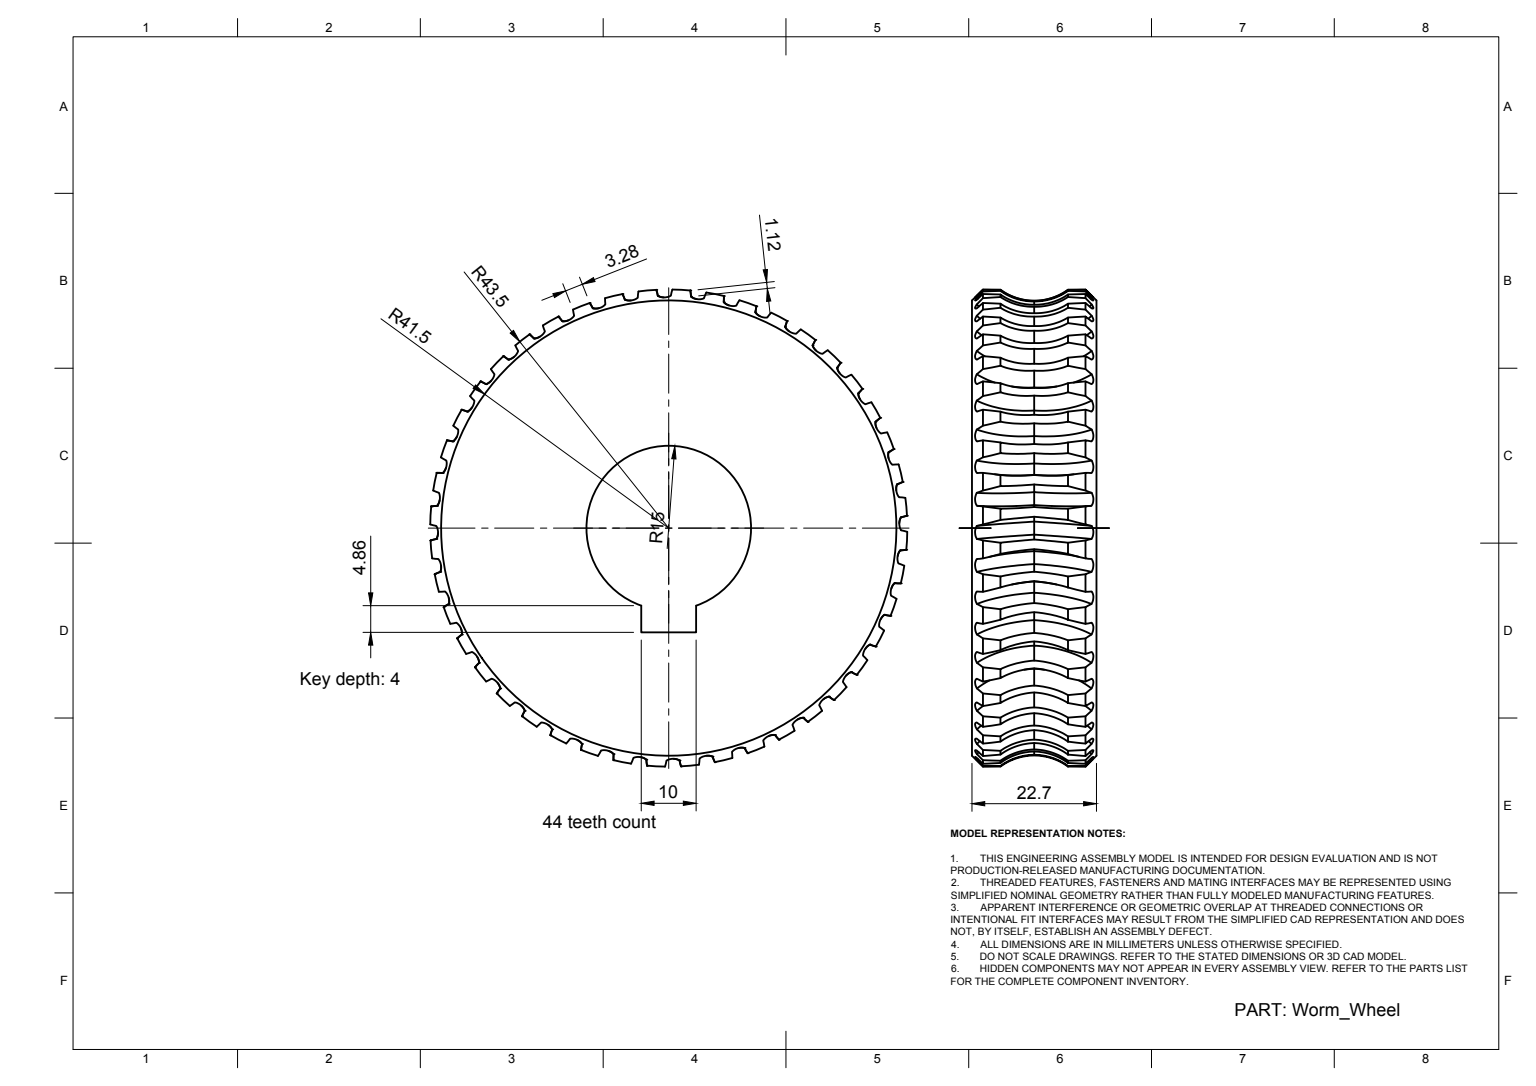
ISO-10303-21;
HEADER;
/* Generated by software containing ST-Developer
 * from STEP Tools, Inc. (www.steptools.com) 
 */

FILE_DESCRIPTION(
/* description */ ('STEP AP214'),
/* implementation_level */ '2;1');

FILE_NAME(
/* name */ 'Worm_Wheel.step',
/* time_stamp */ '2026-10-05T13:15:56-07:00',
/* author */ (''),
/* organization */ (''),
/* preprocessor_version */ 'ST-DEVELOPER v20.2',
/* originating_system */ 'Autodesk Translation Framework v15.15.0.0',
/* authorisation */ '');

FILE_SCHEMA (('AUTOMOTIVE_DESIGN { 1 0 10303 214 3 1 1 }'));
ENDSEC;

DATA;
#10=MECHANICAL_DESIGN_GEOMETRIC_PRESENTATION_REPRESENTATION('',(#1348),#37881);
#183=TOROIDAL_SURFACE('',#11111,52.,10.5);
#184=TOROIDAL_SURFACE('',#11114,52.,10.5);
#185=TOROIDAL_SURFACE('',#11117,52.,10.5);
#186=TOROIDAL_SURFACE('',#11120,52.,10.5);
#187=TOROIDAL_SURFACE('',#11123,52.,10.5);
#188=TOROIDAL_SURFACE('',#11126,52.,10.5);
#189=TOROIDAL_SURFACE('',#11129,52.,10.5);
#190=TOROIDAL_SURFACE('',#11132,52.,10.5);
#191=TOROIDAL_SURFACE('',#11135,52.,10.5);
#192=TOROIDAL_SURFACE('',#11138,52.,10.5);
#193=TOROIDAL_SURFACE('',#11141,52.,10.5);
#194=TOROIDAL_SURFACE('',#11144,52.,10.5);
#195=TOROIDAL_SURFACE('',#11147,52.,10.5);
#196=TOROIDAL_SURFACE('',#11150,52.,10.5);
#197=TOROIDAL_SURFACE('',#11153,52.,10.5);
#198=TOROIDAL_SURFACE('',#11156,52.,10.5);
#199=TOROIDAL_SURFACE('',#11159,52.,10.5);
#200=TOROIDAL_SURFACE('',#11162,52.,10.5);
#201=TOROIDAL_SURFACE('',#11165,52.,10.5);
#202=TOROIDAL_SURFACE('',#11168,52.,10.5);
#203=TOROIDAL_SURFACE('',#11171,52.,10.5);
#204=TOROIDAL_SURFACE('',#11174,52.,10.5);
#205=TOROIDAL_SURFACE('',#11177,52.,10.5);
#206=TOROIDAL_SURFACE('',#11180,52.,10.5);
#207=TOROIDAL_SURFACE('',#11183,52.,10.5);
#208=TOROIDAL_SURFACE('',#11186,52.,10.5);
#209=TOROIDAL_SURFACE('',#11189,52.,10.5);
#210=TOROIDAL_SURFACE('',#11192,52.,10.5);
#211=TOROIDAL_SURFACE('',#11195,52.,10.5);
#212=TOROIDAL_SURFACE('',#11198,52.,10.5);
#213=TOROIDAL_SURFACE('',#11201,52.,10.5);
#214=TOROIDAL_SURFACE('',#11204,52.,10.5);
#215=TOROIDAL_SURFACE('',#11207,52.,10.5);
#216=TOROIDAL_SURFACE('',#11210,52.,10.5);
#217=TOROIDAL_SURFACE('',#11213,52.,10.5);
#218=TOROIDAL_SURFACE('',#11216,52.,10.5);
#219=TOROIDAL_SURFACE('',#11219,52.,10.5);
#220=TOROIDAL_SURFACE('',#11222,52.,10.5);
#221=TOROIDAL_SURFACE('',#11225,52.,10.5);
#222=TOROIDAL_SURFACE('',#11228,52.,10.5);
#223=TOROIDAL_SURFACE('',#11231,52.,10.5);
#224=TOROIDAL_SURFACE('',#11234,52.,10.5);
#225=TOROIDAL_SURFACE('',#11237,52.,10.5);
#226=TOROIDAL_SURFACE('',#11240,52.,10.5);
#232=(
BOUNDED_CURVE()
B_SPLINE_CURVE(2,(#22947,#22948,#22949,#22950,#22951),.UNSPECIFIED.,.F.,
 .F.)
B_SPLINE_CURVE_WITH_KNOTS((3,2,3),(0.,0.25,0.459577358091282),
 .UNSPECIFIED.)
CURVE()
GEOMETRIC_REPRESENTATION_ITEM()
RATIONAL_B_SPLINE_CURVE((1.,0.974927912181824,1.,0.978981832292936,0.9932031210656))
REPRESENTATION_ITEM('')
);
#233=(
BOUNDED_CURVE()
B_SPLINE_CURVE(3,(#23082,#23083,#23084,#23085,#23086,#23087,#23088,#23089),
 .UNSPECIFIED.,.F.,.F.)
B_SPLINE_CURVE_WITH_KNOTS((4,2,2,4),(0.0783698293107414,0.308777371982556,
0.539184914655036,0.563918778704656),.UNSPECIFIED.)
CURVE()
GEOMETRIC_REPRESENTATION_ITEM()
RATIONAL_B_SPLINE_CURVE((1.,1.,1.,1.,1.,1.,1.,1.))
REPRESENTATION_ITEM('')
);
#234=(
BOUNDED_CURVE()
B_SPLINE_CURVE(2,(#23313,#23314,#23315,#23316,#23317),.UNSPECIFIED.,.F.,
 .F.)
B_SPLINE_CURVE_WITH_KNOTS((3,2,3),(0.,0.25,0.459577358091282),
 .UNSPECIFIED.)
CURVE()
GEOMETRIC_REPRESENTATION_ITEM()
RATIONAL_B_SPLINE_CURVE((1.,0.974927912181824,1.,0.978981832292936,0.9932031210656))
REPRESENTATION_ITEM('')
);
#235=(
BOUNDED_CURVE()
B_SPLINE_CURVE(2,(#23485,#23486,#23487,#23488,#23489),.UNSPECIFIED.,.F.,
 .F.)
B_SPLINE_CURVE_WITH_KNOTS((3,2,3),(0.,0.25,0.459577358091281),
 .UNSPECIFIED.)
CURVE()
GEOMETRIC_REPRESENTATION_ITEM()
RATIONAL_B_SPLINE_CURVE((1.,0.974927912181824,1.,0.978981832292936,0.9932031210656))
REPRESENTATION_ITEM('')
);
#236=(
BOUNDED_CURVE()
B_SPLINE_CURVE(2,(#23568,#23569,#23570,#23571,#23572),.UNSPECIFIED.,.F.,
 .F.)
B_SPLINE_CURVE_WITH_KNOTS((3,2,3),(0.,0.25,0.460808762537663),
 .UNSPECIFIED.)
CURVE()
GEOMETRIC_REPRESENTATION_ITEM()
RATIONAL_B_SPLINE_CURVE((1.,0.974927912181824,1.,0.978858336771259,0.993371456448429))
REPRESENTATION_ITEM('')
);
#237=(
BOUNDED_CURVE()
B_SPLINE_CURVE(2,(#23610,#23611,#23612,#23613,#23614),.UNSPECIFIED.,.F.,
 .F.)
B_SPLINE_CURVE_WITH_KNOTS((3,2,3),(0.,0.25,0.459577358091282),
 .UNSPECIFIED.)
CURVE()
GEOMETRIC_REPRESENTATION_ITEM()
RATIONAL_B_SPLINE_CURVE((1.,0.974927912181824,1.,0.978981832292936,0.9932031210656))
REPRESENTATION_ITEM('')
);
#238=(
BOUNDED_CURVE()
B_SPLINE_CURVE(2,(#23782,#23783,#23784,#23785,#23786),.UNSPECIFIED.,.F.,
 .F.)
B_SPLINE_CURVE_WITH_KNOTS((3,2,3),(0.,0.25,0.459577358091282),
 .UNSPECIFIED.)
CURVE()
GEOMETRIC_REPRESENTATION_ITEM()
RATIONAL_B_SPLINE_CURVE((1.,0.974927912181824,1.,0.978981832292936,0.9932031210656))
REPRESENTATION_ITEM('')
);
#239=(
BOUNDED_CURVE()
B_SPLINE_CURVE(2,(#23954,#23955,#23956,#23957,#23958),.UNSPECIFIED.,.F.,
 .F.)
B_SPLINE_CURVE_WITH_KNOTS((3,2,3),(0.,0.25,0.459577358091282),
 .UNSPECIFIED.)
CURVE()
GEOMETRIC_REPRESENTATION_ITEM()
RATIONAL_B_SPLINE_CURVE((1.,0.974927912181824,1.,0.978981832292936,0.9932031210656))
REPRESENTATION_ITEM('')
);
#240=(
BOUNDED_CURVE()
B_SPLINE_CURVE(2,(#24126,#24127,#24128,#24129,#24130),.UNSPECIFIED.,.F.,
 .F.)
B_SPLINE_CURVE_WITH_KNOTS((3,2,3),(0.,0.25,0.459577358091283),
 .UNSPECIFIED.)
CURVE()
GEOMETRIC_REPRESENTATION_ITEM()
RATIONAL_B_SPLINE_CURVE((1.,0.974927912181824,1.,0.978981832292936,0.9932031210656))
REPRESENTATION_ITEM('')
);
#241=(
BOUNDED_CURVE()
B_SPLINE_CURVE(2,(#24298,#24299,#24300,#24301,#24302),.UNSPECIFIED.,.F.,
 .F.)
B_SPLINE_CURVE_WITH_KNOTS((3,2,3),(0.,0.25,0.459577358091282),
 .UNSPECIFIED.)
CURVE()
GEOMETRIC_REPRESENTATION_ITEM()
RATIONAL_B_SPLINE_CURVE((1.,0.974927912181824,1.,0.978981832292936,0.9932031210656))
REPRESENTATION_ITEM('')
);
#242=(
BOUNDED_CURVE()
B_SPLINE_CURVE(2,(#24470,#24471,#24472,#24473,#24474),.UNSPECIFIED.,.F.,
 .F.)
B_SPLINE_CURVE_WITH_KNOTS((3,2,3),(0.,0.25,0.459577358091282),
 .UNSPECIFIED.)
CURVE()
GEOMETRIC_REPRESENTATION_ITEM()
RATIONAL_B_SPLINE_CURVE((1.,0.974927912181824,1.,0.978981832292936,0.9932031210656))
REPRESENTATION_ITEM('')
);
#243=(
BOUNDED_CURVE()
B_SPLINE_CURVE(2,(#24642,#24643,#24644,#24645,#24646),.UNSPECIFIED.,.F.,
 .F.)
B_SPLINE_CURVE_WITH_KNOTS((3,2,3),(0.,0.25,0.459577358091282),
 .UNSPECIFIED.)
CURVE()
GEOMETRIC_REPRESENTATION_ITEM()
RATIONAL_B_SPLINE_CURVE((1.,0.974927912181824,1.,0.978981832292936,0.9932031210656))
REPRESENTATION_ITEM('')
);
#244=(
BOUNDED_CURVE()
B_SPLINE_CURVE(2,(#24814,#24815,#24816,#24817,#24818),.UNSPECIFIED.,.F.,
 .F.)
B_SPLINE_CURVE_WITH_KNOTS((3,2,3),(0.,0.25,0.459577358091282),
 .UNSPECIFIED.)
CURVE()
GEOMETRIC_REPRESENTATION_ITEM()
RATIONAL_B_SPLINE_CURVE((1.,0.974927912181824,1.,0.978981832292936,0.9932031210656))
REPRESENTATION_ITEM('')
);
#245=(
BOUNDED_CURVE()
B_SPLINE_CURVE(2,(#24986,#24987,#24988,#24989,#24990),.UNSPECIFIED.,.F.,
 .F.)
B_SPLINE_CURVE_WITH_KNOTS((3,2,3),(0.,0.25,0.459577358091283),
 .UNSPECIFIED.)
CURVE()
GEOMETRIC_REPRESENTATION_ITEM()
RATIONAL_B_SPLINE_CURVE((1.,0.974927912181824,1.,0.978981832292936,0.9932031210656))
REPRESENTATION_ITEM('')
);
#246=(
BOUNDED_CURVE()
B_SPLINE_CURVE(2,(#25069,#25070,#25071,#25072,#25073),.UNSPECIFIED.,.F.,
 .F.)
B_SPLINE_CURVE_WITH_KNOTS((3,2,3),(0.,0.25,0.460808762537663),
 .UNSPECIFIED.)
CURVE()
GEOMETRIC_REPRESENTATION_ITEM()
RATIONAL_B_SPLINE_CURVE((1.,0.974927912181824,1.,0.978858336771258,0.993371456448429))
REPRESENTATION_ITEM('')
);
#247=(
BOUNDED_CURVE()
B_SPLINE_CURVE(2,(#25111,#25112,#25113,#25114,#25115),.UNSPECIFIED.,.F.,
 .F.)
B_SPLINE_CURVE_WITH_KNOTS((3,2,3),(0.,0.25,0.459577358091282),
 .UNSPECIFIED.)
CURVE()
GEOMETRIC_REPRESENTATION_ITEM()
RATIONAL_B_SPLINE_CURVE((1.,0.974927912181824,1.,0.978981832292936,0.9932031210656))
REPRESENTATION_ITEM('')
);
#248=(
BOUNDED_CURVE()
B_SPLINE_CURVE(2,(#25283,#25284,#25285,#25286,#25287),.UNSPECIFIED.,.F.,
 .F.)
B_SPLINE_CURVE_WITH_KNOTS((3,2,3),(0.,0.25,0.459577358091282),
 .UNSPECIFIED.)
CURVE()
GEOMETRIC_REPRESENTATION_ITEM()
RATIONAL_B_SPLINE_CURVE((1.,0.974927912181824,1.,0.978981832292936,0.9932031210656))
REPRESENTATION_ITEM('')
);
#249=(
BOUNDED_CURVE()
B_SPLINE_CURVE(2,(#25455,#25456,#25457,#25458,#25459),.UNSPECIFIED.,.F.,
 .F.)
B_SPLINE_CURVE_WITH_KNOTS((3,2,3),(0.,0.25,0.459577358091283),
 .UNSPECIFIED.)
CURVE()
GEOMETRIC_REPRESENTATION_ITEM()
RATIONAL_B_SPLINE_CURVE((1.,0.974927912181824,1.,0.978981832292936,0.9932031210656))
REPRESENTATION_ITEM('')
);
#250=(
BOUNDED_CURVE()
B_SPLINE_CURVE(2,(#25537,#25538,#25539,#25540,#25541),.UNSPECIFIED.,.F.,
 .F.)
B_SPLINE_CURVE_WITH_KNOTS((3,2,3),(0.,0.0714285714285714,0.131307816597586),
 .UNSPECIFIED.)
CURVE()
GEOMETRIC_REPRESENTATION_ITEM()
RATIONAL_B_SPLINE_CURVE((1.,0.974927912181824,1.,0.978981832292909,0.993203121065636))
REPRESENTATION_ITEM('')
);
#251=(
BOUNDED_CURVE()
B_SPLINE_CURVE(2,(#25581,#25582,#25583,#25584,#25585),.UNSPECIFIED.,.F.,
 .F.)
B_SPLINE_CURVE_WITH_KNOTS((3,2,3),(0.,0.0714285714285714,0.131659646439332),
 .UNSPECIFIED.)
CURVE()
GEOMETRIC_REPRESENTATION_ITEM()
RATIONAL_B_SPLINE_CURVE((1.,0.974927912181824,1.,0.978858336771259,0.993371456448429))
REPRESENTATION_ITEM('')
);
#252=(
BOUNDED_CURVE()
B_SPLINE_CURVE(2,(#25752,#25753,#25754,#25755,#25756),.UNSPECIFIED.,.F.,
 .F.)
B_SPLINE_CURVE_WITH_KNOTS((3,2,3),(0.,0.25,0.459577358091283),
 .UNSPECIFIED.)
CURVE()
GEOMETRIC_REPRESENTATION_ITEM()
RATIONAL_B_SPLINE_CURVE((1.,0.974927912181824,1.,0.978981832292936,0.9932031210656))
REPRESENTATION_ITEM('')
);
#253=(
BOUNDED_CURVE()
B_SPLINE_CURVE(2,(#25924,#25925,#25926,#25927,#25928),.UNSPECIFIED.,.F.,
 .F.)
B_SPLINE_CURVE_WITH_KNOTS((3,2,3),(0.,0.25,0.459577358091282),
 .UNSPECIFIED.)
CURVE()
GEOMETRIC_REPRESENTATION_ITEM()
RATIONAL_B_SPLINE_CURVE((1.,0.974927912181824,1.,0.978981832292936,0.9932031210656))
REPRESENTATION_ITEM('')
);
#254=(
BOUNDED_CURVE()
B_SPLINE_CURVE(2,(#26096,#26097,#26098,#26099,#26100),.UNSPECIFIED.,.F.,
 .F.)
B_SPLINE_CURVE_WITH_KNOTS((3,2,3),(0.,0.25,0.459577358091282),
 .UNSPECIFIED.)
CURVE()
GEOMETRIC_REPRESENTATION_ITEM()
RATIONAL_B_SPLINE_CURVE((1.,0.974927912181824,1.,0.978981832292936,0.9932031210656))
REPRESENTATION_ITEM('')
);
#255=(
BOUNDED_CURVE()
B_SPLINE_CURVE(2,(#26268,#26269,#26270,#26271,#26272),.UNSPECIFIED.,.F.,
 .F.)
B_SPLINE_CURVE_WITH_KNOTS((3,2,3),(0.,0.25,0.459577358091282),
 .UNSPECIFIED.)
CURVE()
GEOMETRIC_REPRESENTATION_ITEM()
RATIONAL_B_SPLINE_CURVE((1.,0.974927912181824,1.,0.978981832292936,0.9932031210656))
REPRESENTATION_ITEM('')
);
#256=(
BOUNDED_CURVE()
B_SPLINE_CURVE(2,(#26440,#26441,#26442,#26443,#26444),.UNSPECIFIED.,.F.,
 .F.)
B_SPLINE_CURVE_WITH_KNOTS((3,2,3),(0.,0.25,0.459577358091282),
 .UNSPECIFIED.)
CURVE()
GEOMETRIC_REPRESENTATION_ITEM()
RATIONAL_B_SPLINE_CURVE((1.,0.974927912181824,1.,0.978981832292936,0.9932031210656))
REPRESENTATION_ITEM('')
);
#257=(
BOUNDED_CURVE()
B_SPLINE_CURVE(2,(#26612,#26613,#26614,#26615,#26616),.UNSPECIFIED.,.F.,
 .F.)
B_SPLINE_CURVE_WITH_KNOTS((3,2,3),(0.,0.25,0.459577358091282),
 .UNSPECIFIED.)
CURVE()
GEOMETRIC_REPRESENTATION_ITEM()
RATIONAL_B_SPLINE_CURVE((1.,0.974927912181824,1.,0.978981832292936,0.9932031210656))
REPRESENTATION_ITEM('')
);
#258=(
BOUNDED_CURVE()
B_SPLINE_CURVE(2,(#26784,#26785,#26786,#26787,#26788),.UNSPECIFIED.,.F.,
 .F.)
B_SPLINE_CURVE_WITH_KNOTS((3,2,3),(0.,0.25,0.459577358091282),
 .UNSPECIFIED.)
CURVE()
GEOMETRIC_REPRESENTATION_ITEM()
RATIONAL_B_SPLINE_CURVE((1.,0.974927912181824,1.,0.978981832292936,0.9932031210656))
REPRESENTATION_ITEM('')
);
#259=(
BOUNDED_CURVE()
B_SPLINE_CURVE(2,(#26956,#26957,#26958,#26959,#26960),.UNSPECIFIED.,.F.,
 .F.)
B_SPLINE_CURVE_WITH_KNOTS((3,2,3),(0.,0.25,0.459577358091282),
 .UNSPECIFIED.)
CURVE()
GEOMETRIC_REPRESENTATION_ITEM()
RATIONAL_B_SPLINE_CURVE((1.,0.974927912181824,1.,0.978981832292936,0.9932031210656))
REPRESENTATION_ITEM('')
);
#260=(
BOUNDED_CURVE()
B_SPLINE_CURVE(2,(#27128,#27129,#27130,#27131,#27132),.UNSPECIFIED.,.F.,
 .F.)
B_SPLINE_CURVE_WITH_KNOTS((3,2,3),(0.,0.25,0.459577358091283),
 .UNSPECIFIED.)
CURVE()
GEOMETRIC_REPRESENTATION_ITEM()
RATIONAL_B_SPLINE_CURVE((1.,0.974927912181824,1.,0.978981832292936,0.9932031210656))
REPRESENTATION_ITEM('')
);
#261=(
BOUNDED_CURVE()
B_SPLINE_CURVE(2,(#27211,#27212,#27213,#27214,#27215),.UNSPECIFIED.,.F.,
 .F.)
B_SPLINE_CURVE_WITH_KNOTS((3,2,3),(0.,0.25,0.460808762537664),
 .UNSPECIFIED.)
CURVE()
GEOMETRIC_REPRESENTATION_ITEM()
RATIONAL_B_SPLINE_CURVE((1.,0.974927912181824,1.,0.978858336771258,0.993371456448429))
REPRESENTATION_ITEM('')
);
#262=(
BOUNDED_CURVE()
B_SPLINE_CURVE(2,(#27253,#27254,#27255,#27256,#27257),.UNSPECIFIED.,.F.,
 .F.)
B_SPLINE_CURVE_WITH_KNOTS((3,2,3),(0.,0.25,0.459577358091283),
 .UNSPECIFIED.)
CURVE()
GEOMETRIC_REPRESENTATION_ITEM()
RATIONAL_B_SPLINE_CURVE((1.,0.974927912181824,1.,0.978981832292936,0.9932031210656))
REPRESENTATION_ITEM('')
);
#263=(
BOUNDED_CURVE()
B_SPLINE_CURVE(2,(#27336,#27337,#27338,#27339,#27340),.UNSPECIFIED.,.F.,
 .F.)
B_SPLINE_CURVE_WITH_KNOTS((3,2,3),(0.,0.25,0.460808762537663),
 .UNSPECIFIED.)
CURVE()
GEOMETRIC_REPRESENTATION_ITEM()
RATIONAL_B_SPLINE_CURVE((1.,0.974927912181824,1.,0.978858336771258,0.993371456448429))
REPRESENTATION_ITEM('')
);
#264=(
BOUNDED_CURVE()
B_SPLINE_CURVE(2,(#27378,#27379,#27380,#27381,#27382),.UNSPECIFIED.,.F.,
 .F.)
B_SPLINE_CURVE_WITH_KNOTS((3,2,3),(0.,0.25,0.459577358091282),
 .UNSPECIFIED.)
CURVE()
GEOMETRIC_REPRESENTATION_ITEM()
RATIONAL_B_SPLINE_CURVE((1.,0.974927912181824,1.,0.978981832292936,0.9932031210656))
REPRESENTATION_ITEM('')
);
#265=(
BOUNDED_CURVE()
B_SPLINE_CURVE(2,(#27550,#27551,#27552,#27553,#27554),.UNSPECIFIED.,.F.,
 .F.)
B_SPLINE_CURVE_WITH_KNOTS((3,2,3),(0.,0.25,0.459577358091282),
 .UNSPECIFIED.)
CURVE()
GEOMETRIC_REPRESENTATION_ITEM()
RATIONAL_B_SPLINE_CURVE((1.,0.974927912181824,1.,0.978981832292936,0.9932031210656))
REPRESENTATION_ITEM('')
);
#266=(
BOUNDED_CURVE()
B_SPLINE_CURVE(2,(#27722,#27723,#27724,#27725,#27726),.UNSPECIFIED.,.F.,
 .F.)
B_SPLINE_CURVE_WITH_KNOTS((3,2,3),(0.,0.25,0.459577358091282),
 .UNSPECIFIED.)
CURVE()
GEOMETRIC_REPRESENTATION_ITEM()
RATIONAL_B_SPLINE_CURVE((1.,0.974927912181824,1.,0.978981832292936,0.9932031210656))
REPRESENTATION_ITEM('')
);
#267=(
BOUNDED_CURVE()
B_SPLINE_CURVE(2,(#27894,#27895,#27896,#27897,#27898),.UNSPECIFIED.,.F.,
 .F.)
B_SPLINE_CURVE_WITH_KNOTS((3,2,3),(0.,0.25,0.459577358091282),
 .UNSPECIFIED.)
CURVE()
GEOMETRIC_REPRESENTATION_ITEM()
RATIONAL_B_SPLINE_CURVE((1.,0.974927912181824,1.,0.978981832292936,0.9932031210656))
REPRESENTATION_ITEM('')
);
#268=(
BOUNDED_CURVE()
B_SPLINE_CURVE(2,(#28066,#28067,#28068,#28069,#28070),.UNSPECIFIED.,.F.,
 .F.)
B_SPLINE_CURVE_WITH_KNOTS((3,2,3),(0.,0.25,0.459577358091282),
 .UNSPECIFIED.)
CURVE()
GEOMETRIC_REPRESENTATION_ITEM()
RATIONAL_B_SPLINE_CURVE((1.,0.974927912181824,1.,0.978981832292936,0.9932031210656))
REPRESENTATION_ITEM('')
);
#269=(
BOUNDED_CURVE()
B_SPLINE_CURVE(2,(#28238,#28239,#28240,#28241,#28242),.UNSPECIFIED.,.F.,
 .F.)
B_SPLINE_CURVE_WITH_KNOTS((3,2,3),(0.,0.25,0.459577358091282),
 .UNSPECIFIED.)
CURVE()
GEOMETRIC_REPRESENTATION_ITEM()
RATIONAL_B_SPLINE_CURVE((1.,0.974927912181824,1.,0.978981832292936,0.9932031210656))
REPRESENTATION_ITEM('')
);
#270=(
BOUNDED_CURVE()
B_SPLINE_CURVE(2,(#28410,#28411,#28412,#28413,#28414),.UNSPECIFIED.,.F.,
 .F.)
B_SPLINE_CURVE_WITH_KNOTS((3,2,3),(0.,0.25,0.459577358091283),
 .UNSPECIFIED.)
CURVE()
GEOMETRIC_REPRESENTATION_ITEM()
RATIONAL_B_SPLINE_CURVE((1.,0.974927912181824,1.,0.978981832292936,0.9932031210656))
REPRESENTATION_ITEM('')
);
#271=(
BOUNDED_CURVE()
B_SPLINE_CURVE(2,(#28493,#28494,#28495,#28496,#28497),.UNSPECIFIED.,.F.,
 .F.)
B_SPLINE_CURVE_WITH_KNOTS((3,2,3),(0.,0.25,0.460808762537662),
 .UNSPECIFIED.)
CURVE()
GEOMETRIC_REPRESENTATION_ITEM()
RATIONAL_B_SPLINE_CURVE((1.,0.974927912181824,1.,0.978858336771259,0.993371456448429))
REPRESENTATION_ITEM('')
);
#272=(
BOUNDED_CURVE()
B_SPLINE_CURVE(2,(#28535,#28536,#28537,#28538,#28539),.UNSPECIFIED.,.F.,
 .F.)
B_SPLINE_CURVE_WITH_KNOTS((3,2,3),(0.,0.25,0.459577358091282),
 .UNSPECIFIED.)
CURVE()
GEOMETRIC_REPRESENTATION_ITEM()
RATIONAL_B_SPLINE_CURVE((1.,0.974927912181824,1.,0.978981832292936,0.9932031210656))
REPRESENTATION_ITEM('')
);
#273=(
BOUNDED_CURVE()
B_SPLINE_CURVE(2,(#28618,#28619,#28620,#28621,#28622),.UNSPECIFIED.,.F.,
 .F.)
B_SPLINE_CURVE_WITH_KNOTS((3,2,3),(0.,0.25,0.460808762537662),
 .UNSPECIFIED.)
CURVE()
GEOMETRIC_REPRESENTATION_ITEM()
RATIONAL_B_SPLINE_CURVE((1.,0.974927912181824,1.,0.978858336771259,0.993371456448429))
REPRESENTATION_ITEM('')
);
#274=(
BOUNDED_CURVE()
B_SPLINE_CURVE(2,(#28660,#28661,#28662,#28663,#28664),.UNSPECIFIED.,.F.,
 .F.)
B_SPLINE_CURVE_WITH_KNOTS((3,2,3),(0.,0.25,0.459577358091282),
 .UNSPECIFIED.)
CURVE()
GEOMETRIC_REPRESENTATION_ITEM()
RATIONAL_B_SPLINE_CURVE((1.,0.974927912181824,1.,0.978981832292936,0.9932031210656))
REPRESENTATION_ITEM('')
);
#275=(
BOUNDED_CURVE()
B_SPLINE_CURVE(2,(#28832,#28833,#28834,#28835,#28836),.UNSPECIFIED.,.F.,
 .F.)
B_SPLINE_CURVE_WITH_KNOTS((3,2,3),(0.,0.25,0.459577358091282),
 .UNSPECIFIED.)
CURVE()
GEOMETRIC_REPRESENTATION_ITEM()
RATIONAL_B_SPLINE_CURVE((1.,0.974927912181824,1.,0.978981832292936,0.9932031210656))
REPRESENTATION_ITEM('')
);
#276=(
BOUNDED_CURVE()
B_SPLINE_CURVE(2,(#29004,#29005,#29006,#29007,#29008),.UNSPECIFIED.,.F.,
 .F.)
B_SPLINE_CURVE_WITH_KNOTS((3,2,3),(0.,0.25,0.459577358091281),
 .UNSPECIFIED.)
CURVE()
GEOMETRIC_REPRESENTATION_ITEM()
RATIONAL_B_SPLINE_CURVE((1.,0.974927912181824,1.,0.978981832292936,0.9932031210656))
REPRESENTATION_ITEM('')
);
#277=(
BOUNDED_CURVE()
B_SPLINE_CURVE(2,(#29086,#29087,#29088,#29089,#29090),.UNSPECIFIED.,.F.,
 .F.)
B_SPLINE_CURVE_WITH_KNOTS((3,2,3),(0.,0.0714285714285714,0.131307816597586),
 .UNSPECIFIED.)
CURVE()
GEOMETRIC_REPRESENTATION_ITEM()
RATIONAL_B_SPLINE_CURVE((1.,0.974927912181824,1.,0.978981832292909,0.993203121065636))
REPRESENTATION_ITEM('')
);
#278=(
BOUNDED_CURVE()
B_SPLINE_CURVE(2,(#29130,#29131,#29132,#29133,#29134),.UNSPECIFIED.,.F.,
 .F.)
B_SPLINE_CURVE_WITH_KNOTS((3,2,3),(0.,0.0714285714285714,0.131659646439332),
 .UNSPECIFIED.)
CURVE()
GEOMETRIC_REPRESENTATION_ITEM()
RATIONAL_B_SPLINE_CURVE((1.,0.974927912181824,1.,0.978858336771259,0.993371456448429))
REPRESENTATION_ITEM('')
);
#279=(
BOUNDED_CURVE()
B_SPLINE_CURVE(2,(#29301,#29302,#29303,#29304,#29305),.UNSPECIFIED.,.F.,
 .F.)
B_SPLINE_CURVE_WITH_KNOTS((3,2,3),(0.,0.25,0.459577358091283),
 .UNSPECIFIED.)
CURVE()
GEOMETRIC_REPRESENTATION_ITEM()
RATIONAL_B_SPLINE_CURVE((1.,0.974927912181824,1.,0.978981832292936,0.9932031210656))
REPRESENTATION_ITEM('')
);
#280=(
BOUNDED_CURVE()
B_SPLINE_CURVE(2,(#29473,#29474,#29475,#29476,#29477),.UNSPECIFIED.,.F.,
 .F.)
B_SPLINE_CURVE_WITH_KNOTS((3,2,3),(0.,0.25,0.459577358091283),
 .UNSPECIFIED.)
CURVE()
GEOMETRIC_REPRESENTATION_ITEM()
RATIONAL_B_SPLINE_CURVE((1.,0.974927912181824,1.,0.978981832292936,0.9932031210656))
REPRESENTATION_ITEM('')
);
#281=(
BOUNDED_CURVE()
B_SPLINE_CURVE(2,(#29645,#29646,#29647,#29648,#29649),.UNSPECIFIED.,.F.,
 .F.)
B_SPLINE_CURVE_WITH_KNOTS((3,2,3),(0.,0.25,0.459577358091282),
 .UNSPECIFIED.)
CURVE()
GEOMETRIC_REPRESENTATION_ITEM()
RATIONAL_B_SPLINE_CURVE((1.,0.974927912181824,1.,0.978981832292936,0.9932031210656))
REPRESENTATION_ITEM('')
);
#282=(
BOUNDED_CURVE()
B_SPLINE_CURVE(2,(#29817,#29818,#29819,#29820,#29821),.UNSPECIFIED.,.F.,
 .F.)
B_SPLINE_CURVE_WITH_KNOTS((3,2,3),(0.,0.25,0.459577358091283),
 .UNSPECIFIED.)
CURVE()
GEOMETRIC_REPRESENTATION_ITEM()
RATIONAL_B_SPLINE_CURVE((1.,0.974927912181824,1.,0.978981832292936,0.9932031210656))
REPRESENTATION_ITEM('')
);
#283=(
BOUNDED_CURVE()
B_SPLINE_CURVE(2,(#29989,#29990,#29991,#29992,#29993),.UNSPECIFIED.,.F.,
 .F.)
B_SPLINE_CURVE_WITH_KNOTS((3,2,3),(0.,0.25,0.459577358091282),
 .UNSPECIFIED.)
CURVE()
GEOMETRIC_REPRESENTATION_ITEM()
RATIONAL_B_SPLINE_CURVE((1.,0.974927912181824,1.,0.978981832292936,0.9932031210656))
REPRESENTATION_ITEM('')
);
#284=(
BOUNDED_CURVE()
B_SPLINE_CURVE(2,(#30072,#30073,#30074,#30075,#30076),.UNSPECIFIED.,.F.,
 .F.)
B_SPLINE_CURVE_WITH_KNOTS((3,2,3),(0.,0.25,0.460808762537663),
 .UNSPECIFIED.)
CURVE()
GEOMETRIC_REPRESENTATION_ITEM()
RATIONAL_B_SPLINE_CURVE((1.,0.974927912181824,1.,0.978858336771258,0.993371456448429))
REPRESENTATION_ITEM('')
);
#285=(
BOUNDED_CURVE()
B_SPLINE_CURVE(2,(#30114,#30115,#30116,#30117,#30118),.UNSPECIFIED.,.F.,
 .F.)
B_SPLINE_CURVE_WITH_KNOTS((3,2,3),(0.,0.25,0.459577358091282),
 .UNSPECIFIED.)
CURVE()
GEOMETRIC_REPRESENTATION_ITEM()
RATIONAL_B_SPLINE_CURVE((1.,0.974927912181824,1.,0.978981832292936,0.9932031210656))
REPRESENTATION_ITEM('')
);
#286=(
BOUNDED_CURVE()
B_SPLINE_CURVE(3,(#30215,#30216,#30217,#30218,#30219,#30220,#30221,#30222),
 .UNSPECIFIED.,.F.,.F.)
B_SPLINE_CURVE_WITH_KNOTS((4,2,2,4),(0.0783698352504338,0.308777376437326,
0.539184917624882,0.563918781515205),.UNSPECIFIED.)
CURVE()
GEOMETRIC_REPRESENTATION_ITEM()
RATIONAL_B_SPLINE_CURVE((1.,1.,1.,1.,1.,1.,1.,1.))
REPRESENTATION_ITEM('')
);
#287=(
BOUNDED_CURVE()
B_SPLINE_CURVE(3,(#30375,#30376,#30377,#30378,#30379,#30380,#30381,#30382),
 .UNSPECIFIED.,.F.,.F.)
B_SPLINE_CURVE_WITH_KNOTS((4,2,2,4),(0.0783698388401176,0.308777379129589,
0.539184919419725,0.563918783213387),.UNSPECIFIED.)
CURVE()
GEOMETRIC_REPRESENTATION_ITEM()
RATIONAL_B_SPLINE_CURVE((1.,1.,1.,1.,1.,1.,1.,1.))
REPRESENTATION_ITEM('')
);
#288=(
BOUNDED_CURVE()
B_SPLINE_CURVE(3,(#30721,#30722,#30723,#30724,#30725,#30726,#30727,#30728),
 .UNSPECIFIED.,.F.,.F.)
B_SPLINE_CURVE_WITH_KNOTS((4,2,2,4),(0.0783698481609191,0.30877738612019,
0.539184924080125,0.563918787623825),.UNSPECIFIED.)
CURVE()
GEOMETRIC_REPRESENTATION_ITEM()
RATIONAL_B_SPLINE_CURVE((1.,1.,1.,1.,1.,1.,1.,1.))
REPRESENTATION_ITEM('')
);
#289=(
BOUNDED_CURVE()
B_SPLINE_CURVE(3,(#30881,#30882,#30883,#30884,#30885,#30886,#30887,#30888),
 .UNSPECIFIED.,.F.,.F.)
B_SPLINE_CURVE_WITH_KNOTS((4,2,2,4),(0.0783698504851113,0.308777387863334,
0.539184925242222,0.563918788723451),.UNSPECIFIED.)
CURVE()
GEOMETRIC_REPRESENTATION_ITEM()
RATIONAL_B_SPLINE_CURVE((1.,1.,1.,1.,1.,1.,1.,1.))
REPRESENTATION_ITEM('')
);
#290=(
BOUNDED_CURVE()
B_SPLINE_CURVE(3,(#31041,#31042,#31043,#31044,#31045,#31046,#31047,#31048),
 .UNSPECIFIED.,.F.,.F.)
B_SPLINE_CURVE_WITH_KNOTS((4,2,2,4),(0.0783698504851048,0.308777387863329,
0.539184925242218,0.563918788723618),.UNSPECIFIED.)
CURVE()
GEOMETRIC_REPRESENTATION_ITEM()
RATIONAL_B_SPLINE_CURVE((1.,1.,1.,1.,1.,1.,1.,1.))
REPRESENTATION_ITEM('')
);
#291=(
BOUNDED_CURVE()
B_SPLINE_CURVE(3,(#31201,#31202,#31203,#31204,#31205,#31206,#31207,#31208),
 .UNSPECIFIED.,.F.,.F.)
B_SPLINE_CURVE_WITH_KNOTS((4,2,2,4),(0.0783698481609166,0.308777386120188,
0.539184924080124,0.563918787623731),.UNSPECIFIED.)
CURVE()
GEOMETRIC_REPRESENTATION_ITEM()
RATIONAL_B_SPLINE_CURVE((1.,1.,1.,1.,1.,1.,1.,1.))
REPRESENTATION_ITEM('')
);
#292=(
BOUNDED_CURVE()
B_SPLINE_CURVE(3,(#31361,#31362,#31363,#31364,#31365,#31366,#31367,#31368),
 .UNSPECIFIED.,.F.,.F.)
B_SPLINE_CURVE_WITH_KNOTS((4,2,2,4),(0.0783698437311068,0.308777382797831,
0.539184921865219,0.56391878552778),.UNSPECIFIED.)
CURVE()
GEOMETRIC_REPRESENTATION_ITEM()
RATIONAL_B_SPLINE_CURVE((1.,1.,1.,1.,1.,1.,1.,1.))
REPRESENTATION_ITEM('')
);
#293=(
BOUNDED_CURVE()
B_SPLINE_CURVE(3,(#31521,#31522,#31523,#31524,#31525,#31526,#31527,#31528),
 .UNSPECIFIED.,.F.,.F.)
B_SPLINE_CURVE_WITH_KNOTS((4,2,2,4),(0.078369838840124,0.308777379129593,
0.539184919419728,0.563918783213485),.UNSPECIFIED.)
CURVE()
GEOMETRIC_REPRESENTATION_ITEM()
RATIONAL_B_SPLINE_CURVE((1.,1.,1.,1.,1.,1.,1.,1.))
REPRESENTATION_ITEM('')
);
#294=(
BOUNDED_CURVE()
B_SPLINE_CURVE(3,(#31681,#31682,#31683,#31684,#31685,#31686,#31687,#31688),
 .UNSPECIFIED.,.F.,.F.)
B_SPLINE_CURVE_WITH_KNOTS((4,2,2,4),(0.0783698352504276,0.308777376437321,
0.539184917624879,0.563918781514921),.UNSPECIFIED.)
CURVE()
GEOMETRIC_REPRESENTATION_ITEM()
RATIONAL_B_SPLINE_CURVE((1.,1.,1.,1.,1.,1.,1.,1.))
REPRESENTATION_ITEM('')
);
#295=(
BOUNDED_CURVE()
B_SPLINE_CURVE(3,(#31841,#31842,#31843,#31844,#31845,#31846,#31847,#31848),
 .UNSPECIFIED.,.F.,.F.)
B_SPLINE_CURVE_WITH_KNOTS((4,2,2,4),(0.0783698293107417,0.308777371982557,
0.539184914655036,0.563918778704716),.UNSPECIFIED.)
CURVE()
GEOMETRIC_REPRESENTATION_ITEM()
RATIONAL_B_SPLINE_CURVE((1.,1.,1.,1.,1.,1.,1.,1.))
REPRESENTATION_ITEM('')
);
#296=(
BOUNDED_CURVE()
B_SPLINE_CURVE(3,(#32187,#32188,#32189,#32190,#32191,#32192,#32193,#32194),
 .UNSPECIFIED.,.F.,.F.)
B_SPLINE_CURVE_WITH_KNOTS((4,2,2,4),(0.0783698388401176,0.308777379129589,
0.539184919419725,0.563918783213641),.UNSPECIFIED.)
CURVE()
GEOMETRIC_REPRESENTATION_ITEM()
RATIONAL_B_SPLINE_CURVE((1.,1.,1.,1.,1.,1.,1.,1.))
REPRESENTATION_ITEM('')
);
#297=(
BOUNDED_CURVE()
B_SPLINE_CURVE(3,(#32347,#32348,#32349,#32350,#32351,#32352,#32353,#32354),
 .UNSPECIFIED.,.F.,.F.)
B_SPLINE_CURVE_WITH_KNOTS((4,2,2,4),(0.0783698437311062,0.30877738279783,
0.539184921865219,0.563918785528064),.UNSPECIFIED.)
CURVE()
GEOMETRIC_REPRESENTATION_ITEM()
RATIONAL_B_SPLINE_CURVE((1.,1.,1.,1.,1.,1.,1.,1.))
REPRESENTATION_ITEM('')
);
#298=(
BOUNDED_CURVE()
B_SPLINE_CURVE(3,(#32499,#32500,#32501,#32502,#32503,#32504,#32505,#32506),
 .UNSPECIFIED.,.F.,.F.)
B_SPLINE_CURVE_WITH_KNOTS((4,2,2,4),(0.0783698481609152,0.308777386120187,
0.539184924080123,0.563918787623673),.UNSPECIFIED.)
CURVE()
GEOMETRIC_REPRESENTATION_ITEM()
RATIONAL_B_SPLINE_CURVE((1.,1.,1.,1.,1.,1.,1.,1.))
REPRESENTATION_ITEM('')
);
#299=(
BOUNDED_CURVE()
B_SPLINE_CURVE(3,(#32667,#32668,#32669,#32670,#32671,#32672,#32673,#32674),
 .UNSPECIFIED.,.F.,.F.)
B_SPLINE_CURVE_WITH_KNOTS((4,2,2,4),(0.0783698504851105,0.308777387863333,
0.539184925242221,0.563918788723755),.UNSPECIFIED.)
CURVE()
GEOMETRIC_REPRESENTATION_ITEM()
RATIONAL_B_SPLINE_CURVE((1.,1.,1.,1.,1.,1.,1.,1.))
REPRESENTATION_ITEM('')
);
#300=(
BOUNDED_CURVE()
B_SPLINE_CURVE(3,(#32827,#32828,#32829,#32830,#32831,#32832,#32833,#32834),
 .UNSPECIFIED.,.F.,.F.)
B_SPLINE_CURVE_WITH_KNOTS((4,2,2,4),(0.0783698504851009,0.308777387863326,
0.539184925242216,0.563918788723615),.UNSPECIFIED.)
CURVE()
GEOMETRIC_REPRESENTATION_ITEM()
RATIONAL_B_SPLINE_CURVE((1.,1.,1.,1.,1.,1.,1.,1.))
REPRESENTATION_ITEM('')
);
#301=(
BOUNDED_CURVE()
B_SPLINE_CURVE(3,(#32987,#32988,#32989,#32990,#32991,#32992,#32993,#32994),
 .UNSPECIFIED.,.F.,.F.)
B_SPLINE_CURVE_WITH_KNOTS((4,2,2,4),(0.0783698481609159,0.308777386120187,
0.539184924080124,0.563918787623773),.UNSPECIFIED.)
CURVE()
GEOMETRIC_REPRESENTATION_ITEM()
RATIONAL_B_SPLINE_CURVE((1.,1.,1.,1.,1.,1.,1.,1.))
REPRESENTATION_ITEM('')
);
#302=(
BOUNDED_CURVE()
B_SPLINE_CURVE(3,(#33147,#33148,#33149,#33150,#33151,#33152,#33153,#33154),
 .UNSPECIFIED.,.F.,.F.)
B_SPLINE_CURVE_WITH_KNOTS((4,2,2,4),(0.0783698437310911,0.308777382797819,
0.539184921865211,0.563918785527635),.UNSPECIFIED.)
CURVE()
GEOMETRIC_REPRESENTATION_ITEM()
RATIONAL_B_SPLINE_CURVE((1.,1.,1.,1.,1.,1.,1.,1.))
REPRESENTATION_ITEM('')
);
#303=(
BOUNDED_CURVE()
B_SPLINE_CURVE(3,(#33307,#33308,#33309,#33310,#33311,#33312,#33313,#33314),
 .UNSPECIFIED.,.F.,.F.)
B_SPLINE_CURVE_WITH_KNOTS((4,2,2,4),(0.0783698388401225,0.308777379129592,
0.539184919419727,0.563918783213193),.UNSPECIFIED.)
CURVE()
GEOMETRIC_REPRESENTATION_ITEM()
RATIONAL_B_SPLINE_CURVE((1.,1.,1.,1.,1.,1.,1.,1.))
REPRESENTATION_ITEM('')
);
#304=(
BOUNDED_CURVE()
B_SPLINE_CURVE(3,(#33467,#33468,#33469,#33470,#33471,#33472,#33473,#33474),
 .UNSPECIFIED.,.F.,.F.)
B_SPLINE_CURVE_WITH_KNOTS((4,2,2,4),(0.078369835250435,0.308777376437327,
0.539184917624883,0.563918781515067),.UNSPECIFIED.)
CURVE()
GEOMETRIC_REPRESENTATION_ITEM()
RATIONAL_B_SPLINE_CURVE((1.,1.,1.,1.,1.,1.,1.,1.))
REPRESENTATION_ITEM('')
);
#305=(
BOUNDED_CURVE()
B_SPLINE_CURVE(3,(#33627,#33628,#33629,#33630,#33631,#33632,#33633,#33634),
 .UNSPECIFIED.,.F.,.F.)
B_SPLINE_CURVE_WITH_KNOTS((4,2,2,4),(0.0783698293107414,0.308777371982556,
0.539184914655036,0.563918778704657),.UNSPECIFIED.)
CURVE()
GEOMETRIC_REPRESENTATION_ITEM()
RATIONAL_B_SPLINE_CURVE((1.,1.,1.,1.,1.,1.,1.,1.))
REPRESENTATION_ITEM('')
);
#306=(
BOUNDED_CURVE()
B_SPLINE_CURVE(3,(#33787,#33788,#33789,#33790,#33791,#33792,#33793,#33794),
 .UNSPECIFIED.,.F.,.F.)
B_SPLINE_CURVE_WITH_KNOTS((4,2,2,4),(0.0783698352504223,0.308777376437317,
0.539184917624877,0.563918781514814),.UNSPECIFIED.)
CURVE()
GEOMETRIC_REPRESENTATION_ITEM()
RATIONAL_B_SPLINE_CURVE((1.,1.,1.,1.,1.,1.,1.,1.))
REPRESENTATION_ITEM('')
);
#307=(
BOUNDED_CURVE()
B_SPLINE_CURVE(3,(#33947,#33948,#33949,#33950,#33951,#33952,#33953,#33954),
 .UNSPECIFIED.,.F.,.F.)
B_SPLINE_CURVE_WITH_KNOTS((4,2,2,4),(0.0783698388401235,0.308777379129593,
0.539184919419728,0.563918783213176),.UNSPECIFIED.)
CURVE()
GEOMETRIC_REPRESENTATION_ITEM()
RATIONAL_B_SPLINE_CURVE((1.,1.,1.,1.,1.,1.,1.,1.))
REPRESENTATION_ITEM('')
);
#308=(
BOUNDED_CURVE()
B_SPLINE_CURVE(3,(#34479,#34480,#34481,#34482,#34483,#34484,#34485,#34486),
 .UNSPECIFIED.,.F.,.F.)
B_SPLINE_CURVE_WITH_KNOTS((4,2,2,4),(0.0783698504850856,0.308777387863315,
0.539184925242209,0.56391878872357),.UNSPECIFIED.)
CURVE()
GEOMETRIC_REPRESENTATION_ITEM()
RATIONAL_B_SPLINE_CURVE((1.,1.,1.,1.,1.,1.,1.,1.))
REPRESENTATION_ITEM('')
);
#309=(
BOUNDED_CURVE()
B_SPLINE_CURVE(3,(#34639,#34640,#34641,#34642,#34643,#34644,#34645,#34646),
 .UNSPECIFIED.,.F.,.F.)
B_SPLINE_CURVE_WITH_KNOTS((4,2,2,4),(0.0783698504851055,0.30877738786333,
0.539184925242219,0.563918788723501),.UNSPECIFIED.)
CURVE()
GEOMETRIC_REPRESENTATION_ITEM()
RATIONAL_B_SPLINE_CURVE((1.,1.,1.,1.,1.,1.,1.,1.))
REPRESENTATION_ITEM('')
);
#310=(
BOUNDED_CURVE()
B_SPLINE_CURVE(3,(#34799,#34800,#34801,#34802,#34803,#34804,#34805,#34806),
 .UNSPECIFIED.,.F.,.F.)
B_SPLINE_CURVE_WITH_KNOTS((4,2,2,4),(0.0783698481609002,0.308777386120176,
0.539184924080116,0.563918787623726),.UNSPECIFIED.)
CURVE()
GEOMETRIC_REPRESENTATION_ITEM()
RATIONAL_B_SPLINE_CURVE((1.,1.,1.,1.,1.,1.,1.,1.))
REPRESENTATION_ITEM('')
);
#311=(
BOUNDED_CURVE()
B_SPLINE_CURVE(3,(#34959,#34960,#34961,#34962,#34963,#34964,#34965,#34966),
 .UNSPECIFIED.,.F.,.F.)
B_SPLINE_CURVE_WITH_KNOTS((4,2,2,4),(0.0783698437310988,0.308777382797825,
0.539184921865215,0.563918785527758),.UNSPECIFIED.)
CURVE()
GEOMETRIC_REPRESENTATION_ITEM()
RATIONAL_B_SPLINE_CURVE((1.,1.,1.,1.,1.,1.,1.,1.))
REPRESENTATION_ITEM('')
);
#312=(
BOUNDED_CURVE()
B_SPLINE_CURVE(3,(#35119,#35120,#35121,#35122,#35123,#35124,#35125,#35126),
 .UNSPECIFIED.,.F.,.F.)
B_SPLINE_CURVE_WITH_KNOTS((4,2,2,4),(0.078369838840116,0.308777379129587,
0.539184919419724,0.563918783213258),.UNSPECIFIED.)
CURVE()
GEOMETRIC_REPRESENTATION_ITEM()
RATIONAL_B_SPLINE_CURVE((1.,1.,1.,1.,1.,1.,1.,1.))
REPRESENTATION_ITEM('')
);
#313=(
BOUNDED_CURVE()
B_SPLINE_CURVE(3,(#35279,#35280,#35281,#35282,#35283,#35284,#35285,#35286),
 .UNSPECIFIED.,.F.,.F.)
B_SPLINE_CURVE_WITH_KNOTS((4,2,2,4),(0.0783698352504284,0.308777376437322,
0.53918491762488,0.563918781514946),.UNSPECIFIED.)
CURVE()
GEOMETRIC_REPRESENTATION_ITEM()
RATIONAL_B_SPLINE_CURVE((1.,1.,1.,1.,1.,1.,1.,1.))
REPRESENTATION_ITEM('')
);
#314=(
BOUNDED_CURVE()
B_SPLINE_CURVE(3,(#35811,#35812,#35813,#35814,#35815,#35816,#35817,#35818),
 .UNSPECIFIED.,.F.,.F.)
B_SPLINE_CURVE_WITH_KNOTS((4,2,2,4),(0.078369838840114,0.308777379129586,
0.539184919419723,0.56391878321367),.UNSPECIFIED.)
CURVE()
GEOMETRIC_REPRESENTATION_ITEM()
RATIONAL_B_SPLINE_CURVE((1.,1.,1.,1.,1.,1.,1.,1.))
REPRESENTATION_ITEM('')
);
#315=(
BOUNDED_CURVE()
B_SPLINE_CURVE(3,(#35971,#35972,#35973,#35974,#35975,#35976,#35977,#35978),
 .UNSPECIFIED.,.F.,.F.)
B_SPLINE_CURVE_WITH_KNOTS((4,2,2,4),(0.078369843731106,0.30877738279783,
0.539184921865219,0.563918785527521),.UNSPECIFIED.)
CURVE()
GEOMETRIC_REPRESENTATION_ITEM()
RATIONAL_B_SPLINE_CURVE((1.,1.,1.,1.,1.,1.,1.,1.))
REPRESENTATION_ITEM('')
);
#316=(
BOUNDED_CURVE()
B_SPLINE_CURVE(3,(#36123,#36124,#36125,#36126,#36127,#36128,#36129,#36130),
 .UNSPECIFIED.,.F.,.F.)
B_SPLINE_CURVE_WITH_KNOTS((4,2,2,4),(0.0783698481609171,0.308777386120188,
0.539184924080125,0.563918787623751),.UNSPECIFIED.)
CURVE()
GEOMETRIC_REPRESENTATION_ITEM()
RATIONAL_B_SPLINE_CURVE((1.,1.,1.,1.,1.,1.,1.,1.))
REPRESENTATION_ITEM('')
);
#317=(
BOUNDED_CURVE()
B_SPLINE_CURVE(3,(#36291,#36292,#36293,#36294,#36295,#36296,#36297,#36298),
 .UNSPECIFIED.,.F.,.F.)
B_SPLINE_CURVE_WITH_KNOTS((4,2,2,4),(0.0783698504850854,0.308777387863314,
0.539184925242208,0.563918788723659),.UNSPECIFIED.)
CURVE()
GEOMETRIC_REPRESENTATION_ITEM()
RATIONAL_B_SPLINE_CURVE((1.,1.,1.,1.,1.,1.,1.,1.))
REPRESENTATION_ITEM('')
);
#318=(
BOUNDED_CURVE()
B_SPLINE_CURVE(3,(#36451,#36452,#36453,#36454,#36455,#36456,#36457,#36458),
 .UNSPECIFIED.,.F.,.F.)
B_SPLINE_CURVE_WITH_KNOTS((4,2,2,4),(0.0783698504851048,0.308777387863329,
0.539184925242218,0.563918788723504),.UNSPECIFIED.)
CURVE()
GEOMETRIC_REPRESENTATION_ITEM()
RATIONAL_B_SPLINE_CURVE((1.,1.,1.,1.,1.,1.,1.,1.))
REPRESENTATION_ITEM('')
);
#319=(
BOUNDED_CURVE()
B_SPLINE_CURVE(3,(#36611,#36612,#36613,#36614,#36615,#36616,#36617,#36618),
 .UNSPECIFIED.,.F.,.F.)
B_SPLINE_CURVE_WITH_KNOTS((4,2,2,4),(0.0783698481609187,0.30877738612019,
0.539184924080125,0.563918787623611),.UNSPECIFIED.)
CURVE()
GEOMETRIC_REPRESENTATION_ITEM()
RATIONAL_B_SPLINE_CURVE((1.,1.,1.,1.,1.,1.,1.,1.))
REPRESENTATION_ITEM('')
);
#320=(
BOUNDED_CURVE()
B_SPLINE_CURVE(3,(#36771,#36772,#36773,#36774,#36775,#36776,#36777,#36778),
 .UNSPECIFIED.,.F.,.F.)
B_SPLINE_CURVE_WITH_KNOTS((4,2,2,4),(0.0783698437311103,0.308777382797833,
0.539184921865221,0.563918785527852),.UNSPECIFIED.)
CURVE()
GEOMETRIC_REPRESENTATION_ITEM()
RATIONAL_B_SPLINE_CURVE((1.,1.,1.,1.,1.,1.,1.,1.))
REPRESENTATION_ITEM('')
);
#321=(
BOUNDED_CURVE()
B_SPLINE_CURVE(3,(#36931,#36932,#36933,#36934,#36935,#36936,#36937,#36938),
 .UNSPECIFIED.,.F.,.F.)
B_SPLINE_CURVE_WITH_KNOTS((4,2,2,4),(0.0783698388401129,0.308777379129585,
0.539184919419723,0.563918783213525),.UNSPECIFIED.)
CURVE()
GEOMETRIC_REPRESENTATION_ITEM()
RATIONAL_B_SPLINE_CURVE((1.,1.,1.,1.,1.,1.,1.,1.))
REPRESENTATION_ITEM('')
);
#328=(
BOUNDED_SURFACE()
B_SPLINE_SURFACE(3,2,((#22854,#22855,#22856,#22857,#22858,#22859,#22860,
#22861,#22862),(#22863,#22864,#22865,#22866,#22867,#22868,#22869,#22870,
#22871),(#22872,#22873,#22874,#22875,#22876,#22877,#22878,#22879,#22880),
(#22881,#22882,#22883,#22884,#22885,#22886,#22887,#22888,#22889)),
 .UNSPECIFIED.,.F.,.F.,.F.)
B_SPLINE_SURFACE_WITH_KNOTS((4,4),(3,2,2,2,3),(0.,1.),(0.,0.25,0.5,0.75,
1.),.UNSPECIFIED.)
GEOMETRIC_REPRESENTATION_ITEM()
RATIONAL_B_SPLINE_SURFACE(((1.,0.974927912181824,1.,0.974927912181824,1.,
0.974927912181824,1.,0.974927912181824,1.),(0.833333333333332,0.812439926818185,
0.833333333333332,0.812439926818185,0.833333333333332,0.812439926818185,
0.833333333333332,0.812439926818185,0.833333333333332),(0.833333333333332,
0.812439926818185,0.833333333333332,0.812439926818185,0.833333333333332,
0.812439926818185,0.833333333333332,0.812439926818185,0.833333333333332),
(1.,0.974927912181824,1.,0.974927912181824,1.,0.974927912181824,1.,0.974927912181824,
1.)))
REPRESENTATION_ITEM('')
SURFACE()
);
#329=(
BOUNDED_SURFACE()
B_SPLINE_SURFACE(3,2,((#22952,#22953,#22954,#22955,#22956,#22957,#22958,
#22959,#22960),(#22961,#22962,#22963,#22964,#22965,#22966,#22967,#22968,
#22969),(#22970,#22971,#22972,#22973,#22974,#22975,#22976,#22977,#22978),
(#22979,#22980,#22981,#22982,#22983,#22984,#22985,#22986,#22987)),
 .UNSPECIFIED.,.F.,.F.,.F.)
B_SPLINE_SURFACE_WITH_KNOTS((4,4),(3,2,2,2,3),(0.,1.),(0.,0.25,0.5,0.75,
1.),.UNSPECIFIED.)
GEOMETRIC_REPRESENTATION_ITEM()
RATIONAL_B_SPLINE_SURFACE(((1.,0.974927912181824,1.,0.974927912181824,1.,
0.974927912181824,1.,0.974927912181824,1.),(0.987189825241073,0.962438915249418,
0.987189825241073,0.962438915249418,0.987189825241073,0.962438915249418,
0.987189825241073,0.962438915249418,0.987189825241073),(0.987189825241073,
0.962438915249418,0.987189825241073,0.962438915249418,0.987189825241073,
0.962438915249418,0.987189825241073,0.962438915249418,0.987189825241073),
(1.,0.974927912181824,1.,0.974927912181824,1.,0.974927912181824,1.,0.974927912181824,
1.)))
REPRESENTATION_ITEM('')
SURFACE()
);
#330=(
BOUNDED_SURFACE()
B_SPLINE_SURFACE(3,2,((#22989,#22990,#22991,#22992,#22993,#22994,#22995,
#22996,#22997),(#22998,#22999,#23000,#23001,#23002,#23003,#23004,#23005,
#23006),(#23007,#23008,#23009,#23010,#23011,#23012,#23013,#23014,#23015),
(#23016,#23017,#23018,#23019,#23020,#23021,#23022,#23023,#23024)),
 .UNSPECIFIED.,.F.,.F.,.F.)
B_SPLINE_SURFACE_WITH_KNOTS((4,4),(3,2,2,2,3),(0.,1.),(0.,0.25,0.5,0.75,
1.),.UNSPECIFIED.)
GEOMETRIC_REPRESENTATION_ITEM()
RATIONAL_B_SPLINE_SURFACE(((1.,0.974927912181824,1.,0.974927912181824,1.,
0.974927912181824,1.,0.974927912181824,1.),(0.987189825241073,0.962438915249418,
0.987189825241073,0.962438915249418,0.987189825241073,0.962438915249418,
0.987189825241073,0.962438915249418,0.987189825241073),(0.987189825241073,
0.962438915249418,0.987189825241073,0.962438915249418,0.987189825241073,
0.962438915249418,0.987189825241073,0.962438915249418,0.987189825241073),
(1.,0.974927912181824,1.,0.974927912181824,1.,0.974927912181824,1.,0.974927912181824,
1.)))
REPRESENTATION_ITEM('')
SURFACE()
);
#331=(
BOUNDED_SURFACE()
B_SPLINE_SURFACE(3,3,((#23026,#23027,#23028,#23029,#23030,#23031,#23032,
#23033,#23034,#23035,#23036,#23037),(#23038,#23039,#23040,#23041,#23042,
#23043,#23044,#23045,#23046,#23047,#23048,#23049),(#23050,#23051,#23052,
#23053,#23054,#23055,#23056,#23057,#23058,#23059,#23060,#23061),(#23062,
#23063,#23064,#23065,#23066,#23067,#23068,#23069,#23070,#23071,#23072,#23073)),
 .UNSPECIFIED.,.F.,.F.,.F.)
B_SPLINE_SURFACE_WITH_KNOTS((4,4),(4,2,2,2,2,4),(0.,1.),(0.,0.0783698293107414,
0.308777371982556,0.539184914655036,0.769592457327518,1.),.UNSPECIFIED.)
GEOMETRIC_REPRESENTATION_ITEM()
RATIONAL_B_SPLINE_SURFACE(((1.,1.,1.,1.,1.,1.,1.,1.,1.,1.,1.,1.),(0.833333333333332,
0.833333333333332,0.833333333333332,0.833333333333332,0.833333333333332,
0.833333333333332,0.833333333333332,0.833333333333332,0.833333333333332,
0.833333333333332,0.833333333333332,0.833333333333332),(0.833333333333332,
0.833333333333332,0.833333333333332,0.833333333333332,0.833333333333332,
0.833333333333332,0.833333333333332,0.833333333333332,0.833333333333332,
0.833333333333332,0.833333333333332,0.833333333333332),(1.,1.,1.,1.,1.,
1.,1.,1.,1.,1.,1.,1.)))
REPRESENTATION_ITEM('')
SURFACE()
);
#332=(
BOUNDED_SURFACE()
B_SPLINE_SURFACE(3,3,((#23090,#23091,#23092,#23093,#23094,#23095,#23096,
#23097,#23098,#23099,#23100,#23101),(#23102,#23103,#23104,#23105,#23106,
#23107,#23108,#23109,#23110,#23111,#23112,#23113),(#23114,#23115,#23116,
#23117,#23118,#23119,#23120,#23121,#23122,#23123,#23124,#23125),(#23126,
#23127,#23128,#23129,#23130,#23131,#23132,#23133,#23134,#23135,#23136,#23137)),
 .UNSPECIFIED.,.F.,.F.,.F.)
B_SPLINE_SURFACE_WITH_KNOTS((4,4),(4,2,2,2,2,4),(0.,1.),(0.,0.0783698293107414,
0.308777371982556,0.539184914655036,0.769592457327518,1.),.UNSPECIFIED.)
GEOMETRIC_REPRESENTATION_ITEM()
RATIONAL_B_SPLINE_SURFACE(((1.,1.,1.,1.,1.,1.,1.,1.,1.,1.,1.,1.),(0.987189825241073,
0.987189825241073,0.987189825241073,0.987189825241073,0.987189825241073,
0.987189825241073,0.987189825241073,0.987189825241073,0.987189825241073,
0.987189825241073,0.987189825241073,0.987189825241073),(0.987189825241073,
0.987189825241073,0.987189825241073,0.987189825241073,0.987189825241073,
0.987189825241073,0.987189825241073,0.987189825241073,0.987189825241073,
0.987189825241073,0.987189825241073,0.987189825241073),(1.,1.,1.,1.,1.,
1.,1.,1.,1.,1.,1.,1.)))
REPRESENTATION_ITEM('')
SURFACE()
);
#333=(
BOUNDED_SURFACE()
B_SPLINE_SURFACE(3,3,((#23138,#23139,#23140,#23141,#23142,#23143,#23144,
#23145,#23146,#23147,#23148,#23149),(#23150,#23151,#23152,#23153,#23154,
#23155,#23156,#23157,#23158,#23159,#23160,#23161),(#23162,#23163,#23164,
#23165,#23166,#23167,#23168,#23169,#23170,#23171,#23172,#23173),(#23174,
#23175,#23176,#23177,#23178,#23179,#23180,#23181,#23182,#23183,#23184,#23185)),
 .UNSPECIFIED.,.F.,.F.,.F.)
B_SPLINE_SURFACE_WITH_KNOTS((4,4),(4,2,2,2,2,4),(0.,1.),(0.,0.0783698293107414,
0.308777371982556,0.539184914655036,0.769592457327518,1.),.UNSPECIFIED.)
GEOMETRIC_REPRESENTATION_ITEM()
RATIONAL_B_SPLINE_SURFACE(((1.,1.,1.,1.,1.,1.,1.,1.,1.,1.,1.,1.),(0.987189825241073,
0.987189825241073,0.987189825241073,0.987189825241073,0.987189825241073,
0.987189825241073,0.987189825241073,0.987189825241073,0.987189825241073,
0.987189825241073,0.987189825241073,0.987189825241073),(0.987189825241073,
0.987189825241073,0.987189825241073,0.987189825241073,0.987189825241073,
0.987189825241073,0.987189825241073,0.987189825241073,0.987189825241073,
0.987189825241073,0.987189825241073,0.987189825241073),(1.,1.,1.,1.,1.,
1.,1.,1.,1.,1.,1.,1.)))
REPRESENTATION_ITEM('')
SURFACE()
);
#334=(
BOUNDED_SURFACE()
B_SPLINE_SURFACE(3,2,((#23186,#23187,#23188,#23189,#23190,#23191,#23192,
#23193,#23194),(#23195,#23196,#23197,#23198,#23199,#23200,#23201,#23202,
#23203),(#23204,#23205,#23206,#23207,#23208,#23209,#23210,#23211,#23212),
(#23213,#23214,#23215,#23216,#23217,#23218,#23219,#23220,#23221)),
 .UNSPECIFIED.,.F.,.F.,.F.)
B_SPLINE_SURFACE_WITH_KNOTS((4,4),(3,2,2,2,3),(0.,1.),(0.,0.25,0.5,0.75,
1.),.UNSPECIFIED.)
GEOMETRIC_REPRESENTATION_ITEM()
RATIONAL_B_SPLINE_SURFACE(((1.,0.974927912181824,1.,0.974927912181824,1.,
0.974927912181824,1.,0.974927912181824,1.),(0.987189825241073,0.962438915249418,
0.987189825241073,0.962438915249418,0.987189825241073,0.962438915249418,
0.987189825241073,0.962438915249418,0.987189825241073),(0.987189825241073,
0.962438915249418,0.987189825241073,0.962438915249418,0.987189825241073,
0.962438915249418,0.987189825241073,0.962438915249418,0.987189825241073),
(1.,0.974927912181824,1.,0.974927912181824,1.,0.974927912181824,1.,0.974927912181824,
1.)))
REPRESENTATION_ITEM('')
SURFACE()
);
#335=(
BOUNDED_SURFACE()
B_SPLINE_SURFACE(3,2,((#23276,#23277,#23278,#23279,#23280,#23281,#23282,
#23283,#23284),(#23285,#23286,#23287,#23288,#23289,#23290,#23291,#23292,
#23293),(#23294,#23295,#23296,#23297,#23298,#23299,#23300,#23301,#23302),
(#23303,#23304,#23305,#23306,#23307,#23308,#23309,#23310,#23311)),
 .UNSPECIFIED.,.F.,.F.,.F.)
B_SPLINE_SURFACE_WITH_KNOTS((4,4),(3,2,2,2,3),(0.,1.),(0.,0.25,0.5,0.75,
1.),.UNSPECIFIED.)
GEOMETRIC_REPRESENTATION_ITEM()
RATIONAL_B_SPLINE_SURFACE(((1.,0.974927912181824,1.,0.974927912181824,1.,
0.974927912181824,1.,0.974927912181824,1.),(0.987189825241073,0.962438915249418,
0.987189825241073,0.962438915249418,0.987189825241073,0.962438915249418,
0.987189825241073,0.962438915249418,0.987189825241073),(0.987189825241073,
0.962438915249418,0.987189825241073,0.962438915249418,0.987189825241073,
0.962438915249418,0.987189825241073,0.962438915249418,0.987189825241073),
(1.,0.974927912181824,1.,0.974927912181824,1.,0.974927912181824,1.,0.974927912181824,
1.)))
REPRESENTATION_ITEM('')
SURFACE()
);
#336=(
BOUNDED_SURFACE()
B_SPLINE_SURFACE(3,2,((#23319,#23320,#23321,#23322,#23323,#23324,#23325,
#23326,#23327),(#23328,#23329,#23330,#23331,#23332,#23333,#23334,#23335,
#23336),(#23337,#23338,#23339,#23340,#23341,#23342,#23343,#23344,#23345),
(#23346,#23347,#23348,#23349,#23350,#23351,#23352,#23353,#23354)),
 .UNSPECIFIED.,.F.,.F.,.F.)
B_SPLINE_SURFACE_WITH_KNOTS((4,4),(3,2,2,2,3),(0.,1.),(0.,0.25,0.5,0.75,
1.),.UNSPECIFIED.)
GEOMETRIC_REPRESENTATION_ITEM()
RATIONAL_B_SPLINE_SURFACE(((1.,0.974927912181824,1.,0.974927912181824,1.,
0.974927912181824,1.,0.974927912181824,1.),(0.833333333333332,0.812439926818185,
0.833333333333332,0.812439926818185,0.833333333333332,0.812439926818185,
0.833333333333332,0.812439926818185,0.833333333333332),(0.833333333333332,
0.812439926818185,0.833333333333332,0.812439926818185,0.833333333333332,
0.812439926818185,0.833333333333332,0.812439926818185,0.833333333333332),
(1.,0.974927912181824,1.,0.974927912181824,1.,0.974927912181824,1.,0.974927912181824,
1.)))
REPRESENTATION_ITEM('')
SURFACE()
);
#337=(
BOUNDED_SURFACE()
B_SPLINE_SURFACE(3,2,((#23358,#23359,#23360,#23361,#23362,#23363,#23364,
#23365,#23366),(#23367,#23368,#23369,#23370,#23371,#23372,#23373,#23374,
#23375),(#23376,#23377,#23378,#23379,#23380,#23381,#23382,#23383,#23384),
(#23385,#23386,#23387,#23388,#23389,#23390,#23391,#23392,#23393)),
 .UNSPECIFIED.,.F.,.F.,.F.)
B_SPLINE_SURFACE_WITH_KNOTS((4,4),(3,2,2,2,3),(0.,1.),(0.,0.25,0.5,0.75,
1.),.UNSPECIFIED.)
GEOMETRIC_REPRESENTATION_ITEM()
RATIONAL_B_SPLINE_SURFACE(((1.,0.974927912181824,1.,0.974927912181824,1.,
0.974927912181824,1.,0.974927912181824,1.),(0.987189825241073,0.962438915249418,
0.987189825241073,0.962438915249418,0.987189825241073,0.962438915249418,
0.987189825241073,0.962438915249418,0.987189825241073),(0.987189825241073,
0.962438915249418,0.987189825241073,0.962438915249418,0.987189825241073,
0.962438915249418,0.987189825241073,0.962438915249418,0.987189825241073),
(1.,0.974927912181824,1.,0.974927912181824,1.,0.974927912181824,1.,0.974927912181824,
1.)))
REPRESENTATION_ITEM('')
SURFACE()
);
#338=(
BOUNDED_SURFACE()
B_SPLINE_SURFACE(3,2,((#23448,#23449,#23450,#23451,#23452,#23453,#23454,
#23455,#23456),(#23457,#23458,#23459,#23460,#23461,#23462,#23463,#23464,
#23465),(#23466,#23467,#23468,#23469,#23470,#23471,#23472,#23473,#23474),
(#23475,#23476,#23477,#23478,#23479,#23480,#23481,#23482,#23483)),
 .UNSPECIFIED.,.F.,.F.,.F.)
B_SPLINE_SURFACE_WITH_KNOTS((4,4),(3,2,2,2,3),(0.,1.),(0.,0.25,0.5,0.75,
1.),.UNSPECIFIED.)
GEOMETRIC_REPRESENTATION_ITEM()
RATIONAL_B_SPLINE_SURFACE(((1.,0.974927912181824,1.,0.974927912181824,1.,
0.974927912181824,1.,0.974927912181824,1.),(0.987189825241073,0.962438915249418,
0.987189825241073,0.962438915249418,0.987189825241073,0.962438915249418,
0.987189825241073,0.962438915249418,0.987189825241073),(0.987189825241073,
0.962438915249418,0.987189825241073,0.962438915249418,0.987189825241073,
0.962438915249418,0.987189825241073,0.962438915249418,0.987189825241073),
(1.,0.974927912181824,1.,0.974927912181824,1.,0.974927912181824,1.,0.974927912181824,
1.)))
REPRESENTATION_ITEM('')
SURFACE()
);
#339=(
BOUNDED_SURFACE()
B_SPLINE_SURFACE(3,2,((#23491,#23492,#23493,#23494,#23495,#23496,#23497,
#23498,#23499),(#23500,#23501,#23502,#23503,#23504,#23505,#23506,#23507,
#23508),(#23509,#23510,#23511,#23512,#23513,#23514,#23515,#23516,#23517),
(#23518,#23519,#23520,#23521,#23522,#23523,#23524,#23525,#23526)),
 .UNSPECIFIED.,.F.,.F.,.F.)
B_SPLINE_SURFACE_WITH_KNOTS((4,4),(3,2,2,2,3),(0.,1.),(0.,0.25,0.5,0.75,
1.),.UNSPECIFIED.)
GEOMETRIC_REPRESENTATION_ITEM()
RATIONAL_B_SPLINE_SURFACE(((1.,0.974927912181824,1.,0.974927912181824,1.,
0.974927912181824,1.,0.974927912181824,1.),(0.833333333333333,0.812439926818186,
0.833333333333333,0.812439926818186,0.833333333333333,0.812439926818186,
0.833333333333333,0.812439926818186,0.833333333333333),(0.833333333333333,
0.812439926818186,0.833333333333333,0.812439926818186,0.833333333333333,
0.812439926818186,0.833333333333333,0.812439926818186,0.833333333333333),
(1.,0.974927912181824,1.,0.974927912181824,1.,0.974927912181824,1.,0.974927912181824,
1.)))
REPRESENTATION_ITEM('')
SURFACE()
);
#340=(
BOUNDED_SURFACE()
B_SPLINE_SURFACE(3,2,((#23530,#23531,#23532,#23533,#23534,#23535,#23536,
#23537,#23538),(#23539,#23540,#23541,#23542,#23543,#23544,#23545,#23546,
#23547),(#23548,#23549,#23550,#23551,#23552,#23553,#23554,#23555,#23556),
(#23557,#23558,#23559,#23560,#23561,#23562,#23563,#23564,#23565)),
 .UNSPECIFIED.,.F.,.F.,.F.)
B_SPLINE_SURFACE_WITH_KNOTS((4,4),(3,2,2,2,3),(0.,1.),(0.,0.25,0.5,0.75,
1.),.UNSPECIFIED.)
GEOMETRIC_REPRESENTATION_ITEM()
RATIONAL_B_SPLINE_SURFACE(((1.,0.974927912181824,1.,0.974927912181824,1.,
0.974927912181824,1.,0.974927912181824,1.),(0.987189825241073,0.962438915249418,
0.987189825241073,0.962438915249418,0.987189825241073,0.962438915249418,
0.987189825241073,0.962438915249418,0.987189825241073),(0.987189825241073,
0.962438915249418,0.987189825241073,0.962438915249418,0.987189825241073,
0.962438915249418,0.987189825241073,0.962438915249418,0.987189825241073),
(1.,0.974927912181824,1.,0.974927912181824,1.,0.974927912181824,1.,0.974927912181824,
1.)))
REPRESENTATION_ITEM('')
SURFACE()
);
#341=(
BOUNDED_SURFACE()
B_SPLINE_SURFACE(3,2,((#23573,#23574,#23575,#23576,#23577,#23578,#23579,
#23580,#23581),(#23582,#23583,#23584,#23585,#23586,#23587,#23588,#23589,
#23590),(#23591,#23592,#23593,#23594,#23595,#23596,#23597,#23598,#23599),
(#23600,#23601,#23602,#23603,#23604,#23605,#23606,#23607,#23608)),
 .UNSPECIFIED.,.F.,.F.,.F.)
B_SPLINE_SURFACE_WITH_KNOTS((4,4),(3,2,2,2,3),(0.,1.),(0.,0.25,0.5,0.75,
1.),.UNSPECIFIED.)
GEOMETRIC_REPRESENTATION_ITEM()
RATIONAL_B_SPLINE_SURFACE(((1.,0.974927912181824,1.,0.974927912181824,1.,
0.974927912181824,1.,0.974927912181824,1.),(0.987189825241073,0.962438915249418,
0.987189825241073,0.962438915249418,0.987189825241073,0.962438915249418,
0.987189825241073,0.962438915249418,0.987189825241073),(0.987189825241073,
0.962438915249418,0.987189825241073,0.962438915249418,0.987189825241073,
0.962438915249418,0.987189825241073,0.962438915249418,0.987189825241073),
(1.,0.974927912181824,1.,0.974927912181824,1.,0.974927912181824,1.,0.974927912181824,
1.)))
REPRESENTATION_ITEM('')
SURFACE()
);
#342=(
BOUNDED_SURFACE()
B_SPLINE_SURFACE(3,2,((#23616,#23617,#23618,#23619,#23620,#23621,#23622,
#23623,#23624),(#23625,#23626,#23627,#23628,#23629,#23630,#23631,#23632,
#23633),(#23634,#23635,#23636,#23637,#23638,#23639,#23640,#23641,#23642),
(#23643,#23644,#23645,#23646,#23647,#23648,#23649,#23650,#23651)),
 .UNSPECIFIED.,.F.,.F.,.F.)
B_SPLINE_SURFACE_WITH_KNOTS((4,4),(3,2,2,2,3),(0.,1.),(0.,0.25,0.5,0.75,
1.),.UNSPECIFIED.)
GEOMETRIC_REPRESENTATION_ITEM()
RATIONAL_B_SPLINE_SURFACE(((1.,0.974927912181824,1.,0.974927912181824,1.,
0.974927912181824,1.,0.974927912181824,1.),(0.833333333333331,0.812439926818184,
0.833333333333331,0.812439926818184,0.833333333333331,0.812439926818184,
0.833333333333331,0.812439926818184,0.833333333333331),(0.833333333333331,
0.812439926818184,0.833333333333331,0.812439926818184,0.833333333333331,
0.812439926818184,0.833333333333331,0.812439926818184,0.833333333333331),
(1.,0.974927912181824,1.,0.974927912181824,1.,0.974927912181824,1.,0.974927912181824,
1.)))
REPRESENTATION_ITEM('')
SURFACE()
);
#343=(
BOUNDED_SURFACE()
B_SPLINE_SURFACE(3,2,((#23655,#23656,#23657,#23658,#23659,#23660,#23661,
#23662,#23663),(#23664,#23665,#23666,#23667,#23668,#23669,#23670,#23671,
#23672),(#23673,#23674,#23675,#23676,#23677,#23678,#23679,#23680,#23681),
(#23682,#23683,#23684,#23685,#23686,#23687,#23688,#23689,#23690)),
 .UNSPECIFIED.,.F.,.F.,.F.)
B_SPLINE_SURFACE_WITH_KNOTS((4,4),(3,2,2,2,3),(0.,1.),(0.,0.25,0.5,0.75,
1.),.UNSPECIFIED.)
GEOMETRIC_REPRESENTATION_ITEM()
RATIONAL_B_SPLINE_SURFACE(((1.,0.974927912181824,1.,0.974927912181824,1.,
0.974927912181824,1.,0.974927912181824,1.),(0.987189825241073,0.962438915249418,
0.987189825241073,0.962438915249418,0.987189825241073,0.962438915249418,
0.987189825241073,0.962438915249418,0.987189825241073),(0.987189825241073,
0.962438915249418,0.987189825241073,0.962438915249418,0.987189825241073,
0.962438915249418,0.987189825241073,0.962438915249418,0.987189825241073),
(1.,0.974927912181824,1.,0.974927912181824,1.,0.974927912181824,1.,0.974927912181824,
1.)))
REPRESENTATION_ITEM('')
SURFACE()
);
#344=(
BOUNDED_SURFACE()
B_SPLINE_SURFACE(3,2,((#23745,#23746,#23747,#23748,#23749,#23750,#23751,
#23752,#23753),(#23754,#23755,#23756,#23757,#23758,#23759,#23760,#23761,
#23762),(#23763,#23764,#23765,#23766,#23767,#23768,#23769,#23770,#23771),
(#23772,#23773,#23774,#23775,#23776,#23777,#23778,#23779,#23780)),
 .UNSPECIFIED.,.F.,.F.,.F.)
B_SPLINE_SURFACE_WITH_KNOTS((4,4),(3,2,2,2,3),(0.,1.),(0.,0.25,0.5,0.75,
1.),.UNSPECIFIED.)
GEOMETRIC_REPRESENTATION_ITEM()
RATIONAL_B_SPLINE_SURFACE(((1.,0.974927912181824,1.,0.974927912181824,1.,
0.974927912181824,1.,0.974927912181824,1.),(0.987189825241073,0.962438915249418,
0.987189825241073,0.962438915249418,0.987189825241073,0.962438915249418,
0.987189825241073,0.962438915249418,0.987189825241073),(0.987189825241073,
0.962438915249418,0.987189825241073,0.962438915249418,0.987189825241073,
0.962438915249418,0.987189825241073,0.962438915249418,0.987189825241073),
(1.,0.974927912181824,1.,0.974927912181824,1.,0.974927912181824,1.,0.974927912181824,
1.)))
REPRESENTATION_ITEM('')
SURFACE()
);
#345=(
BOUNDED_SURFACE()
B_SPLINE_SURFACE(3,2,((#23788,#23789,#23790,#23791,#23792,#23793,#23794,
#23795,#23796),(#23797,#23798,#23799,#23800,#23801,#23802,#23803,#23804,
#23805),(#23806,#23807,#23808,#23809,#23810,#23811,#23812,#23813,#23814),
(#23815,#23816,#23817,#23818,#23819,#23820,#23821,#23822,#23823)),
 .UNSPECIFIED.,.F.,.F.,.F.)
B_SPLINE_SURFACE_WITH_KNOTS((4,4),(3,2,2,2,3),(0.,1.),(0.,0.25,0.5,0.75,
1.),.UNSPECIFIED.)
GEOMETRIC_REPRESENTATION_ITEM()
RATIONAL_B_SPLINE_SURFACE(((1.,0.974927912181824,1.,0.974927912181824,1.,
0.974927912181824,1.,0.974927912181824,1.),(0.833333333333333,0.812439926818186,
0.833333333333333,0.812439926818186,0.833333333333333,0.812439926818186,
0.833333333333333,0.812439926818186,0.833333333333333),(0.833333333333333,
0.812439926818186,0.833333333333333,0.812439926818186,0.833333333333333,
0.812439926818186,0.833333333333333,0.812439926818186,0.833333333333333),
(1.,0.974927912181824,1.,0.974927912181824,1.,0.974927912181824,1.,0.974927912181824,
1.)))
REPRESENTATION_ITEM('')
SURFACE()
);
#346=(
BOUNDED_SURFACE()
B_SPLINE_SURFACE(3,2,((#23827,#23828,#23829,#23830,#23831,#23832,#23833,
#23834,#23835),(#23836,#23837,#23838,#23839,#23840,#23841,#23842,#23843,
#23844),(#23845,#23846,#23847,#23848,#23849,#23850,#23851,#23852,#23853),
(#23854,#23855,#23856,#23857,#23858,#23859,#23860,#23861,#23862)),
 .UNSPECIFIED.,.F.,.F.,.F.)
B_SPLINE_SURFACE_WITH_KNOTS((4,4),(3,2,2,2,3),(0.,1.),(0.,0.25,0.5,0.75,
1.),.UNSPECIFIED.)
GEOMETRIC_REPRESENTATION_ITEM()
RATIONAL_B_SPLINE_SURFACE(((1.,0.974927912181824,1.,0.974927912181824,1.,
0.974927912181824,1.,0.974927912181824,1.),(0.987189825241073,0.962438915249418,
0.987189825241073,0.962438915249418,0.987189825241073,0.962438915249418,
0.987189825241073,0.962438915249418,0.987189825241073),(0.987189825241073,
0.962438915249418,0.987189825241073,0.962438915249418,0.987189825241073,
0.962438915249418,0.987189825241073,0.962438915249418,0.987189825241073),
(1.,0.974927912181824,1.,0.974927912181824,1.,0.974927912181824,1.,0.974927912181824,
1.)))
REPRESENTATION_ITEM('')
SURFACE()
);
#347=(
BOUNDED_SURFACE()
B_SPLINE_SURFACE(3,2,((#23917,#23918,#23919,#23920,#23921,#23922,#23923,
#23924,#23925),(#23926,#23927,#23928,#23929,#23930,#23931,#23932,#23933,
#23934),(#23935,#23936,#23937,#23938,#23939,#23940,#23941,#23942,#23943),
(#23944,#23945,#23946,#23947,#23948,#23949,#23950,#23951,#23952)),
 .UNSPECIFIED.,.F.,.F.,.F.)
B_SPLINE_SURFACE_WITH_KNOTS((4,4),(3,2,2,2,3),(0.,1.),(0.,0.25,0.5,0.75,
1.),.UNSPECIFIED.)
GEOMETRIC_REPRESENTATION_ITEM()
RATIONAL_B_SPLINE_SURFACE(((1.,0.974927912181824,1.,0.974927912181824,1.,
0.974927912181824,1.,0.974927912181824,1.),(0.987189825241073,0.962438915249418,
0.987189825241073,0.962438915249418,0.987189825241073,0.962438915249418,
0.987189825241073,0.962438915249418,0.987189825241073),(0.987189825241073,
0.962438915249418,0.987189825241073,0.962438915249418,0.987189825241073,
0.962438915249418,0.987189825241073,0.962438915249418,0.987189825241073),
(1.,0.974927912181824,1.,0.974927912181824,1.,0.974927912181824,1.,0.974927912181824,
1.)))
REPRESENTATION_ITEM('')
SURFACE()
);
#348=(
BOUNDED_SURFACE()
B_SPLINE_SURFACE(3,2,((#23960,#23961,#23962,#23963,#23964,#23965,#23966,
#23967,#23968),(#23969,#23970,#23971,#23972,#23973,#23974,#23975,#23976,
#23977),(#23978,#23979,#23980,#23981,#23982,#23983,#23984,#23985,#23986),
(#23987,#23988,#23989,#23990,#23991,#23992,#23993,#23994,#23995)),
 .UNSPECIFIED.,.F.,.F.,.F.)
B_SPLINE_SURFACE_WITH_KNOTS((4,4),(3,2,2,2,3),(0.,1.),(0.,0.25,0.5,0.75,
1.),.UNSPECIFIED.)
GEOMETRIC_REPRESENTATION_ITEM()
RATIONAL_B_SPLINE_SURFACE(((1.,0.974927912181824,1.,0.974927912181824,1.,
0.974927912181824,1.,0.974927912181824,1.),(0.833333333333332,0.812439926818185,
0.833333333333332,0.812439926818185,0.833333333333332,0.812439926818185,
0.833333333333332,0.812439926818185,0.833333333333332),(0.833333333333332,
0.812439926818185,0.833333333333332,0.812439926818185,0.833333333333332,
0.812439926818185,0.833333333333332,0.812439926818185,0.833333333333332),
(1.,0.974927912181824,1.,0.974927912181824,1.,0.974927912181824,1.,0.974927912181824,
1.)))
REPRESENTATION_ITEM('')
SURFACE()
);
#349=(
BOUNDED_SURFACE()
B_SPLINE_SURFACE(3,2,((#23999,#24000,#24001,#24002,#24003,#24004,#24005,
#24006,#24007),(#24008,#24009,#24010,#24011,#24012,#24013,#24014,#24015,
#24016),(#24017,#24018,#24019,#24020,#24021,#24022,#24023,#24024,#24025),
(#24026,#24027,#24028,#24029,#24030,#24031,#24032,#24033,#24034)),
 .UNSPECIFIED.,.F.,.F.,.F.)
B_SPLINE_SURFACE_WITH_KNOTS((4,4),(3,2,2,2,3),(0.,1.),(0.,0.25,0.5,0.75,
1.),.UNSPECIFIED.)
GEOMETRIC_REPRESENTATION_ITEM()
RATIONAL_B_SPLINE_SURFACE(((1.,0.974927912181824,1.,0.974927912181824,1.,
0.974927912181824,1.,0.974927912181824,1.),(0.987189825241073,0.962438915249418,
0.987189825241073,0.962438915249418,0.987189825241073,0.962438915249418,
0.987189825241073,0.962438915249418,0.987189825241073),(0.987189825241073,
0.962438915249418,0.987189825241073,0.962438915249418,0.987189825241073,
0.962438915249418,0.987189825241073,0.962438915249418,0.987189825241073),
(1.,0.974927912181824,1.,0.974927912181824,1.,0.974927912181824,1.,0.974927912181824,
1.)))
REPRESENTATION_ITEM('')
SURFACE()
);
#350=(
BOUNDED_SURFACE()
B_SPLINE_SURFACE(3,2,((#24089,#24090,#24091,#24092,#24093,#24094,#24095,
#24096,#24097),(#24098,#24099,#24100,#24101,#24102,#24103,#24104,#24105,
#24106),(#24107,#24108,#24109,#24110,#24111,#24112,#24113,#24114,#24115),
(#24116,#24117,#24118,#24119,#24120,#24121,#24122,#24123,#24124)),
 .UNSPECIFIED.,.F.,.F.,.F.)
B_SPLINE_SURFACE_WITH_KNOTS((4,4),(3,2,2,2,3),(0.,1.),(0.,0.25,0.5,0.75,
1.),.UNSPECIFIED.)
GEOMETRIC_REPRESENTATION_ITEM()
RATIONAL_B_SPLINE_SURFACE(((1.,0.974927912181824,1.,0.974927912181824,1.,
0.974927912181824,1.,0.974927912181824,1.),(0.987189825241073,0.962438915249418,
0.987189825241073,0.962438915249418,0.987189825241073,0.962438915249418,
0.987189825241073,0.962438915249418,0.987189825241073),(0.987189825241073,
0.962438915249418,0.987189825241073,0.962438915249418,0.987189825241073,
0.962438915249418,0.987189825241073,0.962438915249418,0.987189825241073),
(1.,0.974927912181824,1.,0.974927912181824,1.,0.974927912181824,1.,0.974927912181824,
1.)))
REPRESENTATION_ITEM('')
SURFACE()
);
#351=(
BOUNDED_SURFACE()
B_SPLINE_SURFACE(3,2,((#24132,#24133,#24134,#24135,#24136,#24137,#24138,
#24139,#24140),(#24141,#24142,#24143,#24144,#24145,#24146,#24147,#24148,
#24149),(#24150,#24151,#24152,#24153,#24154,#24155,#24156,#24157,#24158),
(#24159,#24160,#24161,#24162,#24163,#24164,#24165,#24166,#24167)),
 .UNSPECIFIED.,.F.,.F.,.F.)
B_SPLINE_SURFACE_WITH_KNOTS((4,4),(3,2,2,2,3),(0.,1.),(0.,0.25,0.5,0.75,
1.),.UNSPECIFIED.)
GEOMETRIC_REPRESENTATION_ITEM()
RATIONAL_B_SPLINE_SURFACE(((1.,0.974927912181824,1.,0.974927912181824,1.,
0.974927912181824,1.,0.974927912181824,1.),(0.833333333333332,0.812439926818185,
0.833333333333332,0.812439926818185,0.833333333333332,0.812439926818185,
0.833333333333332,0.812439926818185,0.833333333333332),(0.833333333333332,
0.812439926818185,0.833333333333332,0.812439926818185,0.833333333333332,
0.812439926818185,0.833333333333332,0.812439926818185,0.833333333333332),
(1.,0.974927912181824,1.,0.974927912181824,1.,0.974927912181824,1.,0.974927912181824,
1.)))
REPRESENTATION_ITEM('')
SURFACE()
);
#352=(
BOUNDED_SURFACE()
B_SPLINE_SURFACE(3,2,((#24171,#24172,#24173,#24174,#24175,#24176,#24177,
#24178,#24179),(#24180,#24181,#24182,#24183,#24184,#24185,#24186,#24187,
#24188),(#24189,#24190,#24191,#24192,#24193,#24194,#24195,#24196,#24197),
(#24198,#24199,#24200,#24201,#24202,#24203,#24204,#24205,#24206)),
 .UNSPECIFIED.,.F.,.F.,.F.)
B_SPLINE_SURFACE_WITH_KNOTS((4,4),(3,2,2,2,3),(0.,1.),(0.,0.25,0.5,0.75,
1.),.UNSPECIFIED.)
GEOMETRIC_REPRESENTATION_ITEM()
RATIONAL_B_SPLINE_SURFACE(((1.,0.974927912181824,1.,0.974927912181824,1.,
0.974927912181824,1.,0.974927912181824,1.),(0.987189825241073,0.962438915249418,
0.987189825241073,0.962438915249418,0.987189825241073,0.962438915249418,
0.987189825241073,0.962438915249418,0.987189825241073),(0.987189825241073,
0.962438915249418,0.987189825241073,0.962438915249418,0.987189825241073,
0.962438915249418,0.987189825241073,0.962438915249418,0.987189825241073),
(1.,0.974927912181824,1.,0.974927912181824,1.,0.974927912181824,1.,0.974927912181824,
1.)))
REPRESENTATION_ITEM('')
SURFACE()
);
#353=(
BOUNDED_SURFACE()
B_SPLINE_SURFACE(3,2,((#24261,#24262,#24263,#24264,#24265,#24266,#24267,
#24268,#24269),(#24270,#24271,#24272,#24273,#24274,#24275,#24276,#24277,
#24278),(#24279,#24280,#24281,#24282,#24283,#24284,#24285,#24286,#24287),
(#24288,#24289,#24290,#24291,#24292,#24293,#24294,#24295,#24296)),
 .UNSPECIFIED.,.F.,.F.,.F.)
B_SPLINE_SURFACE_WITH_KNOTS((4,4),(3,2,2,2,3),(0.,1.),(0.,0.25,0.5,0.75,
1.),.UNSPECIFIED.)
GEOMETRIC_REPRESENTATION_ITEM()
RATIONAL_B_SPLINE_SURFACE(((1.,0.974927912181824,1.,0.974927912181824,1.,
0.974927912181824,1.,0.974927912181824,1.),(0.987189825241073,0.962438915249418,
0.987189825241073,0.962438915249418,0.987189825241073,0.962438915249418,
0.987189825241073,0.962438915249418,0.987189825241073),(0.987189825241073,
0.962438915249418,0.987189825241073,0.962438915249418,0.987189825241073,
0.962438915249418,0.987189825241073,0.962438915249418,0.987189825241073),
(1.,0.974927912181824,1.,0.974927912181824,1.,0.974927912181824,1.,0.974927912181824,
1.)))
REPRESENTATION_ITEM('')
SURFACE()
);
#354=(
BOUNDED_SURFACE()
B_SPLINE_SURFACE(3,2,((#24304,#24305,#24306,#24307,#24308,#24309,#24310,
#24311,#24312),(#24313,#24314,#24315,#24316,#24317,#24318,#24319,#24320,
#24321),(#24322,#24323,#24324,#24325,#24326,#24327,#24328,#24329,#24330),
(#24331,#24332,#24333,#24334,#24335,#24336,#24337,#24338,#24339)),
 .UNSPECIFIED.,.F.,.F.,.F.)
B_SPLINE_SURFACE_WITH_KNOTS((4,4),(3,2,2,2,3),(0.,1.),(0.,0.25,0.5,0.75,
1.),.UNSPECIFIED.)
GEOMETRIC_REPRESENTATION_ITEM()
RATIONAL_B_SPLINE_SURFACE(((1.,0.974927912181824,1.,0.974927912181824,1.,
0.974927912181824,1.,0.974927912181824,1.),(0.833333333333333,0.812439926818186,
0.833333333333333,0.812439926818186,0.833333333333333,0.812439926818186,
0.833333333333333,0.812439926818186,0.833333333333333),(0.833333333333333,
0.812439926818186,0.833333333333333,0.812439926818186,0.833333333333333,
0.812439926818186,0.833333333333333,0.812439926818186,0.833333333333333),
(1.,0.974927912181824,1.,0.974927912181824,1.,0.974927912181824,1.,0.974927912181824,
1.)))
REPRESENTATION_ITEM('')
SURFACE()
);
#355=(
BOUNDED_SURFACE()
B_SPLINE_SURFACE(3,2,((#24343,#24344,#24345,#24346,#24347,#24348,#24349,
#24350,#24351),(#24352,#24353,#24354,#24355,#24356,#24357,#24358,#24359,
#24360),(#24361,#24362,#24363,#24364,#24365,#24366,#24367,#24368,#24369),
(#24370,#24371,#24372,#24373,#24374,#24375,#24376,#24377,#24378)),
 .UNSPECIFIED.,.F.,.F.,.F.)
B_SPLINE_SURFACE_WITH_KNOTS((4,4),(3,2,2,2,3),(0.,1.),(0.,0.25,0.5,0.75,
1.),.UNSPECIFIED.)
GEOMETRIC_REPRESENTATION_ITEM()
RATIONAL_B_SPLINE_SURFACE(((1.,0.974927912181824,1.,0.974927912181824,1.,
0.974927912181824,1.,0.974927912181824,1.),(0.987189825241073,0.962438915249418,
0.987189825241073,0.962438915249418,0.987189825241073,0.962438915249418,
0.987189825241073,0.962438915249418,0.987189825241073),(0.987189825241073,
0.962438915249418,0.987189825241073,0.962438915249418,0.987189825241073,
0.962438915249418,0.987189825241073,0.962438915249418,0.987189825241073),
(1.,0.974927912181824,1.,0.974927912181824,1.,0.974927912181824,1.,0.974927912181824,
1.)))
REPRESENTATION_ITEM('')
SURFACE()
);
#356=(
BOUNDED_SURFACE()
B_SPLINE_SURFACE(3,2,((#24433,#24434,#24435,#24436,#24437,#24438,#24439,
#24440,#24441),(#24442,#24443,#24444,#24445,#24446,#24447,#24448,#24449,
#24450),(#24451,#24452,#24453,#24454,#24455,#24456,#24457,#24458,#24459),
(#24460,#24461,#24462,#24463,#24464,#24465,#24466,#24467,#24468)),
 .UNSPECIFIED.,.F.,.F.,.F.)
B_SPLINE_SURFACE_WITH_KNOTS((4,4),(3,2,2,2,3),(0.,1.),(0.,0.25,0.5,0.75,
1.),.UNSPECIFIED.)
GEOMETRIC_REPRESENTATION_ITEM()
RATIONAL_B_SPLINE_SURFACE(((1.,0.974927912181824,1.,0.974927912181824,1.,
0.974927912181824,1.,0.974927912181824,1.),(0.987189825241073,0.962438915249418,
0.987189825241073,0.962438915249418,0.987189825241073,0.962438915249418,
0.987189825241073,0.962438915249418,0.987189825241073),(0.987189825241073,
0.962438915249418,0.987189825241073,0.962438915249418,0.987189825241073,
0.962438915249418,0.987189825241073,0.962438915249418,0.987189825241073),
(1.,0.974927912181824,1.,0.974927912181824,1.,0.974927912181824,1.,0.974927912181824,
1.)))
REPRESENTATION_ITEM('')
SURFACE()
);
#357=(
BOUNDED_SURFACE()
B_SPLINE_SURFACE(3,2,((#24476,#24477,#24478,#24479,#24480,#24481,#24482,
#24483,#24484),(#24485,#24486,#24487,#24488,#24489,#24490,#24491,#24492,
#24493),(#24494,#24495,#24496,#24497,#24498,#24499,#24500,#24501,#24502),
(#24503,#24504,#24505,#24506,#24507,#24508,#24509,#24510,#24511)),
 .UNSPECIFIED.,.F.,.F.,.F.)
B_SPLINE_SURFACE_WITH_KNOTS((4,4),(3,2,2,2,3),(0.,1.),(0.,0.25,0.5,0.75,
1.),.UNSPECIFIED.)
GEOMETRIC_REPRESENTATION_ITEM()
RATIONAL_B_SPLINE_SURFACE(((1.,0.974927912181824,1.,0.974927912181824,1.,
0.974927912181824,1.,0.974927912181824,1.),(0.833333333333331,0.812439926818184,
0.833333333333331,0.812439926818184,0.833333333333331,0.812439926818184,
0.833333333333331,0.812439926818184,0.833333333333331),(0.833333333333331,
0.812439926818184,0.833333333333331,0.812439926818184,0.833333333333331,
0.812439926818184,0.833333333333331,0.812439926818184,0.833333333333331),
(1.,0.974927912181824,1.,0.974927912181824,1.,0.974927912181824,1.,0.974927912181824,
1.)))
REPRESENTATION_ITEM('')
SURFACE()
);
#358=(
BOUNDED_SURFACE()
B_SPLINE_SURFACE(3,2,((#24515,#24516,#24517,#24518,#24519,#24520,#24521,
#24522,#24523),(#24524,#24525,#24526,#24527,#24528,#24529,#24530,#24531,
#24532),(#24533,#24534,#24535,#24536,#24537,#24538,#24539,#24540,#24541),
(#24542,#24543,#24544,#24545,#24546,#24547,#24548,#24549,#24550)),
 .UNSPECIFIED.,.F.,.F.,.F.)
B_SPLINE_SURFACE_WITH_KNOTS((4,4),(3,2,2,2,3),(0.,1.),(0.,0.25,0.5,0.75,
1.),.UNSPECIFIED.)
GEOMETRIC_REPRESENTATION_ITEM()
RATIONAL_B_SPLINE_SURFACE(((1.,0.974927912181824,1.,0.974927912181824,1.,
0.974927912181824,1.,0.974927912181824,1.),(0.987189825241073,0.962438915249418,
0.987189825241073,0.962438915249418,0.987189825241073,0.962438915249418,
0.987189825241073,0.962438915249418,0.987189825241073),(0.987189825241073,
0.962438915249418,0.987189825241073,0.962438915249418,0.987189825241073,
0.962438915249418,0.987189825241073,0.962438915249418,0.987189825241073),
(1.,0.974927912181824,1.,0.974927912181824,1.,0.974927912181824,1.,0.974927912181824,
1.)))
REPRESENTATION_ITEM('')
SURFACE()
);
#359=(
BOUNDED_SURFACE()
B_SPLINE_SURFACE(3,2,((#24605,#24606,#24607,#24608,#24609,#24610,#24611,
#24612,#24613),(#24614,#24615,#24616,#24617,#24618,#24619,#24620,#24621,
#24622),(#24623,#24624,#24625,#24626,#24627,#24628,#24629,#24630,#24631),
(#24632,#24633,#24634,#24635,#24636,#24637,#24638,#24639,#24640)),
 .UNSPECIFIED.,.F.,.F.,.F.)
B_SPLINE_SURFACE_WITH_KNOTS((4,4),(3,2,2,2,3),(0.,1.),(0.,0.25,0.5,0.75,
1.),.UNSPECIFIED.)
GEOMETRIC_REPRESENTATION_ITEM()
RATIONAL_B_SPLINE_SURFACE(((1.,0.974927912181824,1.,0.974927912181824,1.,
0.974927912181824,1.,0.974927912181824,1.),(0.987189825241073,0.962438915249418,
0.987189825241073,0.962438915249418,0.987189825241073,0.962438915249418,
0.987189825241073,0.962438915249418,0.987189825241073),(0.987189825241073,
0.962438915249418,0.987189825241073,0.962438915249418,0.987189825241073,
0.962438915249418,0.987189825241073,0.962438915249418,0.987189825241073),
(1.,0.974927912181824,1.,0.974927912181824,1.,0.974927912181824,1.,0.974927912181824,
1.)))
REPRESENTATION_ITEM('')
SURFACE()
);
#360=(
BOUNDED_SURFACE()
B_SPLINE_SURFACE(3,2,((#24648,#24649,#24650,#24651,#24652,#24653,#24654,
#24655,#24656),(#24657,#24658,#24659,#24660,#24661,#24662,#24663,#24664,
#24665),(#24666,#24667,#24668,#24669,#24670,#24671,#24672,#24673,#24674),
(#24675,#24676,#24677,#24678,#24679,#24680,#24681,#24682,#24683)),
 .UNSPECIFIED.,.F.,.F.,.F.)
B_SPLINE_SURFACE_WITH_KNOTS((4,4),(3,2,2,2,3),(0.,1.),(0.,0.25,0.5,0.75,
1.),.UNSPECIFIED.)
GEOMETRIC_REPRESENTATION_ITEM()
RATIONAL_B_SPLINE_SURFACE(((1.,0.974927912181824,1.,0.974927912181824,1.,
0.974927912181824,1.,0.974927912181824,1.),(0.833333333333332,0.812439926818185,
0.833333333333332,0.812439926818185,0.833333333333332,0.812439926818185,
0.833333333333332,0.812439926818185,0.833333333333332),(0.833333333333332,
0.812439926818185,0.833333333333332,0.812439926818185,0.833333333333332,
0.812439926818185,0.833333333333332,0.812439926818185,0.833333333333332),
(1.,0.974927912181824,1.,0.974927912181824,1.,0.974927912181824,1.,0.974927912181824,
1.)))
REPRESENTATION_ITEM('')
SURFACE()
);
#361=(
BOUNDED_SURFACE()
B_SPLINE_SURFACE(3,2,((#24687,#24688,#24689,#24690,#24691,#24692,#24693,
#24694,#24695),(#24696,#24697,#24698,#24699,#24700,#24701,#24702,#24703,
#24704),(#24705,#24706,#24707,#24708,#24709,#24710,#24711,#24712,#24713),
(#24714,#24715,#24716,#24717,#24718,#24719,#24720,#24721,#24722)),
 .UNSPECIFIED.,.F.,.F.,.F.)
B_SPLINE_SURFACE_WITH_KNOTS((4,4),(3,2,2,2,3),(0.,1.),(0.,0.25,0.5,0.75,
1.),.UNSPECIFIED.)
GEOMETRIC_REPRESENTATION_ITEM()
RATIONAL_B_SPLINE_SURFACE(((1.,0.974927912181824,1.,0.974927912181824,1.,
0.974927912181824,1.,0.974927912181824,1.),(0.987189825241073,0.962438915249418,
0.987189825241073,0.962438915249418,0.987189825241073,0.962438915249418,
0.987189825241073,0.962438915249418,0.987189825241073),(0.987189825241073,
0.962438915249418,0.987189825241073,0.962438915249418,0.987189825241073,
0.962438915249418,0.987189825241073,0.962438915249418,0.987189825241073),
(1.,0.974927912181824,1.,0.974927912181824,1.,0.974927912181824,1.,0.974927912181824,
1.)))
REPRESENTATION_ITEM('')
SURFACE()
);
#362=(
BOUNDED_SURFACE()
B_SPLINE_SURFACE(3,2,((#24777,#24778,#24779,#24780,#24781,#24782,#24783,
#24784,#24785),(#24786,#24787,#24788,#24789,#24790,#24791,#24792,#24793,
#24794),(#24795,#24796,#24797,#24798,#24799,#24800,#24801,#24802,#24803),
(#24804,#24805,#24806,#24807,#24808,#24809,#24810,#24811,#24812)),
 .UNSPECIFIED.,.F.,.F.,.F.)
B_SPLINE_SURFACE_WITH_KNOTS((4,4),(3,2,2,2,3),(0.,1.),(0.,0.25,0.5,0.75,
1.),.UNSPECIFIED.)
GEOMETRIC_REPRESENTATION_ITEM()
RATIONAL_B_SPLINE_SURFACE(((1.,0.974927912181824,1.,0.974927912181824,1.,
0.974927912181824,1.,0.974927912181824,1.),(0.987189825241073,0.962438915249418,
0.987189825241073,0.962438915249418,0.987189825241073,0.962438915249418,
0.987189825241073,0.962438915249418,0.987189825241073),(0.987189825241073,
0.962438915249418,0.987189825241073,0.962438915249418,0.987189825241073,
0.962438915249418,0.987189825241073,0.962438915249418,0.987189825241073),
(1.,0.974927912181824,1.,0.974927912181824,1.,0.974927912181824,1.,0.974927912181824,
1.)))
REPRESENTATION_ITEM('')
SURFACE()
);
#363=(
BOUNDED_SURFACE()
B_SPLINE_SURFACE(3,2,((#24820,#24821,#24822,#24823,#24824,#24825,#24826,
#24827,#24828),(#24829,#24830,#24831,#24832,#24833,#24834,#24835,#24836,
#24837),(#24838,#24839,#24840,#24841,#24842,#24843,#24844,#24845,#24846),
(#24847,#24848,#24849,#24850,#24851,#24852,#24853,#24854,#24855)),
 .UNSPECIFIED.,.F.,.F.,.F.)
B_SPLINE_SURFACE_WITH_KNOTS((4,4),(3,2,2,2,3),(0.,1.),(0.,0.25,0.5,0.75,
1.),.UNSPECIFIED.)
GEOMETRIC_REPRESENTATION_ITEM()
RATIONAL_B_SPLINE_SURFACE(((1.,0.974927912181824,1.,0.974927912181824,1.,
0.974927912181824,1.,0.974927912181824,1.),(0.833333333333332,0.812439926818185,
0.833333333333332,0.812439926818185,0.833333333333332,0.812439926818185,
0.833333333333332,0.812439926818185,0.833333333333332),(0.833333333333332,
0.812439926818185,0.833333333333332,0.812439926818185,0.833333333333332,
0.812439926818185,0.833333333333332,0.812439926818185,0.833333333333332),
(1.,0.974927912181824,1.,0.974927912181824,1.,0.974927912181824,1.,0.974927912181824,
1.)))
REPRESENTATION_ITEM('')
SURFACE()
);
#364=(
BOUNDED_SURFACE()
B_SPLINE_SURFACE(3,2,((#24859,#24860,#24861,#24862,#24863,#24864,#24865,
#24866,#24867),(#24868,#24869,#24870,#24871,#24872,#24873,#24874,#24875,
#24876),(#24877,#24878,#24879,#24880,#24881,#24882,#24883,#24884,#24885),
(#24886,#24887,#24888,#24889,#24890,#24891,#24892,#24893,#24894)),
 .UNSPECIFIED.,.F.,.F.,.F.)
B_SPLINE_SURFACE_WITH_KNOTS((4,4),(3,2,2,2,3),(0.,1.),(0.,0.25,0.5,0.75,
1.),.UNSPECIFIED.)
GEOMETRIC_REPRESENTATION_ITEM()
RATIONAL_B_SPLINE_SURFACE(((1.,0.974927912181824,1.,0.974927912181824,1.,
0.974927912181824,1.,0.974927912181824,1.),(0.987189825241073,0.962438915249418,
0.987189825241073,0.962438915249418,0.987189825241073,0.962438915249418,
0.987189825241073,0.962438915249418,0.987189825241073),(0.987189825241073,
0.962438915249418,0.987189825241073,0.962438915249418,0.987189825241073,
0.962438915249418,0.987189825241073,0.962438915249418,0.987189825241073),
(1.,0.974927912181824,1.,0.974927912181824,1.,0.974927912181824,1.,0.974927912181824,
1.)))
REPRESENTATION_ITEM('')
SURFACE()
);
#365=(
BOUNDED_SURFACE()
B_SPLINE_SURFACE(3,2,((#24949,#24950,#24951,#24952,#24953,#24954,#24955,
#24956,#24957),(#24958,#24959,#24960,#24961,#24962,#24963,#24964,#24965,
#24966),(#24967,#24968,#24969,#24970,#24971,#24972,#24973,#24974,#24975),
(#24976,#24977,#24978,#24979,#24980,#24981,#24982,#24983,#24984)),
 .UNSPECIFIED.,.F.,.F.,.F.)
B_SPLINE_SURFACE_WITH_KNOTS((4,4),(3,2,2,2,3),(0.,1.),(0.,0.25,0.5,0.75,
1.),.UNSPECIFIED.)
GEOMETRIC_REPRESENTATION_ITEM()
RATIONAL_B_SPLINE_SURFACE(((1.,0.974927912181824,1.,0.974927912181824,1.,
0.974927912181824,1.,0.974927912181824,1.),(0.987189825241073,0.962438915249418,
0.987189825241073,0.962438915249418,0.987189825241073,0.962438915249418,
0.987189825241073,0.962438915249418,0.987189825241073),(0.987189825241073,
0.962438915249418,0.987189825241073,0.962438915249418,0.987189825241073,
0.962438915249418,0.987189825241073,0.962438915249418,0.987189825241073),
(1.,0.974927912181824,1.,0.974927912181824,1.,0.974927912181824,1.,0.974927912181824,
1.)))
REPRESENTATION_ITEM('')
SURFACE()
);
#366=(
BOUNDED_SURFACE()
B_SPLINE_SURFACE(3,2,((#24992,#24993,#24994,#24995,#24996,#24997,#24998,
#24999,#25000),(#25001,#25002,#25003,#25004,#25005,#25006,#25007,#25008,
#25009),(#25010,#25011,#25012,#25013,#25014,#25015,#25016,#25017,#25018),
(#25019,#25020,#25021,#25022,#25023,#25024,#25025,#25026,#25027)),
 .UNSPECIFIED.,.F.,.F.,.F.)
B_SPLINE_SURFACE_WITH_KNOTS((4,4),(3,2,2,2,3),(0.,1.),(0.,0.25,0.5,0.75,
1.),.UNSPECIFIED.)
GEOMETRIC_REPRESENTATION_ITEM()
RATIONAL_B_SPLINE_SURFACE(((1.,0.974927912181824,1.,0.974927912181824,1.,
0.974927912181824,1.,0.974927912181824,1.),(0.833333333333332,0.812439926818185,
0.833333333333332,0.812439926818185,0.833333333333332,0.812439926818185,
0.833333333333332,0.812439926818185,0.833333333333332),(0.833333333333332,
0.812439926818185,0.833333333333332,0.812439926818185,0.833333333333332,
0.812439926818185,0.833333333333332,0.812439926818185,0.833333333333332),
(1.,0.974927912181824,1.,0.974927912181824,1.,0.974927912181824,1.,0.974927912181824,
1.)))
REPRESENTATION_ITEM('')
SURFACE()
);
#367=(
BOUNDED_SURFACE()
B_SPLINE_SURFACE(3,2,((#25031,#25032,#25033,#25034,#25035,#25036,#25037,
#25038,#25039),(#25040,#25041,#25042,#25043,#25044,#25045,#25046,#25047,
#25048),(#25049,#25050,#25051,#25052,#25053,#25054,#25055,#25056,#25057),
(#25058,#25059,#25060,#25061,#25062,#25063,#25064,#25065,#25066)),
 .UNSPECIFIED.,.F.,.F.,.F.)
B_SPLINE_SURFACE_WITH_KNOTS((4,4),(3,2,2,2,3),(0.,1.),(0.,0.25,0.5,0.75,
1.),.UNSPECIFIED.)
GEOMETRIC_REPRESENTATION_ITEM()
RATIONAL_B_SPLINE_SURFACE(((1.,0.974927912181824,1.,0.974927912181824,1.,
0.974927912181824,1.,0.974927912181824,1.),(0.987189825241073,0.962438915249418,
0.987189825241073,0.962438915249418,0.987189825241073,0.962438915249418,
0.987189825241073,0.962438915249418,0.987189825241073),(0.987189825241073,
0.962438915249418,0.987189825241073,0.962438915249418,0.987189825241073,
0.962438915249418,0.987189825241073,0.962438915249418,0.987189825241073),
(1.,0.974927912181824,1.,0.974927912181824,1.,0.974927912181824,1.,0.974927912181824,
1.)))
REPRESENTATION_ITEM('')
SURFACE()
);
#368=(
BOUNDED_SURFACE()
B_SPLINE_SURFACE(3,2,((#25074,#25075,#25076,#25077,#25078,#25079,#25080,
#25081,#25082),(#25083,#25084,#25085,#25086,#25087,#25088,#25089,#25090,
#25091),(#25092,#25093,#25094,#25095,#25096,#25097,#25098,#25099,#25100),
(#25101,#25102,#25103,#25104,#25105,#25106,#25107,#25108,#25109)),
 .UNSPECIFIED.,.F.,.F.,.F.)
B_SPLINE_SURFACE_WITH_KNOTS((4,4),(3,2,2,2,3),(0.,1.),(0.,0.25,0.5,0.75,
1.),.UNSPECIFIED.)
GEOMETRIC_REPRESENTATION_ITEM()
RATIONAL_B_SPLINE_SURFACE(((1.,0.974927912181824,1.,0.974927912181824,1.,
0.974927912181824,1.,0.974927912181824,1.),(0.987189825241073,0.962438915249418,
0.987189825241073,0.962438915249418,0.987189825241073,0.962438915249418,
0.987189825241073,0.962438915249418,0.987189825241073),(0.987189825241073,
0.962438915249418,0.987189825241073,0.962438915249418,0.987189825241073,
0.962438915249418,0.987189825241073,0.962438915249418,0.987189825241073),
(1.,0.974927912181824,1.,0.974927912181824,1.,0.974927912181824,1.,0.974927912181824,
1.)))
REPRESENTATION_ITEM('')
SURFACE()
);
#369=(
BOUNDED_SURFACE()
B_SPLINE_SURFACE(3,2,((#25117,#25118,#25119,#25120,#25121,#25122,#25123,
#25124,#25125),(#25126,#25127,#25128,#25129,#25130,#25131,#25132,#25133,
#25134),(#25135,#25136,#25137,#25138,#25139,#25140,#25141,#25142,#25143),
(#25144,#25145,#25146,#25147,#25148,#25149,#25150,#25151,#25152)),
 .UNSPECIFIED.,.F.,.F.,.F.)
B_SPLINE_SURFACE_WITH_KNOTS((4,4),(3,2,2,2,3),(0.,1.),(0.,0.25,0.5,0.75,
1.),.UNSPECIFIED.)
GEOMETRIC_REPRESENTATION_ITEM()
RATIONAL_B_SPLINE_SURFACE(((1.,0.974927912181824,1.,0.974927912181824,1.,
0.974927912181824,1.,0.974927912181824,1.),(0.833333333333332,0.812439926818185,
0.833333333333332,0.812439926818185,0.833333333333332,0.812439926818185,
0.833333333333332,0.812439926818185,0.833333333333332),(0.833333333333332,
0.812439926818185,0.833333333333332,0.812439926818185,0.833333333333332,
0.812439926818185,0.833333333333332,0.812439926818185,0.833333333333332),
(1.,0.974927912181824,1.,0.974927912181824,1.,0.974927912181824,1.,0.974927912181824,
1.)))
REPRESENTATION_ITEM('')
SURFACE()
);
#370=(
BOUNDED_SURFACE()
B_SPLINE_SURFACE(3,2,((#25156,#25157,#25158,#25159,#25160,#25161,#25162,
#25163,#25164),(#25165,#25166,#25167,#25168,#25169,#25170,#25171,#25172,
#25173),(#25174,#25175,#25176,#25177,#25178,#25179,#25180,#25181,#25182),
(#25183,#25184,#25185,#25186,#25187,#25188,#25189,#25190,#25191)),
 .UNSPECIFIED.,.F.,.F.,.F.)
B_SPLINE_SURFACE_WITH_KNOTS((4,4),(3,2,2,2,3),(0.,1.),(0.,0.25,0.5,0.75,
1.),.UNSPECIFIED.)
GEOMETRIC_REPRESENTATION_ITEM()
RATIONAL_B_SPLINE_SURFACE(((1.,0.974927912181824,1.,0.974927912181824,1.,
0.974927912181824,1.,0.974927912181824,1.),(0.987189825241073,0.962438915249418,
0.987189825241073,0.962438915249418,0.987189825241073,0.962438915249418,
0.987189825241073,0.962438915249418,0.987189825241073),(0.987189825241073,
0.962438915249418,0.987189825241073,0.962438915249418,0.987189825241073,
0.962438915249418,0.987189825241073,0.962438915249418,0.987189825241073),
(1.,0.974927912181824,1.,0.974927912181824,1.,0.974927912181824,1.,0.974927912181824,
1.)))
REPRESENTATION_ITEM('')
SURFACE()
);
#371=(
BOUNDED_SURFACE()
B_SPLINE_SURFACE(3,2,((#25246,#25247,#25248,#25249,#25250,#25251,#25252,
#25253,#25254),(#25255,#25256,#25257,#25258,#25259,#25260,#25261,#25262,
#25263),(#25264,#25265,#25266,#25267,#25268,#25269,#25270,#25271,#25272),
(#25273,#25274,#25275,#25276,#25277,#25278,#25279,#25280,#25281)),
 .UNSPECIFIED.,.F.,.F.,.F.)
B_SPLINE_SURFACE_WITH_KNOTS((4,4),(3,2,2,2,3),(0.,1.),(0.,0.25,0.5,0.75,
1.),.UNSPECIFIED.)
GEOMETRIC_REPRESENTATION_ITEM()
RATIONAL_B_SPLINE_SURFACE(((1.,0.974927912181824,1.,0.974927912181824,1.,
0.974927912181824,1.,0.974927912181824,1.),(0.987189825241073,0.962438915249418,
0.987189825241073,0.962438915249418,0.987189825241073,0.962438915249418,
0.987189825241073,0.962438915249418,0.987189825241073),(0.987189825241073,
0.962438915249418,0.987189825241073,0.962438915249418,0.987189825241073,
0.962438915249418,0.987189825241073,0.962438915249418,0.987189825241073),
(1.,0.974927912181824,1.,0.974927912181824,1.,0.974927912181824,1.,0.974927912181824,
1.)))
REPRESENTATION_ITEM('')
SURFACE()
);
#372=(
BOUNDED_SURFACE()
B_SPLINE_SURFACE(3,2,((#25289,#25290,#25291,#25292,#25293,#25294,#25295,
#25296,#25297),(#25298,#25299,#25300,#25301,#25302,#25303,#25304,#25305,
#25306),(#25307,#25308,#25309,#25310,#25311,#25312,#25313,#25314,#25315),
(#25316,#25317,#25318,#25319,#25320,#25321,#25322,#25323,#25324)),
 .UNSPECIFIED.,.F.,.F.,.F.)
B_SPLINE_SURFACE_WITH_KNOTS((4,4),(3,2,2,2,3),(0.,1.),(0.,0.25,0.5,0.75,
1.),.UNSPECIFIED.)
GEOMETRIC_REPRESENTATION_ITEM()
RATIONAL_B_SPLINE_SURFACE(((1.,0.974927912181824,1.,0.974927912181824,1.,
0.974927912181824,1.,0.974927912181824,1.),(0.833333333333331,0.812439926818184,
0.833333333333331,0.812439926818184,0.833333333333331,0.812439926818184,
0.833333333333331,0.812439926818184,0.833333333333331),(0.833333333333331,
0.812439926818184,0.833333333333331,0.812439926818184,0.833333333333331,
0.812439926818184,0.833333333333331,0.812439926818184,0.833333333333331),
(1.,0.974927912181824,1.,0.974927912181824,1.,0.974927912181824,1.,0.974927912181824,
1.)))
REPRESENTATION_ITEM('')
SURFACE()
);
#373=(
BOUNDED_SURFACE()
B_SPLINE_SURFACE(3,2,((#25328,#25329,#25330,#25331,#25332,#25333,#25334,
#25335,#25336),(#25337,#25338,#25339,#25340,#25341,#25342,#25343,#25344,
#25345),(#25346,#25347,#25348,#25349,#25350,#25351,#25352,#25353,#25354),
(#25355,#25356,#25357,#25358,#25359,#25360,#25361,#25362,#25363)),
 .UNSPECIFIED.,.F.,.F.,.F.)
B_SPLINE_SURFACE_WITH_KNOTS((4,4),(3,2,2,2,3),(0.,1.),(0.,0.25,0.5,0.75,
1.),.UNSPECIFIED.)
GEOMETRIC_REPRESENTATION_ITEM()
RATIONAL_B_SPLINE_SURFACE(((1.,0.974927912181824,1.,0.974927912181824,1.,
0.974927912181824,1.,0.974927912181824,1.),(0.987189825241073,0.962438915249418,
0.987189825241073,0.962438915249418,0.987189825241073,0.962438915249418,
0.987189825241073,0.962438915249418,0.987189825241073),(0.987189825241073,
0.962438915249418,0.987189825241073,0.962438915249418,0.987189825241073,
0.962438915249418,0.987189825241073,0.962438915249418,0.987189825241073),
(1.,0.974927912181824,1.,0.974927912181824,1.,0.974927912181824,1.,0.974927912181824,
1.)))
REPRESENTATION_ITEM('')
SURFACE()
);
#374=(
BOUNDED_SURFACE()
B_SPLINE_SURFACE(3,2,((#25418,#25419,#25420,#25421,#25422,#25423,#25424,
#25425,#25426),(#25427,#25428,#25429,#25430,#25431,#25432,#25433,#25434,
#25435),(#25436,#25437,#25438,#25439,#25440,#25441,#25442,#25443,#25444),
(#25445,#25446,#25447,#25448,#25449,#25450,#25451,#25452,#25453)),
 .UNSPECIFIED.,.F.,.F.,.F.)
B_SPLINE_SURFACE_WITH_KNOTS((4,4),(3,2,2,2,3),(0.,1.),(0.,0.25,0.5,0.75,
1.),.UNSPECIFIED.)
GEOMETRIC_REPRESENTATION_ITEM()
RATIONAL_B_SPLINE_SURFACE(((1.,0.974927912181824,1.,0.974927912181824,1.,
0.974927912181824,1.,0.974927912181824,1.),(0.987189825241073,0.962438915249418,
0.987189825241073,0.962438915249418,0.987189825241073,0.962438915249418,
0.987189825241073,0.962438915249418,0.987189825241073),(0.987189825241073,
0.962438915249418,0.987189825241073,0.962438915249418,0.987189825241073,
0.962438915249418,0.987189825241073,0.962438915249418,0.987189825241073),
(1.,0.974927912181824,1.,0.974927912181824,1.,0.974927912181824,1.,0.974927912181824,
1.)))
REPRESENTATION_ITEM('')
SURFACE()
);
#375=(
BOUNDED_SURFACE()
B_SPLINE_SURFACE(3,2,((#25461,#25462,#25463,#25464,#25465,#25466,#25467,
#25468,#25469),(#25470,#25471,#25472,#25473,#25474,#25475,#25476,#25477,
#25478),(#25479,#25480,#25481,#25482,#25483,#25484,#25485,#25486,#25487),
(#25488,#25489,#25490,#25491,#25492,#25493,#25494,#25495,#25496)),
 .UNSPECIFIED.,.F.,.F.,.F.)
B_SPLINE_SURFACE_WITH_KNOTS((4,4),(3,2,2,2,3),(0.,1.),(0.,0.25,0.5,0.75,
1.),.UNSPECIFIED.)
GEOMETRIC_REPRESENTATION_ITEM()
RATIONAL_B_SPLINE_SURFACE(((1.,0.974927912181824,1.,0.974927912181824,1.,
0.974927912181824,1.,0.974927912181824,1.),(0.833333333333332,0.812439926818185,
0.833333333333332,0.812439926818185,0.833333333333332,0.812439926818185,
0.833333333333332,0.812439926818185,0.833333333333332),(0.833333333333332,
0.812439926818185,0.833333333333332,0.812439926818185,0.833333333333332,
0.812439926818185,0.833333333333332,0.812439926818185,0.833333333333332),
(1.,0.974927912181824,1.,0.974927912181824,1.,0.974927912181824,1.,0.974927912181824,
1.)))
REPRESENTATION_ITEM('')
SURFACE()
);
#376=(
BOUNDED_SURFACE()
B_SPLINE_SURFACE(3,2,((#25500,#25501,#25502,#25503,#25504,#25505,#25506,
#25507,#25508),(#25509,#25510,#25511,#25512,#25513,#25514,#25515,#25516,
#25517),(#25518,#25519,#25520,#25521,#25522,#25523,#25524,#25525,#25526),
(#25527,#25528,#25529,#25530,#25531,#25532,#25533,#25534,#25535)),
 .UNSPECIFIED.,.F.,.F.,.F.)
B_SPLINE_SURFACE_WITH_KNOTS((4,4),(3,2,2,2,3),(0.,1.),(0.,0.0714285714285714,
0.142857142857143,0.214285714285714,0.25),.UNSPECIFIED.)
GEOMETRIC_REPRESENTATION_ITEM()
RATIONAL_B_SPLINE_SURFACE(((1.,0.974927912181824,1.,0.974927912181824,1.,
0.974927912181824,1.,0.987463956090912,0.987463956090912),(0.987189825241073,
0.962438915249418,0.987189825241073,0.962438915249418,0.987189825241073,
0.962438915249418,0.987189825241073,0.974814370245245,0.974814370245245),
(0.987189825241073,0.962438915249418,0.987189825241073,0.962438915249418,
0.987189825241073,0.962438915249418,0.987189825241073,0.974814370245245,
0.974814370245245),(1.,0.974927912181824,1.,0.974927912181824,1.,0.974927912181824,
1.,0.987463956090912,0.987463956090912)))
REPRESENTATION_ITEM('')
SURFACE()
);
#377=(
BOUNDED_SURFACE()
B_SPLINE_SURFACE(3,2,((#25543,#25544,#25545,#25546,#25547,#25548,#25549,
#25550,#25551),(#25552,#25553,#25554,#25555,#25556,#25557,#25558,#25559,
#25560),(#25561,#25562,#25563,#25564,#25565,#25566,#25567,#25568,#25569),
(#25570,#25571,#25572,#25573,#25574,#25575,#25576,#25577,#25578)),
 .UNSPECIFIED.,.F.,.F.,.F.)
B_SPLINE_SURFACE_WITH_KNOTS((4,4),(3,2,2,2,3),(0.,1.),(0.,0.0714285714285714,
0.142857142857143,0.214285714285714,0.25),.UNSPECIFIED.)
GEOMETRIC_REPRESENTATION_ITEM()
RATIONAL_B_SPLINE_SURFACE(((1.,0.974927912181824,1.,0.974927912181824,1.,
0.974927912181824,1.,0.987463956090912,0.987463956090912),(0.987189825241073,
0.962438915249418,0.987189825241073,0.962438915249418,0.987189825241073,
0.962438915249418,0.987189825241073,0.974814370245245,0.974814370245246),
(0.987189825241073,0.962438915249418,0.987189825241073,0.962438915249418,
0.987189825241073,0.962438915249418,0.987189825241073,0.974814370245245,
0.974814370245246),(1.,0.974927912181824,1.,0.974927912181824,1.,0.974927912181824,
1.,0.987463956090912,0.987463956090912)))
REPRESENTATION_ITEM('')
SURFACE()
);
#378=(
BOUNDED_SURFACE()
B_SPLINE_SURFACE(3,2,((#25586,#25587,#25588,#25589,#25590,#25591,#25592,
#25593,#25594),(#25595,#25596,#25597,#25598,#25599,#25600,#25601,#25602,
#25603),(#25604,#25605,#25606,#25607,#25608,#25609,#25610,#25611,#25612),
(#25613,#25614,#25615,#25616,#25617,#25618,#25619,#25620,#25621)),
 .UNSPECIFIED.,.F.,.F.,.F.)
B_SPLINE_SURFACE_WITH_KNOTS((4,4),(3,2,2,2,3),(0.,1.),(0.,0.0714285714285714,
0.142857142857143,0.214285714285714,0.25),.UNSPECIFIED.)
GEOMETRIC_REPRESENTATION_ITEM()
RATIONAL_B_SPLINE_SURFACE(((1.,0.974927912181824,1.,0.974927912181824,1.,
0.974927912181824,1.,0.987463956090912,0.987463956090912),(0.83333333333333,
0.812439926818183,0.83333333333333,0.812439926818183,0.83333333333333,0.812439926818183,
0.83333333333333,0.822886630075756,0.822886630075757),(0.83333333333333,
0.812439926818183,0.83333333333333,0.812439926818183,0.83333333333333,0.812439926818183,
0.83333333333333,0.822886630075756,0.822886630075757),(1.,0.974927912181824,
1.,0.974927912181824,1.,0.974927912181824,1.,0.987463956090912,0.987463956090912)))
REPRESENTATION_ITEM('')
SURFACE()
);
#379=(
BOUNDED_SURFACE()
B_SPLINE_SURFACE(3,2,((#25625,#25626,#25627,#25628,#25629,#25630,#25631,
#25632,#25633),(#25634,#25635,#25636,#25637,#25638,#25639,#25640,#25641,
#25642),(#25643,#25644,#25645,#25646,#25647,#25648,#25649,#25650,#25651),
(#25652,#25653,#25654,#25655,#25656,#25657,#25658,#25659,#25660)),
 .UNSPECIFIED.,.F.,.F.,.F.)
B_SPLINE_SURFACE_WITH_KNOTS((4,4),(3,2,2,2,3),(0.,1.),(0.,0.25,0.5,0.75,
1.),.UNSPECIFIED.)
GEOMETRIC_REPRESENTATION_ITEM()
RATIONAL_B_SPLINE_SURFACE(((1.,0.974927912181824,1.,0.974927912181824,1.,
0.974927912181824,1.,0.974927912181824,1.),(0.987189825241073,0.962438915249418,
0.987189825241073,0.962438915249418,0.987189825241073,0.962438915249418,
0.987189825241073,0.962438915249418,0.987189825241073),(0.987189825241073,
0.962438915249418,0.987189825241073,0.962438915249418,0.987189825241073,
0.962438915249418,0.987189825241073,0.962438915249418,0.987189825241073),
(1.,0.974927912181824,1.,0.974927912181824,1.,0.974927912181824,1.,0.974927912181824,
1.)))
REPRESENTATION_ITEM('')
SURFACE()
);
#380=(
BOUNDED_SURFACE()
B_SPLINE_SURFACE(3,2,((#25715,#25716,#25717,#25718,#25719,#25720,#25721,
#25722,#25723),(#25724,#25725,#25726,#25727,#25728,#25729,#25730,#25731,
#25732),(#25733,#25734,#25735,#25736,#25737,#25738,#25739,#25740,#25741),
(#25742,#25743,#25744,#25745,#25746,#25747,#25748,#25749,#25750)),
 .UNSPECIFIED.,.F.,.F.,.F.)
B_SPLINE_SURFACE_WITH_KNOTS((4,4),(3,2,2,2,3),(0.,1.),(0.,0.25,0.5,0.75,
1.),.UNSPECIFIED.)
GEOMETRIC_REPRESENTATION_ITEM()
RATIONAL_B_SPLINE_SURFACE(((1.,0.974927912181824,1.,0.974927912181824,1.,
0.974927912181824,1.,0.974927912181824,1.),(0.987189825241073,0.962438915249418,
0.987189825241073,0.962438915249418,0.987189825241073,0.962438915249418,
0.987189825241073,0.962438915249418,0.987189825241073),(0.987189825241073,
0.962438915249418,0.987189825241073,0.962438915249418,0.987189825241073,
0.962438915249418,0.987189825241073,0.962438915249418,0.987189825241073),
(1.,0.974927912181824,1.,0.974927912181824,1.,0.974927912181824,1.,0.974927912181824,
1.)))
REPRESENTATION_ITEM('')
SURFACE()
);
#381=(
BOUNDED_SURFACE()
B_SPLINE_SURFACE(3,2,((#25758,#25759,#25760,#25761,#25762,#25763,#25764,
#25765,#25766),(#25767,#25768,#25769,#25770,#25771,#25772,#25773,#25774,
#25775),(#25776,#25777,#25778,#25779,#25780,#25781,#25782,#25783,#25784),
(#25785,#25786,#25787,#25788,#25789,#25790,#25791,#25792,#25793)),
 .UNSPECIFIED.,.F.,.F.,.F.)
B_SPLINE_SURFACE_WITH_KNOTS((4,4),(3,2,2,2,3),(0.,1.),(0.,0.25,0.5,0.75,
1.),.UNSPECIFIED.)
GEOMETRIC_REPRESENTATION_ITEM()
RATIONAL_B_SPLINE_SURFACE(((1.,0.974927912181824,1.,0.974927912181824,1.,
0.974927912181824,1.,0.974927912181824,1.),(0.833333333333333,0.812439926818186,
0.833333333333333,0.812439926818186,0.833333333333333,0.812439926818186,
0.833333333333333,0.812439926818186,0.833333333333333),(0.833333333333333,
0.812439926818186,0.833333333333333,0.812439926818186,0.833333333333333,
0.812439926818186,0.833333333333333,0.812439926818186,0.833333333333333),
(1.,0.974927912181824,1.,0.974927912181824,1.,0.974927912181824,1.,0.974927912181824,
1.)))
REPRESENTATION_ITEM('')
SURFACE()
);
#382=(
BOUNDED_SURFACE()
B_SPLINE_SURFACE(3,2,((#25797,#25798,#25799,#25800,#25801,#25802,#25803,
#25804,#25805),(#25806,#25807,#25808,#25809,#25810,#25811,#25812,#25813,
#25814),(#25815,#25816,#25817,#25818,#25819,#25820,#25821,#25822,#25823),
(#25824,#25825,#25826,#25827,#25828,#25829,#25830,#25831,#25832)),
 .UNSPECIFIED.,.F.,.F.,.F.)
B_SPLINE_SURFACE_WITH_KNOTS((4,4),(3,2,2,2,3),(0.,1.),(0.,0.25,0.5,0.75,
1.),.UNSPECIFIED.)
GEOMETRIC_REPRESENTATION_ITEM()
RATIONAL_B_SPLINE_SURFACE(((1.,0.974927912181824,1.,0.974927912181824,1.,
0.974927912181824,1.,0.974927912181824,1.),(0.987189825241073,0.962438915249418,
0.987189825241073,0.962438915249418,0.987189825241073,0.962438915249418,
0.987189825241073,0.962438915249418,0.987189825241073),(0.987189825241073,
0.962438915249418,0.987189825241073,0.962438915249418,0.987189825241073,
0.962438915249418,0.987189825241073,0.962438915249418,0.987189825241073),
(1.,0.974927912181824,1.,0.974927912181824,1.,0.974927912181824,1.,0.974927912181824,
1.)))
REPRESENTATION_ITEM('')
SURFACE()
);
#383=(
BOUNDED_SURFACE()
B_SPLINE_SURFACE(3,2,((#25887,#25888,#25889,#25890,#25891,#25892,#25893,
#25894,#25895),(#25896,#25897,#25898,#25899,#25900,#25901,#25902,#25903,
#25904),(#25905,#25906,#25907,#25908,#25909,#25910,#25911,#25912,#25913),
(#25914,#25915,#25916,#25917,#25918,#25919,#25920,#25921,#25922)),
 .UNSPECIFIED.,.F.,.F.,.F.)
B_SPLINE_SURFACE_WITH_KNOTS((4,4),(3,2,2,2,3),(0.,1.),(0.,0.25,0.5,0.75,
1.),.UNSPECIFIED.)
GEOMETRIC_REPRESENTATION_ITEM()
RATIONAL_B_SPLINE_SURFACE(((1.,0.974927912181824,1.,0.974927912181824,1.,
0.974927912181824,1.,0.974927912181824,1.),(0.987189825241073,0.962438915249418,
0.987189825241073,0.962438915249418,0.987189825241073,0.962438915249418,
0.987189825241073,0.962438915249418,0.987189825241073),(0.987189825241073,
0.962438915249418,0.987189825241073,0.962438915249418,0.987189825241073,
0.962438915249418,0.987189825241073,0.962438915249418,0.987189825241073),
(1.,0.974927912181824,1.,0.974927912181824,1.,0.974927912181824,1.,0.974927912181824,
1.)))
REPRESENTATION_ITEM('')
SURFACE()
);
#384=(
BOUNDED_SURFACE()
B_SPLINE_SURFACE(3,2,((#25930,#25931,#25932,#25933,#25934,#25935,#25936,
#25937,#25938),(#25939,#25940,#25941,#25942,#25943,#25944,#25945,#25946,
#25947),(#25948,#25949,#25950,#25951,#25952,#25953,#25954,#25955,#25956),
(#25957,#25958,#25959,#25960,#25961,#25962,#25963,#25964,#25965)),
 .UNSPECIFIED.,.F.,.F.,.F.)
B_SPLINE_SURFACE_WITH_KNOTS((4,4),(3,2,2,2,3),(0.,1.),(0.,0.25,0.5,0.75,
1.),.UNSPECIFIED.)
GEOMETRIC_REPRESENTATION_ITEM()
RATIONAL_B_SPLINE_SURFACE(((1.,0.974927912181824,1.,0.974927912181824,1.,
0.974927912181824,1.,0.974927912181824,1.),(0.833333333333333,0.812439926818186,
0.833333333333333,0.812439926818186,0.833333333333333,0.812439926818186,
0.833333333333333,0.812439926818186,0.833333333333333),(0.833333333333333,
0.812439926818186,0.833333333333333,0.812439926818186,0.833333333333333,
0.812439926818186,0.833333333333333,0.812439926818186,0.833333333333333),
(1.,0.974927912181824,1.,0.974927912181824,1.,0.974927912181824,1.,0.974927912181824,
1.)))
REPRESENTATION_ITEM('')
SURFACE()
);
#385=(
BOUNDED_SURFACE()
B_SPLINE_SURFACE(3,2,((#25969,#25970,#25971,#25972,#25973,#25974,#25975,
#25976,#25977),(#25978,#25979,#25980,#25981,#25982,#25983,#25984,#25985,
#25986),(#25987,#25988,#25989,#25990,#25991,#25992,#25993,#25994,#25995),
(#25996,#25997,#25998,#25999,#26000,#26001,#26002,#26003,#26004)),
 .UNSPECIFIED.,.F.,.F.,.F.)
B_SPLINE_SURFACE_WITH_KNOTS((4,4),(3,2,2,2,3),(0.,1.),(0.,0.25,0.5,0.75,
1.),.UNSPECIFIED.)
GEOMETRIC_REPRESENTATION_ITEM()
RATIONAL_B_SPLINE_SURFACE(((1.,0.974927912181824,1.,0.974927912181824,1.,
0.974927912181824,1.,0.974927912181824,1.),(0.987189825241073,0.962438915249418,
0.987189825241073,0.962438915249418,0.987189825241073,0.962438915249418,
0.987189825241073,0.962438915249418,0.987189825241073),(0.987189825241073,
0.962438915249418,0.987189825241073,0.962438915249418,0.987189825241073,
0.962438915249418,0.987189825241073,0.962438915249418,0.987189825241073),
(1.,0.974927912181824,1.,0.974927912181824,1.,0.974927912181824,1.,0.974927912181824,
1.)))
REPRESENTATION_ITEM('')
SURFACE()
);
#386=(
BOUNDED_SURFACE()
B_SPLINE_SURFACE(3,2,((#26059,#26060,#26061,#26062,#26063,#26064,#26065,
#26066,#26067),(#26068,#26069,#26070,#26071,#26072,#26073,#26074,#26075,
#26076),(#26077,#26078,#26079,#26080,#26081,#26082,#26083,#26084,#26085),
(#26086,#26087,#26088,#26089,#26090,#26091,#26092,#26093,#26094)),
 .UNSPECIFIED.,.F.,.F.,.F.)
B_SPLINE_SURFACE_WITH_KNOTS((4,4),(3,2,2,2,3),(0.,1.),(0.,0.25,0.5,0.75,
1.),.UNSPECIFIED.)
GEOMETRIC_REPRESENTATION_ITEM()
RATIONAL_B_SPLINE_SURFACE(((1.,0.974927912181824,1.,0.974927912181824,1.,
0.974927912181824,1.,0.974927912181824,1.),(0.987189825241073,0.962438915249418,
0.987189825241073,0.962438915249418,0.987189825241073,0.962438915249418,
0.987189825241073,0.962438915249418,0.987189825241073),(0.987189825241073,
0.962438915249418,0.987189825241073,0.962438915249418,0.987189825241073,
0.962438915249418,0.987189825241073,0.962438915249418,0.987189825241073),
(1.,0.974927912181824,1.,0.974927912181824,1.,0.974927912181824,1.,0.974927912181824,
1.)))
REPRESENTATION_ITEM('')
SURFACE()
);
#387=(
BOUNDED_SURFACE()
B_SPLINE_SURFACE(3,2,((#26102,#26103,#26104,#26105,#26106,#26107,#26108,
#26109,#26110),(#26111,#26112,#26113,#26114,#26115,#26116,#26117,#26118,
#26119),(#26120,#26121,#26122,#26123,#26124,#26125,#26126,#26127,#26128),
(#26129,#26130,#26131,#26132,#26133,#26134,#26135,#26136,#26137)),
 .UNSPECIFIED.,.F.,.F.,.F.)
B_SPLINE_SURFACE_WITH_KNOTS((4,4),(3,2,2,2,3),(0.,1.),(0.,0.25,0.5,0.75,
1.),.UNSPECIFIED.)
GEOMETRIC_REPRESENTATION_ITEM()
RATIONAL_B_SPLINE_SURFACE(((1.,0.974927912181824,1.,0.974927912181824,1.,
0.974927912181824,1.,0.974927912181824,1.),(0.833333333333332,0.812439926818185,
0.833333333333332,0.812439926818185,0.833333333333332,0.812439926818185,
0.833333333333332,0.812439926818185,0.833333333333332),(0.833333333333332,
0.812439926818185,0.833333333333332,0.812439926818185,0.833333333333332,
0.812439926818185,0.833333333333332,0.812439926818185,0.833333333333332),
(1.,0.974927912181824,1.,0.974927912181824,1.,0.974927912181824,1.,0.974927912181824,
1.)))
REPRESENTATION_ITEM('')
SURFACE()
);
#388=(
BOUNDED_SURFACE()
B_SPLINE_SURFACE(3,2,((#26141,#26142,#26143,#26144,#26145,#26146,#26147,
#26148,#26149),(#26150,#26151,#26152,#26153,#26154,#26155,#26156,#26157,
#26158),(#26159,#26160,#26161,#26162,#26163,#26164,#26165,#26166,#26167),
(#26168,#26169,#26170,#26171,#26172,#26173,#26174,#26175,#26176)),
 .UNSPECIFIED.,.F.,.F.,.F.)
B_SPLINE_SURFACE_WITH_KNOTS((4,4),(3,2,2,2,3),(0.,1.),(0.,0.25,0.5,0.75,
1.),.UNSPECIFIED.)
GEOMETRIC_REPRESENTATION_ITEM()
RATIONAL_B_SPLINE_SURFACE(((1.,0.974927912181824,1.,0.974927912181824,1.,
0.974927912181824,1.,0.974927912181824,1.),(0.987189825241073,0.962438915249418,
0.987189825241073,0.962438915249418,0.987189825241073,0.962438915249418,
0.987189825241073,0.962438915249418,0.987189825241073),(0.987189825241073,
0.962438915249418,0.987189825241073,0.962438915249418,0.987189825241073,
0.962438915249418,0.987189825241073,0.962438915249418,0.987189825241073),
(1.,0.974927912181824,1.,0.974927912181824,1.,0.974927912181824,1.,0.974927912181824,
1.)))
REPRESENTATION_ITEM('')
SURFACE()
);
#389=(
BOUNDED_SURFACE()
B_SPLINE_SURFACE(3,2,((#26231,#26232,#26233,#26234,#26235,#26236,#26237,
#26238,#26239),(#26240,#26241,#26242,#26243,#26244,#26245,#26246,#26247,
#26248),(#26249,#26250,#26251,#26252,#26253,#26254,#26255,#26256,#26257),
(#26258,#26259,#26260,#26261,#26262,#26263,#26264,#26265,#26266)),
 .UNSPECIFIED.,.F.,.F.,.F.)
B_SPLINE_SURFACE_WITH_KNOTS((4,4),(3,2,2,2,3),(0.,1.),(0.,0.25,0.5,0.75,
1.),.UNSPECIFIED.)
GEOMETRIC_REPRESENTATION_ITEM()
RATIONAL_B_SPLINE_SURFACE(((1.,0.974927912181824,1.,0.974927912181824,1.,
0.974927912181824,1.,0.974927912181824,1.),(0.987189825241073,0.962438915249418,
0.987189825241073,0.962438915249418,0.987189825241073,0.962438915249418,
0.987189825241073,0.962438915249418,0.987189825241073),(0.987189825241073,
0.962438915249418,0.987189825241073,0.962438915249418,0.987189825241073,
0.962438915249418,0.987189825241073,0.962438915249418,0.987189825241073),
(1.,0.974927912181824,1.,0.974927912181824,1.,0.974927912181824,1.,0.974927912181824,
1.)))
REPRESENTATION_ITEM('')
SURFACE()
);
#390=(
BOUNDED_SURFACE()
B_SPLINE_SURFACE(3,2,((#26274,#26275,#26276,#26277,#26278,#26279,#26280,
#26281,#26282),(#26283,#26284,#26285,#26286,#26287,#26288,#26289,#26290,
#26291),(#26292,#26293,#26294,#26295,#26296,#26297,#26298,#26299,#26300),
(#26301,#26302,#26303,#26304,#26305,#26306,#26307,#26308,#26309)),
 .UNSPECIFIED.,.F.,.F.,.F.)
B_SPLINE_SURFACE_WITH_KNOTS((4,4),(3,2,2,2,3),(0.,1.),(0.,0.25,0.5,0.75,
1.),.UNSPECIFIED.)
GEOMETRIC_REPRESENTATION_ITEM()
RATIONAL_B_SPLINE_SURFACE(((1.,0.974927912181824,1.,0.974927912181824,1.,
0.974927912181824,1.,0.974927912181824,1.),(0.833333333333333,0.812439926818186,
0.833333333333333,0.812439926818186,0.833333333333333,0.812439926818186,
0.833333333333333,0.812439926818186,0.833333333333333),(0.833333333333333,
0.812439926818186,0.833333333333333,0.812439926818186,0.833333333333333,
0.812439926818186,0.833333333333333,0.812439926818186,0.833333333333333),
(1.,0.974927912181824,1.,0.974927912181824,1.,0.974927912181824,1.,0.974927912181824,
1.)))
REPRESENTATION_ITEM('')
SURFACE()
);
#391=(
BOUNDED_SURFACE()
B_SPLINE_SURFACE(3,2,((#26313,#26314,#26315,#26316,#26317,#26318,#26319,
#26320,#26321),(#26322,#26323,#26324,#26325,#26326,#26327,#26328,#26329,
#26330),(#26331,#26332,#26333,#26334,#26335,#26336,#26337,#26338,#26339),
(#26340,#26341,#26342,#26343,#26344,#26345,#26346,#26347,#26348)),
 .UNSPECIFIED.,.F.,.F.,.F.)
B_SPLINE_SURFACE_WITH_KNOTS((4,4),(3,2,2,2,3),(0.,1.),(0.,0.25,0.5,0.75,
1.),.UNSPECIFIED.)
GEOMETRIC_REPRESENTATION_ITEM()
RATIONAL_B_SPLINE_SURFACE(((1.,0.974927912181824,1.,0.974927912181824,1.,
0.974927912181824,1.,0.974927912181824,1.),(0.987189825241073,0.962438915249418,
0.987189825241073,0.962438915249418,0.987189825241073,0.962438915249418,
0.987189825241073,0.962438915249418,0.987189825241073),(0.987189825241073,
0.962438915249418,0.987189825241073,0.962438915249418,0.987189825241073,
0.962438915249418,0.987189825241073,0.962438915249418,0.987189825241073),
(1.,0.974927912181824,1.,0.974927912181824,1.,0.974927912181824,1.,0.974927912181824,
1.)))
REPRESENTATION_ITEM('')
SURFACE()
);
#392=(
BOUNDED_SURFACE()
B_SPLINE_SURFACE(3,2,((#26403,#26404,#26405,#26406,#26407,#26408,#26409,
#26410,#26411),(#26412,#26413,#26414,#26415,#26416,#26417,#26418,#26419,
#26420),(#26421,#26422,#26423,#26424,#26425,#26426,#26427,#26428,#26429),
(#26430,#26431,#26432,#26433,#26434,#26435,#26436,#26437,#26438)),
 .UNSPECIFIED.,.F.,.F.,.F.)
B_SPLINE_SURFACE_WITH_KNOTS((4,4),(3,2,2,2,3),(0.,1.),(0.,0.25,0.5,0.75,
1.),.UNSPECIFIED.)
GEOMETRIC_REPRESENTATION_ITEM()
RATIONAL_B_SPLINE_SURFACE(((1.,0.974927912181824,1.,0.974927912181824,1.,
0.974927912181824,1.,0.974927912181824,1.),(0.987189825241073,0.962438915249418,
0.987189825241073,0.962438915249418,0.987189825241073,0.962438915249418,
0.987189825241073,0.962438915249418,0.987189825241073),(0.987189825241073,
0.962438915249418,0.987189825241073,0.962438915249418,0.987189825241073,
0.962438915249418,0.987189825241073,0.962438915249418,0.987189825241073),
(1.,0.974927912181824,1.,0.974927912181824,1.,0.974927912181824,1.,0.974927912181824,
1.)))
REPRESENTATION_ITEM('')
SURFACE()
);
#393=(
BOUNDED_SURFACE()
B_SPLINE_SURFACE(3,2,((#26446,#26447,#26448,#26449,#26450,#26451,#26452,
#26453,#26454),(#26455,#26456,#26457,#26458,#26459,#26460,#26461,#26462,
#26463),(#26464,#26465,#26466,#26467,#26468,#26469,#26470,#26471,#26472),
(#26473,#26474,#26475,#26476,#26477,#26478,#26479,#26480,#26481)),
 .UNSPECIFIED.,.F.,.F.,.F.)
B_SPLINE_SURFACE_WITH_KNOTS((4,4),(3,2,2,2,3),(0.,1.),(0.,0.25,0.5,0.75,
1.),.UNSPECIFIED.)
GEOMETRIC_REPRESENTATION_ITEM()
RATIONAL_B_SPLINE_SURFACE(((1.,0.974927912181824,1.,0.974927912181824,1.,
0.974927912181824,1.,0.974927912181824,1.),(0.833333333333332,0.812439926818185,
0.833333333333332,0.812439926818185,0.833333333333332,0.812439926818185,
0.833333333333332,0.812439926818185,0.833333333333332),(0.833333333333332,
0.812439926818185,0.833333333333332,0.812439926818185,0.833333333333332,
0.812439926818185,0.833333333333332,0.812439926818185,0.833333333333332),
(1.,0.974927912181824,1.,0.974927912181824,1.,0.974927912181824,1.,0.974927912181824,
1.)))
REPRESENTATION_ITEM('')
SURFACE()
);
#394=(
BOUNDED_SURFACE()
B_SPLINE_SURFACE(3,2,((#26485,#26486,#26487,#26488,#26489,#26490,#26491,
#26492,#26493),(#26494,#26495,#26496,#26497,#26498,#26499,#26500,#26501,
#26502),(#26503,#26504,#26505,#26506,#26507,#26508,#26509,#26510,#26511),
(#26512,#26513,#26514,#26515,#26516,#26517,#26518,#26519,#26520)),
 .UNSPECIFIED.,.F.,.F.,.F.)
B_SPLINE_SURFACE_WITH_KNOTS((4,4),(3,2,2,2,3),(0.,1.),(0.,0.25,0.5,0.75,
1.),.UNSPECIFIED.)
GEOMETRIC_REPRESENTATION_ITEM()
RATIONAL_B_SPLINE_SURFACE(((1.,0.974927912181824,1.,0.974927912181824,1.,
0.974927912181824,1.,0.974927912181824,1.),(0.987189825241073,0.962438915249418,
0.987189825241073,0.962438915249418,0.987189825241073,0.962438915249418,
0.987189825241073,0.962438915249418,0.987189825241073),(0.987189825241073,
0.962438915249418,0.987189825241073,0.962438915249418,0.987189825241073,
0.962438915249418,0.987189825241073,0.962438915249418,0.987189825241073),
(1.,0.974927912181824,1.,0.974927912181824,1.,0.974927912181824,1.,0.974927912181824,
1.)))
REPRESENTATION_ITEM('')
SURFACE()
);
#395=(
BOUNDED_SURFACE()
B_SPLINE_SURFACE(3,2,((#26575,#26576,#26577,#26578,#26579,#26580,#26581,
#26582,#26583),(#26584,#26585,#26586,#26587,#26588,#26589,#26590,#26591,
#26592),(#26593,#26594,#26595,#26596,#26597,#26598,#26599,#26600,#26601),
(#26602,#26603,#26604,#26605,#26606,#26607,#26608,#26609,#26610)),
 .UNSPECIFIED.,.F.,.F.,.F.)
B_SPLINE_SURFACE_WITH_KNOTS((4,4),(3,2,2,2,3),(0.,1.),(0.,0.25,0.5,0.75,
1.),.UNSPECIFIED.)
GEOMETRIC_REPRESENTATION_ITEM()
RATIONAL_B_SPLINE_SURFACE(((1.,0.974927912181824,1.,0.974927912181824,1.,
0.974927912181824,1.,0.974927912181824,1.),(0.987189825241073,0.962438915249418,
0.987189825241073,0.962438915249418,0.987189825241073,0.962438915249418,
0.987189825241073,0.962438915249418,0.987189825241073),(0.987189825241073,
0.962438915249418,0.987189825241073,0.962438915249418,0.987189825241073,
0.962438915249418,0.987189825241073,0.962438915249418,0.987189825241073),
(1.,0.974927912181824,1.,0.974927912181824,1.,0.974927912181824,1.,0.974927912181824,
1.)))
REPRESENTATION_ITEM('')
SURFACE()
);
#396=(
BOUNDED_SURFACE()
B_SPLINE_SURFACE(3,2,((#26618,#26619,#26620,#26621,#26622,#26623,#26624,
#26625,#26626),(#26627,#26628,#26629,#26630,#26631,#26632,#26633,#26634,
#26635),(#26636,#26637,#26638,#26639,#26640,#26641,#26642,#26643,#26644),
(#26645,#26646,#26647,#26648,#26649,#26650,#26651,#26652,#26653)),
 .UNSPECIFIED.,.F.,.F.,.F.)
B_SPLINE_SURFACE_WITH_KNOTS((4,4),(3,2,2,2,3),(0.,1.),(0.,0.25,0.5,0.75,
1.),.UNSPECIFIED.)
GEOMETRIC_REPRESENTATION_ITEM()
RATIONAL_B_SPLINE_SURFACE(((1.,0.974927912181824,1.,0.974927912181824,1.,
0.974927912181824,1.,0.974927912181824,1.),(0.833333333333333,0.812439926818186,
0.833333333333333,0.812439926818186,0.833333333333333,0.812439926818186,
0.833333333333333,0.812439926818186,0.833333333333333),(0.833333333333333,
0.812439926818186,0.833333333333333,0.812439926818186,0.833333333333333,
0.812439926818186,0.833333333333333,0.812439926818186,0.833333333333333),
(1.,0.974927912181824,1.,0.974927912181824,1.,0.974927912181824,1.,0.974927912181824,
1.)))
REPRESENTATION_ITEM('')
SURFACE()
);
#397=(
BOUNDED_SURFACE()
B_SPLINE_SURFACE(3,2,((#26657,#26658,#26659,#26660,#26661,#26662,#26663,
#26664,#26665),(#26666,#26667,#26668,#26669,#26670,#26671,#26672,#26673,
#26674),(#26675,#26676,#26677,#26678,#26679,#26680,#26681,#26682,#26683),
(#26684,#26685,#26686,#26687,#26688,#26689,#26690,#26691,#26692)),
 .UNSPECIFIED.,.F.,.F.,.F.)
B_SPLINE_SURFACE_WITH_KNOTS((4,4),(3,2,2,2,3),(0.,1.),(0.,0.25,0.5,0.75,
1.),.UNSPECIFIED.)
GEOMETRIC_REPRESENTATION_ITEM()
RATIONAL_B_SPLINE_SURFACE(((1.,0.974927912181824,1.,0.974927912181824,1.,
0.974927912181824,1.,0.974927912181824,1.),(0.987189825241073,0.962438915249418,
0.987189825241073,0.962438915249418,0.987189825241073,0.962438915249418,
0.987189825241073,0.962438915249418,0.987189825241073),(0.987189825241073,
0.962438915249418,0.987189825241073,0.962438915249418,0.987189825241073,
0.962438915249418,0.987189825241073,0.962438915249418,0.987189825241073),
(1.,0.974927912181824,1.,0.974927912181824,1.,0.974927912181824,1.,0.974927912181824,
1.)))
REPRESENTATION_ITEM('')
SURFACE()
);
#398=(
BOUNDED_SURFACE()
B_SPLINE_SURFACE(3,2,((#26747,#26748,#26749,#26750,#26751,#26752,#26753,
#26754,#26755),(#26756,#26757,#26758,#26759,#26760,#26761,#26762,#26763,
#26764),(#26765,#26766,#26767,#26768,#26769,#26770,#26771,#26772,#26773),
(#26774,#26775,#26776,#26777,#26778,#26779,#26780,#26781,#26782)),
 .UNSPECIFIED.,.F.,.F.,.F.)
B_SPLINE_SURFACE_WITH_KNOTS((4,4),(3,2,2,2,3),(0.,1.),(0.,0.25,0.5,0.75,
1.),.UNSPECIFIED.)
GEOMETRIC_REPRESENTATION_ITEM()
RATIONAL_B_SPLINE_SURFACE(((1.,0.974927912181824,1.,0.974927912181824,1.,
0.974927912181824,1.,0.974927912181824,1.),(0.987189825241073,0.962438915249418,
0.987189825241073,0.962438915249418,0.987189825241073,0.962438915249418,
0.987189825241073,0.962438915249418,0.987189825241073),(0.987189825241073,
0.962438915249418,0.987189825241073,0.962438915249418,0.987189825241073,
0.962438915249418,0.987189825241073,0.962438915249418,0.987189825241073),
(1.,0.974927912181824,1.,0.974927912181824,1.,0.974927912181824,1.,0.974927912181824,
1.)))
REPRESENTATION_ITEM('')
SURFACE()
);
#399=(
BOUNDED_SURFACE()
B_SPLINE_SURFACE(3,2,((#26790,#26791,#26792,#26793,#26794,#26795,#26796,
#26797,#26798),(#26799,#26800,#26801,#26802,#26803,#26804,#26805,#26806,
#26807),(#26808,#26809,#26810,#26811,#26812,#26813,#26814,#26815,#26816),
(#26817,#26818,#26819,#26820,#26821,#26822,#26823,#26824,#26825)),
 .UNSPECIFIED.,.F.,.F.,.F.)
B_SPLINE_SURFACE_WITH_KNOTS((4,4),(3,2,2,2,3),(0.,1.),(0.,0.25,0.5,0.75,
1.),.UNSPECIFIED.)
GEOMETRIC_REPRESENTATION_ITEM()
RATIONAL_B_SPLINE_SURFACE(((1.,0.974927912181824,1.,0.974927912181824,1.,
0.974927912181824,1.,0.974927912181824,1.),(0.833333333333332,0.812439926818185,
0.833333333333332,0.812439926818185,0.833333333333332,0.812439926818185,
0.833333333333332,0.812439926818185,0.833333333333332),(0.833333333333332,
0.812439926818185,0.833333333333332,0.812439926818185,0.833333333333332,
0.812439926818185,0.833333333333332,0.812439926818185,0.833333333333332),
(1.,0.974927912181824,1.,0.974927912181824,1.,0.974927912181824,1.,0.974927912181824,
1.)))
REPRESENTATION_ITEM('')
SURFACE()
);
#400=(
BOUNDED_SURFACE()
B_SPLINE_SURFACE(3,2,((#26829,#26830,#26831,#26832,#26833,#26834,#26835,
#26836,#26837),(#26838,#26839,#26840,#26841,#26842,#26843,#26844,#26845,
#26846),(#26847,#26848,#26849,#26850,#26851,#26852,#26853,#26854,#26855),
(#26856,#26857,#26858,#26859,#26860,#26861,#26862,#26863,#26864)),
 .UNSPECIFIED.,.F.,.F.,.F.)
B_SPLINE_SURFACE_WITH_KNOTS((4,4),(3,2,2,2,3),(0.,1.),(0.,0.25,0.5,0.75,
1.),.UNSPECIFIED.)
GEOMETRIC_REPRESENTATION_ITEM()
RATIONAL_B_SPLINE_SURFACE(((1.,0.974927912181824,1.,0.974927912181824,1.,
0.974927912181824,1.,0.974927912181824,1.),(0.987189825241073,0.962438915249418,
0.987189825241073,0.962438915249418,0.987189825241073,0.962438915249418,
0.987189825241073,0.962438915249418,0.987189825241073),(0.987189825241073,
0.962438915249418,0.987189825241073,0.962438915249418,0.987189825241073,
0.962438915249418,0.987189825241073,0.962438915249418,0.987189825241073),
(1.,0.974927912181824,1.,0.974927912181824,1.,0.974927912181824,1.,0.974927912181824,
1.)))
REPRESENTATION_ITEM('')
SURFACE()
);
#401=(
BOUNDED_SURFACE()
B_SPLINE_SURFACE(3,2,((#26919,#26920,#26921,#26922,#26923,#26924,#26925,
#26926,#26927),(#26928,#26929,#26930,#26931,#26932,#26933,#26934,#26935,
#26936),(#26937,#26938,#26939,#26940,#26941,#26942,#26943,#26944,#26945),
(#26946,#26947,#26948,#26949,#26950,#26951,#26952,#26953,#26954)),
 .UNSPECIFIED.,.F.,.F.,.F.)
B_SPLINE_SURFACE_WITH_KNOTS((4,4),(3,2,2,2,3),(0.,1.),(0.,0.25,0.5,0.75,
1.),.UNSPECIFIED.)
GEOMETRIC_REPRESENTATION_ITEM()
RATIONAL_B_SPLINE_SURFACE(((1.,0.974927912181824,1.,0.974927912181824,1.,
0.974927912181824,1.,0.974927912181824,1.),(0.987189825241073,0.962438915249418,
0.987189825241073,0.962438915249418,0.987189825241073,0.962438915249418,
0.987189825241073,0.962438915249418,0.987189825241073),(0.987189825241073,
0.962438915249418,0.987189825241073,0.962438915249418,0.987189825241073,
0.962438915249418,0.987189825241073,0.962438915249418,0.987189825241073),
(1.,0.974927912181824,1.,0.974927912181824,1.,0.974927912181824,1.,0.974927912181824,
1.)))
REPRESENTATION_ITEM('')
SURFACE()
);
#402=(
BOUNDED_SURFACE()
B_SPLINE_SURFACE(3,2,((#26962,#26963,#26964,#26965,#26966,#26967,#26968,
#26969,#26970),(#26971,#26972,#26973,#26974,#26975,#26976,#26977,#26978,
#26979),(#26980,#26981,#26982,#26983,#26984,#26985,#26986,#26987,#26988),
(#26989,#26990,#26991,#26992,#26993,#26994,#26995,#26996,#26997)),
 .UNSPECIFIED.,.F.,.F.,.F.)
B_SPLINE_SURFACE_WITH_KNOTS((4,4),(3,2,2,2,3),(0.,1.),(0.,0.25,0.5,0.75,
1.),.UNSPECIFIED.)
GEOMETRIC_REPRESENTATION_ITEM()
RATIONAL_B_SPLINE_SURFACE(((1.,0.974927912181824,1.,0.974927912181824,1.,
0.974927912181824,1.,0.974927912181824,1.),(0.833333333333332,0.812439926818185,
0.833333333333332,0.812439926818185,0.833333333333332,0.812439926818185,
0.833333333333332,0.812439926818185,0.833333333333332),(0.833333333333332,
0.812439926818185,0.833333333333332,0.812439926818185,0.833333333333332,
0.812439926818185,0.833333333333332,0.812439926818185,0.833333333333332),
(1.,0.974927912181824,1.,0.974927912181824,1.,0.974927912181824,1.,0.974927912181824,
1.)))
REPRESENTATION_ITEM('')
SURFACE()
);
#403=(
BOUNDED_SURFACE()
B_SPLINE_SURFACE(3,2,((#27001,#27002,#27003,#27004,#27005,#27006,#27007,
#27008,#27009),(#27010,#27011,#27012,#27013,#27014,#27015,#27016,#27017,
#27018),(#27019,#27020,#27021,#27022,#27023,#27024,#27025,#27026,#27027),
(#27028,#27029,#27030,#27031,#27032,#27033,#27034,#27035,#27036)),
 .UNSPECIFIED.,.F.,.F.,.F.)
B_SPLINE_SURFACE_WITH_KNOTS((4,4),(3,2,2,2,3),(0.,1.),(0.,0.25,0.5,0.75,
1.),.UNSPECIFIED.)
GEOMETRIC_REPRESENTATION_ITEM()
RATIONAL_B_SPLINE_SURFACE(((1.,0.974927912181824,1.,0.974927912181824,1.,
0.974927912181824,1.,0.974927912181824,1.),(0.987189825241073,0.962438915249418,
0.987189825241073,0.962438915249418,0.987189825241073,0.962438915249418,
0.987189825241073,0.962438915249418,0.987189825241073),(0.987189825241073,
0.962438915249418,0.987189825241073,0.962438915249418,0.987189825241073,
0.962438915249418,0.987189825241073,0.962438915249418,0.987189825241073),
(1.,0.974927912181824,1.,0.974927912181824,1.,0.974927912181824,1.,0.974927912181824,
1.)))
REPRESENTATION_ITEM('')
SURFACE()
);
#404=(
BOUNDED_SURFACE()
B_SPLINE_SURFACE(3,2,((#27091,#27092,#27093,#27094,#27095,#27096,#27097,
#27098,#27099),(#27100,#27101,#27102,#27103,#27104,#27105,#27106,#27107,
#27108),(#27109,#27110,#27111,#27112,#27113,#27114,#27115,#27116,#27117),
(#27118,#27119,#27120,#27121,#27122,#27123,#27124,#27125,#27126)),
 .UNSPECIFIED.,.F.,.F.,.F.)
B_SPLINE_SURFACE_WITH_KNOTS((4,4),(3,2,2,2,3),(0.,1.),(0.,0.25,0.5,0.75,
1.),.UNSPECIFIED.)
GEOMETRIC_REPRESENTATION_ITEM()
RATIONAL_B_SPLINE_SURFACE(((1.,0.974927912181824,1.,0.974927912181824,1.,
0.974927912181824,1.,0.974927912181824,1.),(0.987189825241073,0.962438915249418,
0.987189825241073,0.962438915249418,0.987189825241073,0.962438915249418,
0.987189825241073,0.962438915249418,0.987189825241073),(0.987189825241073,
0.962438915249418,0.987189825241073,0.962438915249418,0.987189825241073,
0.962438915249418,0.987189825241073,0.962438915249418,0.987189825241073),
(1.,0.974927912181824,1.,0.974927912181824,1.,0.974927912181824,1.,0.974927912181824,
1.)))
REPRESENTATION_ITEM('')
SURFACE()
);
#405=(
BOUNDED_SURFACE()
B_SPLINE_SURFACE(3,2,((#27134,#27135,#27136,#27137,#27138,#27139,#27140,
#27141,#27142),(#27143,#27144,#27145,#27146,#27147,#27148,#27149,#27150,
#27151),(#27152,#27153,#27154,#27155,#27156,#27157,#27158,#27159,#27160),
(#27161,#27162,#27163,#27164,#27165,#27166,#27167,#27168,#27169)),
 .UNSPECIFIED.,.F.,.F.,.F.)
B_SPLINE_SURFACE_WITH_KNOTS((4,4),(3,2,2,2,3),(0.,1.),(0.,0.25,0.5,0.75,
1.),.UNSPECIFIED.)
GEOMETRIC_REPRESENTATION_ITEM()
RATIONAL_B_SPLINE_SURFACE(((1.,0.974927912181824,1.,0.974927912181824,1.,
0.974927912181824,1.,0.974927912181824,1.),(0.833333333333332,0.812439926818185,
0.833333333333332,0.812439926818185,0.833333333333332,0.812439926818185,
0.833333333333332,0.812439926818185,0.833333333333332),(0.833333333333332,
0.812439926818185,0.833333333333332,0.812439926818185,0.833333333333332,
0.812439926818185,0.833333333333332,0.812439926818185,0.833333333333332),
(1.,0.974927912181824,1.,0.974927912181824,1.,0.974927912181824,1.,0.974927912181824,
1.)))
REPRESENTATION_ITEM('')
SURFACE()
);
#406=(
BOUNDED_SURFACE()
B_SPLINE_SURFACE(3,2,((#27173,#27174,#27175,#27176,#27177,#27178,#27179,
#27180,#27181),(#27182,#27183,#27184,#27185,#27186,#27187,#27188,#27189,
#27190),(#27191,#27192,#27193,#27194,#27195,#27196,#27197,#27198,#27199),
(#27200,#27201,#27202,#27203,#27204,#27205,#27206,#27207,#27208)),
 .UNSPECIFIED.,.F.,.F.,.F.)
B_SPLINE_SURFACE_WITH_KNOTS((4,4),(3,2,2,2,3),(0.,1.),(0.,0.25,0.5,0.75,
1.),.UNSPECIFIED.)
GEOMETRIC_REPRESENTATION_ITEM()
RATIONAL_B_SPLINE_SURFACE(((1.,0.974927912181824,1.,0.974927912181824,1.,
0.974927912181824,1.,0.974927912181824,1.),(0.987189825241073,0.962438915249418,
0.987189825241073,0.962438915249418,0.987189825241073,0.962438915249418,
0.987189825241073,0.962438915249418,0.987189825241073),(0.987189825241073,
0.962438915249418,0.987189825241073,0.962438915249418,0.987189825241073,
0.962438915249418,0.987189825241073,0.962438915249418,0.987189825241073),
(1.,0.974927912181824,1.,0.974927912181824,1.,0.974927912181824,1.,0.974927912181824,
1.)))
REPRESENTATION_ITEM('')
SURFACE()
);
#407=(
BOUNDED_SURFACE()
B_SPLINE_SURFACE(3,2,((#27216,#27217,#27218,#27219,#27220,#27221,#27222,
#27223,#27224),(#27225,#27226,#27227,#27228,#27229,#27230,#27231,#27232,
#27233),(#27234,#27235,#27236,#27237,#27238,#27239,#27240,#27241,#27242),
(#27243,#27244,#27245,#27246,#27247,#27248,#27249,#27250,#27251)),
 .UNSPECIFIED.,.F.,.F.,.F.)
B_SPLINE_SURFACE_WITH_KNOTS((4,4),(3,2,2,2,3),(0.,1.),(0.,0.25,0.5,0.75,
1.),.UNSPECIFIED.)
GEOMETRIC_REPRESENTATION_ITEM()
RATIONAL_B_SPLINE_SURFACE(((1.,0.974927912181824,1.,0.974927912181824,1.,
0.974927912181824,1.,0.974927912181824,1.),(0.987189825241073,0.962438915249418,
0.987189825241073,0.962438915249418,0.987189825241073,0.962438915249418,
0.987189825241073,0.962438915249418,0.987189825241073),(0.987189825241073,
0.962438915249418,0.987189825241073,0.962438915249418,0.987189825241073,
0.962438915249418,0.987189825241073,0.962438915249418,0.987189825241073),
(1.,0.974927912181824,1.,0.974927912181824,1.,0.974927912181824,1.,0.974927912181824,
1.)))
REPRESENTATION_ITEM('')
SURFACE()
);
#408=(
BOUNDED_SURFACE()
B_SPLINE_SURFACE(3,2,((#27259,#27260,#27261,#27262,#27263,#27264,#27265,
#27266,#27267),(#27268,#27269,#27270,#27271,#27272,#27273,#27274,#27275,
#27276),(#27277,#27278,#27279,#27280,#27281,#27282,#27283,#27284,#27285),
(#27286,#27287,#27288,#27289,#27290,#27291,#27292,#27293,#27294)),
 .UNSPECIFIED.,.F.,.F.,.F.)
B_SPLINE_SURFACE_WITH_KNOTS((4,4),(3,2,2,2,3),(0.,1.),(0.,0.25,0.5,0.75,
1.),.UNSPECIFIED.)
GEOMETRIC_REPRESENTATION_ITEM()
RATIONAL_B_SPLINE_SURFACE(((1.,0.974927912181824,1.,0.974927912181824,1.,
0.974927912181824,1.,0.974927912181824,1.),(0.833333333333332,0.812439926818185,
0.833333333333332,0.812439926818185,0.833333333333332,0.812439926818185,
0.833333333333332,0.812439926818185,0.833333333333332),(0.833333333333332,
0.812439926818185,0.833333333333332,0.812439926818185,0.833333333333332,
0.812439926818185,0.833333333333332,0.812439926818185,0.833333333333332),
(1.,0.974927912181824,1.,0.974927912181824,1.,0.974927912181824,1.,0.974927912181824,
1.)))
REPRESENTATION_ITEM('')
SURFACE()
);
#409=(
BOUNDED_SURFACE()
B_SPLINE_SURFACE(3,2,((#27298,#27299,#27300,#27301,#27302,#27303,#27304,
#27305,#27306),(#27307,#27308,#27309,#27310,#27311,#27312,#27313,#27314,
#27315),(#27316,#27317,#27318,#27319,#27320,#27321,#27322,#27323,#27324),
(#27325,#27326,#27327,#27328,#27329,#27330,#27331,#27332,#27333)),
 .UNSPECIFIED.,.F.,.F.,.F.)
B_SPLINE_SURFACE_WITH_KNOTS((4,4),(3,2,2,2,3),(0.,1.),(0.,0.25,0.5,0.75,
1.),.UNSPECIFIED.)
GEOMETRIC_REPRESENTATION_ITEM()
RATIONAL_B_SPLINE_SURFACE(((1.,0.974927912181824,1.,0.974927912181824,1.,
0.974927912181824,1.,0.974927912181824,1.),(0.987189825241073,0.962438915249418,
0.987189825241073,0.962438915249418,0.987189825241073,0.962438915249418,
0.987189825241073,0.962438915249418,0.987189825241073),(0.987189825241073,
0.962438915249418,0.987189825241073,0.962438915249418,0.987189825241073,
0.962438915249418,0.987189825241073,0.962438915249418,0.987189825241073),
(1.,0.974927912181824,1.,0.974927912181824,1.,0.974927912181824,1.,0.974927912181824,
1.)))
REPRESENTATION_ITEM('')
SURFACE()
);
#410=(
BOUNDED_SURFACE()
B_SPLINE_SURFACE(3,2,((#27341,#27342,#27343,#27344,#27345,#27346,#27347,
#27348,#27349),(#27350,#27351,#27352,#27353,#27354,#27355,#27356,#27357,
#27358),(#27359,#27360,#27361,#27362,#27363,#27364,#27365,#27366,#27367),
(#27368,#27369,#27370,#27371,#27372,#27373,#27374,#27375,#27376)),
 .UNSPECIFIED.,.F.,.F.,.F.)
B_SPLINE_SURFACE_WITH_KNOTS((4,4),(3,2,2,2,3),(0.,1.),(0.,0.25,0.5,0.75,
1.),.UNSPECIFIED.)
GEOMETRIC_REPRESENTATION_ITEM()
RATIONAL_B_SPLINE_SURFACE(((1.,0.974927912181824,1.,0.974927912181824,1.,
0.974927912181824,1.,0.974927912181824,1.),(0.987189825241073,0.962438915249418,
0.987189825241073,0.962438915249418,0.987189825241073,0.962438915249418,
0.987189825241073,0.962438915249418,0.987189825241073),(0.987189825241073,
0.962438915249418,0.987189825241073,0.962438915249418,0.987189825241073,
0.962438915249418,0.987189825241073,0.962438915249418,0.987189825241073),
(1.,0.974927912181824,1.,0.974927912181824,1.,0.974927912181824,1.,0.974927912181824,
1.)))
REPRESENTATION_ITEM('')
SURFACE()
);
#411=(
BOUNDED_SURFACE()
B_SPLINE_SURFACE(3,2,((#27384,#27385,#27386,#27387,#27388,#27389,#27390,
#27391,#27392),(#27393,#27394,#27395,#27396,#27397,#27398,#27399,#27400,
#27401),(#27402,#27403,#27404,#27405,#27406,#27407,#27408,#27409,#27410),
(#27411,#27412,#27413,#27414,#27415,#27416,#27417,#27418,#27419)),
 .UNSPECIFIED.,.F.,.F.,.F.)
B_SPLINE_SURFACE_WITH_KNOTS((4,4),(3,2,2,2,3),(0.,1.),(0.,0.25,0.5,0.75,
1.),.UNSPECIFIED.)
GEOMETRIC_REPRESENTATION_ITEM()
RATIONAL_B_SPLINE_SURFACE(((1.,0.974927912181824,1.,0.974927912181824,1.,
0.974927912181824,1.,0.974927912181824,1.),(0.833333333333333,0.812439926818186,
0.833333333333333,0.812439926818186,0.833333333333333,0.812439926818186,
0.833333333333333,0.812439926818186,0.833333333333333),(0.833333333333333,
0.812439926818186,0.833333333333333,0.812439926818186,0.833333333333333,
0.812439926818186,0.833333333333333,0.812439926818186,0.833333333333333),
(1.,0.974927912181824,1.,0.974927912181824,1.,0.974927912181824,1.,0.974927912181824,
1.)))
REPRESENTATION_ITEM('')
SURFACE()
);
#412=(
BOUNDED_SURFACE()
B_SPLINE_SURFACE(3,2,((#27423,#27424,#27425,#27426,#27427,#27428,#27429,
#27430,#27431),(#27432,#27433,#27434,#27435,#27436,#27437,#27438,#27439,
#27440),(#27441,#27442,#27443,#27444,#27445,#27446,#27447,#27448,#27449),
(#27450,#27451,#27452,#27453,#27454,#27455,#27456,#27457,#27458)),
 .UNSPECIFIED.,.F.,.F.,.F.)
B_SPLINE_SURFACE_WITH_KNOTS((4,4),(3,2,2,2,3),(0.,1.),(0.,0.25,0.5,0.75,
1.),.UNSPECIFIED.)
GEOMETRIC_REPRESENTATION_ITEM()
RATIONAL_B_SPLINE_SURFACE(((1.,0.974927912181824,1.,0.974927912181824,1.,
0.974927912181824,1.,0.974927912181824,1.),(0.987189825241073,0.962438915249418,
0.987189825241073,0.962438915249418,0.987189825241073,0.962438915249418,
0.987189825241073,0.962438915249418,0.987189825241073),(0.987189825241073,
0.962438915249418,0.987189825241073,0.962438915249418,0.987189825241073,
0.962438915249418,0.987189825241073,0.962438915249418,0.987189825241073),
(1.,0.974927912181824,1.,0.974927912181824,1.,0.974927912181824,1.,0.974927912181824,
1.)))
REPRESENTATION_ITEM('')
SURFACE()
);
#413=(
BOUNDED_SURFACE()
B_SPLINE_SURFACE(3,2,((#27513,#27514,#27515,#27516,#27517,#27518,#27519,
#27520,#27521),(#27522,#27523,#27524,#27525,#27526,#27527,#27528,#27529,
#27530),(#27531,#27532,#27533,#27534,#27535,#27536,#27537,#27538,#27539),
(#27540,#27541,#27542,#27543,#27544,#27545,#27546,#27547,#27548)),
 .UNSPECIFIED.,.F.,.F.,.F.)
B_SPLINE_SURFACE_WITH_KNOTS((4,4),(3,2,2,2,3),(0.,1.),(0.,0.25,0.5,0.75,
1.),.UNSPECIFIED.)
GEOMETRIC_REPRESENTATION_ITEM()
RATIONAL_B_SPLINE_SURFACE(((1.,0.974927912181824,1.,0.974927912181824,1.,
0.974927912181824,1.,0.974927912181824,1.),(0.987189825241073,0.962438915249418,
0.987189825241073,0.962438915249418,0.987189825241073,0.962438915249418,
0.987189825241073,0.962438915249418,0.987189825241073),(0.987189825241073,
0.962438915249418,0.987189825241073,0.962438915249418,0.987189825241073,
0.962438915249418,0.987189825241073,0.962438915249418,0.987189825241073),
(1.,0.974927912181824,1.,0.974927912181824,1.,0.974927912181824,1.,0.974927912181824,
1.)))
REPRESENTATION_ITEM('')
SURFACE()
);
#414=(
BOUNDED_SURFACE()
B_SPLINE_SURFACE(3,2,((#27556,#27557,#27558,#27559,#27560,#27561,#27562,
#27563,#27564),(#27565,#27566,#27567,#27568,#27569,#27570,#27571,#27572,
#27573),(#27574,#27575,#27576,#27577,#27578,#27579,#27580,#27581,#27582),
(#27583,#27584,#27585,#27586,#27587,#27588,#27589,#27590,#27591)),
 .UNSPECIFIED.,.F.,.F.,.F.)
B_SPLINE_SURFACE_WITH_KNOTS((4,4),(3,2,2,2,3),(0.,1.),(0.,0.25,0.5,0.75,
1.),.UNSPECIFIED.)
GEOMETRIC_REPRESENTATION_ITEM()
RATIONAL_B_SPLINE_SURFACE(((1.,0.974927912181824,1.,0.974927912181824,1.,
0.974927912181824,1.,0.974927912181824,1.),(0.833333333333333,0.812439926818186,
0.833333333333333,0.812439926818186,0.833333333333333,0.812439926818186,
0.833333333333333,0.812439926818186,0.833333333333333),(0.833333333333333,
0.812439926818186,0.833333333333333,0.812439926818186,0.833333333333333,
0.812439926818186,0.833333333333333,0.812439926818186,0.833333333333333),
(1.,0.974927912181824,1.,0.974927912181824,1.,0.974927912181824,1.,0.974927912181824,
1.)))
REPRESENTATION_ITEM('')
SURFACE()
);
#415=(
BOUNDED_SURFACE()
B_SPLINE_SURFACE(3,2,((#27595,#27596,#27597,#27598,#27599,#27600,#27601,
#27602,#27603),(#27604,#27605,#27606,#27607,#27608,#27609,#27610,#27611,
#27612),(#27613,#27614,#27615,#27616,#27617,#27618,#27619,#27620,#27621),
(#27622,#27623,#27624,#27625,#27626,#27627,#27628,#27629,#27630)),
 .UNSPECIFIED.,.F.,.F.,.F.)
B_SPLINE_SURFACE_WITH_KNOTS((4,4),(3,2,2,2,3),(0.,1.),(0.,0.25,0.5,0.75,
1.),.UNSPECIFIED.)
GEOMETRIC_REPRESENTATION_ITEM()
RATIONAL_B_SPLINE_SURFACE(((1.,0.974927912181824,1.,0.974927912181824,1.,
0.974927912181824,1.,0.974927912181824,1.),(0.987189825241073,0.962438915249418,
0.987189825241073,0.962438915249418,0.987189825241073,0.962438915249418,
0.987189825241073,0.962438915249418,0.987189825241073),(0.987189825241073,
0.962438915249418,0.987189825241073,0.962438915249418,0.987189825241073,
0.962438915249418,0.987189825241073,0.962438915249418,0.987189825241073),
(1.,0.974927912181824,1.,0.974927912181824,1.,0.974927912181824,1.,0.974927912181824,
1.)))
REPRESENTATION_ITEM('')
SURFACE()
);
#416=(
BOUNDED_SURFACE()
B_SPLINE_SURFACE(3,2,((#27685,#27686,#27687,#27688,#27689,#27690,#27691,
#27692,#27693),(#27694,#27695,#27696,#27697,#27698,#27699,#27700,#27701,
#27702),(#27703,#27704,#27705,#27706,#27707,#27708,#27709,#27710,#27711),
(#27712,#27713,#27714,#27715,#27716,#27717,#27718,#27719,#27720)),
 .UNSPECIFIED.,.F.,.F.,.F.)
B_SPLINE_SURFACE_WITH_KNOTS((4,4),(3,2,2,2,3),(0.,1.),(0.,0.25,0.5,0.75,
1.),.UNSPECIFIED.)
GEOMETRIC_REPRESENTATION_ITEM()
RATIONAL_B_SPLINE_SURFACE(((1.,0.974927912181824,1.,0.974927912181824,1.,
0.974927912181824,1.,0.974927912181824,1.),(0.987189825241073,0.962438915249418,
0.987189825241073,0.962438915249418,0.987189825241073,0.962438915249418,
0.987189825241073,0.962438915249418,0.987189825241073),(0.987189825241073,
0.962438915249418,0.987189825241073,0.962438915249418,0.987189825241073,
0.962438915249418,0.987189825241073,0.962438915249418,0.987189825241073),
(1.,0.974927912181824,1.,0.974927912181824,1.,0.974927912181824,1.,0.974927912181824,
1.)))
REPRESENTATION_ITEM('')
SURFACE()
);
#417=(
BOUNDED_SURFACE()
B_SPLINE_SURFACE(3,2,((#27728,#27729,#27730,#27731,#27732,#27733,#27734,
#27735,#27736),(#27737,#27738,#27739,#27740,#27741,#27742,#27743,#27744,
#27745),(#27746,#27747,#27748,#27749,#27750,#27751,#27752,#27753,#27754),
(#27755,#27756,#27757,#27758,#27759,#27760,#27761,#27762,#27763)),
 .UNSPECIFIED.,.F.,.F.,.F.)
B_SPLINE_SURFACE_WITH_KNOTS((4,4),(3,2,2,2,3),(0.,1.),(0.,0.25,0.5,0.75,
1.),.UNSPECIFIED.)
GEOMETRIC_REPRESENTATION_ITEM()
RATIONAL_B_SPLINE_SURFACE(((1.,0.974927912181824,1.,0.974927912181824,1.,
0.974927912181824,1.,0.974927912181824,1.),(0.833333333333332,0.812439926818185,
0.833333333333332,0.812439926818185,0.833333333333332,0.812439926818185,
0.833333333333332,0.812439926818185,0.833333333333332),(0.833333333333332,
0.812439926818185,0.833333333333332,0.812439926818185,0.833333333333332,
0.812439926818185,0.833333333333332,0.812439926818185,0.833333333333332),
(1.,0.974927912181824,1.,0.974927912181824,1.,0.974927912181824,1.,0.974927912181824,
1.)))
REPRESENTATION_ITEM('')
SURFACE()
);
#418=(
BOUNDED_SURFACE()
B_SPLINE_SURFACE(3,2,((#27767,#27768,#27769,#27770,#27771,#27772,#27773,
#27774,#27775),(#27776,#27777,#27778,#27779,#27780,#27781,#27782,#27783,
#27784),(#27785,#27786,#27787,#27788,#27789,#27790,#27791,#27792,#27793),
(#27794,#27795,#27796,#27797,#27798,#27799,#27800,#27801,#27802)),
 .UNSPECIFIED.,.F.,.F.,.F.)
B_SPLINE_SURFACE_WITH_KNOTS((4,4),(3,2,2,2,3),(0.,1.),(0.,0.25,0.5,0.75,
1.),.UNSPECIFIED.)
GEOMETRIC_REPRESENTATION_ITEM()
RATIONAL_B_SPLINE_SURFACE(((1.,0.974927912181824,1.,0.974927912181824,1.,
0.974927912181824,1.,0.974927912181824,1.),(0.987189825241073,0.962438915249418,
0.987189825241073,0.962438915249418,0.987189825241073,0.962438915249418,
0.987189825241073,0.962438915249418,0.987189825241073),(0.987189825241073,
0.962438915249418,0.987189825241073,0.962438915249418,0.987189825241073,
0.962438915249418,0.987189825241073,0.962438915249418,0.987189825241073),
(1.,0.974927912181824,1.,0.974927912181824,1.,0.974927912181824,1.,0.974927912181824,
1.)))
REPRESENTATION_ITEM('')
SURFACE()
);
#419=(
BOUNDED_SURFACE()
B_SPLINE_SURFACE(3,2,((#27857,#27858,#27859,#27860,#27861,#27862,#27863,
#27864,#27865),(#27866,#27867,#27868,#27869,#27870,#27871,#27872,#27873,
#27874),(#27875,#27876,#27877,#27878,#27879,#27880,#27881,#27882,#27883),
(#27884,#27885,#27886,#27887,#27888,#27889,#27890,#27891,#27892)),
 .UNSPECIFIED.,.F.,.F.,.F.)
B_SPLINE_SURFACE_WITH_KNOTS((4,4),(3,2,2,2,3),(0.,1.),(0.,0.25,0.5,0.75,
1.),.UNSPECIFIED.)
GEOMETRIC_REPRESENTATION_ITEM()
RATIONAL_B_SPLINE_SURFACE(((1.,0.974927912181824,1.,0.974927912181824,1.,
0.974927912181824,1.,0.974927912181824,1.),(0.987189825241073,0.962438915249418,
0.987189825241073,0.962438915249418,0.987189825241073,0.962438915249418,
0.987189825241073,0.962438915249418,0.987189825241073),(0.987189825241073,
0.962438915249418,0.987189825241073,0.962438915249418,0.987189825241073,
0.962438915249418,0.987189825241073,0.962438915249418,0.987189825241073),
(1.,0.974927912181824,1.,0.974927912181824,1.,0.974927912181824,1.,0.974927912181824,
1.)))
REPRESENTATION_ITEM('')
SURFACE()
);
#420=(
BOUNDED_SURFACE()
B_SPLINE_SURFACE(3,2,((#27900,#27901,#27902,#27903,#27904,#27905,#27906,
#27907,#27908),(#27909,#27910,#27911,#27912,#27913,#27914,#27915,#27916,
#27917),(#27918,#27919,#27920,#27921,#27922,#27923,#27924,#27925,#27926),
(#27927,#27928,#27929,#27930,#27931,#27932,#27933,#27934,#27935)),
 .UNSPECIFIED.,.F.,.F.,.F.)
B_SPLINE_SURFACE_WITH_KNOTS((4,4),(3,2,2,2,3),(0.,1.),(0.,0.25,0.5,0.75,
1.),.UNSPECIFIED.)
GEOMETRIC_REPRESENTATION_ITEM()
RATIONAL_B_SPLINE_SURFACE(((1.,0.974927912181824,1.,0.974927912181824,1.,
0.974927912181824,1.,0.974927912181824,1.),(0.833333333333333,0.812439926818186,
0.833333333333333,0.812439926818186,0.833333333333333,0.812439926818186,
0.833333333333333,0.812439926818186,0.833333333333333),(0.833333333333333,
0.812439926818186,0.833333333333333,0.812439926818186,0.833333333333333,
0.812439926818186,0.833333333333333,0.812439926818186,0.833333333333333),
(1.,0.974927912181824,1.,0.974927912181824,1.,0.974927912181824,1.,0.974927912181824,
1.)))
REPRESENTATION_ITEM('')
SURFACE()
);
#421=(
BOUNDED_SURFACE()
B_SPLINE_SURFACE(3,2,((#27939,#27940,#27941,#27942,#27943,#27944,#27945,
#27946,#27947),(#27948,#27949,#27950,#27951,#27952,#27953,#27954,#27955,
#27956),(#27957,#27958,#27959,#27960,#27961,#27962,#27963,#27964,#27965),
(#27966,#27967,#27968,#27969,#27970,#27971,#27972,#27973,#27974)),
 .UNSPECIFIED.,.F.,.F.,.F.)
B_SPLINE_SURFACE_WITH_KNOTS((4,4),(3,2,2,2,3),(0.,1.),(0.,0.25,0.5,0.75,
1.),.UNSPECIFIED.)
GEOMETRIC_REPRESENTATION_ITEM()
RATIONAL_B_SPLINE_SURFACE(((1.,0.974927912181824,1.,0.974927912181824,1.,
0.974927912181824,1.,0.974927912181824,1.),(0.987189825241073,0.962438915249418,
0.987189825241073,0.962438915249418,0.987189825241073,0.962438915249418,
0.987189825241073,0.962438915249418,0.987189825241073),(0.987189825241073,
0.962438915249418,0.987189825241073,0.962438915249418,0.987189825241073,
0.962438915249418,0.987189825241073,0.962438915249418,0.987189825241073),
(1.,0.974927912181824,1.,0.974927912181824,1.,0.974927912181824,1.,0.974927912181824,
1.)))
REPRESENTATION_ITEM('')
SURFACE()
);
#422=(
BOUNDED_SURFACE()
B_SPLINE_SURFACE(3,2,((#28029,#28030,#28031,#28032,#28033,#28034,#28035,
#28036,#28037),(#28038,#28039,#28040,#28041,#28042,#28043,#28044,#28045,
#28046),(#28047,#28048,#28049,#28050,#28051,#28052,#28053,#28054,#28055),
(#28056,#28057,#28058,#28059,#28060,#28061,#28062,#28063,#28064)),
 .UNSPECIFIED.,.F.,.F.,.F.)
B_SPLINE_SURFACE_WITH_KNOTS((4,4),(3,2,2,2,3),(0.,1.),(0.,0.25,0.5,0.75,
1.),.UNSPECIFIED.)
GEOMETRIC_REPRESENTATION_ITEM()
RATIONAL_B_SPLINE_SURFACE(((1.,0.974927912181824,1.,0.974927912181824,1.,
0.974927912181824,1.,0.974927912181824,1.),(0.987189825241073,0.962438915249418,
0.987189825241073,0.962438915249418,0.987189825241073,0.962438915249418,
0.987189825241073,0.962438915249418,0.987189825241073),(0.987189825241073,
0.962438915249418,0.987189825241073,0.962438915249418,0.987189825241073,
0.962438915249418,0.987189825241073,0.962438915249418,0.987189825241073),
(1.,0.974927912181824,1.,0.974927912181824,1.,0.974927912181824,1.,0.974927912181824,
1.)))
REPRESENTATION_ITEM('')
SURFACE()
);
#423=(
BOUNDED_SURFACE()
B_SPLINE_SURFACE(3,2,((#28072,#28073,#28074,#28075,#28076,#28077,#28078,
#28079,#28080),(#28081,#28082,#28083,#28084,#28085,#28086,#28087,#28088,
#28089),(#28090,#28091,#28092,#28093,#28094,#28095,#28096,#28097,#28098),
(#28099,#28100,#28101,#28102,#28103,#28104,#28105,#28106,#28107)),
 .UNSPECIFIED.,.F.,.F.,.F.)
B_SPLINE_SURFACE_WITH_KNOTS((4,4),(3,2,2,2,3),(0.,1.),(0.,0.25,0.5,0.75,
1.),.UNSPECIFIED.)
GEOMETRIC_REPRESENTATION_ITEM()
RATIONAL_B_SPLINE_SURFACE(((1.,0.974927912181824,1.,0.974927912181824,1.,
0.974927912181824,1.,0.974927912181824,1.),(0.833333333333332,0.812439926818185,
0.833333333333332,0.812439926818185,0.833333333333332,0.812439926818185,
0.833333333333332,0.812439926818185,0.833333333333332),(0.833333333333332,
0.812439926818185,0.833333333333332,0.812439926818185,0.833333333333332,
0.812439926818185,0.833333333333332,0.812439926818185,0.833333333333332),
(1.,0.974927912181824,1.,0.974927912181824,1.,0.974927912181824,1.,0.974927912181824,
1.)))
REPRESENTATION_ITEM('')
SURFACE()
);
#424=(
BOUNDED_SURFACE()
B_SPLINE_SURFACE(3,2,((#28111,#28112,#28113,#28114,#28115,#28116,#28117,
#28118,#28119),(#28120,#28121,#28122,#28123,#28124,#28125,#28126,#28127,
#28128),(#28129,#28130,#28131,#28132,#28133,#28134,#28135,#28136,#28137),
(#28138,#28139,#28140,#28141,#28142,#28143,#28144,#28145,#28146)),
 .UNSPECIFIED.,.F.,.F.,.F.)
B_SPLINE_SURFACE_WITH_KNOTS((4,4),(3,2,2,2,3),(0.,1.),(0.,0.25,0.5,0.75,
1.),.UNSPECIFIED.)
GEOMETRIC_REPRESENTATION_ITEM()
RATIONAL_B_SPLINE_SURFACE(((1.,0.974927912181824,1.,0.974927912181824,1.,
0.974927912181824,1.,0.974927912181824,1.),(0.987189825241073,0.962438915249418,
0.987189825241073,0.962438915249418,0.987189825241073,0.962438915249418,
0.987189825241073,0.962438915249418,0.987189825241073),(0.987189825241073,
0.962438915249418,0.987189825241073,0.962438915249418,0.987189825241073,
0.962438915249418,0.987189825241073,0.962438915249418,0.987189825241073),
(1.,0.974927912181824,1.,0.974927912181824,1.,0.974927912181824,1.,0.974927912181824,
1.)))
REPRESENTATION_ITEM('')
SURFACE()
);
#425=(
BOUNDED_SURFACE()
B_SPLINE_SURFACE(3,2,((#28201,#28202,#28203,#28204,#28205,#28206,#28207,
#28208,#28209),(#28210,#28211,#28212,#28213,#28214,#28215,#28216,#28217,
#28218),(#28219,#28220,#28221,#28222,#28223,#28224,#28225,#28226,#28227),
(#28228,#28229,#28230,#28231,#28232,#28233,#28234,#28235,#28236)),
 .UNSPECIFIED.,.F.,.F.,.F.)
B_SPLINE_SURFACE_WITH_KNOTS((4,4),(3,2,2,2,3),(0.,1.),(0.,0.25,0.5,0.75,
1.),.UNSPECIFIED.)
GEOMETRIC_REPRESENTATION_ITEM()
RATIONAL_B_SPLINE_SURFACE(((1.,0.974927912181824,1.,0.974927912181824,1.,
0.974927912181824,1.,0.974927912181824,1.),(0.987189825241073,0.962438915249418,
0.987189825241073,0.962438915249418,0.987189825241073,0.962438915249418,
0.987189825241073,0.962438915249418,0.987189825241073),(0.987189825241073,
0.962438915249418,0.987189825241073,0.962438915249418,0.987189825241073,
0.962438915249418,0.987189825241073,0.962438915249418,0.987189825241073),
(1.,0.974927912181824,1.,0.974927912181824,1.,0.974927912181824,1.,0.974927912181824,
1.)))
REPRESENTATION_ITEM('')
SURFACE()
);
#426=(
BOUNDED_SURFACE()
B_SPLINE_SURFACE(3,2,((#28244,#28245,#28246,#28247,#28248,#28249,#28250,
#28251,#28252),(#28253,#28254,#28255,#28256,#28257,#28258,#28259,#28260,
#28261),(#28262,#28263,#28264,#28265,#28266,#28267,#28268,#28269,#28270),
(#28271,#28272,#28273,#28274,#28275,#28276,#28277,#28278,#28279)),
 .UNSPECIFIED.,.F.,.F.,.F.)
B_SPLINE_SURFACE_WITH_KNOTS((4,4),(3,2,2,2,3),(0.,1.),(0.,0.25,0.5,0.75,
1.),.UNSPECIFIED.)
GEOMETRIC_REPRESENTATION_ITEM()
RATIONAL_B_SPLINE_SURFACE(((1.,0.974927912181824,1.,0.974927912181824,1.,
0.974927912181824,1.,0.974927912181824,1.),(0.833333333333333,0.812439926818186,
0.833333333333333,0.812439926818186,0.833333333333333,0.812439926818186,
0.833333333333333,0.812439926818186,0.833333333333333),(0.833333333333333,
0.812439926818186,0.833333333333333,0.812439926818186,0.833333333333333,
0.812439926818186,0.833333333333333,0.812439926818186,0.833333333333333),
(1.,0.974927912181824,1.,0.974927912181824,1.,0.974927912181824,1.,0.974927912181824,
1.)))
REPRESENTATION_ITEM('')
SURFACE()
);
#427=(
BOUNDED_SURFACE()
B_SPLINE_SURFACE(3,2,((#28283,#28284,#28285,#28286,#28287,#28288,#28289,
#28290,#28291),(#28292,#28293,#28294,#28295,#28296,#28297,#28298,#28299,
#28300),(#28301,#28302,#28303,#28304,#28305,#28306,#28307,#28308,#28309),
(#28310,#28311,#28312,#28313,#28314,#28315,#28316,#28317,#28318)),
 .UNSPECIFIED.,.F.,.F.,.F.)
B_SPLINE_SURFACE_WITH_KNOTS((4,4),(3,2,2,2,3),(0.,1.),(0.,0.25,0.5,0.75,
1.),.UNSPECIFIED.)
GEOMETRIC_REPRESENTATION_ITEM()
RATIONAL_B_SPLINE_SURFACE(((1.,0.974927912181824,1.,0.974927912181824,1.,
0.974927912181824,1.,0.974927912181824,1.),(0.987189825241073,0.962438915249418,
0.987189825241073,0.962438915249418,0.987189825241073,0.962438915249418,
0.987189825241073,0.962438915249418,0.987189825241073),(0.987189825241073,
0.962438915249418,0.987189825241073,0.962438915249418,0.987189825241073,
0.962438915249418,0.987189825241073,0.962438915249418,0.987189825241073),
(1.,0.974927912181824,1.,0.974927912181824,1.,0.974927912181824,1.,0.974927912181824,
1.)))
REPRESENTATION_ITEM('')
SURFACE()
);
#428=(
BOUNDED_SURFACE()
B_SPLINE_SURFACE(3,2,((#28373,#28374,#28375,#28376,#28377,#28378,#28379,
#28380,#28381),(#28382,#28383,#28384,#28385,#28386,#28387,#28388,#28389,
#28390),(#28391,#28392,#28393,#28394,#28395,#28396,#28397,#28398,#28399),
(#28400,#28401,#28402,#28403,#28404,#28405,#28406,#28407,#28408)),
 .UNSPECIFIED.,.F.,.F.,.F.)
B_SPLINE_SURFACE_WITH_KNOTS((4,4),(3,2,2,2,3),(0.,1.),(0.,0.25,0.5,0.75,
1.),.UNSPECIFIED.)
GEOMETRIC_REPRESENTATION_ITEM()
RATIONAL_B_SPLINE_SURFACE(((1.,0.974927912181824,1.,0.974927912181824,1.,
0.974927912181824,1.,0.974927912181824,1.),(0.987189825241073,0.962438915249418,
0.987189825241073,0.962438915249418,0.987189825241073,0.962438915249418,
0.987189825241073,0.962438915249418,0.987189825241073),(0.987189825241073,
0.962438915249418,0.987189825241073,0.962438915249418,0.987189825241073,
0.962438915249418,0.987189825241073,0.962438915249418,0.987189825241073),
(1.,0.974927912181824,1.,0.974927912181824,1.,0.974927912181824,1.,0.974927912181824,
1.)))
REPRESENTATION_ITEM('')
SURFACE()
);
#429=(
BOUNDED_SURFACE()
B_SPLINE_SURFACE(3,2,((#28416,#28417,#28418,#28419,#28420,#28421,#28422,
#28423,#28424),(#28425,#28426,#28427,#28428,#28429,#28430,#28431,#28432,
#28433),(#28434,#28435,#28436,#28437,#28438,#28439,#28440,#28441,#28442),
(#28443,#28444,#28445,#28446,#28447,#28448,#28449,#28450,#28451)),
 .UNSPECIFIED.,.F.,.F.,.F.)
B_SPLINE_SURFACE_WITH_KNOTS((4,4),(3,2,2,2,3),(0.,1.),(0.,0.25,0.5,0.75,
1.),.UNSPECIFIED.)
GEOMETRIC_REPRESENTATION_ITEM()
RATIONAL_B_SPLINE_SURFACE(((1.,0.974927912181824,1.,0.974927912181824,1.,
0.974927912181824,1.,0.974927912181824,1.),(0.833333333333332,0.812439926818185,
0.833333333333332,0.812439926818185,0.833333333333332,0.812439926818185,
0.833333333333332,0.812439926818185,0.833333333333332),(0.833333333333332,
0.812439926818185,0.833333333333332,0.812439926818185,0.833333333333332,
0.812439926818185,0.833333333333332,0.812439926818185,0.833333333333332),
(1.,0.974927912181824,1.,0.974927912181824,1.,0.974927912181824,1.,0.974927912181824,
1.)))
REPRESENTATION_ITEM('')
SURFACE()
);
#430=(
BOUNDED_SURFACE()
B_SPLINE_SURFACE(3,2,((#28455,#28456,#28457,#28458,#28459,#28460,#28461,
#28462,#28463),(#28464,#28465,#28466,#28467,#28468,#28469,#28470,#28471,
#28472),(#28473,#28474,#28475,#28476,#28477,#28478,#28479,#28480,#28481),
(#28482,#28483,#28484,#28485,#28486,#28487,#28488,#28489,#28490)),
 .UNSPECIFIED.,.F.,.F.,.F.)
B_SPLINE_SURFACE_WITH_KNOTS((4,4),(3,2,2,2,3),(0.,1.),(0.,0.25,0.5,0.75,
1.),.UNSPECIFIED.)
GEOMETRIC_REPRESENTATION_ITEM()
RATIONAL_B_SPLINE_SURFACE(((1.,0.974927912181824,1.,0.974927912181824,1.,
0.974927912181824,1.,0.974927912181824,1.),(0.987189825241073,0.962438915249418,
0.987189825241073,0.962438915249418,0.987189825241073,0.962438915249418,
0.987189825241073,0.962438915249418,0.987189825241073),(0.987189825241073,
0.962438915249418,0.987189825241073,0.962438915249418,0.987189825241073,
0.962438915249418,0.987189825241073,0.962438915249418,0.987189825241073),
(1.,0.974927912181824,1.,0.974927912181824,1.,0.974927912181824,1.,0.974927912181824,
1.)))
REPRESENTATION_ITEM('')
SURFACE()
);
#431=(
BOUNDED_SURFACE()
B_SPLINE_SURFACE(3,2,((#28498,#28499,#28500,#28501,#28502,#28503,#28504,
#28505,#28506),(#28507,#28508,#28509,#28510,#28511,#28512,#28513,#28514,
#28515),(#28516,#28517,#28518,#28519,#28520,#28521,#28522,#28523,#28524),
(#28525,#28526,#28527,#28528,#28529,#28530,#28531,#28532,#28533)),
 .UNSPECIFIED.,.F.,.F.,.F.)
B_SPLINE_SURFACE_WITH_KNOTS((4,4),(3,2,2,2,3),(0.,1.),(0.,0.25,0.5,0.75,
1.),.UNSPECIFIED.)
GEOMETRIC_REPRESENTATION_ITEM()
RATIONAL_B_SPLINE_SURFACE(((1.,0.974927912181824,1.,0.974927912181824,1.,
0.974927912181824,1.,0.974927912181824,1.),(0.987189825241073,0.962438915249418,
0.987189825241073,0.962438915249418,0.987189825241073,0.962438915249418,
0.987189825241073,0.962438915249418,0.987189825241073),(0.987189825241073,
0.962438915249418,0.987189825241073,0.962438915249418,0.987189825241073,
0.962438915249418,0.987189825241073,0.962438915249418,0.987189825241073),
(1.,0.974927912181824,1.,0.974927912181824,1.,0.974927912181824,1.,0.974927912181824,
1.)))
REPRESENTATION_ITEM('')
SURFACE()
);
#432=(
BOUNDED_SURFACE()
B_SPLINE_SURFACE(3,2,((#28541,#28542,#28543,#28544,#28545,#28546,#28547,
#28548,#28549),(#28550,#28551,#28552,#28553,#28554,#28555,#28556,#28557,
#28558),(#28559,#28560,#28561,#28562,#28563,#28564,#28565,#28566,#28567),
(#28568,#28569,#28570,#28571,#28572,#28573,#28574,#28575,#28576)),
 .UNSPECIFIED.,.F.,.F.,.F.)
B_SPLINE_SURFACE_WITH_KNOTS((4,4),(3,2,2,2,3),(0.,1.),(0.,0.25,0.5,0.75,
1.),.UNSPECIFIED.)
GEOMETRIC_REPRESENTATION_ITEM()
RATIONAL_B_SPLINE_SURFACE(((1.,0.974927912181824,1.,0.974927912181824,1.,
0.974927912181824,1.,0.974927912181824,1.),(0.833333333333332,0.812439926818185,
0.833333333333332,0.812439926818185,0.833333333333332,0.812439926818185,
0.833333333333332,0.812439926818185,0.833333333333332),(0.833333333333332,
0.812439926818185,0.833333333333332,0.812439926818185,0.833333333333332,
0.812439926818185,0.833333333333332,0.812439926818185,0.833333333333332),
(1.,0.974927912181824,1.,0.974927912181824,1.,0.974927912181824,1.,0.974927912181824,
1.)))
REPRESENTATION_ITEM('')
SURFACE()
);
#433=(
BOUNDED_SURFACE()
B_SPLINE_SURFACE(3,2,((#28580,#28581,#28582,#28583,#28584,#28585,#28586,
#28587,#28588),(#28589,#28590,#28591,#28592,#28593,#28594,#28595,#28596,
#28597),(#28598,#28599,#28600,#28601,#28602,#28603,#28604,#28605,#28606),
(#28607,#28608,#28609,#28610,#28611,#28612,#28613,#28614,#28615)),
 .UNSPECIFIED.,.F.,.F.,.F.)
B_SPLINE_SURFACE_WITH_KNOTS((4,4),(3,2,2,2,3),(0.,1.),(0.,0.25,0.5,0.75,
1.),.UNSPECIFIED.)
GEOMETRIC_REPRESENTATION_ITEM()
RATIONAL_B_SPLINE_SURFACE(((1.,0.974927912181824,1.,0.974927912181824,1.,
0.974927912181824,1.,0.974927912181824,1.),(0.987189825241073,0.962438915249418,
0.987189825241073,0.962438915249418,0.987189825241073,0.962438915249418,
0.987189825241073,0.962438915249418,0.987189825241073),(0.987189825241073,
0.962438915249418,0.987189825241073,0.962438915249418,0.987189825241073,
0.962438915249418,0.987189825241073,0.962438915249418,0.987189825241073),
(1.,0.974927912181824,1.,0.974927912181824,1.,0.974927912181824,1.,0.974927912181824,
1.)))
REPRESENTATION_ITEM('')
SURFACE()
);
#434=(
BOUNDED_SURFACE()
B_SPLINE_SURFACE(3,2,((#28623,#28624,#28625,#28626,#28627,#28628,#28629,
#28630,#28631),(#28632,#28633,#28634,#28635,#28636,#28637,#28638,#28639,
#28640),(#28641,#28642,#28643,#28644,#28645,#28646,#28647,#28648,#28649),
(#28650,#28651,#28652,#28653,#28654,#28655,#28656,#28657,#28658)),
 .UNSPECIFIED.,.F.,.F.,.F.)
B_SPLINE_SURFACE_WITH_KNOTS((4,4),(3,2,2,2,3),(0.,1.),(0.,0.25,0.5,0.75,
1.),.UNSPECIFIED.)
GEOMETRIC_REPRESENTATION_ITEM()
RATIONAL_B_SPLINE_SURFACE(((1.,0.974927912181824,1.,0.974927912181824,1.,
0.974927912181824,1.,0.974927912181824,1.),(0.987189825241073,0.962438915249418,
0.987189825241073,0.962438915249418,0.987189825241073,0.962438915249418,
0.987189825241073,0.962438915249418,0.987189825241073),(0.987189825241073,
0.962438915249418,0.987189825241073,0.962438915249418,0.987189825241073,
0.962438915249418,0.987189825241073,0.962438915249418,0.987189825241073),
(1.,0.974927912181824,1.,0.974927912181824,1.,0.974927912181824,1.,0.974927912181824,
1.)))
REPRESENTATION_ITEM('')
SURFACE()
);
#435=(
BOUNDED_SURFACE()
B_SPLINE_SURFACE(3,2,((#28666,#28667,#28668,#28669,#28670,#28671,#28672,
#28673,#28674),(#28675,#28676,#28677,#28678,#28679,#28680,#28681,#28682,
#28683),(#28684,#28685,#28686,#28687,#28688,#28689,#28690,#28691,#28692),
(#28693,#28694,#28695,#28696,#28697,#28698,#28699,#28700,#28701)),
 .UNSPECIFIED.,.F.,.F.,.F.)
B_SPLINE_SURFACE_WITH_KNOTS((4,4),(3,2,2,2,3),(0.,1.),(0.,0.25,0.5,0.75,
1.),.UNSPECIFIED.)
GEOMETRIC_REPRESENTATION_ITEM()
RATIONAL_B_SPLINE_SURFACE(((1.,0.974927912181824,1.,0.974927912181824,1.,
0.974927912181824,1.,0.974927912181824,1.),(0.833333333333333,0.812439926818186,
0.833333333333333,0.812439926818186,0.833333333333333,0.812439926818186,
0.833333333333333,0.812439926818186,0.833333333333333),(0.833333333333333,
0.812439926818186,0.833333333333333,0.812439926818186,0.833333333333333,
0.812439926818186,0.833333333333333,0.812439926818186,0.833333333333333),
(1.,0.974927912181824,1.,0.974927912181824,1.,0.974927912181824,1.,0.974927912181824,
1.)))
REPRESENTATION_ITEM('')
SURFACE()
);
#436=(
BOUNDED_SURFACE()
B_SPLINE_SURFACE(3,2,((#28705,#28706,#28707,#28708,#28709,#28710,#28711,
#28712,#28713),(#28714,#28715,#28716,#28717,#28718,#28719,#28720,#28721,
#28722),(#28723,#28724,#28725,#28726,#28727,#28728,#28729,#28730,#28731),
(#28732,#28733,#28734,#28735,#28736,#28737,#28738,#28739,#28740)),
 .UNSPECIFIED.,.F.,.F.,.F.)
B_SPLINE_SURFACE_WITH_KNOTS((4,4),(3,2,2,2,3),(0.,1.),(0.,0.25,0.5,0.75,
1.),.UNSPECIFIED.)
GEOMETRIC_REPRESENTATION_ITEM()
RATIONAL_B_SPLINE_SURFACE(((1.,0.974927912181824,1.,0.974927912181824,1.,
0.974927912181824,1.,0.974927912181824,1.),(0.987189825241073,0.962438915249418,
0.987189825241073,0.962438915249418,0.987189825241073,0.962438915249418,
0.987189825241073,0.962438915249418,0.987189825241073),(0.987189825241073,
0.962438915249418,0.987189825241073,0.962438915249418,0.987189825241073,
0.962438915249418,0.987189825241073,0.962438915249418,0.987189825241073),
(1.,0.974927912181824,1.,0.974927912181824,1.,0.974927912181824,1.,0.974927912181824,
1.)))
REPRESENTATION_ITEM('')
SURFACE()
);
#437=(
BOUNDED_SURFACE()
B_SPLINE_SURFACE(3,2,((#28795,#28796,#28797,#28798,#28799,#28800,#28801,
#28802,#28803),(#28804,#28805,#28806,#28807,#28808,#28809,#28810,#28811,
#28812),(#28813,#28814,#28815,#28816,#28817,#28818,#28819,#28820,#28821),
(#28822,#28823,#28824,#28825,#28826,#28827,#28828,#28829,#28830)),
 .UNSPECIFIED.,.F.,.F.,.F.)
B_SPLINE_SURFACE_WITH_KNOTS((4,4),(3,2,2,2,3),(0.,1.),(0.,0.25,0.5,0.75,
1.),.UNSPECIFIED.)
GEOMETRIC_REPRESENTATION_ITEM()
RATIONAL_B_SPLINE_SURFACE(((1.,0.974927912181824,1.,0.974927912181824,1.,
0.974927912181824,1.,0.974927912181824,1.),(0.987189825241073,0.962438915249418,
0.987189825241073,0.962438915249418,0.987189825241073,0.962438915249418,
0.987189825241073,0.962438915249418,0.987189825241073),(0.987189825241073,
0.962438915249418,0.987189825241073,0.962438915249418,0.987189825241073,
0.962438915249418,0.987189825241073,0.962438915249418,0.987189825241073),
(1.,0.974927912181824,1.,0.974927912181824,1.,0.974927912181824,1.,0.974927912181824,
1.)))
REPRESENTATION_ITEM('')
SURFACE()
);
#438=(
BOUNDED_SURFACE()
B_SPLINE_SURFACE(3,2,((#28838,#28839,#28840,#28841,#28842,#28843,#28844,
#28845,#28846),(#28847,#28848,#28849,#28850,#28851,#28852,#28853,#28854,
#28855),(#28856,#28857,#28858,#28859,#28860,#28861,#28862,#28863,#28864),
(#28865,#28866,#28867,#28868,#28869,#28870,#28871,#28872,#28873)),
 .UNSPECIFIED.,.F.,.F.,.F.)
B_SPLINE_SURFACE_WITH_KNOTS((4,4),(3,2,2,2,3),(0.,1.),(0.,0.25,0.5,0.75,
1.),.UNSPECIFIED.)
GEOMETRIC_REPRESENTATION_ITEM()
RATIONAL_B_SPLINE_SURFACE(((1.,0.974927912181824,1.,0.974927912181824,1.,
0.974927912181824,1.,0.974927912181824,1.),(0.833333333333332,0.812439926818185,
0.833333333333332,0.812439926818185,0.833333333333332,0.812439926818185,
0.833333333333332,0.812439926818185,0.833333333333332),(0.833333333333332,
0.812439926818185,0.833333333333332,0.812439926818185,0.833333333333332,
0.812439926818185,0.833333333333332,0.812439926818185,0.833333333333332),
(1.,0.974927912181824,1.,0.974927912181824,1.,0.974927912181824,1.,0.974927912181824,
1.)))
REPRESENTATION_ITEM('')
SURFACE()
);
#439=(
BOUNDED_SURFACE()
B_SPLINE_SURFACE(3,2,((#28877,#28878,#28879,#28880,#28881,#28882,#28883,
#28884,#28885),(#28886,#28887,#28888,#28889,#28890,#28891,#28892,#28893,
#28894),(#28895,#28896,#28897,#28898,#28899,#28900,#28901,#28902,#28903),
(#28904,#28905,#28906,#28907,#28908,#28909,#28910,#28911,#28912)),
 .UNSPECIFIED.,.F.,.F.,.F.)
B_SPLINE_SURFACE_WITH_KNOTS((4,4),(3,2,2,2,3),(0.,1.),(0.,0.25,0.5,0.75,
1.),.UNSPECIFIED.)
GEOMETRIC_REPRESENTATION_ITEM()
RATIONAL_B_SPLINE_SURFACE(((1.,0.974927912181824,1.,0.974927912181824,1.,
0.974927912181824,1.,0.974927912181824,1.),(0.987189825241073,0.962438915249418,
0.987189825241073,0.962438915249418,0.987189825241073,0.962438915249418,
0.987189825241073,0.962438915249418,0.987189825241073),(0.987189825241073,
0.962438915249418,0.987189825241073,0.962438915249418,0.987189825241073,
0.962438915249418,0.987189825241073,0.962438915249418,0.987189825241073),
(1.,0.974927912181824,1.,0.974927912181824,1.,0.974927912181824,1.,0.974927912181824,
1.)))
REPRESENTATION_ITEM('')
SURFACE()
);
#440=(
BOUNDED_SURFACE()
B_SPLINE_SURFACE(3,2,((#28967,#28968,#28969,#28970,#28971,#28972,#28973,
#28974,#28975),(#28976,#28977,#28978,#28979,#28980,#28981,#28982,#28983,
#28984),(#28985,#28986,#28987,#28988,#28989,#28990,#28991,#28992,#28993),
(#28994,#28995,#28996,#28997,#28998,#28999,#29000,#29001,#29002)),
 .UNSPECIFIED.,.F.,.F.,.F.)
B_SPLINE_SURFACE_WITH_KNOTS((4,4),(3,2,2,2,3),(0.,1.),(0.,0.25,0.5,0.75,
1.),.UNSPECIFIED.)
GEOMETRIC_REPRESENTATION_ITEM()
RATIONAL_B_SPLINE_SURFACE(((1.,0.974927912181824,1.,0.974927912181824,1.,
0.974927912181824,1.,0.974927912181824,1.),(0.987189825241073,0.962438915249418,
0.987189825241073,0.962438915249418,0.987189825241073,0.962438915249418,
0.987189825241073,0.962438915249418,0.987189825241073),(0.987189825241073,
0.962438915249418,0.987189825241073,0.962438915249418,0.987189825241073,
0.962438915249418,0.987189825241073,0.962438915249418,0.987189825241073),
(1.,0.974927912181824,1.,0.974927912181824,1.,0.974927912181824,1.,0.974927912181824,
1.)))
REPRESENTATION_ITEM('')
SURFACE()
);
#441=(
BOUNDED_SURFACE()
B_SPLINE_SURFACE(3,2,((#29010,#29011,#29012,#29013,#29014,#29015,#29016,
#29017,#29018),(#29019,#29020,#29021,#29022,#29023,#29024,#29025,#29026,
#29027),(#29028,#29029,#29030,#29031,#29032,#29033,#29034,#29035,#29036),
(#29037,#29038,#29039,#29040,#29041,#29042,#29043,#29044,#29045)),
 .UNSPECIFIED.,.F.,.F.,.F.)
B_SPLINE_SURFACE_WITH_KNOTS((4,4),(3,2,2,2,3),(0.,1.),(0.,0.25,0.5,0.75,
1.),.UNSPECIFIED.)
GEOMETRIC_REPRESENTATION_ITEM()
RATIONAL_B_SPLINE_SURFACE(((1.,0.974927912181824,1.,0.974927912181824,1.,
0.974927912181824,1.,0.974927912181824,1.),(0.833333333333331,0.812439926818184,
0.833333333333331,0.812439926818184,0.833333333333331,0.812439926818184,
0.833333333333331,0.812439926818184,0.833333333333331),(0.833333333333331,
0.812439926818184,0.833333333333331,0.812439926818184,0.833333333333331,
0.812439926818184,0.833333333333331,0.812439926818184,0.833333333333331),
(1.,0.974927912181824,1.,0.974927912181824,1.,0.974927912181824,1.,0.974927912181824,
1.)))
REPRESENTATION_ITEM('')
SURFACE()
);
#442=(
BOUNDED_SURFACE()
B_SPLINE_SURFACE(3,2,((#29049,#29050,#29051,#29052,#29053,#29054,#29055,
#29056,#29057),(#29058,#29059,#29060,#29061,#29062,#29063,#29064,#29065,
#29066),(#29067,#29068,#29069,#29070,#29071,#29072,#29073,#29074,#29075),
(#29076,#29077,#29078,#29079,#29080,#29081,#29082,#29083,#29084)),
 .UNSPECIFIED.,.F.,.F.,.F.)
B_SPLINE_SURFACE_WITH_KNOTS((4,4),(3,2,2,2,3),(0.,1.),(0.,0.0714285714285714,
0.142857142857143,0.214285714285714,0.25),.UNSPECIFIED.)
GEOMETRIC_REPRESENTATION_ITEM()
RATIONAL_B_SPLINE_SURFACE(((1.,0.974927912181824,1.,0.974927912181824,1.,
0.974927912181824,1.,0.987463956090912,0.987463956090912),(0.987189825241073,
0.962438915249418,0.987189825241073,0.962438915249418,0.987189825241073,
0.962438915249418,0.987189825241073,0.974814370245245,0.974814370245245),
(0.987189825241073,0.962438915249418,0.987189825241073,0.962438915249418,
0.987189825241073,0.962438915249418,0.987189825241073,0.974814370245245,
0.974814370245245),(1.,0.974927912181824,1.,0.974927912181824,1.,0.974927912181824,
1.,0.987463956090912,0.987463956090912)))
REPRESENTATION_ITEM('')
SURFACE()
);
#443=(
BOUNDED_SURFACE()
B_SPLINE_SURFACE(3,2,((#29092,#29093,#29094,#29095,#29096,#29097,#29098,
#29099,#29100),(#29101,#29102,#29103,#29104,#29105,#29106,#29107,#29108,
#29109),(#29110,#29111,#29112,#29113,#29114,#29115,#29116,#29117,#29118),
(#29119,#29120,#29121,#29122,#29123,#29124,#29125,#29126,#29127)),
 .UNSPECIFIED.,.F.,.F.,.F.)
B_SPLINE_SURFACE_WITH_KNOTS((4,4),(3,2,2,2,3),(0.,1.),(0.,0.0714285714285714,
0.142857142857143,0.214285714285714,0.25),.UNSPECIFIED.)
GEOMETRIC_REPRESENTATION_ITEM()
RATIONAL_B_SPLINE_SURFACE(((1.,0.974927912181824,1.,0.974927912181824,1.,
0.974927912181824,1.,0.987463956090912,0.987463956090912),(0.987189825241073,
0.962438915249418,0.987189825241073,0.962438915249418,0.987189825241073,
0.962438915249418,0.987189825241073,0.974814370245245,0.974814370245245),
(0.987189825241073,0.962438915249418,0.987189825241073,0.962438915249418,
0.987189825241073,0.962438915249418,0.987189825241073,0.974814370245245,
0.974814370245245),(1.,0.974927912181824,1.,0.974927912181824,1.,0.974927912181824,
1.,0.987463956090912,0.987463956090912)))
REPRESENTATION_ITEM('')
SURFACE()
);
#444=(
BOUNDED_SURFACE()
B_SPLINE_SURFACE(3,2,((#29135,#29136,#29137,#29138,#29139,#29140,#29141,
#29142,#29143),(#29144,#29145,#29146,#29147,#29148,#29149,#29150,#29151,
#29152),(#29153,#29154,#29155,#29156,#29157,#29158,#29159,#29160,#29161),
(#29162,#29163,#29164,#29165,#29166,#29167,#29168,#29169,#29170)),
 .UNSPECIFIED.,.F.,.F.,.F.)
B_SPLINE_SURFACE_WITH_KNOTS((4,4),(3,2,2,2,3),(0.,1.),(0.,0.0714285714285714,
0.142857142857143,0.214285714285714,0.25),.UNSPECIFIED.)
GEOMETRIC_REPRESENTATION_ITEM()
RATIONAL_B_SPLINE_SURFACE(((1.,0.974927912181824,1.,0.974927912181824,1.,
0.974927912181824,1.,0.987463956090912,0.987463956090912),(0.833333333333332,
0.812439926818185,0.833333333333332,0.812439926818185,0.833333333333332,
0.812439926818185,0.833333333333332,0.822886630075758,0.822886630075758),
(0.833333333333332,0.812439926818185,0.833333333333332,0.812439926818185,
0.833333333333332,0.812439926818185,0.833333333333332,0.822886630075758,
0.822886630075758),(1.,0.974927912181824,1.,0.974927912181824,1.,0.974927912181824,
1.,0.987463956090912,0.987463956090912)))
REPRESENTATION_ITEM('')
SURFACE()
);
#445=(
BOUNDED_SURFACE()
B_SPLINE_SURFACE(3,2,((#29174,#29175,#29176,#29177,#29178,#29179,#29180,
#29181,#29182),(#29183,#29184,#29185,#29186,#29187,#29188,#29189,#29190,
#29191),(#29192,#29193,#29194,#29195,#29196,#29197,#29198,#29199,#29200),
(#29201,#29202,#29203,#29204,#29205,#29206,#29207,#29208,#29209)),
 .UNSPECIFIED.,.F.,.F.,.F.)
B_SPLINE_SURFACE_WITH_KNOTS((4,4),(3,2,2,2,3),(0.,1.),(0.,0.25,0.5,0.75,
1.),.UNSPECIFIED.)
GEOMETRIC_REPRESENTATION_ITEM()
RATIONAL_B_SPLINE_SURFACE(((1.,0.974927912181824,1.,0.974927912181824,1.,
0.974927912181824,1.,0.974927912181824,1.),(0.987189825241073,0.962438915249418,
0.987189825241073,0.962438915249418,0.987189825241073,0.962438915249418,
0.987189825241073,0.962438915249418,0.987189825241073),(0.987189825241073,
0.962438915249418,0.987189825241073,0.962438915249418,0.987189825241073,
0.962438915249418,0.987189825241073,0.962438915249418,0.987189825241073),
(1.,0.974927912181824,1.,0.974927912181824,1.,0.974927912181824,1.,0.974927912181824,
1.)))
REPRESENTATION_ITEM('')
SURFACE()
);
#446=(
BOUNDED_SURFACE()
B_SPLINE_SURFACE(3,2,((#29264,#29265,#29266,#29267,#29268,#29269,#29270,
#29271,#29272),(#29273,#29274,#29275,#29276,#29277,#29278,#29279,#29280,
#29281),(#29282,#29283,#29284,#29285,#29286,#29287,#29288,#29289,#29290),
(#29291,#29292,#29293,#29294,#29295,#29296,#29297,#29298,#29299)),
 .UNSPECIFIED.,.F.,.F.,.F.)
B_SPLINE_SURFACE_WITH_KNOTS((4,4),(3,2,2,2,3),(0.,1.),(0.,0.25,0.5,0.75,
1.),.UNSPECIFIED.)
GEOMETRIC_REPRESENTATION_ITEM()
RATIONAL_B_SPLINE_SURFACE(((1.,0.974927912181824,1.,0.974927912181824,1.,
0.974927912181824,1.,0.974927912181824,1.),(0.987189825241073,0.962438915249418,
0.987189825241073,0.962438915249418,0.987189825241073,0.962438915249418,
0.987189825241073,0.962438915249418,0.987189825241073),(0.987189825241073,
0.962438915249418,0.987189825241073,0.962438915249418,0.987189825241073,
0.962438915249418,0.987189825241073,0.962438915249418,0.987189825241073),
(1.,0.974927912181824,1.,0.974927912181824,1.,0.974927912181824,1.,0.974927912181824,
1.)))
REPRESENTATION_ITEM('')
SURFACE()
);
#447=(
BOUNDED_SURFACE()
B_SPLINE_SURFACE(3,2,((#29307,#29308,#29309,#29310,#29311,#29312,#29313,
#29314,#29315),(#29316,#29317,#29318,#29319,#29320,#29321,#29322,#29323,
#29324),(#29325,#29326,#29327,#29328,#29329,#29330,#29331,#29332,#29333),
(#29334,#29335,#29336,#29337,#29338,#29339,#29340,#29341,#29342)),
 .UNSPECIFIED.,.F.,.F.,.F.)
B_SPLINE_SURFACE_WITH_KNOTS((4,4),(3,2,2,2,3),(0.,1.),(0.,0.25,0.5,0.75,
1.),.UNSPECIFIED.)
GEOMETRIC_REPRESENTATION_ITEM()
RATIONAL_B_SPLINE_SURFACE(((1.,0.974927912181824,1.,0.974927912181824,1.,
0.974927912181824,1.,0.974927912181824,1.),(0.833333333333333,0.812439926818186,
0.833333333333333,0.812439926818186,0.833333333333333,0.812439926818186,
0.833333333333333,0.812439926818186,0.833333333333333),(0.833333333333333,
0.812439926818186,0.833333333333333,0.812439926818186,0.833333333333333,
0.812439926818186,0.833333333333333,0.812439926818186,0.833333333333333),
(1.,0.974927912181824,1.,0.974927912181824,1.,0.974927912181824,1.,0.974927912181824,
1.)))
REPRESENTATION_ITEM('')
SURFACE()
);
#448=(
BOUNDED_SURFACE()
B_SPLINE_SURFACE(3,2,((#29346,#29347,#29348,#29349,#29350,#29351,#29352,
#29353,#29354),(#29355,#29356,#29357,#29358,#29359,#29360,#29361,#29362,
#29363),(#29364,#29365,#29366,#29367,#29368,#29369,#29370,#29371,#29372),
(#29373,#29374,#29375,#29376,#29377,#29378,#29379,#29380,#29381)),
 .UNSPECIFIED.,.F.,.F.,.F.)
B_SPLINE_SURFACE_WITH_KNOTS((4,4),(3,2,2,2,3),(0.,1.),(0.,0.25,0.5,0.75,
1.),.UNSPECIFIED.)
GEOMETRIC_REPRESENTATION_ITEM()
RATIONAL_B_SPLINE_SURFACE(((1.,0.974927912181824,1.,0.974927912181824,1.,
0.974927912181824,1.,0.974927912181824,1.),(0.987189825241073,0.962438915249418,
0.987189825241073,0.962438915249418,0.987189825241073,0.962438915249418,
0.987189825241073,0.962438915249418,0.987189825241073),(0.987189825241073,
0.962438915249418,0.987189825241073,0.962438915249418,0.987189825241073,
0.962438915249418,0.987189825241073,0.962438915249418,0.987189825241073),
(1.,0.974927912181824,1.,0.974927912181824,1.,0.974927912181824,1.,0.974927912181824,
1.)))
REPRESENTATION_ITEM('')
SURFACE()
);
#449=(
BOUNDED_SURFACE()
B_SPLINE_SURFACE(3,2,((#29436,#29437,#29438,#29439,#29440,#29441,#29442,
#29443,#29444),(#29445,#29446,#29447,#29448,#29449,#29450,#29451,#29452,
#29453),(#29454,#29455,#29456,#29457,#29458,#29459,#29460,#29461,#29462),
(#29463,#29464,#29465,#29466,#29467,#29468,#29469,#29470,#29471)),
 .UNSPECIFIED.,.F.,.F.,.F.)
B_SPLINE_SURFACE_WITH_KNOTS((4,4),(3,2,2,2,3),(0.,1.),(0.,0.25,0.5,0.75,
1.),.UNSPECIFIED.)
GEOMETRIC_REPRESENTATION_ITEM()
RATIONAL_B_SPLINE_SURFACE(((1.,0.974927912181824,1.,0.974927912181824,1.,
0.974927912181824,1.,0.974927912181824,1.),(0.987189825241073,0.962438915249418,
0.987189825241073,0.962438915249418,0.987189825241073,0.962438915249418,
0.987189825241073,0.962438915249418,0.987189825241073),(0.987189825241073,
0.962438915249418,0.987189825241073,0.962438915249418,0.987189825241073,
0.962438915249418,0.987189825241073,0.962438915249418,0.987189825241073),
(1.,0.974927912181824,1.,0.974927912181824,1.,0.974927912181824,1.,0.974927912181824,
1.)))
REPRESENTATION_ITEM('')
SURFACE()
);
#450=(
BOUNDED_SURFACE()
B_SPLINE_SURFACE(3,2,((#29479,#29480,#29481,#29482,#29483,#29484,#29485,
#29486,#29487),(#29488,#29489,#29490,#29491,#29492,#29493,#29494,#29495,
#29496),(#29497,#29498,#29499,#29500,#29501,#29502,#29503,#29504,#29505),
(#29506,#29507,#29508,#29509,#29510,#29511,#29512,#29513,#29514)),
 .UNSPECIFIED.,.F.,.F.,.F.)
B_SPLINE_SURFACE_WITH_KNOTS((4,4),(3,2,2,2,3),(0.,1.),(0.,0.25,0.5,0.75,
1.),.UNSPECIFIED.)
GEOMETRIC_REPRESENTATION_ITEM()
RATIONAL_B_SPLINE_SURFACE(((1.,0.974927912181824,1.,0.974927912181824,1.,
0.974927912181824,1.,0.974927912181824,1.),(0.833333333333332,0.812439926818185,
0.833333333333332,0.812439926818185,0.833333333333332,0.812439926818185,
0.833333333333332,0.812439926818185,0.833333333333332),(0.833333333333332,
0.812439926818185,0.833333333333332,0.812439926818185,0.833333333333332,
0.812439926818185,0.833333333333332,0.812439926818185,0.833333333333332),
(1.,0.974927912181824,1.,0.974927912181824,1.,0.974927912181824,1.,0.974927912181824,
1.)))
REPRESENTATION_ITEM('')
SURFACE()
);
#451=(
BOUNDED_SURFACE()
B_SPLINE_SURFACE(3,2,((#29518,#29519,#29520,#29521,#29522,#29523,#29524,
#29525,#29526),(#29527,#29528,#29529,#29530,#29531,#29532,#29533,#29534,
#29535),(#29536,#29537,#29538,#29539,#29540,#29541,#29542,#29543,#29544),
(#29545,#29546,#29547,#29548,#29549,#29550,#29551,#29552,#29553)),
 .UNSPECIFIED.,.F.,.F.,.F.)
B_SPLINE_SURFACE_WITH_KNOTS((4,4),(3,2,2,2,3),(0.,1.),(0.,0.25,0.5,0.75,
1.),.UNSPECIFIED.)
GEOMETRIC_REPRESENTATION_ITEM()
RATIONAL_B_SPLINE_SURFACE(((1.,0.974927912181824,1.,0.974927912181824,1.,
0.974927912181824,1.,0.974927912181824,1.),(0.987189825241073,0.962438915249418,
0.987189825241073,0.962438915249418,0.987189825241073,0.962438915249418,
0.987189825241073,0.962438915249418,0.987189825241073),(0.987189825241073,
0.962438915249418,0.987189825241073,0.962438915249418,0.987189825241073,
0.962438915249418,0.987189825241073,0.962438915249418,0.987189825241073),
(1.,0.974927912181824,1.,0.974927912181824,1.,0.974927912181824,1.,0.974927912181824,
1.)))
REPRESENTATION_ITEM('')
SURFACE()
);
#452=(
BOUNDED_SURFACE()
B_SPLINE_SURFACE(3,2,((#29608,#29609,#29610,#29611,#29612,#29613,#29614,
#29615,#29616),(#29617,#29618,#29619,#29620,#29621,#29622,#29623,#29624,
#29625),(#29626,#29627,#29628,#29629,#29630,#29631,#29632,#29633,#29634),
(#29635,#29636,#29637,#29638,#29639,#29640,#29641,#29642,#29643)),
 .UNSPECIFIED.,.F.,.F.,.F.)
B_SPLINE_SURFACE_WITH_KNOTS((4,4),(3,2,2,2,3),(0.,1.),(0.,0.25,0.5,0.75,
1.),.UNSPECIFIED.)
GEOMETRIC_REPRESENTATION_ITEM()
RATIONAL_B_SPLINE_SURFACE(((1.,0.974927912181824,1.,0.974927912181824,1.,
0.974927912181824,1.,0.974927912181824,1.),(0.987189825241073,0.962438915249418,
0.987189825241073,0.962438915249418,0.987189825241073,0.962438915249418,
0.987189825241073,0.962438915249418,0.987189825241073),(0.987189825241073,
0.962438915249418,0.987189825241073,0.962438915249418,0.987189825241073,
0.962438915249418,0.987189825241073,0.962438915249418,0.987189825241073),
(1.,0.974927912181824,1.,0.974927912181824,1.,0.974927912181824,1.,0.974927912181824,
1.)))
REPRESENTATION_ITEM('')
SURFACE()
);
#453=(
BOUNDED_SURFACE()
B_SPLINE_SURFACE(3,2,((#29651,#29652,#29653,#29654,#29655,#29656,#29657,
#29658,#29659),(#29660,#29661,#29662,#29663,#29664,#29665,#29666,#29667,
#29668),(#29669,#29670,#29671,#29672,#29673,#29674,#29675,#29676,#29677),
(#29678,#29679,#29680,#29681,#29682,#29683,#29684,#29685,#29686)),
 .UNSPECIFIED.,.F.,.F.,.F.)
B_SPLINE_SURFACE_WITH_KNOTS((4,4),(3,2,2,2,3),(0.,1.),(0.,0.25,0.5,0.75,
1.),.UNSPECIFIED.)
GEOMETRIC_REPRESENTATION_ITEM()
RATIONAL_B_SPLINE_SURFACE(((1.,0.974927912181824,1.,0.974927912181824,1.,
0.974927912181824,1.,0.974927912181824,1.),(0.833333333333332,0.812439926818185,
0.833333333333332,0.812439926818185,0.833333333333332,0.812439926818185,
0.833333333333332,0.812439926818185,0.833333333333332),(0.833333333333332,
0.812439926818185,0.833333333333332,0.812439926818185,0.833333333333332,
0.812439926818185,0.833333333333332,0.812439926818185,0.833333333333332),
(1.,0.974927912181824,1.,0.974927912181824,1.,0.974927912181824,1.,0.974927912181824,
1.)))
REPRESENTATION_ITEM('')
SURFACE()
);
#454=(
BOUNDED_SURFACE()
B_SPLINE_SURFACE(3,2,((#29690,#29691,#29692,#29693,#29694,#29695,#29696,
#29697,#29698),(#29699,#29700,#29701,#29702,#29703,#29704,#29705,#29706,
#29707),(#29708,#29709,#29710,#29711,#29712,#29713,#29714,#29715,#29716),
(#29717,#29718,#29719,#29720,#29721,#29722,#29723,#29724,#29725)),
 .UNSPECIFIED.,.F.,.F.,.F.)
B_SPLINE_SURFACE_WITH_KNOTS((4,4),(3,2,2,2,3),(0.,1.),(0.,0.25,0.5,0.75,
1.),.UNSPECIFIED.)
GEOMETRIC_REPRESENTATION_ITEM()
RATIONAL_B_SPLINE_SURFACE(((1.,0.974927912181824,1.,0.974927912181824,1.,
0.974927912181824,1.,0.974927912181824,1.),(0.987189825241073,0.962438915249418,
0.987189825241073,0.962438915249418,0.987189825241073,0.962438915249418,
0.987189825241073,0.962438915249418,0.987189825241073),(0.987189825241073,
0.962438915249418,0.987189825241073,0.962438915249418,0.987189825241073,
0.962438915249418,0.987189825241073,0.962438915249418,0.987189825241073),
(1.,0.974927912181824,1.,0.974927912181824,1.,0.974927912181824,1.,0.974927912181824,
1.)))
REPRESENTATION_ITEM('')
SURFACE()
);
#455=(
BOUNDED_SURFACE()
B_SPLINE_SURFACE(3,2,((#29780,#29781,#29782,#29783,#29784,#29785,#29786,
#29787,#29788),(#29789,#29790,#29791,#29792,#29793,#29794,#29795,#29796,
#29797),(#29798,#29799,#29800,#29801,#29802,#29803,#29804,#29805,#29806),
(#29807,#29808,#29809,#29810,#29811,#29812,#29813,#29814,#29815)),
 .UNSPECIFIED.,.F.,.F.,.F.)
B_SPLINE_SURFACE_WITH_KNOTS((4,4),(3,2,2,2,3),(0.,1.),(0.,0.25,0.5,0.75,
1.),.UNSPECIFIED.)
GEOMETRIC_REPRESENTATION_ITEM()
RATIONAL_B_SPLINE_SURFACE(((1.,0.974927912181824,1.,0.974927912181824,1.,
0.974927912181824,1.,0.974927912181824,1.),(0.987189825241073,0.962438915249418,
0.987189825241073,0.962438915249418,0.987189825241073,0.962438915249418,
0.987189825241073,0.962438915249418,0.987189825241073),(0.987189825241073,
0.962438915249418,0.987189825241073,0.962438915249418,0.987189825241073,
0.962438915249418,0.987189825241073,0.962438915249418,0.987189825241073),
(1.,0.974927912181824,1.,0.974927912181824,1.,0.974927912181824,1.,0.974927912181824,
1.)))
REPRESENTATION_ITEM('')
SURFACE()
);
#456=(
BOUNDED_SURFACE()
B_SPLINE_SURFACE(3,2,((#29823,#29824,#29825,#29826,#29827,#29828,#29829,
#29830,#29831),(#29832,#29833,#29834,#29835,#29836,#29837,#29838,#29839,
#29840),(#29841,#29842,#29843,#29844,#29845,#29846,#29847,#29848,#29849),
(#29850,#29851,#29852,#29853,#29854,#29855,#29856,#29857,#29858)),
 .UNSPECIFIED.,.F.,.F.,.F.)
B_SPLINE_SURFACE_WITH_KNOTS((4,4),(3,2,2,2,3),(0.,1.),(0.,0.25,0.5,0.75,
1.),.UNSPECIFIED.)
GEOMETRIC_REPRESENTATION_ITEM()
RATIONAL_B_SPLINE_SURFACE(((1.,0.974927912181824,1.,0.974927912181824,1.,
0.974927912181824,1.,0.974927912181824,1.),(0.833333333333332,0.812439926818185,
0.833333333333332,0.812439926818185,0.833333333333332,0.812439926818185,
0.833333333333332,0.812439926818185,0.833333333333332),(0.833333333333332,
0.812439926818185,0.833333333333332,0.812439926818185,0.833333333333332,
0.812439926818185,0.833333333333332,0.812439926818185,0.833333333333332),
(1.,0.974927912181824,1.,0.974927912181824,1.,0.974927912181824,1.,0.974927912181824,
1.)))
REPRESENTATION_ITEM('')
SURFACE()
);
#457=(
BOUNDED_SURFACE()
B_SPLINE_SURFACE(3,2,((#29862,#29863,#29864,#29865,#29866,#29867,#29868,
#29869,#29870),(#29871,#29872,#29873,#29874,#29875,#29876,#29877,#29878,
#29879),(#29880,#29881,#29882,#29883,#29884,#29885,#29886,#29887,#29888),
(#29889,#29890,#29891,#29892,#29893,#29894,#29895,#29896,#29897)),
 .UNSPECIFIED.,.F.,.F.,.F.)
B_SPLINE_SURFACE_WITH_KNOTS((4,4),(3,2,2,2,3),(0.,1.),(0.,0.25,0.5,0.75,
1.),.UNSPECIFIED.)
GEOMETRIC_REPRESENTATION_ITEM()
RATIONAL_B_SPLINE_SURFACE(((1.,0.974927912181824,1.,0.974927912181824,1.,
0.974927912181824,1.,0.974927912181824,1.),(0.987189825241073,0.962438915249418,
0.987189825241073,0.962438915249418,0.987189825241073,0.962438915249418,
0.987189825241073,0.962438915249418,0.987189825241073),(0.987189825241073,
0.962438915249418,0.987189825241073,0.962438915249418,0.987189825241073,
0.962438915249418,0.987189825241073,0.962438915249418,0.987189825241073),
(1.,0.974927912181824,1.,0.974927912181824,1.,0.974927912181824,1.,0.974927912181824,
1.)))
REPRESENTATION_ITEM('')
SURFACE()
);
#458=(
BOUNDED_SURFACE()
B_SPLINE_SURFACE(3,2,((#29952,#29953,#29954,#29955,#29956,#29957,#29958,
#29959,#29960),(#29961,#29962,#29963,#29964,#29965,#29966,#29967,#29968,
#29969),(#29970,#29971,#29972,#29973,#29974,#29975,#29976,#29977,#29978),
(#29979,#29980,#29981,#29982,#29983,#29984,#29985,#29986,#29987)),
 .UNSPECIFIED.,.F.,.F.,.F.)
B_SPLINE_SURFACE_WITH_KNOTS((4,4),(3,2,2,2,3),(0.,1.),(0.,0.25,0.5,0.75,
1.),.UNSPECIFIED.)
GEOMETRIC_REPRESENTATION_ITEM()
RATIONAL_B_SPLINE_SURFACE(((1.,0.974927912181824,1.,0.974927912181824,1.,
0.974927912181824,1.,0.974927912181824,1.),(0.987189825241073,0.962438915249418,
0.987189825241073,0.962438915249418,0.987189825241073,0.962438915249418,
0.987189825241073,0.962438915249418,0.987189825241073),(0.987189825241073,
0.962438915249418,0.987189825241073,0.962438915249418,0.987189825241073,
0.962438915249418,0.987189825241073,0.962438915249418,0.987189825241073),
(1.,0.974927912181824,1.,0.974927912181824,1.,0.974927912181824,1.,0.974927912181824,
1.)))
REPRESENTATION_ITEM('')
SURFACE()
);
#459=(
BOUNDED_SURFACE()
B_SPLINE_SURFACE(3,2,((#29995,#29996,#29997,#29998,#29999,#30000,#30001,
#30002,#30003),(#30004,#30005,#30006,#30007,#30008,#30009,#30010,#30011,
#30012),(#30013,#30014,#30015,#30016,#30017,#30018,#30019,#30020,#30021),
(#30022,#30023,#30024,#30025,#30026,#30027,#30028,#30029,#30030)),
 .UNSPECIFIED.,.F.,.F.,.F.)
B_SPLINE_SURFACE_WITH_KNOTS((4,4),(3,2,2,2,3),(0.,1.),(0.,0.25,0.5,0.75,
1.),.UNSPECIFIED.)
GEOMETRIC_REPRESENTATION_ITEM()
RATIONAL_B_SPLINE_SURFACE(((1.,0.974927912181824,1.,0.974927912181824,1.,
0.974927912181824,1.,0.974927912181824,1.),(0.833333333333333,0.812439926818186,
0.833333333333333,0.812439926818186,0.833333333333333,0.812439926818186,
0.833333333333333,0.812439926818186,0.833333333333333),(0.833333333333333,
0.812439926818186,0.833333333333333,0.812439926818186,0.833333333333333,
0.812439926818186,0.833333333333333,0.812439926818186,0.833333333333333),
(1.,0.974927912181824,1.,0.974927912181824,1.,0.974927912181824,1.,0.974927912181824,
1.)))
REPRESENTATION_ITEM('')
SURFACE()
);
#460=(
BOUNDED_SURFACE()
B_SPLINE_SURFACE(3,2,((#30034,#30035,#30036,#30037,#30038,#30039,#30040,
#30041,#30042),(#30043,#30044,#30045,#30046,#30047,#30048,#30049,#30050,
#30051),(#30052,#30053,#30054,#30055,#30056,#30057,#30058,#30059,#30060),
(#30061,#30062,#30063,#30064,#30065,#30066,#30067,#30068,#30069)),
 .UNSPECIFIED.,.F.,.F.,.F.)
B_SPLINE_SURFACE_WITH_KNOTS((4,4),(3,2,2,2,3),(0.,1.),(0.,0.25,0.5,0.75,
1.),.UNSPECIFIED.)
GEOMETRIC_REPRESENTATION_ITEM()
RATIONAL_B_SPLINE_SURFACE(((1.,0.974927912181824,1.,0.974927912181824,1.,
0.974927912181824,1.,0.974927912181824,1.),(0.987189825241073,0.962438915249418,
0.987189825241073,0.962438915249418,0.987189825241073,0.962438915249418,
0.987189825241073,0.962438915249418,0.987189825241073),(0.987189825241073,
0.962438915249418,0.987189825241073,0.962438915249418,0.987189825241073,
0.962438915249418,0.987189825241073,0.962438915249418,0.987189825241073),
(1.,0.974927912181824,1.,0.974927912181824,1.,0.974927912181824,1.,0.974927912181824,
1.)))
REPRESENTATION_ITEM('')
SURFACE()
);
#461=(
BOUNDED_SURFACE()
B_SPLINE_SURFACE(3,2,((#30077,#30078,#30079,#30080,#30081,#30082,#30083,
#30084,#30085),(#30086,#30087,#30088,#30089,#30090,#30091,#30092,#30093,
#30094),(#30095,#30096,#30097,#30098,#30099,#30100,#30101,#30102,#30103),
(#30104,#30105,#30106,#30107,#30108,#30109,#30110,#30111,#30112)),
 .UNSPECIFIED.,.F.,.F.,.F.)
B_SPLINE_SURFACE_WITH_KNOTS((4,4),(3,2,2,2,3),(0.,1.),(0.,0.25,0.5,0.75,
1.),.UNSPECIFIED.)
GEOMETRIC_REPRESENTATION_ITEM()
RATIONAL_B_SPLINE_SURFACE(((1.,0.974927912181824,1.,0.974927912181824,1.,
0.974927912181824,1.,0.974927912181824,1.),(0.987189825241073,0.962438915249418,
0.987189825241073,0.962438915249418,0.987189825241073,0.962438915249418,
0.987189825241073,0.962438915249418,0.987189825241073),(0.987189825241073,
0.962438915249418,0.987189825241073,0.962438915249418,0.987189825241073,
0.962438915249418,0.987189825241073,0.962438915249418,0.987189825241073),
(1.,0.974927912181824,1.,0.974927912181824,1.,0.974927912181824,1.,0.974927912181824,
1.)))
REPRESENTATION_ITEM('')
SURFACE()
);
#462=(
BOUNDED_SURFACE()
B_SPLINE_SURFACE(3,2,((#30120,#30121,#30122,#30123,#30124,#30125,#30126,
#30127,#30128),(#30129,#30130,#30131,#30132,#30133,#30134,#30135,#30136,
#30137),(#30138,#30139,#30140,#30141,#30142,#30143,#30144,#30145,#30146),
(#30147,#30148,#30149,#30150,#30151,#30152,#30153,#30154,#30155)),
 .UNSPECIFIED.,.F.,.F.,.F.)
B_SPLINE_SURFACE_WITH_KNOTS((4,4),(3,2,2,2,3),(0.,1.),(0.,0.25,0.5,0.75,
1.),.UNSPECIFIED.)
GEOMETRIC_REPRESENTATION_ITEM()
RATIONAL_B_SPLINE_SURFACE(((1.,0.974927912181824,1.,0.974927912181824,1.,
0.974927912181824,1.,0.974927912181824,1.),(0.833333333333332,0.812439926818185,
0.833333333333332,0.812439926818185,0.833333333333332,0.812439926818185,
0.833333333333332,0.812439926818185,0.833333333333332),(0.833333333333332,
0.812439926818185,0.833333333333332,0.812439926818185,0.833333333333332,
0.812439926818185,0.833333333333332,0.812439926818185,0.833333333333332),
(1.,0.974927912181824,1.,0.974927912181824,1.,0.974927912181824,1.,0.974927912181824,
1.)))
REPRESENTATION_ITEM('')
SURFACE()
);
#463=(
BOUNDED_SURFACE()
B_SPLINE_SURFACE(3,3,((#30159,#30160,#30161,#30162,#30163,#30164,#30165,
#30166,#30167,#30168,#30169,#30170),(#30171,#30172,#30173,#30174,#30175,
#30176,#30177,#30178,#30179,#30180,#30181,#30182),(#30183,#30184,#30185,
#30186,#30187,#30188,#30189,#30190,#30191,#30192,#30193,#30194),(#30195,
#30196,#30197,#30198,#30199,#30200,#30201,#30202,#30203,#30204,#30205,#30206)),
 .UNSPECIFIED.,.F.,.F.,.F.)
B_SPLINE_SURFACE_WITH_KNOTS((4,4),(4,2,2,2,2,4),(0.,1.),(0.,0.0783698352504338,
0.308777376437326,0.539184917624882,0.769592458812441,1.),.UNSPECIFIED.)
GEOMETRIC_REPRESENTATION_ITEM()
RATIONAL_B_SPLINE_SURFACE(((1.,1.,1.,1.,1.,1.,1.,1.,1.,1.,1.,1.),(0.833333333333332,
0.833333333333332,0.833333333333332,0.833333333333332,0.833333333333332,
0.833333333333332,0.833333333333332,0.833333333333332,0.833333333333332,
0.833333333333332,0.833333333333332,0.833333333333332),(0.833333333333332,
0.833333333333332,0.833333333333332,0.833333333333332,0.833333333333332,
0.833333333333332,0.833333333333332,0.833333333333332,0.833333333333332,
0.833333333333332,0.833333333333332,0.833333333333332),(1.,1.,1.,1.,1.,
1.,1.,1.,1.,1.,1.,1.)))
REPRESENTATION_ITEM('')
SURFACE()
);
#464=(
BOUNDED_SURFACE()
B_SPLINE_SURFACE(3,3,((#30223,#30224,#30225,#30226,#30227,#30228,#30229,
#30230,#30231,#30232,#30233,#30234),(#30235,#30236,#30237,#30238,#30239,
#30240,#30241,#30242,#30243,#30244,#30245,#30246),(#30247,#30248,#30249,
#30250,#30251,#30252,#30253,#30254,#30255,#30256,#30257,#30258),(#30259,
#30260,#30261,#30262,#30263,#30264,#30265,#30266,#30267,#30268,#30269,#30270)),
 .UNSPECIFIED.,.F.,.F.,.F.)
B_SPLINE_SURFACE_WITH_KNOTS((4,4),(4,2,2,2,2,4),(0.,1.),(0.,0.0783698352504338,
0.308777376437326,0.539184917624882,0.769592458812441,1.),.UNSPECIFIED.)
GEOMETRIC_REPRESENTATION_ITEM()
RATIONAL_B_SPLINE_SURFACE(((1.,1.,1.,1.,1.,1.,1.,1.,1.,1.,1.,1.),(0.987189825241073,
0.987189825241073,0.987189825241073,0.987189825241073,0.987189825241073,
0.987189825241073,0.987189825241073,0.987189825241073,0.987189825241073,
0.987189825241073,0.987189825241073,0.987189825241073),(0.987189825241073,
0.987189825241073,0.987189825241073,0.987189825241073,0.987189825241073,
0.987189825241073,0.987189825241073,0.987189825241073,0.987189825241073,
0.987189825241073,0.987189825241073,0.987189825241073),(1.,1.,1.,1.,1.,
1.,1.,1.,1.,1.,1.,1.)))
REPRESENTATION_ITEM('')
SURFACE()
);
#465=(
BOUNDED_SURFACE()
B_SPLINE_SURFACE(3,3,((#30271,#30272,#30273,#30274,#30275,#30276,#30277,
#30278,#30279,#30280,#30281,#30282),(#30283,#30284,#30285,#30286,#30287,
#30288,#30289,#30290,#30291,#30292,#30293,#30294),(#30295,#30296,#30297,
#30298,#30299,#30300,#30301,#30302,#30303,#30304,#30305,#30306),(#30307,
#30308,#30309,#30310,#30311,#30312,#30313,#30314,#30315,#30316,#30317,#30318)),
 .UNSPECIFIED.,.F.,.F.,.F.)
B_SPLINE_SURFACE_WITH_KNOTS((4,4),(4,2,2,2,2,4),(0.,1.),(0.,0.0783698352504338,
0.308777376437326,0.539184917624882,0.769592458812441,1.),.UNSPECIFIED.)
GEOMETRIC_REPRESENTATION_ITEM()
RATIONAL_B_SPLINE_SURFACE(((1.,1.,1.,1.,1.,1.,1.,1.,1.,1.,1.,1.),(0.987189825241073,
0.987189825241073,0.987189825241073,0.987189825241073,0.987189825241073,
0.987189825241073,0.987189825241073,0.987189825241073,0.987189825241073,
0.987189825241073,0.987189825241073,0.987189825241073),(0.987189825241073,
0.987189825241073,0.987189825241073,0.987189825241073,0.987189825241073,
0.987189825241073,0.987189825241073,0.987189825241073,0.987189825241073,
0.987189825241073,0.987189825241073,0.987189825241073),(1.,1.,1.,1.,1.,
1.,1.,1.,1.,1.,1.,1.)))
REPRESENTATION_ITEM('')
SURFACE()
);
#466=(
BOUNDED_SURFACE()
B_SPLINE_SURFACE(3,3,((#30319,#30320,#30321,#30322,#30323,#30324,#30325,
#30326,#30327,#30328,#30329,#30330),(#30331,#30332,#30333,#30334,#30335,
#30336,#30337,#30338,#30339,#30340,#30341,#30342),(#30343,#30344,#30345,
#30346,#30347,#30348,#30349,#30350,#30351,#30352,#30353,#30354),(#30355,
#30356,#30357,#30358,#30359,#30360,#30361,#30362,#30363,#30364,#30365,#30366)),
 .UNSPECIFIED.,.F.,.F.,.F.)
B_SPLINE_SURFACE_WITH_KNOTS((4,4),(4,2,2,2,2,4),(0.,1.),(0.,0.0783698388401176,
0.308777379129589,0.539184919419725,0.769592459709862,1.),.UNSPECIFIED.)
GEOMETRIC_REPRESENTATION_ITEM()
RATIONAL_B_SPLINE_SURFACE(((1.,1.,1.,1.,1.,1.,1.,1.,1.,1.,1.,1.),(0.833333333333333,
0.833333333333333,0.833333333333333,0.833333333333333,0.833333333333333,
0.833333333333333,0.833333333333333,0.833333333333333,0.833333333333333,
0.833333333333333,0.833333333333333,0.833333333333333),(0.833333333333333,
0.833333333333333,0.833333333333333,0.833333333333333,0.833333333333333,
0.833333333333333,0.833333333333333,0.833333333333333,0.833333333333333,
0.833333333333333,0.833333333333333,0.833333333333333),(1.,1.,1.,1.,1.,
1.,1.,1.,1.,1.,1.,1.)))
REPRESENTATION_ITEM('')
SURFACE()
);
#467=(
BOUNDED_SURFACE()
B_SPLINE_SURFACE(3,3,((#30383,#30384,#30385,#30386,#30387,#30388,#30389,
#30390,#30391,#30392,#30393,#30394),(#30395,#30396,#30397,#30398,#30399,
#30400,#30401,#30402,#30403,#30404,#30405,#30406),(#30407,#30408,#30409,
#30410,#30411,#30412,#30413,#30414,#30415,#30416,#30417,#30418),(#30419,
#30420,#30421,#30422,#30423,#30424,#30425,#30426,#30427,#30428,#30429,#30430)),
 .UNSPECIFIED.,.F.,.F.,.F.)
B_SPLINE_SURFACE_WITH_KNOTS((4,4),(4,2,2,2,2,4),(0.,1.),(0.,0.0783698388401176,
0.308777379129589,0.539184919419725,0.769592459709862,1.),.UNSPECIFIED.)
GEOMETRIC_REPRESENTATION_ITEM()
RATIONAL_B_SPLINE_SURFACE(((1.,1.,1.,1.,1.,1.,1.,1.,1.,1.,1.,1.),(0.987189825241073,
0.987189825241073,0.987189825241073,0.987189825241073,0.987189825241073,
0.987189825241073,0.987189825241073,0.987189825241073,0.987189825241073,
0.987189825241073,0.987189825241073,0.987189825241073),(0.987189825241073,
0.987189825241073,0.987189825241073,0.987189825241073,0.987189825241073,
0.987189825241073,0.987189825241073,0.987189825241073,0.987189825241073,
0.987189825241073,0.987189825241073,0.987189825241073),(1.,1.,1.,1.,1.,
1.,1.,1.,1.,1.,1.,1.)))
REPRESENTATION_ITEM('')
SURFACE()
);
#468=(
BOUNDED_SURFACE()
B_SPLINE_SURFACE(3,3,((#30431,#30432,#30433,#30434,#30435,#30436,#30437,
#30438,#30439,#30440,#30441,#30442),(#30443,#30444,#30445,#30446,#30447,
#30448,#30449,#30450,#30451,#30452,#30453,#30454),(#30455,#30456,#30457,
#30458,#30459,#30460,#30461,#30462,#30463,#30464,#30465,#30466),(#30467,
#30468,#30469,#30470,#30471,#30472,#30473,#30474,#30475,#30476,#30477,#30478)),
 .UNSPECIFIED.,.F.,.F.,.F.)
B_SPLINE_SURFACE_WITH_KNOTS((4,4),(4,2,2,2,2,4),(0.,1.),(0.,0.0783698388401176,
0.308777379129589,0.539184919419725,0.769592459709862,1.),.UNSPECIFIED.)
GEOMETRIC_REPRESENTATION_ITEM()
RATIONAL_B_SPLINE_SURFACE(((1.,1.,1.,1.,1.,1.,1.,1.,1.,1.,1.,1.),(0.987189825241073,
0.987189825241073,0.987189825241073,0.987189825241073,0.987189825241073,
0.987189825241073,0.987189825241073,0.987189825241073,0.987189825241073,
0.987189825241073,0.987189825241073,0.987189825241073),(0.987189825241073,
0.987189825241073,0.987189825241073,0.987189825241073,0.987189825241073,
0.987189825241073,0.987189825241073,0.987189825241073,0.987189825241073,
0.987189825241073,0.987189825241073,0.987189825241073),(1.,1.,1.,1.,1.,
1.,1.,1.,1.,1.,1.,1.)))
REPRESENTATION_ITEM('')
SURFACE()
);
#469=(
BOUNDED_SURFACE()
B_SPLINE_SURFACE(3,3,((#30479,#30480,#30481,#30482,#30483,#30484,#30485,
#30486,#30487,#30488,#30489,#30490,#30491,#30492),(#30493,#30494,#30495,
#30496,#30497,#30498,#30499,#30500,#30501,#30502,#30503,#30504,#30505,#30506),
(#30507,#30508,#30509,#30510,#30511,#30512,#30513,#30514,#30515,#30516,
#30517,#30518,#30519,#30520),(#30521,#30522,#30523,#30524,#30525,#30526,
#30527,#30528,#30529,#30530,#30531,#30532,#30533,#30534)),.UNSPECIFIED.,
 .F.,.F.,.F.)
B_SPLINE_SURFACE_WITH_KNOTS((4,4),(4,2,2,2,2,2,4),(0.,1.),(0.,0.0183879322611553,
0.0783698437311047,0.308777382797829,0.539184921865218,0.769592460932609,
1.),.UNSPECIFIED.)
GEOMETRIC_REPRESENTATION_ITEM()
RATIONAL_B_SPLINE_SURFACE(((1.,1.,1.,1.,1.,1.,1.,1.,1.,1.,1.,1.,1.,1.),
(0.833333333333331,0.833333333333331,0.833333333333331,0.833333333333331,
0.833333333333331,0.833333333333331,0.833333333333331,0.833333333333331,
0.833333333333331,0.833333333333331,0.833333333333331,0.833333333333331,
0.833333333333331,0.833333333333331),(0.833333333333331,0.833333333333331,
0.833333333333331,0.833333333333331,0.833333333333331,0.833333333333331,
0.833333333333331,0.833333333333331,0.833333333333331,0.833333333333331,
0.833333333333331,0.833333333333331,0.833333333333331,0.833333333333331),
(1.,1.,1.,1.,1.,1.,1.,1.,1.,1.,1.,1.,1.,1.)))
REPRESENTATION_ITEM('')
SURFACE()
);
#470=(
BOUNDED_SURFACE()
B_SPLINE_SURFACE(3,3,((#30553,#30554,#30555,#30556,#30557,#30558,#30559,
#30560,#30561,#30562,#30563,#30564,#30565,#30566),(#30567,#30568,#30569,
#30570,#30571,#30572,#30573,#30574,#30575,#30576,#30577,#30578,#30579,#30580),
(#30581,#30582,#30583,#30584,#30585,#30586,#30587,#30588,#30589,#30590,
#30591,#30592,#30593,#30594),(#30595,#30596,#30597,#30598,#30599,#30600,
#30601,#30602,#30603,#30604,#30605,#30606,#30607,#30608)),.UNSPECIFIED.,
 .F.,.F.,.F.)
B_SPLINE_SURFACE_WITH_KNOTS((4,4),(4,2,2,2,2,2,4),(0.,1.),(0.,0.0183879322611553,
0.0783698437311047,0.308777382797829,0.539184921865218,0.769592460932609,
1.),.UNSPECIFIED.)
GEOMETRIC_REPRESENTATION_ITEM()
RATIONAL_B_SPLINE_SURFACE(((1.,1.,1.,1.,1.,1.,1.,1.,1.,1.,1.,1.,1.,1.),
(0.987189825241073,0.987189825241073,0.987189825241073,0.987189825241073,
0.987189825241073,0.987189825241073,0.987189825241073,0.987189825241073,
0.987189825241073,0.987189825241073,0.987189825241073,0.987189825241073,
0.987189825241073,0.987189825241073),(0.987189825241073,0.987189825241073,
0.987189825241073,0.987189825241073,0.987189825241073,0.987189825241073,
0.987189825241073,0.987189825241073,0.987189825241073,0.987189825241073,
0.987189825241073,0.987189825241073,0.987189825241073,0.987189825241073),
(1.,1.,1.,1.,1.,1.,1.,1.,1.,1.,1.,1.,1.,1.)))
REPRESENTATION_ITEM('')
SURFACE()
);
#471=(
BOUNDED_SURFACE()
B_SPLINE_SURFACE(3,3,((#30609,#30610,#30611,#30612,#30613,#30614,#30615,
#30616,#30617,#30618,#30619,#30620,#30621,#30622),(#30623,#30624,#30625,
#30626,#30627,#30628,#30629,#30630,#30631,#30632,#30633,#30634,#30635,#30636),
(#30637,#30638,#30639,#30640,#30641,#30642,#30643,#30644,#30645,#30646,
#30647,#30648,#30649,#30650),(#30651,#30652,#30653,#30654,#30655,#30656,
#30657,#30658,#30659,#30660,#30661,#30662,#30663,#30664)),.UNSPECIFIED.,
 .F.,.F.,.F.)
B_SPLINE_SURFACE_WITH_KNOTS((4,4),(4,2,2,2,2,2,4),(0.,1.),(0.,0.0183879322611553,
0.0783698437311047,0.308777382797829,0.539184921865218,0.769592460932609,
1.),.UNSPECIFIED.)
GEOMETRIC_REPRESENTATION_ITEM()
RATIONAL_B_SPLINE_SURFACE(((1.,1.,1.,1.,1.,1.,1.,1.,1.,1.,1.,1.,1.,1.),
(0.987189825241073,0.987189825241073,0.987189825241073,0.987189825241073,
0.987189825241073,0.987189825241073,0.987189825241073,0.987189825241073,
0.987189825241073,0.987189825241073,0.987189825241073,0.987189825241073,
0.987189825241073,0.987189825241073),(0.987189825241073,0.987189825241073,
0.987189825241073,0.987189825241073,0.987189825241073,0.987189825241073,
0.987189825241073,0.987189825241073,0.987189825241073,0.987189825241073,
0.987189825241073,0.987189825241073,0.987189825241073,0.987189825241073),
(1.,1.,1.,1.,1.,1.,1.,1.,1.,1.,1.,1.,1.,1.)))
REPRESENTATION_ITEM('')
SURFACE()
);
#472=(
BOUNDED_SURFACE()
B_SPLINE_SURFACE(3,3,((#30665,#30666,#30667,#30668,#30669,#30670,#30671,
#30672,#30673,#30674,#30675,#30676),(#30677,#30678,#30679,#30680,#30681,
#30682,#30683,#30684,#30685,#30686,#30687,#30688),(#30689,#30690,#30691,
#30692,#30693,#30694,#30695,#30696,#30697,#30698,#30699,#30700),(#30701,
#30702,#30703,#30704,#30705,#30706,#30707,#30708,#30709,#30710,#30711,#30712)),
 .UNSPECIFIED.,.F.,.F.,.F.)
B_SPLINE_SURFACE_WITH_KNOTS((4,4),(4,2,2,2,2,4),(0.,1.),(0.,0.0783698481609191,
0.30877738612019,0.539184924080125,0.769592462040062,1.),.UNSPECIFIED.)
GEOMETRIC_REPRESENTATION_ITEM()
RATIONAL_B_SPLINE_SURFACE(((1.,1.,1.,1.,1.,1.,1.,1.,1.,1.,1.,1.),(0.833333333333333,
0.833333333333333,0.833333333333333,0.833333333333333,0.833333333333333,
0.833333333333333,0.833333333333333,0.833333333333333,0.833333333333333,
0.833333333333333,0.833333333333333,0.833333333333333),(0.833333333333333,
0.833333333333333,0.833333333333333,0.833333333333333,0.833333333333333,
0.833333333333333,0.833333333333333,0.833333333333333,0.833333333333333,
0.833333333333333,0.833333333333333,0.833333333333333),(1.,1.,1.,1.,1.,
1.,1.,1.,1.,1.,1.,1.)))
REPRESENTATION_ITEM('')
SURFACE()
);
#473=(
BOUNDED_SURFACE()
B_SPLINE_SURFACE(3,3,((#30729,#30730,#30731,#30732,#30733,#30734,#30735,
#30736,#30737,#30738,#30739,#30740),(#30741,#30742,#30743,#30744,#30745,
#30746,#30747,#30748,#30749,#30750,#30751,#30752),(#30753,#30754,#30755,
#30756,#30757,#30758,#30759,#30760,#30761,#30762,#30763,#30764),(#30765,
#30766,#30767,#30768,#30769,#30770,#30771,#30772,#30773,#30774,#30775,#30776)),
 .UNSPECIFIED.,.F.,.F.,.F.)
B_SPLINE_SURFACE_WITH_KNOTS((4,4),(4,2,2,2,2,4),(0.,1.),(0.,0.0783698481609191,
0.30877738612019,0.539184924080125,0.769592462040062,1.),.UNSPECIFIED.)
GEOMETRIC_REPRESENTATION_ITEM()
RATIONAL_B_SPLINE_SURFACE(((1.,1.,1.,1.,1.,1.,1.,1.,1.,1.,1.,1.),(0.987189825241073,
0.987189825241073,0.987189825241073,0.987189825241073,0.987189825241073,
0.987189825241073,0.987189825241073,0.987189825241073,0.987189825241073,
0.987189825241073,0.987189825241073,0.987189825241073),(0.987189825241073,
0.987189825241073,0.987189825241073,0.987189825241073,0.987189825241073,
0.987189825241073,0.987189825241073,0.987189825241073,0.987189825241073,
0.987189825241073,0.987189825241073,0.987189825241073),(1.,1.,1.,1.,1.,
1.,1.,1.,1.,1.,1.,1.)))
REPRESENTATION_ITEM('')
SURFACE()
);
#474=(
BOUNDED_SURFACE()
B_SPLINE_SURFACE(3,3,((#30777,#30778,#30779,#30780,#30781,#30782,#30783,
#30784,#30785,#30786,#30787,#30788),(#30789,#30790,#30791,#30792,#30793,
#30794,#30795,#30796,#30797,#30798,#30799,#30800),(#30801,#30802,#30803,
#30804,#30805,#30806,#30807,#30808,#30809,#30810,#30811,#30812),(#30813,
#30814,#30815,#30816,#30817,#30818,#30819,#30820,#30821,#30822,#30823,#30824)),
 .UNSPECIFIED.,.F.,.F.,.F.)
B_SPLINE_SURFACE_WITH_KNOTS((4,4),(4,2,2,2,2,4),(0.,1.),(0.,0.0783698481609191,
0.30877738612019,0.539184924080125,0.769592462040062,1.),.UNSPECIFIED.)
GEOMETRIC_REPRESENTATION_ITEM()
RATIONAL_B_SPLINE_SURFACE(((1.,1.,1.,1.,1.,1.,1.,1.,1.,1.,1.,1.),(0.987189825241073,
0.987189825241073,0.987189825241073,0.987189825241073,0.987189825241073,
0.987189825241073,0.987189825241073,0.987189825241073,0.987189825241073,
0.987189825241073,0.987189825241073,0.987189825241073),(0.987189825241073,
0.987189825241073,0.987189825241073,0.987189825241073,0.987189825241073,
0.987189825241073,0.987189825241073,0.987189825241073,0.987189825241073,
0.987189825241073,0.987189825241073,0.987189825241073),(1.,1.,1.,1.,1.,
1.,1.,1.,1.,1.,1.,1.)))
REPRESENTATION_ITEM('')
SURFACE()
);
#475=(
BOUNDED_SURFACE()
B_SPLINE_SURFACE(3,3,((#30825,#30826,#30827,#30828,#30829,#30830,#30831,
#30832,#30833,#30834,#30835,#30836),(#30837,#30838,#30839,#30840,#30841,
#30842,#30843,#30844,#30845,#30846,#30847,#30848),(#30849,#30850,#30851,
#30852,#30853,#30854,#30855,#30856,#30857,#30858,#30859,#30860),(#30861,
#30862,#30863,#30864,#30865,#30866,#30867,#30868,#30869,#30870,#30871,#30872)),
 .UNSPECIFIED.,.F.,.F.,.F.)
B_SPLINE_SURFACE_WITH_KNOTS((4,4),(4,2,2,2,2,4),(0.,1.),(0.,0.0783698504851113,
0.308777387863334,0.539184925242222,0.769592462621111,1.),.UNSPECIFIED.)
GEOMETRIC_REPRESENTATION_ITEM()
RATIONAL_B_SPLINE_SURFACE(((1.,1.,1.,1.,1.,1.,1.,1.,1.,1.,1.,1.),(0.833333333333332,
0.833333333333332,0.833333333333332,0.833333333333332,0.833333333333332,
0.833333333333332,0.833333333333332,0.833333333333332,0.833333333333332,
0.833333333333332,0.833333333333332,0.833333333333332),(0.833333333333332,
0.833333333333332,0.833333333333332,0.833333333333332,0.833333333333332,
0.833333333333332,0.833333333333332,0.833333333333332,0.833333333333332,
0.833333333333332,0.833333333333332,0.833333333333332),(1.,1.,1.,1.,1.,
1.,1.,1.,1.,1.,1.,1.)))
REPRESENTATION_ITEM('')
SURFACE()
);
#476=(
BOUNDED_SURFACE()
B_SPLINE_SURFACE(3,3,((#30889,#30890,#30891,#30892,#30893,#30894,#30895,
#30896,#30897,#30898,#30899,#30900),(#30901,#30902,#30903,#30904,#30905,
#30906,#30907,#30908,#30909,#30910,#30911,#30912),(#30913,#30914,#30915,
#30916,#30917,#30918,#30919,#30920,#30921,#30922,#30923,#30924),(#30925,
#30926,#30927,#30928,#30929,#30930,#30931,#30932,#30933,#30934,#30935,#30936)),
 .UNSPECIFIED.,.F.,.F.,.F.)
B_SPLINE_SURFACE_WITH_KNOTS((4,4),(4,2,2,2,2,4),(0.,1.),(0.,0.0783698504851113,
0.308777387863334,0.539184925242222,0.769592462621111,1.),.UNSPECIFIED.)
GEOMETRIC_REPRESENTATION_ITEM()
RATIONAL_B_SPLINE_SURFACE(((1.,1.,1.,1.,1.,1.,1.,1.,1.,1.,1.,1.),(0.987189825241073,
0.987189825241073,0.987189825241073,0.987189825241073,0.987189825241073,
0.987189825241073,0.987189825241073,0.987189825241073,0.987189825241073,
0.987189825241073,0.987189825241073,0.987189825241073),(0.987189825241073,
0.987189825241073,0.987189825241073,0.987189825241073,0.987189825241073,
0.987189825241073,0.987189825241073,0.987189825241073,0.987189825241073,
0.987189825241073,0.987189825241073,0.987189825241073),(1.,1.,1.,1.,1.,
1.,1.,1.,1.,1.,1.,1.)))
REPRESENTATION_ITEM('')
SURFACE()
);
#477=(
BOUNDED_SURFACE()
B_SPLINE_SURFACE(3,3,((#30937,#30938,#30939,#30940,#30941,#30942,#30943,
#30944,#30945,#30946,#30947,#30948),(#30949,#30950,#30951,#30952,#30953,
#30954,#30955,#30956,#30957,#30958,#30959,#30960),(#30961,#30962,#30963,
#30964,#30965,#30966,#30967,#30968,#30969,#30970,#30971,#30972),(#30973,
#30974,#30975,#30976,#30977,#30978,#30979,#30980,#30981,#30982,#30983,#30984)),
 .UNSPECIFIED.,.F.,.F.,.F.)
B_SPLINE_SURFACE_WITH_KNOTS((4,4),(4,2,2,2,2,4),(0.,1.),(0.,0.0783698504851113,
0.308777387863334,0.539184925242222,0.769592462621111,1.),.UNSPECIFIED.)
GEOMETRIC_REPRESENTATION_ITEM()
RATIONAL_B_SPLINE_SURFACE(((1.,1.,1.,1.,1.,1.,1.,1.,1.,1.,1.,1.),(0.987189825241073,
0.987189825241073,0.987189825241073,0.987189825241073,0.987189825241073,
0.987189825241073,0.987189825241073,0.987189825241073,0.987189825241073,
0.987189825241073,0.987189825241073,0.987189825241073),(0.987189825241073,
0.987189825241073,0.987189825241073,0.987189825241073,0.987189825241073,
0.987189825241073,0.987189825241073,0.987189825241073,0.987189825241073,
0.987189825241073,0.987189825241073,0.987189825241073),(1.,1.,1.,1.,1.,
1.,1.,1.,1.,1.,1.,1.)))
REPRESENTATION_ITEM('')
SURFACE()
);
#478=(
BOUNDED_SURFACE()
B_SPLINE_SURFACE(3,3,((#30985,#30986,#30987,#30988,#30989,#30990,#30991,
#30992,#30993,#30994,#30995,#30996),(#30997,#30998,#30999,#31000,#31001,
#31002,#31003,#31004,#31005,#31006,#31007,#31008),(#31009,#31010,#31011,
#31012,#31013,#31014,#31015,#31016,#31017,#31018,#31019,#31020),(#31021,
#31022,#31023,#31024,#31025,#31026,#31027,#31028,#31029,#31030,#31031,#31032)),
 .UNSPECIFIED.,.F.,.F.,.F.)
B_SPLINE_SURFACE_WITH_KNOTS((4,4),(4,2,2,2,2,4),(0.,1.),(0.,0.0783698504851048,
0.308777387863329,0.539184925242218,0.769592462621109,1.),.UNSPECIFIED.)
GEOMETRIC_REPRESENTATION_ITEM()
RATIONAL_B_SPLINE_SURFACE(((1.,1.,1.,1.,1.,1.,1.,1.,1.,1.,1.,1.),(0.833333333333332,
0.833333333333332,0.833333333333332,0.833333333333332,0.833333333333332,
0.833333333333332,0.833333333333332,0.833333333333332,0.833333333333332,
0.833333333333332,0.833333333333332,0.833333333333332),(0.833333333333332,
0.833333333333332,0.833333333333332,0.833333333333332,0.833333333333332,
0.833333333333332,0.833333333333332,0.833333333333332,0.833333333333332,
0.833333333333332,0.833333333333332,0.833333333333332),(1.,1.,1.,1.,1.,
1.,1.,1.,1.,1.,1.,1.)))
REPRESENTATION_ITEM('')
SURFACE()
);
#479=(
BOUNDED_SURFACE()
B_SPLINE_SURFACE(3,3,((#31049,#31050,#31051,#31052,#31053,#31054,#31055,
#31056,#31057,#31058,#31059,#31060),(#31061,#31062,#31063,#31064,#31065,
#31066,#31067,#31068,#31069,#31070,#31071,#31072),(#31073,#31074,#31075,
#31076,#31077,#31078,#31079,#31080,#31081,#31082,#31083,#31084),(#31085,
#31086,#31087,#31088,#31089,#31090,#31091,#31092,#31093,#31094,#31095,#31096)),
 .UNSPECIFIED.,.F.,.F.,.F.)
B_SPLINE_SURFACE_WITH_KNOTS((4,4),(4,2,2,2,2,4),(0.,1.),(0.,0.0783698504851048,
0.308777387863329,0.539184925242218,0.769592462621109,1.),.UNSPECIFIED.)
GEOMETRIC_REPRESENTATION_ITEM()
RATIONAL_B_SPLINE_SURFACE(((1.,1.,1.,1.,1.,1.,1.,1.,1.,1.,1.,1.),(0.987189825241073,
0.987189825241073,0.987189825241073,0.987189825241073,0.987189825241073,
0.987189825241073,0.987189825241073,0.987189825241073,0.987189825241073,
0.987189825241073,0.987189825241073,0.987189825241073),(0.987189825241073,
0.987189825241073,0.987189825241073,0.987189825241073,0.987189825241073,
0.987189825241073,0.987189825241073,0.987189825241073,0.987189825241073,
0.987189825241073,0.987189825241073,0.987189825241073),(1.,1.,1.,1.,1.,
1.,1.,1.,1.,1.,1.,1.)))
REPRESENTATION_ITEM('')
SURFACE()
);
#480=(
BOUNDED_SURFACE()
B_SPLINE_SURFACE(3,3,((#31097,#31098,#31099,#31100,#31101,#31102,#31103,
#31104,#31105,#31106,#31107,#31108),(#31109,#31110,#31111,#31112,#31113,
#31114,#31115,#31116,#31117,#31118,#31119,#31120),(#31121,#31122,#31123,
#31124,#31125,#31126,#31127,#31128,#31129,#31130,#31131,#31132),(#31133,
#31134,#31135,#31136,#31137,#31138,#31139,#31140,#31141,#31142,#31143,#31144)),
 .UNSPECIFIED.,.F.,.F.,.F.)
B_SPLINE_SURFACE_WITH_KNOTS((4,4),(4,2,2,2,2,4),(0.,1.),(0.,0.0783698504851048,
0.308777387863329,0.539184925242218,0.769592462621109,1.),.UNSPECIFIED.)
GEOMETRIC_REPRESENTATION_ITEM()
RATIONAL_B_SPLINE_SURFACE(((1.,1.,1.,1.,1.,1.,1.,1.,1.,1.,1.,1.),(0.987189825241073,
0.987189825241073,0.987189825241073,0.987189825241073,0.987189825241073,
0.987189825241073,0.987189825241073,0.987189825241073,0.987189825241073,
0.987189825241073,0.987189825241073,0.987189825241073),(0.987189825241073,
0.987189825241073,0.987189825241073,0.987189825241073,0.987189825241073,
0.987189825241073,0.987189825241073,0.987189825241073,0.987189825241073,
0.987189825241073,0.987189825241073,0.987189825241073),(1.,1.,1.,1.,1.,
1.,1.,1.,1.,1.,1.,1.)))
REPRESENTATION_ITEM('')
SURFACE()
);
#481=(
BOUNDED_SURFACE()
B_SPLINE_SURFACE(3,3,((#31145,#31146,#31147,#31148,#31149,#31150,#31151,
#31152,#31153,#31154,#31155,#31156),(#31157,#31158,#31159,#31160,#31161,
#31162,#31163,#31164,#31165,#31166,#31167,#31168),(#31169,#31170,#31171,
#31172,#31173,#31174,#31175,#31176,#31177,#31178,#31179,#31180),(#31181,
#31182,#31183,#31184,#31185,#31186,#31187,#31188,#31189,#31190,#31191,#31192)),
 .UNSPECIFIED.,.F.,.F.,.F.)
B_SPLINE_SURFACE_WITH_KNOTS((4,4),(4,2,2,2,2,4),(0.,1.),(0.,0.0783698481609166,
0.308777386120188,0.539184924080124,0.769592462040062,1.),.UNSPECIFIED.)
GEOMETRIC_REPRESENTATION_ITEM()
RATIONAL_B_SPLINE_SURFACE(((1.,1.,1.,1.,1.,1.,1.,1.,1.,1.,1.,1.),(0.833333333333333,
0.833333333333333,0.833333333333333,0.833333333333333,0.833333333333333,
0.833333333333333,0.833333333333333,0.833333333333333,0.833333333333333,
0.833333333333333,0.833333333333333,0.833333333333333),(0.833333333333333,
0.833333333333333,0.833333333333333,0.833333333333333,0.833333333333333,
0.833333333333333,0.833333333333333,0.833333333333333,0.833333333333333,
0.833333333333333,0.833333333333333,0.833333333333333),(1.,1.,1.,1.,1.,
1.,1.,1.,1.,1.,1.,1.)))
REPRESENTATION_ITEM('')
SURFACE()
);
#482=(
BOUNDED_SURFACE()
B_SPLINE_SURFACE(3,3,((#31209,#31210,#31211,#31212,#31213,#31214,#31215,
#31216,#31217,#31218,#31219,#31220),(#31221,#31222,#31223,#31224,#31225,
#31226,#31227,#31228,#31229,#31230,#31231,#31232),(#31233,#31234,#31235,
#31236,#31237,#31238,#31239,#31240,#31241,#31242,#31243,#31244),(#31245,
#31246,#31247,#31248,#31249,#31250,#31251,#31252,#31253,#31254,#31255,#31256)),
 .UNSPECIFIED.,.F.,.F.,.F.)
B_SPLINE_SURFACE_WITH_KNOTS((4,4),(4,2,2,2,2,4),(0.,1.),(0.,0.0783698481609166,
0.308777386120188,0.539184924080124,0.769592462040062,1.),.UNSPECIFIED.)
GEOMETRIC_REPRESENTATION_ITEM()
RATIONAL_B_SPLINE_SURFACE(((1.,1.,1.,1.,1.,1.,1.,1.,1.,1.,1.,1.),(0.987189825241073,
0.987189825241073,0.987189825241073,0.987189825241073,0.987189825241073,
0.987189825241073,0.987189825241073,0.987189825241073,0.987189825241073,
0.987189825241073,0.987189825241073,0.987189825241073),(0.987189825241073,
0.987189825241073,0.987189825241073,0.987189825241073,0.987189825241073,
0.987189825241073,0.987189825241073,0.987189825241073,0.987189825241073,
0.987189825241073,0.987189825241073,0.987189825241073),(1.,1.,1.,1.,1.,
1.,1.,1.,1.,1.,1.,1.)))
REPRESENTATION_ITEM('')
SURFACE()
);
#483=(
BOUNDED_SURFACE()
B_SPLINE_SURFACE(3,3,((#31257,#31258,#31259,#31260,#31261,#31262,#31263,
#31264,#31265,#31266,#31267,#31268),(#31269,#31270,#31271,#31272,#31273,
#31274,#31275,#31276,#31277,#31278,#31279,#31280),(#31281,#31282,#31283,
#31284,#31285,#31286,#31287,#31288,#31289,#31290,#31291,#31292),(#31293,
#31294,#31295,#31296,#31297,#31298,#31299,#31300,#31301,#31302,#31303,#31304)),
 .UNSPECIFIED.,.F.,.F.,.F.)
B_SPLINE_SURFACE_WITH_KNOTS((4,4),(4,2,2,2,2,4),(0.,1.),(0.,0.0783698481609166,
0.308777386120188,0.539184924080124,0.769592462040062,1.),.UNSPECIFIED.)
GEOMETRIC_REPRESENTATION_ITEM()
RATIONAL_B_SPLINE_SURFACE(((1.,1.,1.,1.,1.,1.,1.,1.,1.,1.,1.,1.),(0.987189825241073,
0.987189825241073,0.987189825241073,0.987189825241073,0.987189825241073,
0.987189825241073,0.987189825241073,0.987189825241073,0.987189825241073,
0.987189825241073,0.987189825241073,0.987189825241073),(0.987189825241073,
0.987189825241073,0.987189825241073,0.987189825241073,0.987189825241073,
0.987189825241073,0.987189825241073,0.987189825241073,0.987189825241073,
0.987189825241073,0.987189825241073,0.987189825241073),(1.,1.,1.,1.,1.,
1.,1.,1.,1.,1.,1.,1.)))
REPRESENTATION_ITEM('')
SURFACE()
);
#484=(
BOUNDED_SURFACE()
B_SPLINE_SURFACE(3,3,((#31305,#31306,#31307,#31308,#31309,#31310,#31311,
#31312,#31313,#31314,#31315,#31316),(#31317,#31318,#31319,#31320,#31321,
#31322,#31323,#31324,#31325,#31326,#31327,#31328),(#31329,#31330,#31331,
#31332,#31333,#31334,#31335,#31336,#31337,#31338,#31339,#31340),(#31341,
#31342,#31343,#31344,#31345,#31346,#31347,#31348,#31349,#31350,#31351,#31352)),
 .UNSPECIFIED.,.F.,.F.,.F.)
B_SPLINE_SURFACE_WITH_KNOTS((4,4),(4,2,2,2,2,4),(0.,1.),(0.,0.0783698437311068,
0.308777382797831,0.539184921865219,0.769592460932609,1.),.UNSPECIFIED.)
GEOMETRIC_REPRESENTATION_ITEM()
RATIONAL_B_SPLINE_SURFACE(((1.,1.,1.,1.,1.,1.,1.,1.,1.,1.,1.,1.),(0.833333333333331,
0.833333333333331,0.833333333333331,0.833333333333331,0.833333333333331,
0.833333333333331,0.833333333333331,0.833333333333331,0.833333333333331,
0.833333333333331,0.833333333333331,0.833333333333331),(0.833333333333331,
0.833333333333331,0.833333333333331,0.833333333333331,0.833333333333331,
0.833333333333331,0.833333333333331,0.833333333333331,0.833333333333331,
0.833333333333331,0.833333333333331,0.833333333333331),(1.,1.,1.,1.,1.,
1.,1.,1.,1.,1.,1.,1.)))
REPRESENTATION_ITEM('')
SURFACE()
);
#485=(
BOUNDED_SURFACE()
B_SPLINE_SURFACE(3,3,((#31369,#31370,#31371,#31372,#31373,#31374,#31375,
#31376,#31377,#31378,#31379,#31380),(#31381,#31382,#31383,#31384,#31385,
#31386,#31387,#31388,#31389,#31390,#31391,#31392),(#31393,#31394,#31395,
#31396,#31397,#31398,#31399,#31400,#31401,#31402,#31403,#31404),(#31405,
#31406,#31407,#31408,#31409,#31410,#31411,#31412,#31413,#31414,#31415,#31416)),
 .UNSPECIFIED.,.F.,.F.,.F.)
B_SPLINE_SURFACE_WITH_KNOTS((4,4),(4,2,2,2,2,4),(0.,1.),(0.,0.0783698437311068,
0.308777382797831,0.539184921865219,0.769592460932609,1.),.UNSPECIFIED.)
GEOMETRIC_REPRESENTATION_ITEM()
RATIONAL_B_SPLINE_SURFACE(((1.,1.,1.,1.,1.,1.,1.,1.,1.,1.,1.,1.),(0.987189825241073,
0.987189825241073,0.987189825241073,0.987189825241073,0.987189825241073,
0.987189825241073,0.987189825241073,0.987189825241073,0.987189825241073,
0.987189825241073,0.987189825241073,0.987189825241073),(0.987189825241073,
0.987189825241073,0.987189825241073,0.987189825241073,0.987189825241073,
0.987189825241073,0.987189825241073,0.987189825241073,0.987189825241073,
0.987189825241073,0.987189825241073,0.987189825241073),(1.,1.,1.,1.,1.,
1.,1.,1.,1.,1.,1.,1.)))
REPRESENTATION_ITEM('')
SURFACE()
);
#486=(
BOUNDED_SURFACE()
B_SPLINE_SURFACE(3,3,((#31417,#31418,#31419,#31420,#31421,#31422,#31423,
#31424,#31425,#31426,#31427,#31428),(#31429,#31430,#31431,#31432,#31433,
#31434,#31435,#31436,#31437,#31438,#31439,#31440),(#31441,#31442,#31443,
#31444,#31445,#31446,#31447,#31448,#31449,#31450,#31451,#31452),(#31453,
#31454,#31455,#31456,#31457,#31458,#31459,#31460,#31461,#31462,#31463,#31464)),
 .UNSPECIFIED.,.F.,.F.,.F.)
B_SPLINE_SURFACE_WITH_KNOTS((4,4),(4,2,2,2,2,4),(0.,1.),(0.,0.0783698437311068,
0.308777382797831,0.539184921865219,0.769592460932609,1.),.UNSPECIFIED.)
GEOMETRIC_REPRESENTATION_ITEM()
RATIONAL_B_SPLINE_SURFACE(((1.,1.,1.,1.,1.,1.,1.,1.,1.,1.,1.,1.),(0.987189825241073,
0.987189825241073,0.987189825241073,0.987189825241073,0.987189825241073,
0.987189825241073,0.987189825241073,0.987189825241073,0.987189825241073,
0.987189825241073,0.987189825241073,0.987189825241073),(0.987189825241073,
0.987189825241073,0.987189825241073,0.987189825241073,0.987189825241073,
0.987189825241073,0.987189825241073,0.987189825241073,0.987189825241073,
0.987189825241073,0.987189825241073,0.987189825241073),(1.,1.,1.,1.,1.,
1.,1.,1.,1.,1.,1.,1.)))
REPRESENTATION_ITEM('')
SURFACE()
);
#487=(
BOUNDED_SURFACE()
B_SPLINE_SURFACE(3,3,((#31465,#31466,#31467,#31468,#31469,#31470,#31471,
#31472,#31473,#31474,#31475,#31476),(#31477,#31478,#31479,#31480,#31481,
#31482,#31483,#31484,#31485,#31486,#31487,#31488),(#31489,#31490,#31491,
#31492,#31493,#31494,#31495,#31496,#31497,#31498,#31499,#31500),(#31501,
#31502,#31503,#31504,#31505,#31506,#31507,#31508,#31509,#31510,#31511,#31512)),
 .UNSPECIFIED.,.F.,.F.,.F.)
B_SPLINE_SURFACE_WITH_KNOTS((4,4),(4,2,2,2,2,4),(0.,1.),(0.,0.078369838840124,
0.308777379129593,0.539184919419728,0.769592459709864,1.),.UNSPECIFIED.)
GEOMETRIC_REPRESENTATION_ITEM()
RATIONAL_B_SPLINE_SURFACE(((1.,1.,1.,1.,1.,1.,1.,1.,1.,1.,1.,1.),(0.833333333333332,
0.833333333333332,0.833333333333332,0.833333333333332,0.833333333333332,
0.833333333333332,0.833333333333332,0.833333333333332,0.833333333333332,
0.833333333333332,0.833333333333332,0.833333333333332),(0.833333333333332,
0.833333333333332,0.833333333333332,0.833333333333332,0.833333333333332,
0.833333333333332,0.833333333333332,0.833333333333332,0.833333333333332,
0.833333333333332,0.833333333333332,0.833333333333332),(1.,1.,1.,1.,1.,
1.,1.,1.,1.,1.,1.,1.)))
REPRESENTATION_ITEM('')
SURFACE()
);
#488=(
BOUNDED_SURFACE()
B_SPLINE_SURFACE(3,3,((#31529,#31530,#31531,#31532,#31533,#31534,#31535,
#31536,#31537,#31538,#31539,#31540),(#31541,#31542,#31543,#31544,#31545,
#31546,#31547,#31548,#31549,#31550,#31551,#31552),(#31553,#31554,#31555,
#31556,#31557,#31558,#31559,#31560,#31561,#31562,#31563,#31564),(#31565,
#31566,#31567,#31568,#31569,#31570,#31571,#31572,#31573,#31574,#31575,#31576)),
 .UNSPECIFIED.,.F.,.F.,.F.)
B_SPLINE_SURFACE_WITH_KNOTS((4,4),(4,2,2,2,2,4),(0.,1.),(0.,0.078369838840124,
0.308777379129593,0.539184919419728,0.769592459709864,1.),.UNSPECIFIED.)
GEOMETRIC_REPRESENTATION_ITEM()
RATIONAL_B_SPLINE_SURFACE(((1.,1.,1.,1.,1.,1.,1.,1.,1.,1.,1.,1.),(0.987189825241073,
0.987189825241073,0.987189825241073,0.987189825241073,0.987189825241073,
0.987189825241073,0.987189825241073,0.987189825241073,0.987189825241073,
0.987189825241073,0.987189825241073,0.987189825241073),(0.987189825241073,
0.987189825241073,0.987189825241073,0.987189825241073,0.987189825241073,
0.987189825241073,0.987189825241073,0.987189825241073,0.987189825241073,
0.987189825241073,0.987189825241073,0.987189825241073),(1.,1.,1.,1.,1.,
1.,1.,1.,1.,1.,1.,1.)))
REPRESENTATION_ITEM('')
SURFACE()
);
#489=(
BOUNDED_SURFACE()
B_SPLINE_SURFACE(3,3,((#31577,#31578,#31579,#31580,#31581,#31582,#31583,
#31584,#31585,#31586,#31587,#31588),(#31589,#31590,#31591,#31592,#31593,
#31594,#31595,#31596,#31597,#31598,#31599,#31600),(#31601,#31602,#31603,
#31604,#31605,#31606,#31607,#31608,#31609,#31610,#31611,#31612),(#31613,
#31614,#31615,#31616,#31617,#31618,#31619,#31620,#31621,#31622,#31623,#31624)),
 .UNSPECIFIED.,.F.,.F.,.F.)
B_SPLINE_SURFACE_WITH_KNOTS((4,4),(4,2,2,2,2,4),(0.,1.),(0.,0.078369838840124,
0.308777379129593,0.539184919419728,0.769592459709864,1.),.UNSPECIFIED.)
GEOMETRIC_REPRESENTATION_ITEM()
RATIONAL_B_SPLINE_SURFACE(((1.,1.,1.,1.,1.,1.,1.,1.,1.,1.,1.,1.),(0.987189825241073,
0.987189825241073,0.987189825241073,0.987189825241073,0.987189825241073,
0.987189825241073,0.987189825241073,0.987189825241073,0.987189825241073,
0.987189825241073,0.987189825241073,0.987189825241073),(0.987189825241073,
0.987189825241073,0.987189825241073,0.987189825241073,0.987189825241073,
0.987189825241073,0.987189825241073,0.987189825241073,0.987189825241073,
0.987189825241073,0.987189825241073,0.987189825241073),(1.,1.,1.,1.,1.,
1.,1.,1.,1.,1.,1.,1.)))
REPRESENTATION_ITEM('')
SURFACE()
);
#490=(
BOUNDED_SURFACE()
B_SPLINE_SURFACE(3,3,((#31625,#31626,#31627,#31628,#31629,#31630,#31631,
#31632,#31633,#31634,#31635,#31636),(#31637,#31638,#31639,#31640,#31641,
#31642,#31643,#31644,#31645,#31646,#31647,#31648),(#31649,#31650,#31651,
#31652,#31653,#31654,#31655,#31656,#31657,#31658,#31659,#31660),(#31661,
#31662,#31663,#31664,#31665,#31666,#31667,#31668,#31669,#31670,#31671,#31672)),
 .UNSPECIFIED.,.F.,.F.,.F.)
B_SPLINE_SURFACE_WITH_KNOTS((4,4),(4,2,2,2,2,4),(0.,1.),(0.,0.0783698352504276,
0.308777376437321,0.539184917624879,0.76959245881244,1.),.UNSPECIFIED.)
GEOMETRIC_REPRESENTATION_ITEM()
RATIONAL_B_SPLINE_SURFACE(((1.,1.,1.,1.,1.,1.,1.,1.,1.,1.,1.,1.),(0.833333333333332,
0.833333333333332,0.833333333333332,0.833333333333332,0.833333333333332,
0.833333333333332,0.833333333333332,0.833333333333332,0.833333333333332,
0.833333333333332,0.833333333333332,0.833333333333332),(0.833333333333332,
0.833333333333332,0.833333333333332,0.833333333333332,0.833333333333332,
0.833333333333332,0.833333333333332,0.833333333333332,0.833333333333332,
0.833333333333332,0.833333333333332,0.833333333333332),(1.,1.,1.,1.,1.,
1.,1.,1.,1.,1.,1.,1.)))
REPRESENTATION_ITEM('')
SURFACE()
);
#491=(
BOUNDED_SURFACE()
B_SPLINE_SURFACE(3,3,((#31689,#31690,#31691,#31692,#31693,#31694,#31695,
#31696,#31697,#31698,#31699,#31700),(#31701,#31702,#31703,#31704,#31705,
#31706,#31707,#31708,#31709,#31710,#31711,#31712),(#31713,#31714,#31715,
#31716,#31717,#31718,#31719,#31720,#31721,#31722,#31723,#31724),(#31725,
#31726,#31727,#31728,#31729,#31730,#31731,#31732,#31733,#31734,#31735,#31736)),
 .UNSPECIFIED.,.F.,.F.,.F.)
B_SPLINE_SURFACE_WITH_KNOTS((4,4),(4,2,2,2,2,4),(0.,1.),(0.,0.0783698352504276,
0.308777376437321,0.539184917624879,0.76959245881244,1.),.UNSPECIFIED.)
GEOMETRIC_REPRESENTATION_ITEM()
RATIONAL_B_SPLINE_SURFACE(((1.,1.,1.,1.,1.,1.,1.,1.,1.,1.,1.,1.),(0.987189825241073,
0.987189825241073,0.987189825241073,0.987189825241073,0.987189825241073,
0.987189825241073,0.987189825241073,0.987189825241073,0.987189825241073,
0.987189825241073,0.987189825241073,0.987189825241073),(0.987189825241073,
0.987189825241073,0.987189825241073,0.987189825241073,0.987189825241073,
0.987189825241073,0.987189825241073,0.987189825241073,0.987189825241073,
0.987189825241073,0.987189825241073,0.987189825241073),(1.,1.,1.,1.,1.,
1.,1.,1.,1.,1.,1.,1.)))
REPRESENTATION_ITEM('')
SURFACE()
);
#492=(
BOUNDED_SURFACE()
B_SPLINE_SURFACE(3,3,((#31737,#31738,#31739,#31740,#31741,#31742,#31743,
#31744,#31745,#31746,#31747,#31748),(#31749,#31750,#31751,#31752,#31753,
#31754,#31755,#31756,#31757,#31758,#31759,#31760),(#31761,#31762,#31763,
#31764,#31765,#31766,#31767,#31768,#31769,#31770,#31771,#31772),(#31773,
#31774,#31775,#31776,#31777,#31778,#31779,#31780,#31781,#31782,#31783,#31784)),
 .UNSPECIFIED.,.F.,.F.,.F.)
B_SPLINE_SURFACE_WITH_KNOTS((4,4),(4,2,2,2,2,4),(0.,1.),(0.,0.0783698352504276,
0.308777376437321,0.539184917624879,0.76959245881244,1.),.UNSPECIFIED.)
GEOMETRIC_REPRESENTATION_ITEM()
RATIONAL_B_SPLINE_SURFACE(((1.,1.,1.,1.,1.,1.,1.,1.,1.,1.,1.,1.),(0.987189825241073,
0.987189825241073,0.987189825241073,0.987189825241073,0.987189825241073,
0.987189825241073,0.987189825241073,0.987189825241073,0.987189825241073,
0.987189825241073,0.987189825241073,0.987189825241073),(0.987189825241073,
0.987189825241073,0.987189825241073,0.987189825241073,0.987189825241073,
0.987189825241073,0.987189825241073,0.987189825241073,0.987189825241073,
0.987189825241073,0.987189825241073,0.987189825241073),(1.,1.,1.,1.,1.,
1.,1.,1.,1.,1.,1.,1.)))
REPRESENTATION_ITEM('')
SURFACE()
);
#493=(
BOUNDED_SURFACE()
B_SPLINE_SURFACE(3,3,((#31785,#31786,#31787,#31788,#31789,#31790,#31791,
#31792,#31793,#31794,#31795,#31796),(#31797,#31798,#31799,#31800,#31801,
#31802,#31803,#31804,#31805,#31806,#31807,#31808),(#31809,#31810,#31811,
#31812,#31813,#31814,#31815,#31816,#31817,#31818,#31819,#31820),(#31821,
#31822,#31823,#31824,#31825,#31826,#31827,#31828,#31829,#31830,#31831,#31832)),
 .UNSPECIFIED.,.F.,.F.,.F.)
B_SPLINE_SURFACE_WITH_KNOTS((4,4),(4,2,2,2,2,4),(0.,1.),(0.,0.0783698293107417,
0.308777371982557,0.539184914655036,0.769592457327518,1.),.UNSPECIFIED.)
GEOMETRIC_REPRESENTATION_ITEM()
RATIONAL_B_SPLINE_SURFACE(((1.,1.,1.,1.,1.,1.,1.,1.,1.,1.,1.,1.),(0.833333333333332,
0.833333333333332,0.833333333333332,0.833333333333332,0.833333333333332,
0.833333333333332,0.833333333333332,0.833333333333332,0.833333333333332,
0.833333333333332,0.833333333333332,0.833333333333332),(0.833333333333332,
0.833333333333332,0.833333333333332,0.833333333333332,0.833333333333332,
0.833333333333332,0.833333333333332,0.833333333333332,0.833333333333332,
0.833333333333332,0.833333333333332,0.833333333333332),(1.,1.,1.,1.,1.,
1.,1.,1.,1.,1.,1.,1.)))
REPRESENTATION_ITEM('')
SURFACE()
);
#494=(
BOUNDED_SURFACE()
B_SPLINE_SURFACE(3,3,((#31849,#31850,#31851,#31852,#31853,#31854,#31855,
#31856,#31857,#31858,#31859,#31860),(#31861,#31862,#31863,#31864,#31865,
#31866,#31867,#31868,#31869,#31870,#31871,#31872),(#31873,#31874,#31875,
#31876,#31877,#31878,#31879,#31880,#31881,#31882,#31883,#31884),(#31885,
#31886,#31887,#31888,#31889,#31890,#31891,#31892,#31893,#31894,#31895,#31896)),
 .UNSPECIFIED.,.F.,.F.,.F.)
B_SPLINE_SURFACE_WITH_KNOTS((4,4),(4,2,2,2,2,4),(0.,1.),(0.,0.0783698293107417,
0.308777371982557,0.539184914655036,0.769592457327518,1.),.UNSPECIFIED.)
GEOMETRIC_REPRESENTATION_ITEM()
RATIONAL_B_SPLINE_SURFACE(((1.,1.,1.,1.,1.,1.,1.,1.,1.,1.,1.,1.),(0.987189825241073,
0.987189825241073,0.987189825241073,0.987189825241073,0.987189825241073,
0.987189825241073,0.987189825241073,0.987189825241073,0.987189825241073,
0.987189825241073,0.987189825241073,0.987189825241073),(0.987189825241073,
0.987189825241073,0.987189825241073,0.987189825241073,0.987189825241073,
0.987189825241073,0.987189825241073,0.987189825241073,0.987189825241073,
0.987189825241073,0.987189825241073,0.987189825241073),(1.,1.,1.,1.,1.,
1.,1.,1.,1.,1.,1.,1.)))
REPRESENTATION_ITEM('')
SURFACE()
);
#495=(
BOUNDED_SURFACE()
B_SPLINE_SURFACE(3,3,((#31897,#31898,#31899,#31900,#31901,#31902,#31903,
#31904,#31905,#31906,#31907,#31908),(#31909,#31910,#31911,#31912,#31913,
#31914,#31915,#31916,#31917,#31918,#31919,#31920),(#31921,#31922,#31923,
#31924,#31925,#31926,#31927,#31928,#31929,#31930,#31931,#31932),(#31933,
#31934,#31935,#31936,#31937,#31938,#31939,#31940,#31941,#31942,#31943,#31944)),
 .UNSPECIFIED.,.F.,.F.,.F.)
B_SPLINE_SURFACE_WITH_KNOTS((4,4),(4,2,2,2,2,4),(0.,1.),(0.,0.0783698293107417,
0.308777371982557,0.539184914655036,0.769592457327518,1.),.UNSPECIFIED.)
GEOMETRIC_REPRESENTATION_ITEM()
RATIONAL_B_SPLINE_SURFACE(((1.,1.,1.,1.,1.,1.,1.,1.,1.,1.,1.,1.),(0.987189825241073,
0.987189825241073,0.987189825241073,0.987189825241073,0.987189825241073,
0.987189825241073,0.987189825241073,0.987189825241073,0.987189825241073,
0.987189825241073,0.987189825241073,0.987189825241073),(0.987189825241073,
0.987189825241073,0.987189825241073,0.987189825241073,0.987189825241073,
0.987189825241073,0.987189825241073,0.987189825241073,0.987189825241073,
0.987189825241073,0.987189825241073,0.987189825241073),(1.,1.,1.,1.,1.,
1.,1.,1.,1.,1.,1.,1.)))
REPRESENTATION_ITEM('')
SURFACE()
);
#496=(
BOUNDED_SURFACE()
B_SPLINE_SURFACE(3,3,((#31945,#31946,#31947,#31948,#31949,#31950,#31951,
#31952,#31953,#31954,#31955,#31956,#31957,#31958),(#31959,#31960,#31961,
#31962,#31963,#31964,#31965,#31966,#31967,#31968,#31969,#31970,#31971,#31972),
(#31973,#31974,#31975,#31976,#31977,#31978,#31979,#31980,#31981,#31982,
#31983,#31984,#31985,#31986),(#31987,#31988,#31989,#31990,#31991,#31992,
#31993,#31994,#31995,#31996,#31997,#31998,#31999,#32000)),.UNSPECIFIED.,
 .F.,.F.,.F.)
B_SPLINE_SURFACE_WITH_KNOTS((4,4),(4,2,2,2,2,2,4),(0.,1.),(0.,0.0183879232268621,
0.0783698352504225,0.308777376437317,0.539184917624877,0.769592458812438,
1.),.UNSPECIFIED.)
GEOMETRIC_REPRESENTATION_ITEM()
RATIONAL_B_SPLINE_SURFACE(((1.,1.,1.,1.,1.,1.,1.,1.,1.,1.,1.,1.,1.,1.),
(0.833333333333332,0.833333333333332,0.833333333333332,0.833333333333332,
0.833333333333332,0.833333333333332,0.833333333333332,0.833333333333332,
0.833333333333332,0.833333333333332,0.833333333333332,0.833333333333332,
0.833333333333332,0.833333333333332),(0.833333333333332,0.833333333333332,
0.833333333333332,0.833333333333332,0.833333333333332,0.833333333333332,
0.833333333333332,0.833333333333332,0.833333333333332,0.833333333333332,
0.833333333333332,0.833333333333332,0.833333333333332,0.833333333333332),
(1.,1.,1.,1.,1.,1.,1.,1.,1.,1.,1.,1.,1.,1.)))
REPRESENTATION_ITEM('')
SURFACE()
);
#497=(
BOUNDED_SURFACE()
B_SPLINE_SURFACE(3,3,((#32019,#32020,#32021,#32022,#32023,#32024,#32025,
#32026,#32027,#32028,#32029,#32030,#32031,#32032),(#32033,#32034,#32035,
#32036,#32037,#32038,#32039,#32040,#32041,#32042,#32043,#32044,#32045,#32046),
(#32047,#32048,#32049,#32050,#32051,#32052,#32053,#32054,#32055,#32056,
#32057,#32058,#32059,#32060),(#32061,#32062,#32063,#32064,#32065,#32066,
#32067,#32068,#32069,#32070,#32071,#32072,#32073,#32074)),.UNSPECIFIED.,
 .F.,.F.,.F.)
B_SPLINE_SURFACE_WITH_KNOTS((4,4),(4,2,2,2,2,2,4),(0.,1.),(0.,0.0183879232268621,
0.0783698352504225,0.308777376437317,0.539184917624877,0.769592458812438,
1.),.UNSPECIFIED.)
GEOMETRIC_REPRESENTATION_ITEM()
RATIONAL_B_SPLINE_SURFACE(((1.,1.,1.,1.,1.,1.,1.,1.,1.,1.,1.,1.,1.,1.),
(0.987189825241073,0.987189825241073,0.987189825241073,0.987189825241073,
0.987189825241073,0.987189825241073,0.987189825241073,0.987189825241073,
0.987189825241073,0.987189825241073,0.987189825241073,0.987189825241073,
0.987189825241073,0.987189825241073),(0.987189825241073,0.987189825241073,
0.987189825241073,0.987189825241073,0.987189825241073,0.987189825241073,
0.987189825241073,0.987189825241073,0.987189825241073,0.987189825241073,
0.987189825241073,0.987189825241073,0.987189825241073,0.987189825241073),
(1.,1.,1.,1.,1.,1.,1.,1.,1.,1.,1.,1.,1.,1.)))
REPRESENTATION_ITEM('')
SURFACE()
);
#498=(
BOUNDED_SURFACE()
B_SPLINE_SURFACE(3,3,((#32075,#32076,#32077,#32078,#32079,#32080,#32081,
#32082,#32083,#32084,#32085,#32086,#32087,#32088),(#32089,#32090,#32091,
#32092,#32093,#32094,#32095,#32096,#32097,#32098,#32099,#32100,#32101,#32102),
(#32103,#32104,#32105,#32106,#32107,#32108,#32109,#32110,#32111,#32112,
#32113,#32114,#32115,#32116),(#32117,#32118,#32119,#32120,#32121,#32122,
#32123,#32124,#32125,#32126,#32127,#32128,#32129,#32130)),.UNSPECIFIED.,
 .F.,.F.,.F.)
B_SPLINE_SURFACE_WITH_KNOTS((4,4),(4,2,2,2,2,2,4),(0.,1.),(0.,0.0183879232268621,
0.0783698352504225,0.308777376437317,0.539184917624877,0.769592458812438,
1.),.UNSPECIFIED.)
GEOMETRIC_REPRESENTATION_ITEM()
RATIONAL_B_SPLINE_SURFACE(((1.,1.,1.,1.,1.,1.,1.,1.,1.,1.,1.,1.,1.,1.),
(0.987189825241073,0.987189825241073,0.987189825241073,0.987189825241073,
0.987189825241073,0.987189825241073,0.987189825241073,0.987189825241073,
0.987189825241073,0.987189825241073,0.987189825241073,0.987189825241073,
0.987189825241073,0.987189825241073),(0.987189825241073,0.987189825241073,
0.987189825241073,0.987189825241073,0.987189825241073,0.987189825241073,
0.987189825241073,0.987189825241073,0.987189825241073,0.987189825241073,
0.987189825241073,0.987189825241073,0.987189825241073,0.987189825241073),
(1.,1.,1.,1.,1.,1.,1.,1.,1.,1.,1.,1.,1.,1.)))
REPRESENTATION_ITEM('')
SURFACE()
);
#499=(
BOUNDED_SURFACE()
B_SPLINE_SURFACE(3,3,((#32131,#32132,#32133,#32134,#32135,#32136,#32137,
#32138,#32139,#32140,#32141,#32142),(#32143,#32144,#32145,#32146,#32147,
#32148,#32149,#32150,#32151,#32152,#32153,#32154),(#32155,#32156,#32157,
#32158,#32159,#32160,#32161,#32162,#32163,#32164,#32165,#32166),(#32167,
#32168,#32169,#32170,#32171,#32172,#32173,#32174,#32175,#32176,#32177,#32178)),
 .UNSPECIFIED.,.F.,.F.,.F.)
B_SPLINE_SURFACE_WITH_KNOTS((4,4),(4,2,2,2,2,4),(0.,1.),(0.,0.0783698388401176,
0.308777379129589,0.539184919419725,0.769592459709862,1.),.UNSPECIFIED.)
GEOMETRIC_REPRESENTATION_ITEM()
RATIONAL_B_SPLINE_SURFACE(((1.,1.,1.,1.,1.,1.,1.,1.,1.,1.,1.,1.),(0.833333333333331,
0.833333333333331,0.833333333333331,0.833333333333331,0.833333333333331,
0.833333333333331,0.833333333333331,0.833333333333331,0.833333333333331,
0.833333333333331,0.833333333333331,0.833333333333331),(0.833333333333331,
0.833333333333331,0.833333333333331,0.833333333333331,0.833333333333331,
0.833333333333331,0.833333333333331,0.833333333333331,0.833333333333331,
0.833333333333331,0.833333333333331,0.833333333333331),(1.,1.,1.,1.,1.,
1.,1.,1.,1.,1.,1.,1.)))
REPRESENTATION_ITEM('')
SURFACE()
);
#500=(
BOUNDED_SURFACE()
B_SPLINE_SURFACE(3,3,((#32195,#32196,#32197,#32198,#32199,#32200,#32201,
#32202,#32203,#32204,#32205,#32206),(#32207,#32208,#32209,#32210,#32211,
#32212,#32213,#32214,#32215,#32216,#32217,#32218),(#32219,#32220,#32221,
#32222,#32223,#32224,#32225,#32226,#32227,#32228,#32229,#32230),(#32231,
#32232,#32233,#32234,#32235,#32236,#32237,#32238,#32239,#32240,#32241,#32242)),
 .UNSPECIFIED.,.F.,.F.,.F.)
B_SPLINE_SURFACE_WITH_KNOTS((4,4),(4,2,2,2,2,4),(0.,1.),(0.,0.0783698388401176,
0.308777379129589,0.539184919419725,0.769592459709862,1.),.UNSPECIFIED.)
GEOMETRIC_REPRESENTATION_ITEM()
RATIONAL_B_SPLINE_SURFACE(((1.,1.,1.,1.,1.,1.,1.,1.,1.,1.,1.,1.),(0.987189825241073,
0.987189825241073,0.987189825241073,0.987189825241073,0.987189825241073,
0.987189825241073,0.987189825241073,0.987189825241073,0.987189825241073,
0.987189825241073,0.987189825241073,0.987189825241073),(0.987189825241073,
0.987189825241073,0.987189825241073,0.987189825241073,0.987189825241073,
0.987189825241073,0.987189825241073,0.987189825241073,0.987189825241073,
0.987189825241073,0.987189825241073,0.987189825241073),(1.,1.,1.,1.,1.,
1.,1.,1.,1.,1.,1.,1.)))
REPRESENTATION_ITEM('')
SURFACE()
);
#501=(
BOUNDED_SURFACE()
B_SPLINE_SURFACE(3,3,((#32243,#32244,#32245,#32246,#32247,#32248,#32249,
#32250,#32251,#32252,#32253,#32254),(#32255,#32256,#32257,#32258,#32259,
#32260,#32261,#32262,#32263,#32264,#32265,#32266),(#32267,#32268,#32269,
#32270,#32271,#32272,#32273,#32274,#32275,#32276,#32277,#32278),(#32279,
#32280,#32281,#32282,#32283,#32284,#32285,#32286,#32287,#32288,#32289,#32290)),
 .UNSPECIFIED.,.F.,.F.,.F.)
B_SPLINE_SURFACE_WITH_KNOTS((4,4),(4,2,2,2,2,4),(0.,1.),(0.,0.0783698388401176,
0.308777379129589,0.539184919419725,0.769592459709862,1.),.UNSPECIFIED.)
GEOMETRIC_REPRESENTATION_ITEM()
RATIONAL_B_SPLINE_SURFACE(((1.,1.,1.,1.,1.,1.,1.,1.,1.,1.,1.,1.),(0.987189825241073,
0.987189825241073,0.987189825241073,0.987189825241073,0.987189825241073,
0.987189825241073,0.987189825241073,0.987189825241073,0.987189825241073,
0.987189825241073,0.987189825241073,0.987189825241073),(0.987189825241073,
0.987189825241073,0.987189825241073,0.987189825241073,0.987189825241073,
0.987189825241073,0.987189825241073,0.987189825241073,0.987189825241073,
0.987189825241073,0.987189825241073,0.987189825241073),(1.,1.,1.,1.,1.,
1.,1.,1.,1.,1.,1.,1.)))
REPRESENTATION_ITEM('')
SURFACE()
);
#502=(
BOUNDED_SURFACE()
B_SPLINE_SURFACE(3,3,((#32291,#32292,#32293,#32294,#32295,#32296,#32297,
#32298,#32299,#32300,#32301,#32302),(#32303,#32304,#32305,#32306,#32307,
#32308,#32309,#32310,#32311,#32312,#32313,#32314),(#32315,#32316,#32317,
#32318,#32319,#32320,#32321,#32322,#32323,#32324,#32325,#32326),(#32327,
#32328,#32329,#32330,#32331,#32332,#32333,#32334,#32335,#32336,#32337,#32338)),
 .UNSPECIFIED.,.F.,.F.,.F.)
B_SPLINE_SURFACE_WITH_KNOTS((4,4),(4,2,2,2,2,4),(0.,1.),(0.,0.0783698437311062,
0.30877738279783,0.539184921865219,0.76959246093261,1.),.UNSPECIFIED.)
GEOMETRIC_REPRESENTATION_ITEM()
RATIONAL_B_SPLINE_SURFACE(((1.,1.,1.,1.,1.,1.,1.,1.,1.,1.,1.,1.),(0.833333333333332,
0.833333333333332,0.833333333333332,0.833333333333332,0.833333333333332,
0.833333333333332,0.833333333333332,0.833333333333332,0.833333333333332,
0.833333333333332,0.833333333333332,0.833333333333332),(0.833333333333332,
0.833333333333332,0.833333333333332,0.833333333333332,0.833333333333332,
0.833333333333332,0.833333333333332,0.833333333333332,0.833333333333332,
0.833333333333332,0.833333333333332,0.833333333333332),(1.,1.,1.,1.,1.,
1.,1.,1.,1.,1.,1.,1.)))
REPRESENTATION_ITEM('')
SURFACE()
);
#503=(
BOUNDED_SURFACE()
B_SPLINE_SURFACE(3,3,((#32355,#32356,#32357,#32358,#32359,#32360,#32361,
#32362,#32363,#32364,#32365,#32366),(#32367,#32368,#32369,#32370,#32371,
#32372,#32373,#32374,#32375,#32376,#32377,#32378),(#32379,#32380,#32381,
#32382,#32383,#32384,#32385,#32386,#32387,#32388,#32389,#32390),(#32391,
#32392,#32393,#32394,#32395,#32396,#32397,#32398,#32399,#32400,#32401,#32402)),
 .UNSPECIFIED.,.F.,.F.,.F.)
B_SPLINE_SURFACE_WITH_KNOTS((4,4),(4,2,2,2,2,4),(0.,1.),(0.,0.0783698437311062,
0.30877738279783,0.539184921865219,0.76959246093261,1.),.UNSPECIFIED.)
GEOMETRIC_REPRESENTATION_ITEM()
RATIONAL_B_SPLINE_SURFACE(((1.,1.,1.,1.,1.,1.,1.,1.,1.,1.,1.,1.),(0.987189825241073,
0.987189825241073,0.987189825241073,0.987189825241073,0.987189825241073,
0.987189825241073,0.987189825241073,0.987189825241073,0.987189825241073,
0.987189825241073,0.987189825241073,0.987189825241073),(0.987189825241073,
0.987189825241073,0.987189825241073,0.987189825241073,0.987189825241073,
0.987189825241073,0.987189825241073,0.987189825241073,0.987189825241073,
0.987189825241073,0.987189825241073,0.987189825241073),(1.,1.,1.,1.,1.,
1.,1.,1.,1.,1.,1.,1.)))
REPRESENTATION_ITEM('')
SURFACE()
);
#504=(
BOUNDED_SURFACE()
B_SPLINE_SURFACE(3,3,((#32403,#32404,#32405,#32406,#32407,#32408,#32409,
#32410,#32411,#32412,#32413,#32414),(#32415,#32416,#32417,#32418,#32419,
#32420,#32421,#32422,#32423,#32424,#32425,#32426),(#32427,#32428,#32429,
#32430,#32431,#32432,#32433,#32434,#32435,#32436,#32437,#32438),(#32439,
#32440,#32441,#32442,#32443,#32444,#32445,#32446,#32447,#32448,#32449,#32450)),
 .UNSPECIFIED.,.F.,.F.,.F.)
B_SPLINE_SURFACE_WITH_KNOTS((4,4),(4,2,2,2,2,4),(0.,1.),(0.,0.0783698437311062,
0.30877738279783,0.539184921865219,0.76959246093261,1.),.UNSPECIFIED.)
GEOMETRIC_REPRESENTATION_ITEM()
RATIONAL_B_SPLINE_SURFACE(((1.,1.,1.,1.,1.,1.,1.,1.,1.,1.,1.,1.),(0.987189825241073,
0.987189825241073,0.987189825241073,0.987189825241073,0.987189825241073,
0.987189825241073,0.987189825241073,0.987189825241073,0.987189825241073,
0.987189825241073,0.987189825241073,0.987189825241073),(0.987189825241073,
0.987189825241073,0.987189825241073,0.987189825241073,0.987189825241073,
0.987189825241073,0.987189825241073,0.987189825241073,0.987189825241073,
0.987189825241073,0.987189825241073,0.987189825241073),(1.,1.,1.,1.,1.,
1.,1.,1.,1.,1.,1.,1.)))
REPRESENTATION_ITEM('')
SURFACE()
);
#505=(
BOUNDED_SURFACE()
B_SPLINE_SURFACE(3,3,((#32451,#32452,#32453,#32454,#32455,#32456,#32457,
#32458,#32459,#32460,#32461,#32462),(#32463,#32464,#32465,#32466,#32467,
#32468,#32469,#32470,#32471,#32472,#32473,#32474),(#32475,#32476,#32477,
#32478,#32479,#32480,#32481,#32482,#32483,#32484,#32485,#32486),(#32487,
#32488,#32489,#32490,#32491,#32492,#32493,#32494,#32495,#32496,#32497,#32498)),
 .UNSPECIFIED.,.F.,.F.,.F.)
B_SPLINE_SURFACE_WITH_KNOTS((4,4),(4,2,2,2,2,4),(0.,1.),(0.,0.0783698481609152,
0.308777386120187,0.539184924080123,0.769592462040061,1.),.UNSPECIFIED.)
GEOMETRIC_REPRESENTATION_ITEM()
RATIONAL_B_SPLINE_SURFACE(((1.,1.,1.,1.,1.,1.,1.,1.,1.,1.,1.,1.),(0.987189825241073,
0.987189825241073,0.987189825241073,0.987189825241073,0.987189825241073,
0.987189825241073,0.987189825241073,0.987189825241073,0.987189825241073,
0.987189825241073,0.987189825241073,0.987189825241073),(0.987189825241073,
0.987189825241073,0.987189825241073,0.987189825241073,0.987189825241073,
0.987189825241073,0.987189825241073,0.987189825241073,0.987189825241073,
0.987189825241073,0.987189825241073,0.987189825241073),(1.,1.,1.,1.,1.,
1.,1.,1.,1.,1.,1.,1.)))
REPRESENTATION_ITEM('')
SURFACE()
);
#506=(
BOUNDED_SURFACE()
B_SPLINE_SURFACE(3,3,((#32507,#32508,#32509,#32510,#32511,#32512,#32513,
#32514,#32515,#32516,#32517,#32518),(#32519,#32520,#32521,#32522,#32523,
#32524,#32525,#32526,#32527,#32528,#32529,#32530),(#32531,#32532,#32533,
#32534,#32535,#32536,#32537,#32538,#32539,#32540,#32541,#32542),(#32543,
#32544,#32545,#32546,#32547,#32548,#32549,#32550,#32551,#32552,#32553,#32554)),
 .UNSPECIFIED.,.F.,.F.,.F.)
B_SPLINE_SURFACE_WITH_KNOTS((4,4),(4,2,2,2,2,4),(0.,1.),(0.,0.0783698481609152,
0.308777386120187,0.539184924080123,0.769592462040061,1.),.UNSPECIFIED.)
GEOMETRIC_REPRESENTATION_ITEM()
RATIONAL_B_SPLINE_SURFACE(((1.,1.,1.,1.,1.,1.,1.,1.,1.,1.,1.,1.),(0.987189825241073,
0.987189825241073,0.987189825241073,0.987189825241073,0.987189825241073,
0.987189825241073,0.987189825241073,0.987189825241073,0.987189825241073,
0.987189825241073,0.987189825241073,0.987189825241073),(0.987189825241073,
0.987189825241073,0.987189825241073,0.987189825241073,0.987189825241073,
0.987189825241073,0.987189825241073,0.987189825241073,0.987189825241073,
0.987189825241073,0.987189825241073,0.987189825241073),(1.,1.,1.,1.,1.,
1.,1.,1.,1.,1.,1.,1.)))
REPRESENTATION_ITEM('')
SURFACE()
);
#507=(
BOUNDED_SURFACE()
B_SPLINE_SURFACE(3,3,((#32563,#32564,#32565,#32566,#32567,#32568,#32569,
#32570,#32571,#32572,#32573,#32574),(#32575,#32576,#32577,#32578,#32579,
#32580,#32581,#32582,#32583,#32584,#32585,#32586),(#32587,#32588,#32589,
#32590,#32591,#32592,#32593,#32594,#32595,#32596,#32597,#32598),(#32599,
#32600,#32601,#32602,#32603,#32604,#32605,#32606,#32607,#32608,#32609,#32610)),
 .UNSPECIFIED.,.F.,.F.,.F.)
B_SPLINE_SURFACE_WITH_KNOTS((4,4),(4,2,2,2,2,4),(0.,1.),(0.,0.0783698481609152,
0.308777386120187,0.539184924080123,0.769592462040061,1.),.UNSPECIFIED.)
GEOMETRIC_REPRESENTATION_ITEM()
RATIONAL_B_SPLINE_SURFACE(((1.,1.,1.,1.,1.,1.,1.,1.,1.,1.,1.,1.),(0.833333333333331,
0.833333333333331,0.833333333333331,0.833333333333331,0.833333333333331,
0.833333333333331,0.833333333333331,0.833333333333331,0.833333333333331,
0.833333333333331,0.833333333333331,0.833333333333331),(0.833333333333331,
0.833333333333331,0.833333333333331,0.833333333333331,0.833333333333331,
0.833333333333331,0.833333333333331,0.833333333333331,0.833333333333331,
0.833333333333331,0.833333333333331,0.833333333333331),(1.,1.,1.,1.,1.,
1.,1.,1.,1.,1.,1.,1.)))
REPRESENTATION_ITEM('')
SURFACE()
);
#508=(
BOUNDED_SURFACE()
B_SPLINE_SURFACE(3,3,((#32611,#32612,#32613,#32614,#32615,#32616,#32617,
#32618,#32619,#32620,#32621,#32622),(#32623,#32624,#32625,#32626,#32627,
#32628,#32629,#32630,#32631,#32632,#32633,#32634),(#32635,#32636,#32637,
#32638,#32639,#32640,#32641,#32642,#32643,#32644,#32645,#32646),(#32647,
#32648,#32649,#32650,#32651,#32652,#32653,#32654,#32655,#32656,#32657,#32658)),
 .UNSPECIFIED.,.F.,.F.,.F.)
B_SPLINE_SURFACE_WITH_KNOTS((4,4),(4,2,2,2,2,4),(0.,1.),(0.,0.0783698504851105,
0.308777387863333,0.539184925242221,0.76959246262111,1.),.UNSPECIFIED.)
GEOMETRIC_REPRESENTATION_ITEM()
RATIONAL_B_SPLINE_SURFACE(((1.,1.,1.,1.,1.,1.,1.,1.,1.,1.,1.,1.),(0.833333333333333,
0.833333333333333,0.833333333333333,0.833333333333333,0.833333333333333,
0.833333333333333,0.833333333333333,0.833333333333333,0.833333333333333,
0.833333333333333,0.833333333333333,0.833333333333333),(0.833333333333333,
0.833333333333333,0.833333333333333,0.833333333333333,0.833333333333333,
0.833333333333333,0.833333333333333,0.833333333333333,0.833333333333333,
0.833333333333333,0.833333333333333,0.833333333333333),(1.,1.,1.,1.,1.,
1.,1.,1.,1.,1.,1.,1.)))
REPRESENTATION_ITEM('')
SURFACE()
);
#509=(
BOUNDED_SURFACE()
B_SPLINE_SURFACE(3,3,((#32675,#32676,#32677,#32678,#32679,#32680,#32681,
#32682,#32683,#32684,#32685,#32686),(#32687,#32688,#32689,#32690,#32691,
#32692,#32693,#32694,#32695,#32696,#32697,#32698),(#32699,#32700,#32701,
#32702,#32703,#32704,#32705,#32706,#32707,#32708,#32709,#32710),(#32711,
#32712,#32713,#32714,#32715,#32716,#32717,#32718,#32719,#32720,#32721,#32722)),
 .UNSPECIFIED.,.F.,.F.,.F.)
B_SPLINE_SURFACE_WITH_KNOTS((4,4),(4,2,2,2,2,4),(0.,1.),(0.,0.0783698504851105,
0.308777387863333,0.539184925242221,0.76959246262111,1.),.UNSPECIFIED.)
GEOMETRIC_REPRESENTATION_ITEM()
RATIONAL_B_SPLINE_SURFACE(((1.,1.,1.,1.,1.,1.,1.,1.,1.,1.,1.,1.),(0.987189825241073,
0.987189825241073,0.987189825241073,0.987189825241073,0.987189825241073,
0.987189825241073,0.987189825241073,0.987189825241073,0.987189825241073,
0.987189825241073,0.987189825241073,0.987189825241073),(0.987189825241073,
0.987189825241073,0.987189825241073,0.987189825241073,0.987189825241073,
0.987189825241073,0.987189825241073,0.987189825241073,0.987189825241073,
0.987189825241073,0.987189825241073,0.987189825241073),(1.,1.,1.,1.,1.,
1.,1.,1.,1.,1.,1.,1.)))
REPRESENTATION_ITEM('')
SURFACE()
);
#510=(
BOUNDED_SURFACE()
B_SPLINE_SURFACE(3,3,((#32723,#32724,#32725,#32726,#32727,#32728,#32729,
#32730,#32731,#32732,#32733,#32734),(#32735,#32736,#32737,#32738,#32739,
#32740,#32741,#32742,#32743,#32744,#32745,#32746),(#32747,#32748,#32749,
#32750,#32751,#32752,#32753,#32754,#32755,#32756,#32757,#32758),(#32759,
#32760,#32761,#32762,#32763,#32764,#32765,#32766,#32767,#32768,#32769,#32770)),
 .UNSPECIFIED.,.F.,.F.,.F.)
B_SPLINE_SURFACE_WITH_KNOTS((4,4),(4,2,2,2,2,4),(0.,1.),(0.,0.0783698504851105,
0.308777387863333,0.539184925242221,0.76959246262111,1.),.UNSPECIFIED.)
GEOMETRIC_REPRESENTATION_ITEM()
RATIONAL_B_SPLINE_SURFACE(((1.,1.,1.,1.,1.,1.,1.,1.,1.,1.,1.,1.),(0.987189825241073,
0.987189825241073,0.987189825241073,0.987189825241073,0.987189825241073,
0.987189825241073,0.987189825241073,0.987189825241073,0.987189825241073,
0.987189825241073,0.987189825241073,0.987189825241073),(0.987189825241073,
0.987189825241073,0.987189825241073,0.987189825241073,0.987189825241073,
0.987189825241073,0.987189825241073,0.987189825241073,0.987189825241073,
0.987189825241073,0.987189825241073,0.987189825241073),(1.,1.,1.,1.,1.,
1.,1.,1.,1.,1.,1.,1.)))
REPRESENTATION_ITEM('')
SURFACE()
);
#511=(
BOUNDED_SURFACE()
B_SPLINE_SURFACE(3,3,((#32771,#32772,#32773,#32774,#32775,#32776,#32777,
#32778,#32779,#32780,#32781,#32782),(#32783,#32784,#32785,#32786,#32787,
#32788,#32789,#32790,#32791,#32792,#32793,#32794),(#32795,#32796,#32797,
#32798,#32799,#32800,#32801,#32802,#32803,#32804,#32805,#32806),(#32807,
#32808,#32809,#32810,#32811,#32812,#32813,#32814,#32815,#32816,#32817,#32818)),
 .UNSPECIFIED.,.F.,.F.,.F.)
B_SPLINE_SURFACE_WITH_KNOTS((4,4),(4,2,2,2,2,4),(0.,1.),(0.,0.0783698504851009,
0.308777387863326,0.539184925242216,0.769592462621108,1.),.UNSPECIFIED.)
GEOMETRIC_REPRESENTATION_ITEM()
RATIONAL_B_SPLINE_SURFACE(((1.,1.,1.,1.,1.,1.,1.,1.,1.,1.,1.,1.),(0.833333333333333,
0.833333333333333,0.833333333333333,0.833333333333333,0.833333333333333,
0.833333333333333,0.833333333333333,0.833333333333333,0.833333333333333,
0.833333333333333,0.833333333333333,0.833333333333333),(0.833333333333333,
0.833333333333333,0.833333333333333,0.833333333333333,0.833333333333333,
0.833333333333333,0.833333333333333,0.833333333333333,0.833333333333333,
0.833333333333333,0.833333333333333,0.833333333333333),(1.,1.,1.,1.,1.,
1.,1.,1.,1.,1.,1.,1.)))
REPRESENTATION_ITEM('')
SURFACE()
);
#512=(
BOUNDED_SURFACE()
B_SPLINE_SURFACE(3,3,((#32835,#32836,#32837,#32838,#32839,#32840,#32841,
#32842,#32843,#32844,#32845,#32846),(#32847,#32848,#32849,#32850,#32851,
#32852,#32853,#32854,#32855,#32856,#32857,#32858),(#32859,#32860,#32861,
#32862,#32863,#32864,#32865,#32866,#32867,#32868,#32869,#32870),(#32871,
#32872,#32873,#32874,#32875,#32876,#32877,#32878,#32879,#32880,#32881,#32882)),
 .UNSPECIFIED.,.F.,.F.,.F.)
B_SPLINE_SURFACE_WITH_KNOTS((4,4),(4,2,2,2,2,4),(0.,1.),(0.,0.0783698504851009,
0.308777387863326,0.539184925242216,0.769592462621108,1.),.UNSPECIFIED.)
GEOMETRIC_REPRESENTATION_ITEM()
RATIONAL_B_SPLINE_SURFACE(((1.,1.,1.,1.,1.,1.,1.,1.,1.,1.,1.,1.),(0.987189825241073,
0.987189825241073,0.987189825241073,0.987189825241073,0.987189825241073,
0.987189825241073,0.987189825241073,0.987189825241073,0.987189825241073,
0.987189825241073,0.987189825241073,0.987189825241073),(0.987189825241073,
0.987189825241073,0.987189825241073,0.987189825241073,0.987189825241073,
0.987189825241073,0.987189825241073,0.987189825241073,0.987189825241073,
0.987189825241073,0.987189825241073,0.987189825241073),(1.,1.,1.,1.,1.,
1.,1.,1.,1.,1.,1.,1.)))
REPRESENTATION_ITEM('')
SURFACE()
);
#513=(
BOUNDED_SURFACE()
B_SPLINE_SURFACE(3,3,((#32883,#32884,#32885,#32886,#32887,#32888,#32889,
#32890,#32891,#32892,#32893,#32894),(#32895,#32896,#32897,#32898,#32899,
#32900,#32901,#32902,#32903,#32904,#32905,#32906),(#32907,#32908,#32909,
#32910,#32911,#32912,#32913,#32914,#32915,#32916,#32917,#32918),(#32919,
#32920,#32921,#32922,#32923,#32924,#32925,#32926,#32927,#32928,#32929,#32930)),
 .UNSPECIFIED.,.F.,.F.,.F.)
B_SPLINE_SURFACE_WITH_KNOTS((4,4),(4,2,2,2,2,4),(0.,1.),(0.,0.0783698504851009,
0.308777387863326,0.539184925242216,0.769592462621108,1.),.UNSPECIFIED.)
GEOMETRIC_REPRESENTATION_ITEM()
RATIONAL_B_SPLINE_SURFACE(((1.,1.,1.,1.,1.,1.,1.,1.,1.,1.,1.,1.),(0.987189825241073,
0.987189825241073,0.987189825241073,0.987189825241073,0.987189825241073,
0.987189825241073,0.987189825241073,0.987189825241073,0.987189825241073,
0.987189825241073,0.987189825241073,0.987189825241073),(0.987189825241073,
0.987189825241073,0.987189825241073,0.987189825241073,0.987189825241073,
0.987189825241073,0.987189825241073,0.987189825241073,0.987189825241073,
0.987189825241073,0.987189825241073,0.987189825241073),(1.,1.,1.,1.,1.,
1.,1.,1.,1.,1.,1.,1.)))
REPRESENTATION_ITEM('')
SURFACE()
);
#514=(
BOUNDED_SURFACE()
B_SPLINE_SURFACE(3,3,((#32931,#32932,#32933,#32934,#32935,#32936,#32937,
#32938,#32939,#32940,#32941,#32942),(#32943,#32944,#32945,#32946,#32947,
#32948,#32949,#32950,#32951,#32952,#32953,#32954),(#32955,#32956,#32957,
#32958,#32959,#32960,#32961,#32962,#32963,#32964,#32965,#32966),(#32967,
#32968,#32969,#32970,#32971,#32972,#32973,#32974,#32975,#32976,#32977,#32978)),
 .UNSPECIFIED.,.F.,.F.,.F.)
B_SPLINE_SURFACE_WITH_KNOTS((4,4),(4,2,2,2,2,4),(0.,1.),(0.,0.0783698481609159,
0.308777386120187,0.539184924080124,0.769592462040061,1.),.UNSPECIFIED.)
GEOMETRIC_REPRESENTATION_ITEM()
RATIONAL_B_SPLINE_SURFACE(((1.,1.,1.,1.,1.,1.,1.,1.,1.,1.,1.,1.),(0.833333333333332,
0.833333333333332,0.833333333333332,0.833333333333332,0.833333333333332,
0.833333333333332,0.833333333333332,0.833333333333332,0.833333333333332,
0.833333333333332,0.833333333333332,0.833333333333332),(0.833333333333332,
0.833333333333332,0.833333333333332,0.833333333333332,0.833333333333332,
0.833333333333332,0.833333333333332,0.833333333333332,0.833333333333332,
0.833333333333332,0.833333333333332,0.833333333333332),(1.,1.,1.,1.,1.,
1.,1.,1.,1.,1.,1.,1.)))
REPRESENTATION_ITEM('')
SURFACE()
);
#515=(
BOUNDED_SURFACE()
B_SPLINE_SURFACE(3,3,((#32995,#32996,#32997,#32998,#32999,#33000,#33001,
#33002,#33003,#33004,#33005,#33006),(#33007,#33008,#33009,#33010,#33011,
#33012,#33013,#33014,#33015,#33016,#33017,#33018),(#33019,#33020,#33021,
#33022,#33023,#33024,#33025,#33026,#33027,#33028,#33029,#33030),(#33031,
#33032,#33033,#33034,#33035,#33036,#33037,#33038,#33039,#33040,#33041,#33042)),
 .UNSPECIFIED.,.F.,.F.,.F.)
B_SPLINE_SURFACE_WITH_KNOTS((4,4),(4,2,2,2,2,4),(0.,1.),(0.,0.0783698481609159,
0.308777386120187,0.539184924080124,0.769592462040061,1.),.UNSPECIFIED.)
GEOMETRIC_REPRESENTATION_ITEM()
RATIONAL_B_SPLINE_SURFACE(((1.,1.,1.,1.,1.,1.,1.,1.,1.,1.,1.,1.),(0.987189825241073,
0.987189825241073,0.987189825241073,0.987189825241073,0.987189825241073,
0.987189825241073,0.987189825241073,0.987189825241073,0.987189825241073,
0.987189825241073,0.987189825241073,0.987189825241073),(0.987189825241073,
0.987189825241073,0.987189825241073,0.987189825241073,0.987189825241073,
0.987189825241073,0.987189825241073,0.987189825241073,0.987189825241073,
0.987189825241073,0.987189825241073,0.987189825241073),(1.,1.,1.,1.,1.,
1.,1.,1.,1.,1.,1.,1.)))
REPRESENTATION_ITEM('')
SURFACE()
);
#516=(
BOUNDED_SURFACE()
B_SPLINE_SURFACE(3,3,((#33043,#33044,#33045,#33046,#33047,#33048,#33049,
#33050,#33051,#33052,#33053,#33054),(#33055,#33056,#33057,#33058,#33059,
#33060,#33061,#33062,#33063,#33064,#33065,#33066),(#33067,#33068,#33069,
#33070,#33071,#33072,#33073,#33074,#33075,#33076,#33077,#33078),(#33079,
#33080,#33081,#33082,#33083,#33084,#33085,#33086,#33087,#33088,#33089,#33090)),
 .UNSPECIFIED.,.F.,.F.,.F.)
B_SPLINE_SURFACE_WITH_KNOTS((4,4),(4,2,2,2,2,4),(0.,1.),(0.,0.0783698481609159,
0.308777386120187,0.539184924080124,0.769592462040061,1.),.UNSPECIFIED.)
GEOMETRIC_REPRESENTATION_ITEM()
RATIONAL_B_SPLINE_SURFACE(((1.,1.,1.,1.,1.,1.,1.,1.,1.,1.,1.,1.),(0.987189825241073,
0.987189825241073,0.987189825241073,0.987189825241073,0.987189825241073,
0.987189825241073,0.987189825241073,0.987189825241073,0.987189825241073,
0.987189825241073,0.987189825241073,0.987189825241073),(0.987189825241073,
0.987189825241073,0.987189825241073,0.987189825241073,0.987189825241073,
0.987189825241073,0.987189825241073,0.987189825241073,0.987189825241073,
0.987189825241073,0.987189825241073,0.987189825241073),(1.,1.,1.,1.,1.,
1.,1.,1.,1.,1.,1.,1.)))
REPRESENTATION_ITEM('')
SURFACE()
);
#517=(
BOUNDED_SURFACE()
B_SPLINE_SURFACE(3,3,((#33091,#33092,#33093,#33094,#33095,#33096,#33097,
#33098,#33099,#33100,#33101,#33102),(#33103,#33104,#33105,#33106,#33107,
#33108,#33109,#33110,#33111,#33112,#33113,#33114),(#33115,#33116,#33117,
#33118,#33119,#33120,#33121,#33122,#33123,#33124,#33125,#33126),(#33127,
#33128,#33129,#33130,#33131,#33132,#33133,#33134,#33135,#33136,#33137,#33138)),
 .UNSPECIFIED.,.F.,.F.,.F.)
B_SPLINE_SURFACE_WITH_KNOTS((4,4),(4,2,2,2,2,4),(0.,1.),(0.,0.0783698437310911,
0.308777382797819,0.539184921865211,0.769592460932606,1.),.UNSPECIFIED.)
GEOMETRIC_REPRESENTATION_ITEM()
RATIONAL_B_SPLINE_SURFACE(((1.,1.,1.,1.,1.,1.,1.,1.,1.,1.,1.,1.),(0.833333333333333,
0.833333333333333,0.833333333333333,0.833333333333333,0.833333333333333,
0.833333333333333,0.833333333333333,0.833333333333333,0.833333333333333,
0.833333333333333,0.833333333333333,0.833333333333333),(0.833333333333333,
0.833333333333333,0.833333333333333,0.833333333333333,0.833333333333333,
0.833333333333333,0.833333333333333,0.833333333333333,0.833333333333333,
0.833333333333333,0.833333333333333,0.833333333333333),(1.,1.,1.,1.,1.,
1.,1.,1.,1.,1.,1.,1.)))
REPRESENTATION_ITEM('')
SURFACE()
);
#518=(
BOUNDED_SURFACE()
B_SPLINE_SURFACE(3,3,((#33155,#33156,#33157,#33158,#33159,#33160,#33161,
#33162,#33163,#33164,#33165,#33166),(#33167,#33168,#33169,#33170,#33171,
#33172,#33173,#33174,#33175,#33176,#33177,#33178),(#33179,#33180,#33181,
#33182,#33183,#33184,#33185,#33186,#33187,#33188,#33189,#33190),(#33191,
#33192,#33193,#33194,#33195,#33196,#33197,#33198,#33199,#33200,#33201,#33202)),
 .UNSPECIFIED.,.F.,.F.,.F.)
B_SPLINE_SURFACE_WITH_KNOTS((4,4),(4,2,2,2,2,4),(0.,1.),(0.,0.0783698437310911,
0.308777382797819,0.539184921865211,0.769592460932606,1.),.UNSPECIFIED.)
GEOMETRIC_REPRESENTATION_ITEM()
RATIONAL_B_SPLINE_SURFACE(((1.,1.,1.,1.,1.,1.,1.,1.,1.,1.,1.,1.),(0.987189825241073,
0.987189825241073,0.987189825241073,0.987189825241073,0.987189825241073,
0.987189825241073,0.987189825241073,0.987189825241073,0.987189825241073,
0.987189825241073,0.987189825241073,0.987189825241073),(0.987189825241073,
0.987189825241073,0.987189825241073,0.987189825241073,0.987189825241073,
0.987189825241073,0.987189825241073,0.987189825241073,0.987189825241073,
0.987189825241073,0.987189825241073,0.987189825241073),(1.,1.,1.,1.,1.,
1.,1.,1.,1.,1.,1.,1.)))
REPRESENTATION_ITEM('')
SURFACE()
);
#519=(
BOUNDED_SURFACE()
B_SPLINE_SURFACE(3,3,((#33203,#33204,#33205,#33206,#33207,#33208,#33209,
#33210,#33211,#33212,#33213,#33214),(#33215,#33216,#33217,#33218,#33219,
#33220,#33221,#33222,#33223,#33224,#33225,#33226),(#33227,#33228,#33229,
#33230,#33231,#33232,#33233,#33234,#33235,#33236,#33237,#33238),(#33239,
#33240,#33241,#33242,#33243,#33244,#33245,#33246,#33247,#33248,#33249,#33250)),
 .UNSPECIFIED.,.F.,.F.,.F.)
B_SPLINE_SURFACE_WITH_KNOTS((4,4),(4,2,2,2,2,4),(0.,1.),(0.,0.0783698437310911,
0.308777382797819,0.539184921865211,0.769592460932606,1.),.UNSPECIFIED.)
GEOMETRIC_REPRESENTATION_ITEM()
RATIONAL_B_SPLINE_SURFACE(((1.,1.,1.,1.,1.,1.,1.,1.,1.,1.,1.,1.),(0.987189825241073,
0.987189825241073,0.987189825241073,0.987189825241073,0.987189825241073,
0.987189825241073,0.987189825241073,0.987189825241073,0.987189825241073,
0.987189825241073,0.987189825241073,0.987189825241073),(0.987189825241073,
0.987189825241073,0.987189825241073,0.987189825241073,0.987189825241073,
0.987189825241073,0.987189825241073,0.987189825241073,0.987189825241073,
0.987189825241073,0.987189825241073,0.987189825241073),(1.,1.,1.,1.,1.,
1.,1.,1.,1.,1.,1.,1.)))
REPRESENTATION_ITEM('')
SURFACE()
);
#520=(
BOUNDED_SURFACE()
B_SPLINE_SURFACE(3,3,((#33251,#33252,#33253,#33254,#33255,#33256,#33257,
#33258,#33259,#33260,#33261,#33262),(#33263,#33264,#33265,#33266,#33267,
#33268,#33269,#33270,#33271,#33272,#33273,#33274),(#33275,#33276,#33277,
#33278,#33279,#33280,#33281,#33282,#33283,#33284,#33285,#33286),(#33287,
#33288,#33289,#33290,#33291,#33292,#33293,#33294,#33295,#33296,#33297,#33298)),
 .UNSPECIFIED.,.F.,.F.,.F.)
B_SPLINE_SURFACE_WITH_KNOTS((4,4),(4,2,2,2,2,4),(0.,1.),(0.,0.0783698388401225,
0.308777379129592,0.539184919419727,0.769592459709863,1.),.UNSPECIFIED.)
GEOMETRIC_REPRESENTATION_ITEM()
RATIONAL_B_SPLINE_SURFACE(((1.,1.,1.,1.,1.,1.,1.,1.,1.,1.,1.,1.),(0.833333333333332,
0.833333333333332,0.833333333333332,0.833333333333332,0.833333333333332,
0.833333333333332,0.833333333333332,0.833333333333332,0.833333333333332,
0.833333333333332,0.833333333333332,0.833333333333332),(0.833333333333332,
0.833333333333332,0.833333333333332,0.833333333333332,0.833333333333332,
0.833333333333332,0.833333333333332,0.833333333333332,0.833333333333332,
0.833333333333332,0.833333333333332,0.833333333333332),(1.,1.,1.,1.,1.,
1.,1.,1.,1.,1.,1.,1.)))
REPRESENTATION_ITEM('')
SURFACE()
);
#521=(
BOUNDED_SURFACE()
B_SPLINE_SURFACE(3,3,((#33315,#33316,#33317,#33318,#33319,#33320,#33321,
#33322,#33323,#33324,#33325,#33326),(#33327,#33328,#33329,#33330,#33331,
#33332,#33333,#33334,#33335,#33336,#33337,#33338),(#33339,#33340,#33341,
#33342,#33343,#33344,#33345,#33346,#33347,#33348,#33349,#33350),(#33351,
#33352,#33353,#33354,#33355,#33356,#33357,#33358,#33359,#33360,#33361,#33362)),
 .UNSPECIFIED.,.F.,.F.,.F.)
B_SPLINE_SURFACE_WITH_KNOTS((4,4),(4,2,2,2,2,4),(0.,1.),(0.,0.0783698388401225,
0.308777379129592,0.539184919419727,0.769592459709863,1.),.UNSPECIFIED.)
GEOMETRIC_REPRESENTATION_ITEM()
RATIONAL_B_SPLINE_SURFACE(((1.,1.,1.,1.,1.,1.,1.,1.,1.,1.,1.,1.),(0.987189825241073,
0.987189825241073,0.987189825241073,0.987189825241073,0.987189825241073,
0.987189825241073,0.987189825241073,0.987189825241073,0.987189825241073,
0.987189825241073,0.987189825241073,0.987189825241073),(0.987189825241073,
0.987189825241073,0.987189825241073,0.987189825241073,0.987189825241073,
0.987189825241073,0.987189825241073,0.987189825241073,0.987189825241073,
0.987189825241073,0.987189825241073,0.987189825241073),(1.,1.,1.,1.,1.,
1.,1.,1.,1.,1.,1.,1.)))
REPRESENTATION_ITEM('')
SURFACE()
);
#522=(
BOUNDED_SURFACE()
B_SPLINE_SURFACE(3,3,((#33363,#33364,#33365,#33366,#33367,#33368,#33369,
#33370,#33371,#33372,#33373,#33374),(#33375,#33376,#33377,#33378,#33379,
#33380,#33381,#33382,#33383,#33384,#33385,#33386),(#33387,#33388,#33389,
#33390,#33391,#33392,#33393,#33394,#33395,#33396,#33397,#33398),(#33399,
#33400,#33401,#33402,#33403,#33404,#33405,#33406,#33407,#33408,#33409,#33410)),
 .UNSPECIFIED.,.F.,.F.,.F.)
B_SPLINE_SURFACE_WITH_KNOTS((4,4),(4,2,2,2,2,4),(0.,1.),(0.,0.0783698388401225,
0.308777379129592,0.539184919419727,0.769592459709863,1.),.UNSPECIFIED.)
GEOMETRIC_REPRESENTATION_ITEM()
RATIONAL_B_SPLINE_SURFACE(((1.,1.,1.,1.,1.,1.,1.,1.,1.,1.,1.,1.),(0.987189825241073,
0.987189825241073,0.987189825241073,0.987189825241073,0.987189825241073,
0.987189825241073,0.987189825241073,0.987189825241073,0.987189825241073,
0.987189825241073,0.987189825241073,0.987189825241073),(0.987189825241073,
0.987189825241073,0.987189825241073,0.987189825241073,0.987189825241073,
0.987189825241073,0.987189825241073,0.987189825241073,0.987189825241073,
0.987189825241073,0.987189825241073,0.987189825241073),(1.,1.,1.,1.,1.,
1.,1.,1.,1.,1.,1.,1.)))
REPRESENTATION_ITEM('')
SURFACE()
);
#523=(
BOUNDED_SURFACE()
B_SPLINE_SURFACE(3,3,((#33411,#33412,#33413,#33414,#33415,#33416,#33417,
#33418,#33419,#33420,#33421,#33422),(#33423,#33424,#33425,#33426,#33427,
#33428,#33429,#33430,#33431,#33432,#33433,#33434),(#33435,#33436,#33437,
#33438,#33439,#33440,#33441,#33442,#33443,#33444,#33445,#33446),(#33447,
#33448,#33449,#33450,#33451,#33452,#33453,#33454,#33455,#33456,#33457,#33458)),
 .UNSPECIFIED.,.F.,.F.,.F.)
B_SPLINE_SURFACE_WITH_KNOTS((4,4),(4,2,2,2,2,4),(0.,1.),(0.,0.078369835250435,
0.308777376437327,0.539184917624883,0.769592458812442,1.),.UNSPECIFIED.)
GEOMETRIC_REPRESENTATION_ITEM()
RATIONAL_B_SPLINE_SURFACE(((1.,1.,1.,1.,1.,1.,1.,1.,1.,1.,1.,1.),(0.833333333333333,
0.833333333333333,0.833333333333333,0.833333333333333,0.833333333333333,
0.833333333333333,0.833333333333333,0.833333333333333,0.833333333333333,
0.833333333333333,0.833333333333333,0.833333333333333),(0.833333333333333,
0.833333333333333,0.833333333333333,0.833333333333333,0.833333333333333,
0.833333333333333,0.833333333333333,0.833333333333333,0.833333333333333,
0.833333333333333,0.833333333333333,0.833333333333333),(1.,1.,1.,1.,1.,
1.,1.,1.,1.,1.,1.,1.)))
REPRESENTATION_ITEM('')
SURFACE()
);
#524=(
BOUNDED_SURFACE()
B_SPLINE_SURFACE(3,3,((#33475,#33476,#33477,#33478,#33479,#33480,#33481,
#33482,#33483,#33484,#33485,#33486),(#33487,#33488,#33489,#33490,#33491,
#33492,#33493,#33494,#33495,#33496,#33497,#33498),(#33499,#33500,#33501,
#33502,#33503,#33504,#33505,#33506,#33507,#33508,#33509,#33510),(#33511,
#33512,#33513,#33514,#33515,#33516,#33517,#33518,#33519,#33520,#33521,#33522)),
 .UNSPECIFIED.,.F.,.F.,.F.)
B_SPLINE_SURFACE_WITH_KNOTS((4,4),(4,2,2,2,2,4),(0.,1.),(0.,0.078369835250435,
0.308777376437327,0.539184917624883,0.769592458812442,1.),.UNSPECIFIED.)
GEOMETRIC_REPRESENTATION_ITEM()
RATIONAL_B_SPLINE_SURFACE(((1.,1.,1.,1.,1.,1.,1.,1.,1.,1.,1.,1.),(0.987189825241073,
0.987189825241073,0.987189825241073,0.987189825241073,0.987189825241073,
0.987189825241073,0.987189825241073,0.987189825241073,0.987189825241073,
0.987189825241073,0.987189825241073,0.987189825241073),(0.987189825241073,
0.987189825241073,0.987189825241073,0.987189825241073,0.987189825241073,
0.987189825241073,0.987189825241073,0.987189825241073,0.987189825241073,
0.987189825241073,0.987189825241073,0.987189825241073),(1.,1.,1.,1.,1.,
1.,1.,1.,1.,1.,1.,1.)))
REPRESENTATION_ITEM('')
SURFACE()
);
#525=(
BOUNDED_SURFACE()
B_SPLINE_SURFACE(3,3,((#33523,#33524,#33525,#33526,#33527,#33528,#33529,
#33530,#33531,#33532,#33533,#33534),(#33535,#33536,#33537,#33538,#33539,
#33540,#33541,#33542,#33543,#33544,#33545,#33546),(#33547,#33548,#33549,
#33550,#33551,#33552,#33553,#33554,#33555,#33556,#33557,#33558),(#33559,
#33560,#33561,#33562,#33563,#33564,#33565,#33566,#33567,#33568,#33569,#33570)),
 .UNSPECIFIED.,.F.,.F.,.F.)
B_SPLINE_SURFACE_WITH_KNOTS((4,4),(4,2,2,2,2,4),(0.,1.),(0.,0.078369835250435,
0.308777376437327,0.539184917624883,0.769592458812442,1.),.UNSPECIFIED.)
GEOMETRIC_REPRESENTATION_ITEM()
RATIONAL_B_SPLINE_SURFACE(((1.,1.,1.,1.,1.,1.,1.,1.,1.,1.,1.,1.),(0.987189825241073,
0.987189825241073,0.987189825241073,0.987189825241073,0.987189825241073,
0.987189825241073,0.987189825241073,0.987189825241073,0.987189825241073,
0.987189825241073,0.987189825241073,0.987189825241073),(0.987189825241073,
0.987189825241073,0.987189825241073,0.987189825241073,0.987189825241073,
0.987189825241073,0.987189825241073,0.987189825241073,0.987189825241073,
0.987189825241073,0.987189825241073,0.987189825241073),(1.,1.,1.,1.,1.,
1.,1.,1.,1.,1.,1.,1.)))
REPRESENTATION_ITEM('')
SURFACE()
);
#526=(
BOUNDED_SURFACE()
B_SPLINE_SURFACE(3,3,((#33571,#33572,#33573,#33574,#33575,#33576,#33577,
#33578,#33579,#33580,#33581,#33582),(#33583,#33584,#33585,#33586,#33587,
#33588,#33589,#33590,#33591,#33592,#33593,#33594),(#33595,#33596,#33597,
#33598,#33599,#33600,#33601,#33602,#33603,#33604,#33605,#33606),(#33607,
#33608,#33609,#33610,#33611,#33612,#33613,#33614,#33615,#33616,#33617,#33618)),
 .UNSPECIFIED.,.F.,.F.,.F.)
B_SPLINE_SURFACE_WITH_KNOTS((4,4),(4,2,2,2,2,4),(0.,1.),(0.,0.0783698293107414,
0.308777371982556,0.539184914655036,0.769592457327518,1.),.UNSPECIFIED.)
GEOMETRIC_REPRESENTATION_ITEM()
RATIONAL_B_SPLINE_SURFACE(((1.,1.,1.,1.,1.,1.,1.,1.,1.,1.,1.,1.),(0.833333333333332,
0.833333333333332,0.833333333333332,0.833333333333332,0.833333333333332,
0.833333333333332,0.833333333333332,0.833333333333332,0.833333333333332,
0.833333333333332,0.833333333333332,0.833333333333332),(0.833333333333332,
0.833333333333332,0.833333333333332,0.833333333333332,0.833333333333332,
0.833333333333332,0.833333333333332,0.833333333333332,0.833333333333332,
0.833333333333332,0.833333333333332,0.833333333333332),(1.,1.,1.,1.,1.,
1.,1.,1.,1.,1.,1.,1.)))
REPRESENTATION_ITEM('')
SURFACE()
);
#527=(
BOUNDED_SURFACE()
B_SPLINE_SURFACE(3,3,((#33635,#33636,#33637,#33638,#33639,#33640,#33641,
#33642,#33643,#33644,#33645,#33646),(#33647,#33648,#33649,#33650,#33651,
#33652,#33653,#33654,#33655,#33656,#33657,#33658),(#33659,#33660,#33661,
#33662,#33663,#33664,#33665,#33666,#33667,#33668,#33669,#33670),(#33671,
#33672,#33673,#33674,#33675,#33676,#33677,#33678,#33679,#33680,#33681,#33682)),
 .UNSPECIFIED.,.F.,.F.,.F.)
B_SPLINE_SURFACE_WITH_KNOTS((4,4),(4,2,2,2,2,4),(0.,1.),(0.,0.0783698293107414,
0.308777371982556,0.539184914655036,0.769592457327518,1.),.UNSPECIFIED.)
GEOMETRIC_REPRESENTATION_ITEM()
RATIONAL_B_SPLINE_SURFACE(((1.,1.,1.,1.,1.,1.,1.,1.,1.,1.,1.,1.),(0.987189825241073,
0.987189825241073,0.987189825241073,0.987189825241073,0.987189825241073,
0.987189825241073,0.987189825241073,0.987189825241073,0.987189825241073,
0.987189825241073,0.987189825241073,0.987189825241073),(0.987189825241073,
0.987189825241073,0.987189825241073,0.987189825241073,0.987189825241073,
0.987189825241073,0.987189825241073,0.987189825241073,0.987189825241073,
0.987189825241073,0.987189825241073,0.987189825241073),(1.,1.,1.,1.,1.,
1.,1.,1.,1.,1.,1.,1.)))
REPRESENTATION_ITEM('')
SURFACE()
);
#528=(
BOUNDED_SURFACE()
B_SPLINE_SURFACE(3,3,((#33683,#33684,#33685,#33686,#33687,#33688,#33689,
#33690,#33691,#33692,#33693,#33694),(#33695,#33696,#33697,#33698,#33699,
#33700,#33701,#33702,#33703,#33704,#33705,#33706),(#33707,#33708,#33709,
#33710,#33711,#33712,#33713,#33714,#33715,#33716,#33717,#33718),(#33719,
#33720,#33721,#33722,#33723,#33724,#33725,#33726,#33727,#33728,#33729,#33730)),
 .UNSPECIFIED.,.F.,.F.,.F.)
B_SPLINE_SURFACE_WITH_KNOTS((4,4),(4,2,2,2,2,4),(0.,1.),(0.,0.0783698293107414,
0.308777371982556,0.539184914655036,0.769592457327518,1.),.UNSPECIFIED.)
GEOMETRIC_REPRESENTATION_ITEM()
RATIONAL_B_SPLINE_SURFACE(((1.,1.,1.,1.,1.,1.,1.,1.,1.,1.,1.,1.),(0.987189825241073,
0.987189825241073,0.987189825241073,0.987189825241073,0.987189825241073,
0.987189825241073,0.987189825241073,0.987189825241073,0.987189825241073,
0.987189825241073,0.987189825241073,0.987189825241073),(0.987189825241073,
0.987189825241073,0.987189825241073,0.987189825241073,0.987189825241073,
0.987189825241073,0.987189825241073,0.987189825241073,0.987189825241073,
0.987189825241073,0.987189825241073,0.987189825241073),(1.,1.,1.,1.,1.,
1.,1.,1.,1.,1.,1.,1.)))
REPRESENTATION_ITEM('')
SURFACE()
);
#529=(
BOUNDED_SURFACE()
B_SPLINE_SURFACE(3,3,((#33731,#33732,#33733,#33734,#33735,#33736,#33737,
#33738,#33739,#33740,#33741,#33742),(#33743,#33744,#33745,#33746,#33747,
#33748,#33749,#33750,#33751,#33752,#33753,#33754),(#33755,#33756,#33757,
#33758,#33759,#33760,#33761,#33762,#33763,#33764,#33765,#33766),(#33767,
#33768,#33769,#33770,#33771,#33772,#33773,#33774,#33775,#33776,#33777,#33778)),
 .UNSPECIFIED.,.F.,.F.,.F.)
B_SPLINE_SURFACE_WITH_KNOTS((4,4),(4,2,2,2,2,4),(0.,1.),(0.,0.0783698352504223,
0.308777376437317,0.539184917624877,0.769592458812438,1.),.UNSPECIFIED.)
GEOMETRIC_REPRESENTATION_ITEM()
RATIONAL_B_SPLINE_SURFACE(((1.,1.,1.,1.,1.,1.,1.,1.,1.,1.,1.,1.),(0.833333333333332,
0.833333333333332,0.833333333333332,0.833333333333332,0.833333333333332,
0.833333333333332,0.833333333333332,0.833333333333332,0.833333333333332,
0.833333333333332,0.833333333333332,0.833333333333332),(0.833333333333332,
0.833333333333332,0.833333333333332,0.833333333333332,0.833333333333332,
0.833333333333332,0.833333333333332,0.833333333333332,0.833333333333332,
0.833333333333332,0.833333333333332,0.833333333333332),(1.,1.,1.,1.,1.,
1.,1.,1.,1.,1.,1.,1.)))
REPRESENTATION_ITEM('')
SURFACE()
);
#530=(
BOUNDED_SURFACE()
B_SPLINE_SURFACE(3,3,((#33795,#33796,#33797,#33798,#33799,#33800,#33801,
#33802,#33803,#33804,#33805,#33806),(#33807,#33808,#33809,#33810,#33811,
#33812,#33813,#33814,#33815,#33816,#33817,#33818),(#33819,#33820,#33821,
#33822,#33823,#33824,#33825,#33826,#33827,#33828,#33829,#33830),(#33831,
#33832,#33833,#33834,#33835,#33836,#33837,#33838,#33839,#33840,#33841,#33842)),
 .UNSPECIFIED.,.F.,.F.,.F.)
B_SPLINE_SURFACE_WITH_KNOTS((4,4),(4,2,2,2,2,4),(0.,1.),(0.,0.0783698352504223,
0.308777376437317,0.539184917624877,0.769592458812438,1.),.UNSPECIFIED.)
GEOMETRIC_REPRESENTATION_ITEM()
RATIONAL_B_SPLINE_SURFACE(((1.,1.,1.,1.,1.,1.,1.,1.,1.,1.,1.,1.),(0.987189825241073,
0.987189825241073,0.987189825241073,0.987189825241073,0.987189825241073,
0.987189825241073,0.987189825241073,0.987189825241073,0.987189825241073,
0.987189825241073,0.987189825241073,0.987189825241073),(0.987189825241073,
0.987189825241073,0.987189825241073,0.987189825241073,0.987189825241073,
0.987189825241073,0.987189825241073,0.987189825241073,0.987189825241073,
0.987189825241073,0.987189825241073,0.987189825241073),(1.,1.,1.,1.,1.,
1.,1.,1.,1.,1.,1.,1.)))
REPRESENTATION_ITEM('')
SURFACE()
);
#531=(
BOUNDED_SURFACE()
B_SPLINE_SURFACE(3,3,((#33843,#33844,#33845,#33846,#33847,#33848,#33849,
#33850,#33851,#33852,#33853,#33854),(#33855,#33856,#33857,#33858,#33859,
#33860,#33861,#33862,#33863,#33864,#33865,#33866),(#33867,#33868,#33869,
#33870,#33871,#33872,#33873,#33874,#33875,#33876,#33877,#33878),(#33879,
#33880,#33881,#33882,#33883,#33884,#33885,#33886,#33887,#33888,#33889,#33890)),
 .UNSPECIFIED.,.F.,.F.,.F.)
B_SPLINE_SURFACE_WITH_KNOTS((4,4),(4,2,2,2,2,4),(0.,1.),(0.,0.0783698352504223,
0.308777376437317,0.539184917624877,0.769592458812438,1.),.UNSPECIFIED.)
GEOMETRIC_REPRESENTATION_ITEM()
RATIONAL_B_SPLINE_SURFACE(((1.,1.,1.,1.,1.,1.,1.,1.,1.,1.,1.,1.),(0.987189825241073,
0.987189825241073,0.987189825241073,0.987189825241073,0.987189825241073,
0.987189825241073,0.987189825241073,0.987189825241073,0.987189825241073,
0.987189825241073,0.987189825241073,0.987189825241073),(0.987189825241073,
0.987189825241073,0.987189825241073,0.987189825241073,0.987189825241073,
0.987189825241073,0.987189825241073,0.987189825241073,0.987189825241073,
0.987189825241073,0.987189825241073,0.987189825241073),(1.,1.,1.,1.,1.,
1.,1.,1.,1.,1.,1.,1.)))
REPRESENTATION_ITEM('')
SURFACE()
);
#532=(
BOUNDED_SURFACE()
B_SPLINE_SURFACE(3,3,((#33891,#33892,#33893,#33894,#33895,#33896,#33897,
#33898,#33899,#33900,#33901,#33902),(#33903,#33904,#33905,#33906,#33907,
#33908,#33909,#33910,#33911,#33912,#33913,#33914),(#33915,#33916,#33917,
#33918,#33919,#33920,#33921,#33922,#33923,#33924,#33925,#33926),(#33927,
#33928,#33929,#33930,#33931,#33932,#33933,#33934,#33935,#33936,#33937,#33938)),
 .UNSPECIFIED.,.F.,.F.,.F.)
B_SPLINE_SURFACE_WITH_KNOTS((4,4),(4,2,2,2,2,4),(0.,1.),(0.,0.0783698388401235,
0.308777379129593,0.539184919419728,0.769592459709863,1.),.UNSPECIFIED.)
GEOMETRIC_REPRESENTATION_ITEM()
RATIONAL_B_SPLINE_SURFACE(((1.,1.,1.,1.,1.,1.,1.,1.,1.,1.,1.,1.),(0.833333333333332,
0.833333333333332,0.833333333333332,0.833333333333332,0.833333333333332,
0.833333333333332,0.833333333333332,0.833333333333332,0.833333333333332,
0.833333333333332,0.833333333333332,0.833333333333332),(0.833333333333332,
0.833333333333332,0.833333333333332,0.833333333333332,0.833333333333332,
0.833333333333332,0.833333333333332,0.833333333333332,0.833333333333332,
0.833333333333332,0.833333333333332,0.833333333333332),(1.,1.,1.,1.,1.,
1.,1.,1.,1.,1.,1.,1.)))
REPRESENTATION_ITEM('')
SURFACE()
);
#533=(
BOUNDED_SURFACE()
B_SPLINE_SURFACE(3,3,((#33955,#33956,#33957,#33958,#33959,#33960,#33961,
#33962,#33963,#33964,#33965,#33966),(#33967,#33968,#33969,#33970,#33971,
#33972,#33973,#33974,#33975,#33976,#33977,#33978),(#33979,#33980,#33981,
#33982,#33983,#33984,#33985,#33986,#33987,#33988,#33989,#33990),(#33991,
#33992,#33993,#33994,#33995,#33996,#33997,#33998,#33999,#34000,#34001,#34002)),
 .UNSPECIFIED.,.F.,.F.,.F.)
B_SPLINE_SURFACE_WITH_KNOTS((4,4),(4,2,2,2,2,4),(0.,1.),(0.,0.0783698388401235,
0.308777379129593,0.539184919419728,0.769592459709863,1.),.UNSPECIFIED.)
GEOMETRIC_REPRESENTATION_ITEM()
RATIONAL_B_SPLINE_SURFACE(((1.,1.,1.,1.,1.,1.,1.,1.,1.,1.,1.,1.),(0.987189825241073,
0.987189825241073,0.987189825241073,0.987189825241073,0.987189825241073,
0.987189825241073,0.987189825241073,0.987189825241073,0.987189825241073,
0.987189825241073,0.987189825241073,0.987189825241073),(0.987189825241073,
0.987189825241073,0.987189825241073,0.987189825241073,0.987189825241073,
0.987189825241073,0.987189825241073,0.987189825241073,0.987189825241073,
0.987189825241073,0.987189825241073,0.987189825241073),(1.,1.,1.,1.,1.,
1.,1.,1.,1.,1.,1.,1.)))
REPRESENTATION_ITEM('')
SURFACE()
);
#534=(
BOUNDED_SURFACE()
B_SPLINE_SURFACE(3,3,((#34003,#34004,#34005,#34006,#34007,#34008,#34009,
#34010,#34011,#34012,#34013,#34014),(#34015,#34016,#34017,#34018,#34019,
#34020,#34021,#34022,#34023,#34024,#34025,#34026),(#34027,#34028,#34029,
#34030,#34031,#34032,#34033,#34034,#34035,#34036,#34037,#34038),(#34039,
#34040,#34041,#34042,#34043,#34044,#34045,#34046,#34047,#34048,#34049,#34050)),
 .UNSPECIFIED.,.F.,.F.,.F.)
B_SPLINE_SURFACE_WITH_KNOTS((4,4),(4,2,2,2,2,4),(0.,1.),(0.,0.0783698388401235,
0.308777379129593,0.539184919419728,0.769592459709863,1.),.UNSPECIFIED.)
GEOMETRIC_REPRESENTATION_ITEM()
RATIONAL_B_SPLINE_SURFACE(((1.,1.,1.,1.,1.,1.,1.,1.,1.,1.,1.,1.),(0.987189825241073,
0.987189825241073,0.987189825241073,0.987189825241073,0.987189825241073,
0.987189825241073,0.987189825241073,0.987189825241073,0.987189825241073,
0.987189825241073,0.987189825241073,0.987189825241073),(0.987189825241073,
0.987189825241073,0.987189825241073,0.987189825241073,0.987189825241073,
0.987189825241073,0.987189825241073,0.987189825241073,0.987189825241073,
0.987189825241073,0.987189825241073,0.987189825241073),(1.,1.,1.,1.,1.,
1.,1.,1.,1.,1.,1.,1.)))
REPRESENTATION_ITEM('')
SURFACE()
);
#535=(
BOUNDED_SURFACE()
B_SPLINE_SURFACE(3,3,((#34051,#34052,#34053,#34054,#34055,#34056,#34057,
#34058,#34059,#34060,#34061,#34062,#34063,#34064),(#34065,#34066,#34067,
#34068,#34069,#34070,#34071,#34072,#34073,#34074,#34075,#34076,#34077,#34078),
(#34079,#34080,#34081,#34082,#34083,#34084,#34085,#34086,#34087,#34088,
#34089,#34090,#34091,#34092),(#34093,#34094,#34095,#34096,#34097,#34098,
#34099,#34100,#34101,#34102,#34103,#34104,#34105,#34106)),.UNSPECIFIED.,
 .F.,.F.,.F.)
B_SPLINE_SURFACE_WITH_KNOTS((4,4),(4,2,2,2,2,2,4),(0.,1.),(0.,0.0183879322611598,
0.0783698437311081,0.308777382797832,0.53918492186522,0.76959246093261,
1.),.UNSPECIFIED.)
GEOMETRIC_REPRESENTATION_ITEM()
RATIONAL_B_SPLINE_SURFACE(((1.,1.,1.,1.,1.,1.,1.,1.,1.,1.,1.,1.,1.,1.),
(0.833333333333332,0.833333333333332,0.833333333333332,0.833333333333332,
0.833333333333332,0.833333333333332,0.833333333333332,0.833333333333332,
0.833333333333332,0.833333333333332,0.833333333333332,0.833333333333332,
0.833333333333332,0.833333333333332),(0.833333333333332,0.833333333333332,
0.833333333333332,0.833333333333332,0.833333333333332,0.833333333333332,
0.833333333333332,0.833333333333332,0.833333333333332,0.833333333333332,
0.833333333333332,0.833333333333332,0.833333333333332,0.833333333333332),
(1.,1.,1.,1.,1.,1.,1.,1.,1.,1.,1.,1.,1.,1.)))
REPRESENTATION_ITEM('')
SURFACE()
);
#536=(
BOUNDED_SURFACE()
B_SPLINE_SURFACE(3,3,((#34125,#34126,#34127,#34128,#34129,#34130,#34131,
#34132,#34133,#34134,#34135,#34136,#34137,#34138),(#34139,#34140,#34141,
#34142,#34143,#34144,#34145,#34146,#34147,#34148,#34149,#34150,#34151,#34152),
(#34153,#34154,#34155,#34156,#34157,#34158,#34159,#34160,#34161,#34162,
#34163,#34164,#34165,#34166),(#34167,#34168,#34169,#34170,#34171,#34172,
#34173,#34174,#34175,#34176,#34177,#34178,#34179,#34180)),.UNSPECIFIED.,
 .F.,.F.,.F.)
B_SPLINE_SURFACE_WITH_KNOTS((4,4),(4,2,2,2,2,2,4),(0.,1.),(0.,0.0183879322611598,
0.0783698437311081,0.308777382797832,0.53918492186522,0.76959246093261,
1.),.UNSPECIFIED.)
GEOMETRIC_REPRESENTATION_ITEM()
RATIONAL_B_SPLINE_SURFACE(((1.,1.,1.,1.,1.,1.,1.,1.,1.,1.,1.,1.,1.,1.),
(0.987189825241073,0.987189825241073,0.987189825241073,0.987189825241073,
0.987189825241073,0.987189825241073,0.987189825241073,0.987189825241073,
0.987189825241073,0.987189825241073,0.987189825241073,0.987189825241073,
0.987189825241073,0.987189825241073),(0.987189825241073,0.987189825241073,
0.987189825241073,0.987189825241073,0.987189825241073,0.987189825241073,
0.987189825241073,0.987189825241073,0.987189825241073,0.987189825241073,
0.987189825241073,0.987189825241073,0.987189825241073,0.987189825241073),
(1.,1.,1.,1.,1.,1.,1.,1.,1.,1.,1.,1.,1.,1.)))
REPRESENTATION_ITEM('')
SURFACE()
);
#537=(
BOUNDED_SURFACE()
B_SPLINE_SURFACE(3,3,((#34181,#34182,#34183,#34184,#34185,#34186,#34187,
#34188,#34189,#34190,#34191,#34192,#34193,#34194),(#34195,#34196,#34197,
#34198,#34199,#34200,#34201,#34202,#34203,#34204,#34205,#34206,#34207,#34208),
(#34209,#34210,#34211,#34212,#34213,#34214,#34215,#34216,#34217,#34218,
#34219,#34220,#34221,#34222),(#34223,#34224,#34225,#34226,#34227,#34228,
#34229,#34230,#34231,#34232,#34233,#34234,#34235,#34236)),.UNSPECIFIED.,
 .F.,.F.,.F.)
B_SPLINE_SURFACE_WITH_KNOTS((4,4),(4,2,2,2,2,2,4),(0.,1.),(0.,0.0183879322611598,
0.0783698437311081,0.308777382797832,0.53918492186522,0.76959246093261,
1.),.UNSPECIFIED.)
GEOMETRIC_REPRESENTATION_ITEM()
RATIONAL_B_SPLINE_SURFACE(((1.,1.,1.,1.,1.,1.,1.,1.,1.,1.,1.,1.,1.,1.),
(0.987189825241073,0.987189825241073,0.987189825241073,0.987189825241073,
0.987189825241073,0.987189825241073,0.987189825241073,0.987189825241073,
0.987189825241073,0.987189825241073,0.987189825241073,0.987189825241073,
0.987189825241073,0.987189825241073),(0.987189825241073,0.987189825241073,
0.987189825241073,0.987189825241073,0.987189825241073,0.987189825241073,
0.987189825241073,0.987189825241073,0.987189825241073,0.987189825241073,
0.987189825241073,0.987189825241073,0.987189825241073,0.987189825241073),
(1.,1.,1.,1.,1.,1.,1.,1.,1.,1.,1.,1.,1.,1.)))
REPRESENTATION_ITEM('')
SURFACE()
);
#538=(
BOUNDED_SURFACE()
B_SPLINE_SURFACE(3,3,((#34237,#34238,#34239,#34240,#34241,#34242,#34243,
#34244,#34245,#34246,#34247,#34248,#34249,#34250),(#34251,#34252,#34253,
#34254,#34255,#34256,#34257,#34258,#34259,#34260,#34261,#34262,#34263,#34264),
(#34265,#34266,#34267,#34268,#34269,#34270,#34271,#34272,#34273,#34274,
#34275,#34276,#34277,#34278),(#34279,#34280,#34281,#34282,#34283,#34284,
#34285,#34286,#34287,#34288,#34289,#34290,#34291,#34292)),.UNSPECIFIED.,
 .F.,.F.,.F.)
B_SPLINE_SURFACE_WITH_KNOTS((4,4),(4,2,2,2,2,2,4),(0.,1.),(0.,0.0183879369801425,
0.078369848160917,0.308777386120188,0.539184924080124,0.769592462040062,
1.),.UNSPECIFIED.)
GEOMETRIC_REPRESENTATION_ITEM()
RATIONAL_B_SPLINE_SURFACE(((1.,1.,1.,1.,1.,1.,1.,1.,1.,1.,1.,1.,1.,1.),
(0.833333333333333,0.833333333333333,0.833333333333333,0.833333333333333,
0.833333333333333,0.833333333333333,0.833333333333333,0.833333333333333,
0.833333333333333,0.833333333333333,0.833333333333333,0.833333333333333,
0.833333333333333,0.833333333333333),(0.833333333333333,0.833333333333333,
0.833333333333333,0.833333333333333,0.833333333333333,0.833333333333333,
0.833333333333333,0.833333333333333,0.833333333333333,0.833333333333333,
0.833333333333333,0.833333333333333,0.833333333333333,0.833333333333333),
(1.,1.,1.,1.,1.,1.,1.,1.,1.,1.,1.,1.,1.,1.)))
REPRESENTATION_ITEM('')
SURFACE()
);
#539=(
BOUNDED_SURFACE()
B_SPLINE_SURFACE(3,3,((#34311,#34312,#34313,#34314,#34315,#34316,#34317,
#34318,#34319,#34320,#34321,#34322,#34323,#34324),(#34325,#34326,#34327,
#34328,#34329,#34330,#34331,#34332,#34333,#34334,#34335,#34336,#34337,#34338),
(#34339,#34340,#34341,#34342,#34343,#34344,#34345,#34346,#34347,#34348,
#34349,#34350,#34351,#34352),(#34353,#34354,#34355,#34356,#34357,#34358,
#34359,#34360,#34361,#34362,#34363,#34364,#34365,#34366)),.UNSPECIFIED.,
 .F.,.F.,.F.)
B_SPLINE_SURFACE_WITH_KNOTS((4,4),(4,2,2,2,2,2,4),(0.,1.),(0.,0.0183879369801425,
0.078369848160917,0.308777386120188,0.539184924080124,0.769592462040062,
1.),.UNSPECIFIED.)
GEOMETRIC_REPRESENTATION_ITEM()
RATIONAL_B_SPLINE_SURFACE(((1.,1.,1.,1.,1.,1.,1.,1.,1.,1.,1.,1.,1.,1.),
(0.987189825241073,0.987189825241073,0.987189825241073,0.987189825241073,
0.987189825241073,0.987189825241073,0.987189825241073,0.987189825241073,
0.987189825241073,0.987189825241073,0.987189825241073,0.987189825241073,
0.987189825241073,0.987189825241073),(0.987189825241073,0.987189825241073,
0.987189825241073,0.987189825241073,0.987189825241073,0.987189825241073,
0.987189825241073,0.987189825241073,0.987189825241073,0.987189825241073,
0.987189825241073,0.987189825241073,0.987189825241073,0.987189825241073),
(1.,1.,1.,1.,1.,1.,1.,1.,1.,1.,1.,1.,1.,1.)))
REPRESENTATION_ITEM('')
SURFACE()
);
#540=(
BOUNDED_SURFACE()
B_SPLINE_SURFACE(3,3,((#34367,#34368,#34369,#34370,#34371,#34372,#34373,
#34374,#34375,#34376,#34377,#34378,#34379,#34380),(#34381,#34382,#34383,
#34384,#34385,#34386,#34387,#34388,#34389,#34390,#34391,#34392,#34393,#34394),
(#34395,#34396,#34397,#34398,#34399,#34400,#34401,#34402,#34403,#34404,
#34405,#34406,#34407,#34408),(#34409,#34410,#34411,#34412,#34413,#34414,
#34415,#34416,#34417,#34418,#34419,#34420,#34421,#34422)),.UNSPECIFIED.,
 .F.,.F.,.F.)
B_SPLINE_SURFACE_WITH_KNOTS((4,4),(4,2,2,2,2,2,4),(0.,1.),(0.,0.0183879369801425,
0.078369848160917,0.308777386120188,0.539184924080124,0.769592462040062,
1.),.UNSPECIFIED.)
GEOMETRIC_REPRESENTATION_ITEM()
RATIONAL_B_SPLINE_SURFACE(((1.,1.,1.,1.,1.,1.,1.,1.,1.,1.,1.,1.,1.,1.),
(0.987189825241073,0.987189825241073,0.987189825241073,0.987189825241073,
0.987189825241073,0.987189825241073,0.987189825241073,0.987189825241073,
0.987189825241073,0.987189825241073,0.987189825241073,0.987189825241073,
0.987189825241073,0.987189825241073),(0.987189825241073,0.987189825241073,
0.987189825241073,0.987189825241073,0.987189825241073,0.987189825241073,
0.987189825241073,0.987189825241073,0.987189825241073,0.987189825241073,
0.987189825241073,0.987189825241073,0.987189825241073,0.987189825241073),
(1.,1.,1.,1.,1.,1.,1.,1.,1.,1.,1.,1.,1.,1.)))
REPRESENTATION_ITEM('')
SURFACE()
);
#541=(
BOUNDED_SURFACE()
B_SPLINE_SURFACE(3,3,((#34423,#34424,#34425,#34426,#34427,#34428,#34429,
#34430,#34431,#34432,#34433,#34434),(#34435,#34436,#34437,#34438,#34439,
#34440,#34441,#34442,#34443,#34444,#34445,#34446),(#34447,#34448,#34449,
#34450,#34451,#34452,#34453,#34454,#34455,#34456,#34457,#34458),(#34459,
#34460,#34461,#34462,#34463,#34464,#34465,#34466,#34467,#34468,#34469,#34470)),
 .UNSPECIFIED.,.F.,.F.,.F.)
B_SPLINE_SURFACE_WITH_KNOTS((4,4),(4,2,2,2,2,4),(0.,1.),(0.,0.0783698504850856,
0.308777387863315,0.539184925242209,0.769592462621105,1.),.UNSPECIFIED.)
GEOMETRIC_REPRESENTATION_ITEM()
RATIONAL_B_SPLINE_SURFACE(((1.,1.,1.,1.,1.,1.,1.,1.,1.,1.,1.,1.),(0.833333333333333,
0.833333333333333,0.833333333333333,0.833333333333333,0.833333333333333,
0.833333333333333,0.833333333333333,0.833333333333333,0.833333333333333,
0.833333333333333,0.833333333333333,0.833333333333333),(0.833333333333333,
0.833333333333333,0.833333333333333,0.833333333333333,0.833333333333333,
0.833333333333333,0.833333333333333,0.833333333333333,0.833333333333333,
0.833333333333333,0.833333333333333,0.833333333333333),(1.,1.,1.,1.,1.,
1.,1.,1.,1.,1.,1.,1.)))
REPRESENTATION_ITEM('')
SURFACE()
);
#542=(
BOUNDED_SURFACE()
B_SPLINE_SURFACE(3,3,((#34487,#34488,#34489,#34490,#34491,#34492,#34493,
#34494,#34495,#34496,#34497,#34498),(#34499,#34500,#34501,#34502,#34503,
#34504,#34505,#34506,#34507,#34508,#34509,#34510),(#34511,#34512,#34513,
#34514,#34515,#34516,#34517,#34518,#34519,#34520,#34521,#34522),(#34523,
#34524,#34525,#34526,#34527,#34528,#34529,#34530,#34531,#34532,#34533,#34534)),
 .UNSPECIFIED.,.F.,.F.,.F.)
B_SPLINE_SURFACE_WITH_KNOTS((4,4),(4,2,2,2,2,4),(0.,1.),(0.,0.0783698504850856,
0.308777387863315,0.539184925242209,0.769592462621105,1.),.UNSPECIFIED.)
GEOMETRIC_REPRESENTATION_ITEM()
RATIONAL_B_SPLINE_SURFACE(((1.,1.,1.,1.,1.,1.,1.,1.,1.,1.,1.,1.),(0.987189825241073,
0.987189825241073,0.987189825241073,0.987189825241073,0.987189825241073,
0.987189825241073,0.987189825241073,0.987189825241073,0.987189825241073,
0.987189825241073,0.987189825241073,0.987189825241073),(0.987189825241073,
0.987189825241073,0.987189825241073,0.987189825241073,0.987189825241073,
0.987189825241073,0.987189825241073,0.987189825241073,0.987189825241073,
0.987189825241073,0.987189825241073,0.987189825241073),(1.,1.,1.,1.,1.,
1.,1.,1.,1.,1.,1.,1.)))
REPRESENTATION_ITEM('')
SURFACE()
);
#543=(
BOUNDED_SURFACE()
B_SPLINE_SURFACE(3,3,((#34535,#34536,#34537,#34538,#34539,#34540,#34541,
#34542,#34543,#34544,#34545,#34546),(#34547,#34548,#34549,#34550,#34551,
#34552,#34553,#34554,#34555,#34556,#34557,#34558),(#34559,#34560,#34561,
#34562,#34563,#34564,#34565,#34566,#34567,#34568,#34569,#34570),(#34571,
#34572,#34573,#34574,#34575,#34576,#34577,#34578,#34579,#34580,#34581,#34582)),
 .UNSPECIFIED.,.F.,.F.,.F.)
B_SPLINE_SURFACE_WITH_KNOTS((4,4),(4,2,2,2,2,4),(0.,1.),(0.,0.0783698504850856,
0.308777387863315,0.539184925242209,0.769592462621105,1.),.UNSPECIFIED.)
GEOMETRIC_REPRESENTATION_ITEM()
RATIONAL_B_SPLINE_SURFACE(((1.,1.,1.,1.,1.,1.,1.,1.,1.,1.,1.,1.),(0.987189825241073,
0.987189825241073,0.987189825241073,0.987189825241073,0.987189825241073,
0.987189825241073,0.987189825241073,0.987189825241073,0.987189825241073,
0.987189825241073,0.987189825241073,0.987189825241073),(0.987189825241073,
0.987189825241073,0.987189825241073,0.987189825241073,0.987189825241073,
0.987189825241073,0.987189825241073,0.987189825241073,0.987189825241073,
0.987189825241073,0.987189825241073,0.987189825241073),(1.,1.,1.,1.,1.,
1.,1.,1.,1.,1.,1.,1.)))
REPRESENTATION_ITEM('')
SURFACE()
);
#544=(
BOUNDED_SURFACE()
B_SPLINE_SURFACE(3,3,((#34583,#34584,#34585,#34586,#34587,#34588,#34589,
#34590,#34591,#34592,#34593,#34594),(#34595,#34596,#34597,#34598,#34599,
#34600,#34601,#34602,#34603,#34604,#34605,#34606),(#34607,#34608,#34609,
#34610,#34611,#34612,#34613,#34614,#34615,#34616,#34617,#34618),(#34619,
#34620,#34621,#34622,#34623,#34624,#34625,#34626,#34627,#34628,#34629,#34630)),
 .UNSPECIFIED.,.F.,.F.,.F.)
B_SPLINE_SURFACE_WITH_KNOTS((4,4),(4,2,2,2,2,4),(0.,1.),(0.,0.0783698504851055,
0.30877738786333,0.539184925242219,0.769592462621109,1.),.UNSPECIFIED.)
GEOMETRIC_REPRESENTATION_ITEM()
RATIONAL_B_SPLINE_SURFACE(((1.,1.,1.,1.,1.,1.,1.,1.,1.,1.,1.,1.),(0.833333333333332,
0.833333333333332,0.833333333333332,0.833333333333332,0.833333333333332,
0.833333333333332,0.833333333333332,0.833333333333332,0.833333333333332,
0.833333333333332,0.833333333333332,0.833333333333332),(0.833333333333332,
0.833333333333332,0.833333333333332,0.833333333333332,0.833333333333332,
0.833333333333332,0.833333333333332,0.833333333333332,0.833333333333332,
0.833333333333332,0.833333333333332,0.833333333333332),(1.,1.,1.,1.,1.,
1.,1.,1.,1.,1.,1.,1.)))
REPRESENTATION_ITEM('')
SURFACE()
);
#545=(
BOUNDED_SURFACE()
B_SPLINE_SURFACE(3,3,((#34647,#34648,#34649,#34650,#34651,#34652,#34653,
#34654,#34655,#34656,#34657,#34658),(#34659,#34660,#34661,#34662,#34663,
#34664,#34665,#34666,#34667,#34668,#34669,#34670),(#34671,#34672,#34673,
#34674,#34675,#34676,#34677,#34678,#34679,#34680,#34681,#34682),(#34683,
#34684,#34685,#34686,#34687,#34688,#34689,#34690,#34691,#34692,#34693,#34694)),
 .UNSPECIFIED.,.F.,.F.,.F.)
B_SPLINE_SURFACE_WITH_KNOTS((4,4),(4,2,2,2,2,4),(0.,1.),(0.,0.0783698504851055,
0.30877738786333,0.539184925242219,0.769592462621109,1.),.UNSPECIFIED.)
GEOMETRIC_REPRESENTATION_ITEM()
RATIONAL_B_SPLINE_SURFACE(((1.,1.,1.,1.,1.,1.,1.,1.,1.,1.,1.,1.),(0.987189825241073,
0.987189825241073,0.987189825241073,0.987189825241073,0.987189825241073,
0.987189825241073,0.987189825241073,0.987189825241073,0.987189825241073,
0.987189825241073,0.987189825241073,0.987189825241073),(0.987189825241073,
0.987189825241073,0.987189825241073,0.987189825241073,0.987189825241073,
0.987189825241073,0.987189825241073,0.987189825241073,0.987189825241073,
0.987189825241073,0.987189825241073,0.987189825241073),(1.,1.,1.,1.,1.,
1.,1.,1.,1.,1.,1.,1.)))
REPRESENTATION_ITEM('')
SURFACE()
);
#546=(
BOUNDED_SURFACE()
B_SPLINE_SURFACE(3,3,((#34695,#34696,#34697,#34698,#34699,#34700,#34701,
#34702,#34703,#34704,#34705,#34706),(#34707,#34708,#34709,#34710,#34711,
#34712,#34713,#34714,#34715,#34716,#34717,#34718),(#34719,#34720,#34721,
#34722,#34723,#34724,#34725,#34726,#34727,#34728,#34729,#34730),(#34731,
#34732,#34733,#34734,#34735,#34736,#34737,#34738,#34739,#34740,#34741,#34742)),
 .UNSPECIFIED.,.F.,.F.,.F.)
B_SPLINE_SURFACE_WITH_KNOTS((4,4),(4,2,2,2,2,4),(0.,1.),(0.,0.0783698504851055,
0.30877738786333,0.539184925242219,0.769592462621109,1.),.UNSPECIFIED.)
GEOMETRIC_REPRESENTATION_ITEM()
RATIONAL_B_SPLINE_SURFACE(((1.,1.,1.,1.,1.,1.,1.,1.,1.,1.,1.,1.),(0.987189825241073,
0.987189825241073,0.987189825241073,0.987189825241073,0.987189825241073,
0.987189825241073,0.987189825241073,0.987189825241073,0.987189825241073,
0.987189825241073,0.987189825241073,0.987189825241073),(0.987189825241073,
0.987189825241073,0.987189825241073,0.987189825241073,0.987189825241073,
0.987189825241073,0.987189825241073,0.987189825241073,0.987189825241073,
0.987189825241073,0.987189825241073,0.987189825241073),(1.,1.,1.,1.,1.,
1.,1.,1.,1.,1.,1.,1.)))
REPRESENTATION_ITEM('')
SURFACE()
);
#547=(
BOUNDED_SURFACE()
B_SPLINE_SURFACE(3,3,((#34743,#34744,#34745,#34746,#34747,#34748,#34749,
#34750,#34751,#34752,#34753,#34754),(#34755,#34756,#34757,#34758,#34759,
#34760,#34761,#34762,#34763,#34764,#34765,#34766),(#34767,#34768,#34769,
#34770,#34771,#34772,#34773,#34774,#34775,#34776,#34777,#34778),(#34779,
#34780,#34781,#34782,#34783,#34784,#34785,#34786,#34787,#34788,#34789,#34790)),
 .UNSPECIFIED.,.F.,.F.,.F.)
B_SPLINE_SURFACE_WITH_KNOTS((4,4),(4,2,2,2,2,4),(0.,1.),(0.,0.0783698481609002,
0.308777386120176,0.539184924080116,0.769592462040058,1.),.UNSPECIFIED.)
GEOMETRIC_REPRESENTATION_ITEM()
RATIONAL_B_SPLINE_SURFACE(((1.,1.,1.,1.,1.,1.,1.,1.,1.,1.,1.,1.),(0.833333333333333,
0.833333333333333,0.833333333333333,0.833333333333333,0.833333333333333,
0.833333333333333,0.833333333333333,0.833333333333333,0.833333333333333,
0.833333333333333,0.833333333333333,0.833333333333333),(0.833333333333333,
0.833333333333333,0.833333333333333,0.833333333333333,0.833333333333333,
0.833333333333333,0.833333333333333,0.833333333333333,0.833333333333333,
0.833333333333333,0.833333333333333,0.833333333333333),(1.,1.,1.,1.,1.,
1.,1.,1.,1.,1.,1.,1.)))
REPRESENTATION_ITEM('')
SURFACE()
);
#548=(
BOUNDED_SURFACE()
B_SPLINE_SURFACE(3,3,((#34807,#34808,#34809,#34810,#34811,#34812,#34813,
#34814,#34815,#34816,#34817,#34818),(#34819,#34820,#34821,#34822,#34823,
#34824,#34825,#34826,#34827,#34828,#34829,#34830),(#34831,#34832,#34833,
#34834,#34835,#34836,#34837,#34838,#34839,#34840,#34841,#34842),(#34843,
#34844,#34845,#34846,#34847,#34848,#34849,#34850,#34851,#34852,#34853,#34854)),
 .UNSPECIFIED.,.F.,.F.,.F.)
B_SPLINE_SURFACE_WITH_KNOTS((4,4),(4,2,2,2,2,4),(0.,1.),(0.,0.0783698481609002,
0.308777386120176,0.539184924080116,0.769592462040058,1.),.UNSPECIFIED.)
GEOMETRIC_REPRESENTATION_ITEM()
RATIONAL_B_SPLINE_SURFACE(((1.,1.,1.,1.,1.,1.,1.,1.,1.,1.,1.,1.),(0.987189825241073,
0.987189825241073,0.987189825241073,0.987189825241073,0.987189825241073,
0.987189825241073,0.987189825241073,0.987189825241073,0.987189825241073,
0.987189825241073,0.987189825241073,0.987189825241073),(0.987189825241073,
0.987189825241073,0.987189825241073,0.987189825241073,0.987189825241073,
0.987189825241073,0.987189825241073,0.987189825241073,0.987189825241073,
0.987189825241073,0.987189825241073,0.987189825241073),(1.,1.,1.,1.,1.,
1.,1.,1.,1.,1.,1.,1.)))
REPRESENTATION_ITEM('')
SURFACE()
);
#549=(
BOUNDED_SURFACE()
B_SPLINE_SURFACE(3,3,((#34855,#34856,#34857,#34858,#34859,#34860,#34861,
#34862,#34863,#34864,#34865,#34866),(#34867,#34868,#34869,#34870,#34871,
#34872,#34873,#34874,#34875,#34876,#34877,#34878),(#34879,#34880,#34881,
#34882,#34883,#34884,#34885,#34886,#34887,#34888,#34889,#34890),(#34891,
#34892,#34893,#34894,#34895,#34896,#34897,#34898,#34899,#34900,#34901,#34902)),
 .UNSPECIFIED.,.F.,.F.,.F.)
B_SPLINE_SURFACE_WITH_KNOTS((4,4),(4,2,2,2,2,4),(0.,1.),(0.,0.0783698481609002,
0.308777386120176,0.539184924080116,0.769592462040058,1.),.UNSPECIFIED.)
GEOMETRIC_REPRESENTATION_ITEM()
RATIONAL_B_SPLINE_SURFACE(((1.,1.,1.,1.,1.,1.,1.,1.,1.,1.,1.,1.),(0.987189825241073,
0.987189825241073,0.987189825241073,0.987189825241073,0.987189825241073,
0.987189825241073,0.987189825241073,0.987189825241073,0.987189825241073,
0.987189825241073,0.987189825241073,0.987189825241073),(0.987189825241073,
0.987189825241073,0.987189825241073,0.987189825241073,0.987189825241073,
0.987189825241073,0.987189825241073,0.987189825241073,0.987189825241073,
0.987189825241073,0.987189825241073,0.987189825241073),(1.,1.,1.,1.,1.,
1.,1.,1.,1.,1.,1.,1.)))
REPRESENTATION_ITEM('')
SURFACE()
);
#550=(
BOUNDED_SURFACE()
B_SPLINE_SURFACE(3,3,((#34903,#34904,#34905,#34906,#34907,#34908,#34909,
#34910,#34911,#34912,#34913,#34914),(#34915,#34916,#34917,#34918,#34919,
#34920,#34921,#34922,#34923,#34924,#34925,#34926),(#34927,#34928,#34929,
#34930,#34931,#34932,#34933,#34934,#34935,#34936,#34937,#34938),(#34939,
#34940,#34941,#34942,#34943,#34944,#34945,#34946,#34947,#34948,#34949,#34950)),
 .UNSPECIFIED.,.F.,.F.,.F.)
B_SPLINE_SURFACE_WITH_KNOTS((4,4),(4,2,2,2,2,4),(0.,1.),(0.,0.0783698437310988,
0.308777382797825,0.539184921865215,0.769592460932608,1.),.UNSPECIFIED.)
GEOMETRIC_REPRESENTATION_ITEM()
RATIONAL_B_SPLINE_SURFACE(((1.,1.,1.,1.,1.,1.,1.,1.,1.,1.,1.,1.),(0.833333333333332,
0.833333333333332,0.833333333333332,0.833333333333332,0.833333333333332,
0.833333333333332,0.833333333333332,0.833333333333332,0.833333333333332,
0.833333333333332,0.833333333333332,0.833333333333332),(0.833333333333332,
0.833333333333332,0.833333333333332,0.833333333333332,0.833333333333332,
0.833333333333332,0.833333333333332,0.833333333333332,0.833333333333332,
0.833333333333332,0.833333333333332,0.833333333333332),(1.,1.,1.,1.,1.,
1.,1.,1.,1.,1.,1.,1.)))
REPRESENTATION_ITEM('')
SURFACE()
);
#551=(
BOUNDED_SURFACE()
B_SPLINE_SURFACE(3,3,((#34967,#34968,#34969,#34970,#34971,#34972,#34973,
#34974,#34975,#34976,#34977,#34978),(#34979,#34980,#34981,#34982,#34983,
#34984,#34985,#34986,#34987,#34988,#34989,#34990),(#34991,#34992,#34993,
#34994,#34995,#34996,#34997,#34998,#34999,#35000,#35001,#35002),(#35003,
#35004,#35005,#35006,#35007,#35008,#35009,#35010,#35011,#35012,#35013,#35014)),
 .UNSPECIFIED.,.F.,.F.,.F.)
B_SPLINE_SURFACE_WITH_KNOTS((4,4),(4,2,2,2,2,4),(0.,1.),(0.,0.0783698437310988,
0.308777382797825,0.539184921865215,0.769592460932608,1.),.UNSPECIFIED.)
GEOMETRIC_REPRESENTATION_ITEM()
RATIONAL_B_SPLINE_SURFACE(((1.,1.,1.,1.,1.,1.,1.,1.,1.,1.,1.,1.),(0.987189825241073,
0.987189825241073,0.987189825241073,0.987189825241073,0.987189825241073,
0.987189825241073,0.987189825241073,0.987189825241073,0.987189825241073,
0.987189825241073,0.987189825241073,0.987189825241073),(0.987189825241073,
0.987189825241073,0.987189825241073,0.987189825241073,0.987189825241073,
0.987189825241073,0.987189825241073,0.987189825241073,0.987189825241073,
0.987189825241073,0.987189825241073,0.987189825241073),(1.,1.,1.,1.,1.,
1.,1.,1.,1.,1.,1.,1.)))
REPRESENTATION_ITEM('')
SURFACE()
);
#552=(
BOUNDED_SURFACE()
B_SPLINE_SURFACE(3,3,((#35015,#35016,#35017,#35018,#35019,#35020,#35021,
#35022,#35023,#35024,#35025,#35026),(#35027,#35028,#35029,#35030,#35031,
#35032,#35033,#35034,#35035,#35036,#35037,#35038),(#35039,#35040,#35041,
#35042,#35043,#35044,#35045,#35046,#35047,#35048,#35049,#35050),(#35051,
#35052,#35053,#35054,#35055,#35056,#35057,#35058,#35059,#35060,#35061,#35062)),
 .UNSPECIFIED.,.F.,.F.,.F.)
B_SPLINE_SURFACE_WITH_KNOTS((4,4),(4,2,2,2,2,4),(0.,1.),(0.,0.0783698437310988,
0.308777382797825,0.539184921865215,0.769592460932608,1.),.UNSPECIFIED.)
GEOMETRIC_REPRESENTATION_ITEM()
RATIONAL_B_SPLINE_SURFACE(((1.,1.,1.,1.,1.,1.,1.,1.,1.,1.,1.,1.),(0.987189825241073,
0.987189825241073,0.987189825241073,0.987189825241073,0.987189825241073,
0.987189825241073,0.987189825241073,0.987189825241073,0.987189825241073,
0.987189825241073,0.987189825241073,0.987189825241073),(0.987189825241073,
0.987189825241073,0.987189825241073,0.987189825241073,0.987189825241073,
0.987189825241073,0.987189825241073,0.987189825241073,0.987189825241073,
0.987189825241073,0.987189825241073,0.987189825241073),(1.,1.,1.,1.,1.,
1.,1.,1.,1.,1.,1.,1.)))
REPRESENTATION_ITEM('')
SURFACE()
);
#553=(
BOUNDED_SURFACE()
B_SPLINE_SURFACE(3,3,((#35063,#35064,#35065,#35066,#35067,#35068,#35069,
#35070,#35071,#35072,#35073,#35074),(#35075,#35076,#35077,#35078,#35079,
#35080,#35081,#35082,#35083,#35084,#35085,#35086),(#35087,#35088,#35089,
#35090,#35091,#35092,#35093,#35094,#35095,#35096,#35097,#35098),(#35099,
#35100,#35101,#35102,#35103,#35104,#35105,#35106,#35107,#35108,#35109,#35110)),
 .UNSPECIFIED.,.F.,.F.,.F.)
B_SPLINE_SURFACE_WITH_KNOTS((4,4),(4,2,2,2,2,4),(0.,1.),(0.,0.078369838840116,
0.308777379129587,0.539184919419724,0.769592459709862,1.),.UNSPECIFIED.)
GEOMETRIC_REPRESENTATION_ITEM()
RATIONAL_B_SPLINE_SURFACE(((1.,1.,1.,1.,1.,1.,1.,1.,1.,1.,1.,1.),(0.833333333333333,
0.833333333333333,0.833333333333333,0.833333333333333,0.833333333333333,
0.833333333333333,0.833333333333333,0.833333333333333,0.833333333333333,
0.833333333333333,0.833333333333333,0.833333333333333),(0.833333333333333,
0.833333333333333,0.833333333333333,0.833333333333333,0.833333333333333,
0.833333333333333,0.833333333333333,0.833333333333333,0.833333333333333,
0.833333333333333,0.833333333333333,0.833333333333333),(1.,1.,1.,1.,1.,
1.,1.,1.,1.,1.,1.,1.)))
REPRESENTATION_ITEM('')
SURFACE()
);
#554=(
BOUNDED_SURFACE()
B_SPLINE_SURFACE(3,3,((#35127,#35128,#35129,#35130,#35131,#35132,#35133,
#35134,#35135,#35136,#35137,#35138),(#35139,#35140,#35141,#35142,#35143,
#35144,#35145,#35146,#35147,#35148,#35149,#35150),(#35151,#35152,#35153,
#35154,#35155,#35156,#35157,#35158,#35159,#35160,#35161,#35162),(#35163,
#35164,#35165,#35166,#35167,#35168,#35169,#35170,#35171,#35172,#35173,#35174)),
 .UNSPECIFIED.,.F.,.F.,.F.)
B_SPLINE_SURFACE_WITH_KNOTS((4,4),(4,2,2,2,2,4),(0.,1.),(0.,0.078369838840116,
0.308777379129587,0.539184919419724,0.769592459709862,1.),.UNSPECIFIED.)
GEOMETRIC_REPRESENTATION_ITEM()
RATIONAL_B_SPLINE_SURFACE(((1.,1.,1.,1.,1.,1.,1.,1.,1.,1.,1.,1.),(0.987189825241073,
0.987189825241073,0.987189825241073,0.987189825241073,0.987189825241073,
0.987189825241073,0.987189825241073,0.987189825241073,0.987189825241073,
0.987189825241073,0.987189825241073,0.987189825241073),(0.987189825241073,
0.987189825241073,0.987189825241073,0.987189825241073,0.987189825241073,
0.987189825241073,0.987189825241073,0.987189825241073,0.987189825241073,
0.987189825241073,0.987189825241073,0.987189825241073),(1.,1.,1.,1.,1.,
1.,1.,1.,1.,1.,1.,1.)))
REPRESENTATION_ITEM('')
SURFACE()
);
#555=(
BOUNDED_SURFACE()
B_SPLINE_SURFACE(3,3,((#35175,#35176,#35177,#35178,#35179,#35180,#35181,
#35182,#35183,#35184,#35185,#35186),(#35187,#35188,#35189,#35190,#35191,
#35192,#35193,#35194,#35195,#35196,#35197,#35198),(#35199,#35200,#35201,
#35202,#35203,#35204,#35205,#35206,#35207,#35208,#35209,#35210),(#35211,
#35212,#35213,#35214,#35215,#35216,#35217,#35218,#35219,#35220,#35221,#35222)),
 .UNSPECIFIED.,.F.,.F.,.F.)
B_SPLINE_SURFACE_WITH_KNOTS((4,4),(4,2,2,2,2,4),(0.,1.),(0.,0.078369838840116,
0.308777379129587,0.539184919419724,0.769592459709862,1.),.UNSPECIFIED.)
GEOMETRIC_REPRESENTATION_ITEM()
RATIONAL_B_SPLINE_SURFACE(((1.,1.,1.,1.,1.,1.,1.,1.,1.,1.,1.,1.),(0.987189825241073,
0.987189825241073,0.987189825241073,0.987189825241073,0.987189825241073,
0.987189825241073,0.987189825241073,0.987189825241073,0.987189825241073,
0.987189825241073,0.987189825241073,0.987189825241073),(0.987189825241073,
0.987189825241073,0.987189825241073,0.987189825241073,0.987189825241073,
0.987189825241073,0.987189825241073,0.987189825241073,0.987189825241073,
0.987189825241073,0.987189825241073,0.987189825241073),(1.,1.,1.,1.,1.,
1.,1.,1.,1.,1.,1.,1.)))
REPRESENTATION_ITEM('')
SURFACE()
);
#556=(
BOUNDED_SURFACE()
B_SPLINE_SURFACE(3,3,((#35223,#35224,#35225,#35226,#35227,#35228,#35229,
#35230,#35231,#35232,#35233,#35234),(#35235,#35236,#35237,#35238,#35239,
#35240,#35241,#35242,#35243,#35244,#35245,#35246),(#35247,#35248,#35249,
#35250,#35251,#35252,#35253,#35254,#35255,#35256,#35257,#35258),(#35259,
#35260,#35261,#35262,#35263,#35264,#35265,#35266,#35267,#35268,#35269,#35270)),
 .UNSPECIFIED.,.F.,.F.,.F.)
B_SPLINE_SURFACE_WITH_KNOTS((4,4),(4,2,2,2,2,4),(0.,1.),(0.,0.0783698352504284,
0.308777376437322,0.53918491762488,0.76959245881244,1.),.UNSPECIFIED.)
GEOMETRIC_REPRESENTATION_ITEM()
RATIONAL_B_SPLINE_SURFACE(((1.,1.,1.,1.,1.,1.,1.,1.,1.,1.,1.,1.),(0.833333333333332,
0.833333333333332,0.833333333333332,0.833333333333332,0.833333333333332,
0.833333333333332,0.833333333333332,0.833333333333332,0.833333333333332,
0.833333333333332,0.833333333333332,0.833333333333332),(0.833333333333332,
0.833333333333332,0.833333333333332,0.833333333333332,0.833333333333332,
0.833333333333332,0.833333333333332,0.833333333333332,0.833333333333332,
0.833333333333332,0.833333333333332,0.833333333333332),(1.,1.,1.,1.,1.,
1.,1.,1.,1.,1.,1.,1.)))
REPRESENTATION_ITEM('')
SURFACE()
);
#557=(
BOUNDED_SURFACE()
B_SPLINE_SURFACE(3,3,((#35287,#35288,#35289,#35290,#35291,#35292,#35293,
#35294,#35295,#35296,#35297,#35298),(#35299,#35300,#35301,#35302,#35303,
#35304,#35305,#35306,#35307,#35308,#35309,#35310),(#35311,#35312,#35313,
#35314,#35315,#35316,#35317,#35318,#35319,#35320,#35321,#35322),(#35323,
#35324,#35325,#35326,#35327,#35328,#35329,#35330,#35331,#35332,#35333,#35334)),
 .UNSPECIFIED.,.F.,.F.,.F.)
B_SPLINE_SURFACE_WITH_KNOTS((4,4),(4,2,2,2,2,4),(0.,1.),(0.,0.0783698352504284,
0.308777376437322,0.53918491762488,0.76959245881244,1.),.UNSPECIFIED.)
GEOMETRIC_REPRESENTATION_ITEM()
RATIONAL_B_SPLINE_SURFACE(((1.,1.,1.,1.,1.,1.,1.,1.,1.,1.,1.,1.),(0.987189825241073,
0.987189825241073,0.987189825241073,0.987189825241073,0.987189825241073,
0.987189825241073,0.987189825241073,0.987189825241073,0.987189825241073,
0.987189825241073,0.987189825241073,0.987189825241073),(0.987189825241073,
0.987189825241073,0.987189825241073,0.987189825241073,0.987189825241073,
0.987189825241073,0.987189825241073,0.987189825241073,0.987189825241073,
0.987189825241073,0.987189825241073,0.987189825241073),(1.,1.,1.,1.,1.,
1.,1.,1.,1.,1.,1.,1.)))
REPRESENTATION_ITEM('')
SURFACE()
);
#558=(
BOUNDED_SURFACE()
B_SPLINE_SURFACE(3,3,((#35335,#35336,#35337,#35338,#35339,#35340,#35341,
#35342,#35343,#35344,#35345,#35346),(#35347,#35348,#35349,#35350,#35351,
#35352,#35353,#35354,#35355,#35356,#35357,#35358),(#35359,#35360,#35361,
#35362,#35363,#35364,#35365,#35366,#35367,#35368,#35369,#35370),(#35371,
#35372,#35373,#35374,#35375,#35376,#35377,#35378,#35379,#35380,#35381,#35382)),
 .UNSPECIFIED.,.F.,.F.,.F.)
B_SPLINE_SURFACE_WITH_KNOTS((4,4),(4,2,2,2,2,4),(0.,1.),(0.,0.0783698352504284,
0.308777376437322,0.53918491762488,0.76959245881244,1.),.UNSPECIFIED.)
GEOMETRIC_REPRESENTATION_ITEM()
RATIONAL_B_SPLINE_SURFACE(((1.,1.,1.,1.,1.,1.,1.,1.,1.,1.,1.,1.),(0.987189825241073,
0.987189825241073,0.987189825241073,0.987189825241073,0.987189825241073,
0.987189825241073,0.987189825241073,0.987189825241073,0.987189825241073,
0.987189825241073,0.987189825241073,0.987189825241073),(0.987189825241073,
0.987189825241073,0.987189825241073,0.987189825241073,0.987189825241073,
0.987189825241073,0.987189825241073,0.987189825241073,0.987189825241073,
0.987189825241073,0.987189825241073,0.987189825241073),(1.,1.,1.,1.,1.,
1.,1.,1.,1.,1.,1.,1.)))
REPRESENTATION_ITEM('')
SURFACE()
);
#559=(
BOUNDED_SURFACE()
B_SPLINE_SURFACE(3,3,((#35383,#35384,#35385,#35386,#35387,#35388,#35389,
#35390,#35391,#35392,#35393,#35394,#35395,#35396),(#35397,#35398,#35399,
#35400,#35401,#35402,#35403,#35404,#35405,#35406,#35407,#35408,#35409,#35410),
(#35411,#35412,#35413,#35414,#35415,#35416,#35417,#35418,#35419,#35420,
#35421,#35422,#35423,#35424),(#35425,#35426,#35427,#35428,#35429,#35430,
#35431,#35432,#35433,#35434,#35435,#35436,#35437,#35438)),.UNSPECIFIED.,
 .F.,.F.,.F.)
B_SPLINE_SURFACE_WITH_KNOTS((4,4),(4,2,2,2,2,2,4),(0.,1.),(0.,0.0183879168994272,
0.0783698293107271,0.308777371982546,0.53918491465503,0.769592457327514,
1.),.UNSPECIFIED.)
GEOMETRIC_REPRESENTATION_ITEM()
RATIONAL_B_SPLINE_SURFACE(((1.,1.,1.,1.,1.,1.,1.,1.,1.,1.,1.,1.,1.,1.),
(0.833333333333332,0.833333333333332,0.833333333333332,0.833333333333332,
0.833333333333332,0.833333333333332,0.833333333333332,0.833333333333332,
0.833333333333332,0.833333333333332,0.833333333333332,0.833333333333332,
0.833333333333332,0.833333333333332),(0.833333333333332,0.833333333333332,
0.833333333333332,0.833333333333332,0.833333333333332,0.833333333333332,
0.833333333333332,0.833333333333332,0.833333333333332,0.833333333333332,
0.833333333333332,0.833333333333332,0.833333333333332,0.833333333333332),
(1.,1.,1.,1.,1.,1.,1.,1.,1.,1.,1.,1.,1.,1.)))
REPRESENTATION_ITEM('')
SURFACE()
);
#560=(
BOUNDED_SURFACE()
B_SPLINE_SURFACE(3,3,((#35457,#35458,#35459,#35460,#35461,#35462,#35463,
#35464,#35465,#35466,#35467,#35468,#35469,#35470),(#35471,#35472,#35473,
#35474,#35475,#35476,#35477,#35478,#35479,#35480,#35481,#35482,#35483,#35484),
(#35485,#35486,#35487,#35488,#35489,#35490,#35491,#35492,#35493,#35494,
#35495,#35496,#35497,#35498),(#35499,#35500,#35501,#35502,#35503,#35504,
#35505,#35506,#35507,#35508,#35509,#35510,#35511,#35512)),.UNSPECIFIED.,
 .F.,.F.,.F.)
B_SPLINE_SURFACE_WITH_KNOTS((4,4),(4,2,2,2,2,2,4),(0.,1.),(0.,0.0183879168994272,
0.0783698293107271,0.308777371982546,0.53918491465503,0.769592457327514,
1.),.UNSPECIFIED.)
GEOMETRIC_REPRESENTATION_ITEM()
RATIONAL_B_SPLINE_SURFACE(((1.,1.,1.,1.,1.,1.,1.,1.,1.,1.,1.,1.,1.,1.),
(0.987189825241073,0.987189825241073,0.987189825241073,0.987189825241073,
0.987189825241073,0.987189825241073,0.987189825241073,0.987189825241073,
0.987189825241073,0.987189825241073,0.987189825241073,0.987189825241073,
0.987189825241073,0.987189825241073),(0.987189825241073,0.987189825241073,
0.987189825241073,0.987189825241073,0.987189825241073,0.987189825241073,
0.987189825241073,0.987189825241073,0.987189825241073,0.987189825241073,
0.987189825241073,0.987189825241073,0.987189825241073,0.987189825241073),
(1.,1.,1.,1.,1.,1.,1.,1.,1.,1.,1.,1.,1.,1.)))
REPRESENTATION_ITEM('')
SURFACE()
);
#561=(
BOUNDED_SURFACE()
B_SPLINE_SURFACE(3,3,((#35513,#35514,#35515,#35516,#35517,#35518,#35519,
#35520,#35521,#35522,#35523,#35524,#35525,#35526),(#35527,#35528,#35529,
#35530,#35531,#35532,#35533,#35534,#35535,#35536,#35537,#35538,#35539,#35540),
(#35541,#35542,#35543,#35544,#35545,#35546,#35547,#35548,#35549,#35550,
#35551,#35552,#35553,#35554),(#35555,#35556,#35557,#35558,#35559,#35560,
#35561,#35562,#35563,#35564,#35565,#35566,#35567,#35568)),.UNSPECIFIED.,
 .F.,.F.,.F.)
B_SPLINE_SURFACE_WITH_KNOTS((4,4),(4,2,2,2,2,2,4),(0.,1.),(0.,0.0183879168994272,
0.0783698293107271,0.308777371982546,0.53918491465503,0.769592457327514,
1.),.UNSPECIFIED.)
GEOMETRIC_REPRESENTATION_ITEM()
RATIONAL_B_SPLINE_SURFACE(((1.,1.,1.,1.,1.,1.,1.,1.,1.,1.,1.,1.,1.,1.),
(0.987189825241073,0.987189825241073,0.987189825241073,0.987189825241073,
0.987189825241073,0.987189825241073,0.987189825241073,0.987189825241073,
0.987189825241073,0.987189825241073,0.987189825241073,0.987189825241073,
0.987189825241073,0.987189825241073),(0.987189825241073,0.987189825241073,
0.987189825241073,0.987189825241073,0.987189825241073,0.987189825241073,
0.987189825241073,0.987189825241073,0.987189825241073,0.987189825241073,
0.987189825241073,0.987189825241073,0.987189825241073,0.987189825241073),
(1.,1.,1.,1.,1.,1.,1.,1.,1.,1.,1.,1.,1.,1.)))
REPRESENTATION_ITEM('')
SURFACE()
);
#562=(
BOUNDED_SURFACE()
B_SPLINE_SURFACE(3,3,((#35569,#35570,#35571,#35572,#35573,#35574,#35575,
#35576,#35577,#35578,#35579,#35580,#35581,#35582),(#35583,#35584,#35585,
#35586,#35587,#35588,#35589,#35590,#35591,#35592,#35593,#35594,#35595,#35596),
(#35597,#35598,#35599,#35600,#35601,#35602,#35603,#35604,#35605,#35606,
#35607,#35608,#35609,#35610),(#35611,#35612,#35613,#35614,#35615,#35616,
#35617,#35618,#35619,#35620,#35621,#35622,#35623,#35624)),.UNSPECIFIED.,
 .F.,.F.,.F.)
B_SPLINE_SURFACE_WITH_KNOTS((4,4),(4,2,2,2,2,2,4),(0.,1.),(0.,0.0183879232268624,
0.0783698352504226,0.308777376437317,0.539184917624878,0.769592458812438,
1.),.UNSPECIFIED.)
GEOMETRIC_REPRESENTATION_ITEM()
RATIONAL_B_SPLINE_SURFACE(((1.,1.,1.,1.,1.,1.,1.,1.,1.,1.,1.,1.,1.,1.),
(0.833333333333333,0.833333333333333,0.833333333333333,0.833333333333333,
0.833333333333333,0.833333333333333,0.833333333333333,0.833333333333333,
0.833333333333333,0.833333333333333,0.833333333333333,0.833333333333333,
0.833333333333333,0.833333333333333),(0.833333333333333,0.833333333333333,
0.833333333333333,0.833333333333333,0.833333333333333,0.833333333333333,
0.833333333333333,0.833333333333333,0.833333333333333,0.833333333333333,
0.833333333333333,0.833333333333333,0.833333333333333,0.833333333333333),
(1.,1.,1.,1.,1.,1.,1.,1.,1.,1.,1.,1.,1.,1.)))
REPRESENTATION_ITEM('')
SURFACE()
);
#563=(
BOUNDED_SURFACE()
B_SPLINE_SURFACE(3,3,((#35643,#35644,#35645,#35646,#35647,#35648,#35649,
#35650,#35651,#35652,#35653,#35654,#35655,#35656),(#35657,#35658,#35659,
#35660,#35661,#35662,#35663,#35664,#35665,#35666,#35667,#35668,#35669,#35670),
(#35671,#35672,#35673,#35674,#35675,#35676,#35677,#35678,#35679,#35680,
#35681,#35682,#35683,#35684),(#35685,#35686,#35687,#35688,#35689,#35690,
#35691,#35692,#35693,#35694,#35695,#35696,#35697,#35698)),.UNSPECIFIED.,
 .F.,.F.,.F.)
B_SPLINE_SURFACE_WITH_KNOTS((4,4),(4,2,2,2,2,2,4),(0.,1.),(0.,0.0183879232268624,
0.0783698352504226,0.308777376437317,0.539184917624878,0.769592458812438,
1.),.UNSPECIFIED.)
GEOMETRIC_REPRESENTATION_ITEM()
RATIONAL_B_SPLINE_SURFACE(((1.,1.,1.,1.,1.,1.,1.,1.,1.,1.,1.,1.,1.,1.),
(0.987189825241073,0.987189825241073,0.987189825241073,0.987189825241073,
0.987189825241073,0.987189825241073,0.987189825241073,0.987189825241073,
0.987189825241073,0.987189825241073,0.987189825241073,0.987189825241073,
0.987189825241073,0.987189825241073),(0.987189825241073,0.987189825241073,
0.987189825241073,0.987189825241073,0.987189825241073,0.987189825241073,
0.987189825241073,0.987189825241073,0.987189825241073,0.987189825241073,
0.987189825241073,0.987189825241073,0.987189825241073,0.987189825241073),
(1.,1.,1.,1.,1.,1.,1.,1.,1.,1.,1.,1.,1.,1.)))
REPRESENTATION_ITEM('')
SURFACE()
);
#564=(
BOUNDED_SURFACE()
B_SPLINE_SURFACE(3,3,((#35699,#35700,#35701,#35702,#35703,#35704,#35705,
#35706,#35707,#35708,#35709,#35710,#35711,#35712),(#35713,#35714,#35715,
#35716,#35717,#35718,#35719,#35720,#35721,#35722,#35723,#35724,#35725,#35726),
(#35727,#35728,#35729,#35730,#35731,#35732,#35733,#35734,#35735,#35736,
#35737,#35738,#35739,#35740),(#35741,#35742,#35743,#35744,#35745,#35746,
#35747,#35748,#35749,#35750,#35751,#35752,#35753,#35754)),.UNSPECIFIED.,
 .F.,.F.,.F.)
B_SPLINE_SURFACE_WITH_KNOTS((4,4),(4,2,2,2,2,2,4),(0.,1.),(0.,0.0183879232268624,
0.0783698352504226,0.308777376437317,0.539184917624878,0.769592458812438,
1.),.UNSPECIFIED.)
GEOMETRIC_REPRESENTATION_ITEM()
RATIONAL_B_SPLINE_SURFACE(((1.,1.,1.,1.,1.,1.,1.,1.,1.,1.,1.,1.,1.,1.),
(0.987189825241073,0.987189825241073,0.987189825241073,0.987189825241073,
0.987189825241073,0.987189825241073,0.987189825241073,0.987189825241073,
0.987189825241073,0.987189825241073,0.987189825241073,0.987189825241073,
0.987189825241073,0.987189825241073),(0.987189825241073,0.987189825241073,
0.987189825241073,0.987189825241073,0.987189825241073,0.987189825241073,
0.987189825241073,0.987189825241073,0.987189825241073,0.987189825241073,
0.987189825241073,0.987189825241073,0.987189825241073,0.987189825241073),
(1.,1.,1.,1.,1.,1.,1.,1.,1.,1.,1.,1.,1.,1.)))
REPRESENTATION_ITEM('')
SURFACE()
);
#565=(
BOUNDED_SURFACE()
B_SPLINE_SURFACE(3,3,((#35755,#35756,#35757,#35758,#35759,#35760,#35761,
#35762,#35763,#35764,#35765,#35766),(#35767,#35768,#35769,#35770,#35771,
#35772,#35773,#35774,#35775,#35776,#35777,#35778),(#35779,#35780,#35781,
#35782,#35783,#35784,#35785,#35786,#35787,#35788,#35789,#35790),(#35791,
#35792,#35793,#35794,#35795,#35796,#35797,#35798,#35799,#35800,#35801,#35802)),
 .UNSPECIFIED.,.F.,.F.,.F.)
B_SPLINE_SURFACE_WITH_KNOTS((4,4),(4,2,2,2,2,4),(0.,1.),(0.,0.078369838840114,
0.308777379129586,0.539184919419723,0.769592459709861,1.),.UNSPECIFIED.)
GEOMETRIC_REPRESENTATION_ITEM()
RATIONAL_B_SPLINE_SURFACE(((1.,1.,1.,1.,1.,1.,1.,1.,1.,1.,1.,1.),(0.833333333333332,
0.833333333333332,0.833333333333332,0.833333333333332,0.833333333333332,
0.833333333333332,0.833333333333332,0.833333333333332,0.833333333333332,
0.833333333333332,0.833333333333332,0.833333333333332),(0.833333333333332,
0.833333333333332,0.833333333333332,0.833333333333332,0.833333333333332,
0.833333333333332,0.833333333333332,0.833333333333332,0.833333333333332,
0.833333333333332,0.833333333333332,0.833333333333332),(1.,1.,1.,1.,1.,
1.,1.,1.,1.,1.,1.,1.)))
REPRESENTATION_ITEM('')
SURFACE()
);
#566=(
BOUNDED_SURFACE()
B_SPLINE_SURFACE(3,3,((#35819,#35820,#35821,#35822,#35823,#35824,#35825,
#35826,#35827,#35828,#35829,#35830),(#35831,#35832,#35833,#35834,#35835,
#35836,#35837,#35838,#35839,#35840,#35841,#35842),(#35843,#35844,#35845,
#35846,#35847,#35848,#35849,#35850,#35851,#35852,#35853,#35854),(#35855,
#35856,#35857,#35858,#35859,#35860,#35861,#35862,#35863,#35864,#35865,#35866)),
 .UNSPECIFIED.,.F.,.F.,.F.)
B_SPLINE_SURFACE_WITH_KNOTS((4,4),(4,2,2,2,2,4),(0.,1.),(0.,0.078369838840114,
0.308777379129586,0.539184919419723,0.769592459709861,1.),.UNSPECIFIED.)
GEOMETRIC_REPRESENTATION_ITEM()
RATIONAL_B_SPLINE_SURFACE(((1.,1.,1.,1.,1.,1.,1.,1.,1.,1.,1.,1.),(0.987189825241073,
0.987189825241073,0.987189825241073,0.987189825241073,0.987189825241073,
0.987189825241073,0.987189825241073,0.987189825241073,0.987189825241073,
0.987189825241073,0.987189825241073,0.987189825241073),(0.987189825241073,
0.987189825241073,0.987189825241073,0.987189825241073,0.987189825241073,
0.987189825241073,0.987189825241073,0.987189825241073,0.987189825241073,
0.987189825241073,0.987189825241073,0.987189825241073),(1.,1.,1.,1.,1.,
1.,1.,1.,1.,1.,1.,1.)))
REPRESENTATION_ITEM('')
SURFACE()
);
#567=(
BOUNDED_SURFACE()
B_SPLINE_SURFACE(3,3,((#35867,#35868,#35869,#35870,#35871,#35872,#35873,
#35874,#35875,#35876,#35877,#35878),(#35879,#35880,#35881,#35882,#35883,
#35884,#35885,#35886,#35887,#35888,#35889,#35890),(#35891,#35892,#35893,
#35894,#35895,#35896,#35897,#35898,#35899,#35900,#35901,#35902),(#35903,
#35904,#35905,#35906,#35907,#35908,#35909,#35910,#35911,#35912,#35913,#35914)),
 .UNSPECIFIED.,.F.,.F.,.F.)
B_SPLINE_SURFACE_WITH_KNOTS((4,4),(4,2,2,2,2,4),(0.,1.),(0.,0.078369838840114,
0.308777379129586,0.539184919419723,0.769592459709861,1.),.UNSPECIFIED.)
GEOMETRIC_REPRESENTATION_ITEM()
RATIONAL_B_SPLINE_SURFACE(((1.,1.,1.,1.,1.,1.,1.,1.,1.,1.,1.,1.),(0.987189825241073,
0.987189825241073,0.987189825241073,0.987189825241073,0.987189825241073,
0.987189825241073,0.987189825241073,0.987189825241073,0.987189825241073,
0.987189825241073,0.987189825241073,0.987189825241073),(0.987189825241073,
0.987189825241073,0.987189825241073,0.987189825241073,0.987189825241073,
0.987189825241073,0.987189825241073,0.987189825241073,0.987189825241073,
0.987189825241073,0.987189825241073,0.987189825241073),(1.,1.,1.,1.,1.,
1.,1.,1.,1.,1.,1.,1.)))
REPRESENTATION_ITEM('')
SURFACE()
);
#568=(
BOUNDED_SURFACE()
B_SPLINE_SURFACE(3,3,((#35915,#35916,#35917,#35918,#35919,#35920,#35921,
#35922,#35923,#35924,#35925,#35926),(#35927,#35928,#35929,#35930,#35931,
#35932,#35933,#35934,#35935,#35936,#35937,#35938),(#35939,#35940,#35941,
#35942,#35943,#35944,#35945,#35946,#35947,#35948,#35949,#35950),(#35951,
#35952,#35953,#35954,#35955,#35956,#35957,#35958,#35959,#35960,#35961,#35962)),
 .UNSPECIFIED.,.F.,.F.,.F.)
B_SPLINE_SURFACE_WITH_KNOTS((4,4),(4,2,2,2,2,4),(0.,1.),(0.,0.078369843731106,
0.30877738279783,0.539184921865219,0.769592460932609,1.),.UNSPECIFIED.)
GEOMETRIC_REPRESENTATION_ITEM()
RATIONAL_B_SPLINE_SURFACE(((1.,1.,1.,1.,1.,1.,1.,1.,1.,1.,1.,1.),(0.833333333333331,
0.833333333333331,0.833333333333331,0.833333333333331,0.833333333333331,
0.833333333333331,0.833333333333331,0.833333333333331,0.833333333333331,
0.833333333333331,0.833333333333331,0.833333333333331),(0.833333333333331,
0.833333333333331,0.833333333333331,0.833333333333331,0.833333333333331,
0.833333333333331,0.833333333333331,0.833333333333331,0.833333333333331,
0.833333333333331,0.833333333333331,0.833333333333331),(1.,1.,1.,1.,1.,
1.,1.,1.,1.,1.,1.,1.)))
REPRESENTATION_ITEM('')
SURFACE()
);
#569=(
BOUNDED_SURFACE()
B_SPLINE_SURFACE(3,3,((#35979,#35980,#35981,#35982,#35983,#35984,#35985,
#35986,#35987,#35988,#35989,#35990),(#35991,#35992,#35993,#35994,#35995,
#35996,#35997,#35998,#35999,#36000,#36001,#36002),(#36003,#36004,#36005,
#36006,#36007,#36008,#36009,#36010,#36011,#36012,#36013,#36014),(#36015,
#36016,#36017,#36018,#36019,#36020,#36021,#36022,#36023,#36024,#36025,#36026)),
 .UNSPECIFIED.,.F.,.F.,.F.)
B_SPLINE_SURFACE_WITH_KNOTS((4,4),(4,2,2,2,2,4),(0.,1.),(0.,0.078369843731106,
0.30877738279783,0.539184921865219,0.769592460932609,1.),.UNSPECIFIED.)
GEOMETRIC_REPRESENTATION_ITEM()
RATIONAL_B_SPLINE_SURFACE(((1.,1.,1.,1.,1.,1.,1.,1.,1.,1.,1.,1.),(0.987189825241073,
0.987189825241073,0.987189825241073,0.987189825241073,0.987189825241073,
0.987189825241073,0.987189825241073,0.987189825241073,0.987189825241073,
0.987189825241073,0.987189825241073,0.987189825241073),(0.987189825241073,
0.987189825241073,0.987189825241073,0.987189825241073,0.987189825241073,
0.987189825241073,0.987189825241073,0.987189825241073,0.987189825241073,
0.987189825241073,0.987189825241073,0.987189825241073),(1.,1.,1.,1.,1.,
1.,1.,1.,1.,1.,1.,1.)))
REPRESENTATION_ITEM('')
SURFACE()
);
#570=(
BOUNDED_SURFACE()
B_SPLINE_SURFACE(3,3,((#36027,#36028,#36029,#36030,#36031,#36032,#36033,
#36034,#36035,#36036,#36037,#36038),(#36039,#36040,#36041,#36042,#36043,
#36044,#36045,#36046,#36047,#36048,#36049,#36050),(#36051,#36052,#36053,
#36054,#36055,#36056,#36057,#36058,#36059,#36060,#36061,#36062),(#36063,
#36064,#36065,#36066,#36067,#36068,#36069,#36070,#36071,#36072,#36073,#36074)),
 .UNSPECIFIED.,.F.,.F.,.F.)
B_SPLINE_SURFACE_WITH_KNOTS((4,4),(4,2,2,2,2,4),(0.,1.),(0.,0.078369843731106,
0.30877738279783,0.539184921865219,0.769592460932609,1.),.UNSPECIFIED.)
GEOMETRIC_REPRESENTATION_ITEM()
RATIONAL_B_SPLINE_SURFACE(((1.,1.,1.,1.,1.,1.,1.,1.,1.,1.,1.,1.),(0.987189825241073,
0.987189825241073,0.987189825241073,0.987189825241073,0.987189825241073,
0.987189825241073,0.987189825241073,0.987189825241073,0.987189825241073,
0.987189825241073,0.987189825241073,0.987189825241073),(0.987189825241073,
0.987189825241073,0.987189825241073,0.987189825241073,0.987189825241073,
0.987189825241073,0.987189825241073,0.987189825241073,0.987189825241073,
0.987189825241073,0.987189825241073,0.987189825241073),(1.,1.,1.,1.,1.,
1.,1.,1.,1.,1.,1.,1.)))
REPRESENTATION_ITEM('')
SURFACE()
);
#571=(
BOUNDED_SURFACE()
B_SPLINE_SURFACE(3,3,((#36075,#36076,#36077,#36078,#36079,#36080,#36081,
#36082,#36083,#36084,#36085,#36086),(#36087,#36088,#36089,#36090,#36091,
#36092,#36093,#36094,#36095,#36096,#36097,#36098),(#36099,#36100,#36101,
#36102,#36103,#36104,#36105,#36106,#36107,#36108,#36109,#36110),(#36111,
#36112,#36113,#36114,#36115,#36116,#36117,#36118,#36119,#36120,#36121,#36122)),
 .UNSPECIFIED.,.F.,.F.,.F.)
B_SPLINE_SURFACE_WITH_KNOTS((4,4),(4,2,2,2,2,4),(0.,1.),(0.,0.0783698481609171,
0.308777386120188,0.539184924080125,0.769592462040062,1.),.UNSPECIFIED.)
GEOMETRIC_REPRESENTATION_ITEM()
RATIONAL_B_SPLINE_SURFACE(((1.,1.,1.,1.,1.,1.,1.,1.,1.,1.,1.,1.),(0.987189825241073,
0.987189825241073,0.987189825241073,0.987189825241073,0.987189825241073,
0.987189825241073,0.987189825241073,0.987189825241073,0.987189825241073,
0.987189825241073,0.987189825241073,0.987189825241073),(0.987189825241073,
0.987189825241073,0.987189825241073,0.987189825241073,0.987189825241073,
0.987189825241073,0.987189825241073,0.987189825241073,0.987189825241073,
0.987189825241073,0.987189825241073,0.987189825241073),(1.,1.,1.,1.,1.,
1.,1.,1.,1.,1.,1.,1.)))
REPRESENTATION_ITEM('')
SURFACE()
);
#572=(
BOUNDED_SURFACE()
B_SPLINE_SURFACE(3,3,((#36131,#36132,#36133,#36134,#36135,#36136,#36137,
#36138,#36139,#36140,#36141,#36142),(#36143,#36144,#36145,#36146,#36147,
#36148,#36149,#36150,#36151,#36152,#36153,#36154),(#36155,#36156,#36157,
#36158,#36159,#36160,#36161,#36162,#36163,#36164,#36165,#36166),(#36167,
#36168,#36169,#36170,#36171,#36172,#36173,#36174,#36175,#36176,#36177,#36178)),
 .UNSPECIFIED.,.F.,.F.,.F.)
B_SPLINE_SURFACE_WITH_KNOTS((4,4),(4,2,2,2,2,4),(0.,1.),(0.,0.0783698481609171,
0.308777386120188,0.539184924080125,0.769592462040062,1.),.UNSPECIFIED.)
GEOMETRIC_REPRESENTATION_ITEM()
RATIONAL_B_SPLINE_SURFACE(((1.,1.,1.,1.,1.,1.,1.,1.,1.,1.,1.,1.),(0.987189825241073,
0.987189825241073,0.987189825241073,0.987189825241073,0.987189825241073,
0.987189825241073,0.987189825241073,0.987189825241073,0.987189825241073,
0.987189825241073,0.987189825241073,0.987189825241073),(0.987189825241073,
0.987189825241073,0.987189825241073,0.987189825241073,0.987189825241073,
0.987189825241073,0.987189825241073,0.987189825241073,0.987189825241073,
0.987189825241073,0.987189825241073,0.987189825241073),(1.,1.,1.,1.,1.,
1.,1.,1.,1.,1.,1.,1.)))
REPRESENTATION_ITEM('')
SURFACE()
);
#573=(
BOUNDED_SURFACE()
B_SPLINE_SURFACE(3,3,((#36187,#36188,#36189,#36190,#36191,#36192,#36193,
#36194,#36195,#36196,#36197,#36198),(#36199,#36200,#36201,#36202,#36203,
#36204,#36205,#36206,#36207,#36208,#36209,#36210),(#36211,#36212,#36213,
#36214,#36215,#36216,#36217,#36218,#36219,#36220,#36221,#36222),(#36223,
#36224,#36225,#36226,#36227,#36228,#36229,#36230,#36231,#36232,#36233,#36234)),
 .UNSPECIFIED.,.F.,.F.,.F.)
B_SPLINE_SURFACE_WITH_KNOTS((4,4),(4,2,2,2,2,4),(0.,1.),(0.,0.0783698481609171,
0.308777386120188,0.539184924080125,0.769592462040062,1.),.UNSPECIFIED.)
GEOMETRIC_REPRESENTATION_ITEM()
RATIONAL_B_SPLINE_SURFACE(((1.,1.,1.,1.,1.,1.,1.,1.,1.,1.,1.,1.),(0.833333333333332,
0.833333333333332,0.833333333333332,0.833333333333332,0.833333333333332,
0.833333333333332,0.833333333333332,0.833333333333332,0.833333333333332,
0.833333333333332,0.833333333333332,0.833333333333332),(0.833333333333332,
0.833333333333332,0.833333333333332,0.833333333333332,0.833333333333332,
0.833333333333332,0.833333333333332,0.833333333333332,0.833333333333332,
0.833333333333332,0.833333333333332,0.833333333333332),(1.,1.,1.,1.,1.,
1.,1.,1.,1.,1.,1.,1.)))
REPRESENTATION_ITEM('')
SURFACE()
);
#574=(
BOUNDED_SURFACE()
B_SPLINE_SURFACE(3,3,((#36235,#36236,#36237,#36238,#36239,#36240,#36241,
#36242,#36243,#36244,#36245,#36246),(#36247,#36248,#36249,#36250,#36251,
#36252,#36253,#36254,#36255,#36256,#36257,#36258),(#36259,#36260,#36261,
#36262,#36263,#36264,#36265,#36266,#36267,#36268,#36269,#36270),(#36271,
#36272,#36273,#36274,#36275,#36276,#36277,#36278,#36279,#36280,#36281,#36282)),
 .UNSPECIFIED.,.F.,.F.,.F.)
B_SPLINE_SURFACE_WITH_KNOTS((4,4),(4,2,2,2,2,4),(0.,1.),(0.,0.0783698504850854,
0.308777387863314,0.539184925242208,0.769592462621104,1.),.UNSPECIFIED.)
GEOMETRIC_REPRESENTATION_ITEM()
RATIONAL_B_SPLINE_SURFACE(((1.,1.,1.,1.,1.,1.,1.,1.,1.,1.,1.,1.),(0.833333333333333,
0.833333333333333,0.833333333333333,0.833333333333333,0.833333333333333,
0.833333333333333,0.833333333333333,0.833333333333333,0.833333333333333,
0.833333333333333,0.833333333333333,0.833333333333333),(0.833333333333333,
0.833333333333333,0.833333333333333,0.833333333333333,0.833333333333333,
0.833333333333333,0.833333333333333,0.833333333333333,0.833333333333333,
0.833333333333333,0.833333333333333,0.833333333333333),(1.,1.,1.,1.,1.,
1.,1.,1.,1.,1.,1.,1.)))
REPRESENTATION_ITEM('')
SURFACE()
);
#575=(
BOUNDED_SURFACE()
B_SPLINE_SURFACE(3,3,((#36299,#36300,#36301,#36302,#36303,#36304,#36305,
#36306,#36307,#36308,#36309,#36310),(#36311,#36312,#36313,#36314,#36315,
#36316,#36317,#36318,#36319,#36320,#36321,#36322),(#36323,#36324,#36325,
#36326,#36327,#36328,#36329,#36330,#36331,#36332,#36333,#36334),(#36335,
#36336,#36337,#36338,#36339,#36340,#36341,#36342,#36343,#36344,#36345,#36346)),
 .UNSPECIFIED.,.F.,.F.,.F.)
B_SPLINE_SURFACE_WITH_KNOTS((4,4),(4,2,2,2,2,4),(0.,1.),(0.,0.0783698504850854,
0.308777387863314,0.539184925242208,0.769592462621104,1.),.UNSPECIFIED.)
GEOMETRIC_REPRESENTATION_ITEM()
RATIONAL_B_SPLINE_SURFACE(((1.,1.,1.,1.,1.,1.,1.,1.,1.,1.,1.,1.),(0.987189825241073,
0.987189825241073,0.987189825241073,0.987189825241073,0.987189825241073,
0.987189825241073,0.987189825241073,0.987189825241073,0.987189825241073,
0.987189825241073,0.987189825241073,0.987189825241073),(0.987189825241073,
0.987189825241073,0.987189825241073,0.987189825241073,0.987189825241073,
0.987189825241073,0.987189825241073,0.987189825241073,0.987189825241073,
0.987189825241073,0.987189825241073,0.987189825241073),(1.,1.,1.,1.,1.,
1.,1.,1.,1.,1.,1.,1.)))
REPRESENTATION_ITEM('')
SURFACE()
);
#576=(
BOUNDED_SURFACE()
B_SPLINE_SURFACE(3,3,((#36347,#36348,#36349,#36350,#36351,#36352,#36353,
#36354,#36355,#36356,#36357,#36358),(#36359,#36360,#36361,#36362,#36363,
#36364,#36365,#36366,#36367,#36368,#36369,#36370),(#36371,#36372,#36373,
#36374,#36375,#36376,#36377,#36378,#36379,#36380,#36381,#36382),(#36383,
#36384,#36385,#36386,#36387,#36388,#36389,#36390,#36391,#36392,#36393,#36394)),
 .UNSPECIFIED.,.F.,.F.,.F.)
B_SPLINE_SURFACE_WITH_KNOTS((4,4),(4,2,2,2,2,4),(0.,1.),(0.,0.0783698504850854,
0.308777387863314,0.539184925242208,0.769592462621104,1.),.UNSPECIFIED.)
GEOMETRIC_REPRESENTATION_ITEM()
RATIONAL_B_SPLINE_SURFACE(((1.,1.,1.,1.,1.,1.,1.,1.,1.,1.,1.,1.),(0.987189825241073,
0.987189825241073,0.987189825241073,0.987189825241073,0.987189825241073,
0.987189825241073,0.987189825241073,0.987189825241073,0.987189825241073,
0.987189825241073,0.987189825241073,0.987189825241073),(0.987189825241073,
0.987189825241073,0.987189825241073,0.987189825241073,0.987189825241073,
0.987189825241073,0.987189825241073,0.987189825241073,0.987189825241073,
0.987189825241073,0.987189825241073,0.987189825241073),(1.,1.,1.,1.,1.,
1.,1.,1.,1.,1.,1.,1.)))
REPRESENTATION_ITEM('')
SURFACE()
);
#577=(
BOUNDED_SURFACE()
B_SPLINE_SURFACE(3,3,((#36395,#36396,#36397,#36398,#36399,#36400,#36401,
#36402,#36403,#36404,#36405,#36406),(#36407,#36408,#36409,#36410,#36411,
#36412,#36413,#36414,#36415,#36416,#36417,#36418),(#36419,#36420,#36421,
#36422,#36423,#36424,#36425,#36426,#36427,#36428,#36429,#36430),(#36431,
#36432,#36433,#36434,#36435,#36436,#36437,#36438,#36439,#36440,#36441,#36442)),
 .UNSPECIFIED.,.F.,.F.,.F.)
B_SPLINE_SURFACE_WITH_KNOTS((4,4),(4,2,2,2,2,4),(0.,1.),(0.,0.0783698504851048,
0.308777387863329,0.539184925242218,0.769592462621109,1.),.UNSPECIFIED.)
GEOMETRIC_REPRESENTATION_ITEM()
RATIONAL_B_SPLINE_SURFACE(((1.,1.,1.,1.,1.,1.,1.,1.,1.,1.,1.,1.),(0.833333333333332,
0.833333333333332,0.833333333333332,0.833333333333332,0.833333333333332,
0.833333333333332,0.833333333333332,0.833333333333332,0.833333333333332,
0.833333333333332,0.833333333333332,0.833333333333332),(0.833333333333332,
0.833333333333332,0.833333333333332,0.833333333333332,0.833333333333332,
0.833333333333332,0.833333333333332,0.833333333333332,0.833333333333332,
0.833333333333332,0.833333333333332,0.833333333333332),(1.,1.,1.,1.,1.,
1.,1.,1.,1.,1.,1.,1.)))
REPRESENTATION_ITEM('')
SURFACE()
);
#578=(
BOUNDED_SURFACE()
B_SPLINE_SURFACE(3,3,((#36459,#36460,#36461,#36462,#36463,#36464,#36465,
#36466,#36467,#36468,#36469,#36470),(#36471,#36472,#36473,#36474,#36475,
#36476,#36477,#36478,#36479,#36480,#36481,#36482),(#36483,#36484,#36485,
#36486,#36487,#36488,#36489,#36490,#36491,#36492,#36493,#36494),(#36495,
#36496,#36497,#36498,#36499,#36500,#36501,#36502,#36503,#36504,#36505,#36506)),
 .UNSPECIFIED.,.F.,.F.,.F.)
B_SPLINE_SURFACE_WITH_KNOTS((4,4),(4,2,2,2,2,4),(0.,1.),(0.,0.0783698504851048,
0.308777387863329,0.539184925242218,0.769592462621109,1.),.UNSPECIFIED.)
GEOMETRIC_REPRESENTATION_ITEM()
RATIONAL_B_SPLINE_SURFACE(((1.,1.,1.,1.,1.,1.,1.,1.,1.,1.,1.,1.),(0.987189825241073,
0.987189825241073,0.987189825241073,0.987189825241073,0.987189825241073,
0.987189825241073,0.987189825241073,0.987189825241073,0.987189825241073,
0.987189825241073,0.987189825241073,0.987189825241073),(0.987189825241073,
0.987189825241073,0.987189825241073,0.987189825241073,0.987189825241073,
0.987189825241073,0.987189825241073,0.987189825241073,0.987189825241073,
0.987189825241073,0.987189825241073,0.987189825241073),(1.,1.,1.,1.,1.,
1.,1.,1.,1.,1.,1.,1.)))
REPRESENTATION_ITEM('')
SURFACE()
);
#579=(
BOUNDED_SURFACE()
B_SPLINE_SURFACE(3,3,((#36507,#36508,#36509,#36510,#36511,#36512,#36513,
#36514,#36515,#36516,#36517,#36518),(#36519,#36520,#36521,#36522,#36523,
#36524,#36525,#36526,#36527,#36528,#36529,#36530),(#36531,#36532,#36533,
#36534,#36535,#36536,#36537,#36538,#36539,#36540,#36541,#36542),(#36543,
#36544,#36545,#36546,#36547,#36548,#36549,#36550,#36551,#36552,#36553,#36554)),
 .UNSPECIFIED.,.F.,.F.,.F.)
B_SPLINE_SURFACE_WITH_KNOTS((4,4),(4,2,2,2,2,4),(0.,1.),(0.,0.0783698504851048,
0.308777387863329,0.539184925242218,0.769592462621109,1.),.UNSPECIFIED.)
GEOMETRIC_REPRESENTATION_ITEM()
RATIONAL_B_SPLINE_SURFACE(((1.,1.,1.,1.,1.,1.,1.,1.,1.,1.,1.,1.),(0.987189825241073,
0.987189825241073,0.987189825241073,0.987189825241073,0.987189825241073,
0.987189825241073,0.987189825241073,0.987189825241073,0.987189825241073,
0.987189825241073,0.987189825241073,0.987189825241073),(0.987189825241073,
0.987189825241073,0.987189825241073,0.987189825241073,0.987189825241073,
0.987189825241073,0.987189825241073,0.987189825241073,0.987189825241073,
0.987189825241073,0.987189825241073,0.987189825241073),(1.,1.,1.,1.,1.,
1.,1.,1.,1.,1.,1.,1.)))
REPRESENTATION_ITEM('')
SURFACE()
);
#580=(
BOUNDED_SURFACE()
B_SPLINE_SURFACE(3,3,((#36555,#36556,#36557,#36558,#36559,#36560,#36561,
#36562,#36563,#36564,#36565,#36566),(#36567,#36568,#36569,#36570,#36571,
#36572,#36573,#36574,#36575,#36576,#36577,#36578),(#36579,#36580,#36581,
#36582,#36583,#36584,#36585,#36586,#36587,#36588,#36589,#36590),(#36591,
#36592,#36593,#36594,#36595,#36596,#36597,#36598,#36599,#36600,#36601,#36602)),
 .UNSPECIFIED.,.F.,.F.,.F.)
B_SPLINE_SURFACE_WITH_KNOTS((4,4),(4,2,2,2,2,4),(0.,1.),(0.,0.0783698481609187,
0.30877738612019,0.539184924080125,0.769592462040063,1.),.UNSPECIFIED.)
GEOMETRIC_REPRESENTATION_ITEM()
RATIONAL_B_SPLINE_SURFACE(((1.,1.,1.,1.,1.,1.,1.,1.,1.,1.,1.,1.),(0.833333333333332,
0.833333333333332,0.833333333333332,0.833333333333332,0.833333333333332,
0.833333333333332,0.833333333333332,0.833333333333332,0.833333333333332,
0.833333333333332,0.833333333333332,0.833333333333332),(0.833333333333332,
0.833333333333332,0.833333333333332,0.833333333333332,0.833333333333332,
0.833333333333332,0.833333333333332,0.833333333333332,0.833333333333332,
0.833333333333332,0.833333333333332,0.833333333333332),(1.,1.,1.,1.,1.,
1.,1.,1.,1.,1.,1.,1.)))
REPRESENTATION_ITEM('')
SURFACE()
);
#581=(
BOUNDED_SURFACE()
B_SPLINE_SURFACE(3,3,((#36619,#36620,#36621,#36622,#36623,#36624,#36625,
#36626,#36627,#36628,#36629,#36630),(#36631,#36632,#36633,#36634,#36635,
#36636,#36637,#36638,#36639,#36640,#36641,#36642),(#36643,#36644,#36645,
#36646,#36647,#36648,#36649,#36650,#36651,#36652,#36653,#36654),(#36655,
#36656,#36657,#36658,#36659,#36660,#36661,#36662,#36663,#36664,#36665,#36666)),
 .UNSPECIFIED.,.F.,.F.,.F.)
B_SPLINE_SURFACE_WITH_KNOTS((4,4),(4,2,2,2,2,4),(0.,1.),(0.,0.0783698481609187,
0.30877738612019,0.539184924080125,0.769592462040063,1.),.UNSPECIFIED.)
GEOMETRIC_REPRESENTATION_ITEM()
RATIONAL_B_SPLINE_SURFACE(((1.,1.,1.,1.,1.,1.,1.,1.,1.,1.,1.,1.),(0.987189825241073,
0.987189825241073,0.987189825241073,0.987189825241073,0.987189825241073,
0.987189825241073,0.987189825241073,0.987189825241073,0.987189825241073,
0.987189825241073,0.987189825241073,0.987189825241073),(0.987189825241073,
0.987189825241073,0.987189825241073,0.987189825241073,0.987189825241073,
0.987189825241073,0.987189825241073,0.987189825241073,0.987189825241073,
0.987189825241073,0.987189825241073,0.987189825241073),(1.,1.,1.,1.,1.,
1.,1.,1.,1.,1.,1.,1.)))
REPRESENTATION_ITEM('')
SURFACE()
);
#582=(
BOUNDED_SURFACE()
B_SPLINE_SURFACE(3,3,((#36667,#36668,#36669,#36670,#36671,#36672,#36673,
#36674,#36675,#36676,#36677,#36678),(#36679,#36680,#36681,#36682,#36683,
#36684,#36685,#36686,#36687,#36688,#36689,#36690),(#36691,#36692,#36693,
#36694,#36695,#36696,#36697,#36698,#36699,#36700,#36701,#36702),(#36703,
#36704,#36705,#36706,#36707,#36708,#36709,#36710,#36711,#36712,#36713,#36714)),
 .UNSPECIFIED.,.F.,.F.,.F.)
B_SPLINE_SURFACE_WITH_KNOTS((4,4),(4,2,2,2,2,4),(0.,1.),(0.,0.0783698481609187,
0.30877738612019,0.539184924080125,0.769592462040063,1.),.UNSPECIFIED.)
GEOMETRIC_REPRESENTATION_ITEM()
RATIONAL_B_SPLINE_SURFACE(((1.,1.,1.,1.,1.,1.,1.,1.,1.,1.,1.,1.),(0.987189825241073,
0.987189825241073,0.987189825241073,0.987189825241073,0.987189825241073,
0.987189825241073,0.987189825241073,0.987189825241073,0.987189825241073,
0.987189825241073,0.987189825241073,0.987189825241073),(0.987189825241073,
0.987189825241073,0.987189825241073,0.987189825241073,0.987189825241073,
0.987189825241073,0.987189825241073,0.987189825241073,0.987189825241073,
0.987189825241073,0.987189825241073,0.987189825241073),(1.,1.,1.,1.,1.,
1.,1.,1.,1.,1.,1.,1.)))
REPRESENTATION_ITEM('')
SURFACE()
);
#583=(
BOUNDED_SURFACE()
B_SPLINE_SURFACE(3,3,((#36715,#36716,#36717,#36718,#36719,#36720,#36721,
#36722,#36723,#36724,#36725,#36726),(#36727,#36728,#36729,#36730,#36731,
#36732,#36733,#36734,#36735,#36736,#36737,#36738),(#36739,#36740,#36741,
#36742,#36743,#36744,#36745,#36746,#36747,#36748,#36749,#36750),(#36751,
#36752,#36753,#36754,#36755,#36756,#36757,#36758,#36759,#36760,#36761,#36762)),
 .UNSPECIFIED.,.F.,.F.,.F.)
B_SPLINE_SURFACE_WITH_KNOTS((4,4),(4,2,2,2,2,4),(0.,1.),(0.,0.0783698437311103,
0.308777382797833,0.539184921865221,0.76959246093261,1.),.UNSPECIFIED.)
GEOMETRIC_REPRESENTATION_ITEM()
RATIONAL_B_SPLINE_SURFACE(((1.,1.,1.,1.,1.,1.,1.,1.,1.,1.,1.,1.),(0.833333333333332,
0.833333333333332,0.833333333333332,0.833333333333332,0.833333333333332,
0.833333333333332,0.833333333333332,0.833333333333332,0.833333333333332,
0.833333333333332,0.833333333333332,0.833333333333332),(0.833333333333332,
0.833333333333332,0.833333333333332,0.833333333333332,0.833333333333332,
0.833333333333332,0.833333333333332,0.833333333333332,0.833333333333332,
0.833333333333332,0.833333333333332,0.833333333333332),(1.,1.,1.,1.,1.,
1.,1.,1.,1.,1.,1.,1.)))
REPRESENTATION_ITEM('')
SURFACE()
);
#584=(
BOUNDED_SURFACE()
B_SPLINE_SURFACE(3,3,((#36779,#36780,#36781,#36782,#36783,#36784,#36785,
#36786,#36787,#36788,#36789,#36790),(#36791,#36792,#36793,#36794,#36795,
#36796,#36797,#36798,#36799,#36800,#36801,#36802),(#36803,#36804,#36805,
#36806,#36807,#36808,#36809,#36810,#36811,#36812,#36813,#36814),(#36815,
#36816,#36817,#36818,#36819,#36820,#36821,#36822,#36823,#36824,#36825,#36826)),
 .UNSPECIFIED.,.F.,.F.,.F.)
B_SPLINE_SURFACE_WITH_KNOTS((4,4),(4,2,2,2,2,4),(0.,1.),(0.,0.0783698437311103,
0.308777382797833,0.539184921865221,0.76959246093261,1.),.UNSPECIFIED.)
GEOMETRIC_REPRESENTATION_ITEM()
RATIONAL_B_SPLINE_SURFACE(((1.,1.,1.,1.,1.,1.,1.,1.,1.,1.,1.,1.),(0.987189825241073,
0.987189825241073,0.987189825241073,0.987189825241073,0.987189825241073,
0.987189825241073,0.987189825241073,0.987189825241073,0.987189825241073,
0.987189825241073,0.987189825241073,0.987189825241073),(0.987189825241073,
0.987189825241073,0.987189825241073,0.987189825241073,0.987189825241073,
0.987189825241073,0.987189825241073,0.987189825241073,0.987189825241073,
0.987189825241073,0.987189825241073,0.987189825241073),(1.,1.,1.,1.,1.,
1.,1.,1.,1.,1.,1.,1.)))
REPRESENTATION_ITEM('')
SURFACE()
);
#585=(
BOUNDED_SURFACE()
B_SPLINE_SURFACE(3,3,((#36827,#36828,#36829,#36830,#36831,#36832,#36833,
#36834,#36835,#36836,#36837,#36838),(#36839,#36840,#36841,#36842,#36843,
#36844,#36845,#36846,#36847,#36848,#36849,#36850),(#36851,#36852,#36853,
#36854,#36855,#36856,#36857,#36858,#36859,#36860,#36861,#36862),(#36863,
#36864,#36865,#36866,#36867,#36868,#36869,#36870,#36871,#36872,#36873,#36874)),
 .UNSPECIFIED.,.F.,.F.,.F.)
B_SPLINE_SURFACE_WITH_KNOTS((4,4),(4,2,2,2,2,4),(0.,1.),(0.,0.0783698437311103,
0.308777382797833,0.539184921865221,0.76959246093261,1.),.UNSPECIFIED.)
GEOMETRIC_REPRESENTATION_ITEM()
RATIONAL_B_SPLINE_SURFACE(((1.,1.,1.,1.,1.,1.,1.,1.,1.,1.,1.,1.),(0.987189825241073,
0.987189825241073,0.987189825241073,0.987189825241073,0.987189825241073,
0.987189825241073,0.987189825241073,0.987189825241073,0.987189825241073,
0.987189825241073,0.987189825241073,0.987189825241073),(0.987189825241073,
0.987189825241073,0.987189825241073,0.987189825241073,0.987189825241073,
0.987189825241073,0.987189825241073,0.987189825241073,0.987189825241073,
0.987189825241073,0.987189825241073,0.987189825241073),(1.,1.,1.,1.,1.,
1.,1.,1.,1.,1.,1.,1.)))
REPRESENTATION_ITEM('')
SURFACE()
);
#586=(
BOUNDED_SURFACE()
B_SPLINE_SURFACE(3,3,((#36875,#36876,#36877,#36878,#36879,#36880,#36881,
#36882,#36883,#36884,#36885,#36886),(#36887,#36888,#36889,#36890,#36891,
#36892,#36893,#36894,#36895,#36896,#36897,#36898),(#36899,#36900,#36901,
#36902,#36903,#36904,#36905,#36906,#36907,#36908,#36909,#36910),(#36911,
#36912,#36913,#36914,#36915,#36916,#36917,#36918,#36919,#36920,#36921,#36922)),
 .UNSPECIFIED.,.F.,.F.,.F.)
B_SPLINE_SURFACE_WITH_KNOTS((4,4),(4,2,2,2,2,4),(0.,1.),(0.,0.0783698388401129,
0.308777379129585,0.539184919419723,0.769592459709861,1.),.UNSPECIFIED.)
GEOMETRIC_REPRESENTATION_ITEM()
RATIONAL_B_SPLINE_SURFACE(((1.,1.,1.,1.,1.,1.,1.,1.,1.,1.,1.,1.),(0.833333333333333,
0.833333333333333,0.833333333333333,0.833333333333333,0.833333333333333,
0.833333333333333,0.833333333333333,0.833333333333333,0.833333333333333,
0.833333333333333,0.833333333333333,0.833333333333333),(0.833333333333333,
0.833333333333333,0.833333333333333,0.833333333333333,0.833333333333333,
0.833333333333333,0.833333333333333,0.833333333333333,0.833333333333333,
0.833333333333333,0.833333333333333,0.833333333333333),(1.,1.,1.,1.,1.,
1.,1.,1.,1.,1.,1.,1.)))
REPRESENTATION_ITEM('')
SURFACE()
);
#587=(
BOUNDED_SURFACE()
B_SPLINE_SURFACE(3,3,((#36939,#36940,#36941,#36942,#36943,#36944,#36945,
#36946,#36947,#36948,#36949,#36950),(#36951,#36952,#36953,#36954,#36955,
#36956,#36957,#36958,#36959,#36960,#36961,#36962),(#36963,#36964,#36965,
#36966,#36967,#36968,#36969,#36970,#36971,#36972,#36973,#36974),(#36975,
#36976,#36977,#36978,#36979,#36980,#36981,#36982,#36983,#36984,#36985,#36986)),
 .UNSPECIFIED.,.F.,.F.,.F.)
B_SPLINE_SURFACE_WITH_KNOTS((4,4),(4,2,2,2,2,4),(0.,1.),(0.,0.0783698388401129,
0.308777379129585,0.539184919419723,0.769592459709861,1.),.UNSPECIFIED.)
GEOMETRIC_REPRESENTATION_ITEM()
RATIONAL_B_SPLINE_SURFACE(((1.,1.,1.,1.,1.,1.,1.,1.,1.,1.,1.,1.),(0.987189825241073,
0.987189825241073,0.987189825241073,0.987189825241073,0.987189825241073,
0.987189825241073,0.987189825241073,0.987189825241073,0.987189825241073,
0.987189825241073,0.987189825241073,0.987189825241073),(0.987189825241073,
0.987189825241073,0.987189825241073,0.987189825241073,0.987189825241073,
0.987189825241073,0.987189825241073,0.987189825241073,0.987189825241073,
0.987189825241073,0.987189825241073,0.987189825241073),(1.,1.,1.,1.,1.,
1.,1.,1.,1.,1.,1.,1.)))
REPRESENTATION_ITEM('')
SURFACE()
);
#588=(
BOUNDED_SURFACE()
B_SPLINE_SURFACE(3,3,((#36987,#36988,#36989,#36990,#36991,#36992,#36993,
#36994,#36995,#36996,#36997,#36998),(#36999,#37000,#37001,#37002,#37003,
#37004,#37005,#37006,#37007,#37008,#37009,#37010),(#37011,#37012,#37013,
#37014,#37015,#37016,#37017,#37018,#37019,#37020,#37021,#37022),(#37023,
#37024,#37025,#37026,#37027,#37028,#37029,#37030,#37031,#37032,#37033,#37034)),
 .UNSPECIFIED.,.F.,.F.,.F.)
B_SPLINE_SURFACE_WITH_KNOTS((4,4),(4,2,2,2,2,4),(0.,1.),(0.,0.0783698388401129,
0.308777379129585,0.539184919419723,0.769592459709861,1.),.UNSPECIFIED.)
GEOMETRIC_REPRESENTATION_ITEM()
RATIONAL_B_SPLINE_SURFACE(((1.,1.,1.,1.,1.,1.,1.,1.,1.,1.,1.,1.),(0.987189825241073,
0.987189825241073,0.987189825241073,0.987189825241073,0.987189825241073,
0.987189825241073,0.987189825241073,0.987189825241073,0.987189825241073,
0.987189825241073,0.987189825241073,0.987189825241073),(0.987189825241073,
0.987189825241073,0.987189825241073,0.987189825241073,0.987189825241073,
0.987189825241073,0.987189825241073,0.987189825241073,0.987189825241073,
0.987189825241073,0.987189825241073,0.987189825241073),(1.,1.,1.,1.,1.,
1.,1.,1.,1.,1.,1.,1.)))
REPRESENTATION_ITEM('')
SURFACE()
);
#589=(
BOUNDED_SURFACE()
B_SPLINE_SURFACE(3,3,((#37035,#37036,#37037,#37038,#37039,#37040,#37041,
#37042,#37043,#37044,#37045,#37046,#37047,#37048),(#37049,#37050,#37051,
#37052,#37053,#37054,#37055,#37056,#37057,#37058,#37059,#37060,#37061,#37062),
(#37063,#37064,#37065,#37066,#37067,#37068,#37069,#37070,#37071,#37072,
#37073,#37074,#37075,#37076),(#37077,#37078,#37079,#37080,#37081,#37082,
#37083,#37084,#37085,#37086,#37087,#37088,#37089,#37090)),.UNSPECIFIED.,
 .F.,.F.,.F.)
B_SPLINE_SURFACE_WITH_KNOTS((4,4),(4,2,2,2,2,2,4),(0.,1.),(0.,0.0183879232268686,
0.0783698352504293,0.308777376437322,0.53918491762488,0.769592458812441,
1.),.UNSPECIFIED.)
GEOMETRIC_REPRESENTATION_ITEM()
RATIONAL_B_SPLINE_SURFACE(((1.,1.,1.,1.,1.,1.,1.,1.,1.,1.,1.,1.,1.,1.),
(0.833333333333332,0.833333333333332,0.833333333333332,0.833333333333332,
0.833333333333332,0.833333333333332,0.833333333333332,0.833333333333332,
0.833333333333332,0.833333333333332,0.833333333333332,0.833333333333332,
0.833333333333332,0.833333333333332),(0.833333333333332,0.833333333333332,
0.833333333333332,0.833333333333332,0.833333333333332,0.833333333333332,
0.833333333333332,0.833333333333332,0.833333333333332,0.833333333333332,
0.833333333333332,0.833333333333332,0.833333333333332,0.833333333333332),
(1.,1.,1.,1.,1.,1.,1.,1.,1.,1.,1.,1.,1.,1.)))
REPRESENTATION_ITEM('')
SURFACE()
);
#590=(
BOUNDED_SURFACE()
B_SPLINE_SURFACE(3,3,((#37109,#37110,#37111,#37112,#37113,#37114,#37115,
#37116,#37117,#37118,#37119,#37120,#37121,#37122),(#37123,#37124,#37125,
#37126,#37127,#37128,#37129,#37130,#37131,#37132,#37133,#37134,#37135,#37136),
(#37137,#37138,#37139,#37140,#37141,#37142,#37143,#37144,#37145,#37146,
#37147,#37148,#37149,#37150),(#37151,#37152,#37153,#37154,#37155,#37156,
#37157,#37158,#37159,#37160,#37161,#37162,#37163,#37164)),.UNSPECIFIED.,
 .F.,.F.,.F.)
B_SPLINE_SURFACE_WITH_KNOTS((4,4),(4,2,2,2,2,2,4),(0.,1.),(0.,0.0183879232268686,
0.0783698352504293,0.308777376437322,0.53918491762488,0.769592458812441,
1.),.UNSPECIFIED.)
GEOMETRIC_REPRESENTATION_ITEM()
RATIONAL_B_SPLINE_SURFACE(((1.,1.,1.,1.,1.,1.,1.,1.,1.,1.,1.,1.,1.,1.),
(0.987189825241073,0.987189825241073,0.987189825241073,0.987189825241073,
0.987189825241073,0.987189825241073,0.987189825241073,0.987189825241073,
0.987189825241073,0.987189825241073,0.987189825241073,0.987189825241073,
0.987189825241073,0.987189825241073),(0.987189825241073,0.987189825241073,
0.987189825241073,0.987189825241073,0.987189825241073,0.987189825241073,
0.987189825241073,0.987189825241073,0.987189825241073,0.987189825241073,
0.987189825241073,0.987189825241073,0.987189825241073,0.987189825241073),
(1.,1.,1.,1.,1.,1.,1.,1.,1.,1.,1.,1.,1.,1.)))
REPRESENTATION_ITEM('')
SURFACE()
);
#591=(
BOUNDED_SURFACE()
B_SPLINE_SURFACE(3,3,((#37165,#37166,#37167,#37168,#37169,#37170,#37171,
#37172,#37173,#37174,#37175,#37176,#37177,#37178),(#37179,#37180,#37181,
#37182,#37183,#37184,#37185,#37186,#37187,#37188,#37189,#37190,#37191,#37192),
(#37193,#37194,#37195,#37196,#37197,#37198,#37199,#37200,#37201,#37202,
#37203,#37204,#37205,#37206),(#37207,#37208,#37209,#37210,#37211,#37212,
#37213,#37214,#37215,#37216,#37217,#37218,#37219,#37220)),.UNSPECIFIED.,
 .F.,.F.,.F.)
B_SPLINE_SURFACE_WITH_KNOTS((4,4),(4,2,2,2,2,2,4),(0.,1.),(0.,0.0183879232268686,
0.0783698352504293,0.308777376437322,0.53918491762488,0.769592458812441,
1.),.UNSPECIFIED.)
GEOMETRIC_REPRESENTATION_ITEM()
RATIONAL_B_SPLINE_SURFACE(((1.,1.,1.,1.,1.,1.,1.,1.,1.,1.,1.,1.,1.,1.),
(0.987189825241073,0.987189825241073,0.987189825241073,0.987189825241073,
0.987189825241073,0.987189825241073,0.987189825241073,0.987189825241073,
0.987189825241073,0.987189825241073,0.987189825241073,0.987189825241073,
0.987189825241073,0.987189825241073),(0.987189825241073,0.987189825241073,
0.987189825241073,0.987189825241073,0.987189825241073,0.987189825241073,
0.987189825241073,0.987189825241073,0.987189825241073,0.987189825241073,
0.987189825241073,0.987189825241073,0.987189825241073,0.987189825241073),
(1.,1.,1.,1.,1.,1.,1.,1.,1.,1.,1.,1.,1.,1.)))
REPRESENTATION_ITEM('')
SURFACE()
);
#594=CONICAL_SURFACE('',#11243,41.5,0.785398163397442);
#595=CONICAL_SURFACE('',#11292,43.5,0.78539816339745);
#617=B_SPLINE_CURVE_WITH_KNOTS('',3,(#17305,#17306,#17307,#17308,#17309,
#17310),.UNSPECIFIED.,.F.,.F.,(4,2,4),(-0.662095257781061,-0.331862946603713,
0.),.UNSPECIFIED.);
#618=B_SPLINE_CURVE_WITH_KNOTS('',3,(#17312,#17313,#17314,#17315,#17316,
#17317),.UNSPECIFIED.,.F.,.F.,(4,2,4),(-0.662021637365085,-0.331728159060927,
-1.00000001779232E-6),.UNSPECIFIED.);
#619=B_SPLINE_CURVE_WITH_KNOTS('',3,(#17321,#17322,#17323,#17324,#17325,
#17326,#17327,#17328,#17329,#17330,#17331,#17332,#17333,#17334),
 .UNSPECIFIED.,.F.,.F.,(4,2,2,2,2,2,4),(-0.662550701758967,-0.621305253814006,
-0.580038858839952,-0.497447618999927,-0.332066833308241,-0.165873822514336,
-1.00000000924361E-6),.UNSPECIFIED.);
#620=B_SPLINE_CURVE_WITH_KNOTS('',3,(#17336,#17337,#17338,#17339,#17340,
#17341),.UNSPECIFIED.,.F.,.F.,(4,2,4),(-0.663826635786988,-0.332807172053614,
-1.00000002301037E-6),.UNSPECIFIED.);
#621=B_SPLINE_CURVE_WITH_KNOTS('',3,(#17346,#17347,#17348,#17349,#17350,
#17351),.UNSPECIFIED.,.F.,.F.,(4,2,4),(-0.662095257781062,-0.33186294660371,
0.),.UNSPECIFIED.);
#622=B_SPLINE_CURVE_WITH_KNOTS('',3,(#17353,#17354,#17355,#17356,#17357,
#17358),.UNSPECIFIED.,.F.,.F.,(4,2,4),(-0.662021637522678,-0.331728159132817,
-1.00000001790335E-6),.UNSPECIFIED.);
#623=B_SPLINE_CURVE_WITH_KNOTS('',3,(#17362,#17363,#17364,#17365,#17366,
#17367,#17368,#17369,#17370,#17371,#17372,#17373,#17374,#17375),
 .UNSPECIFIED.,.F.,.F.,(4,2,2,2,2,2,4),(-0.662550616898668,-0.6212954808642,
-0.580019388663314,-0.49740872650569,-0.331989034460226,-0.165834990380567,
-1.0000000096877E-6),.UNSPECIFIED.);
#624=B_SPLINE_CURVE_WITH_KNOTS('',3,(#17377,#17378,#17379,#17380,#17381,
#17382),.UNSPECIFIED.,.F.,.F.,(4,2,4),(-0.663826635787034,-0.332807172053613,
-1.00000001879152E-6),.UNSPECIFIED.);
#625=B_SPLINE_CURVE_WITH_KNOTS('',3,(#17387,#17388,#17389,#17390,#17391,
#17392),.UNSPECIFIED.,.F.,.F.,(4,2,4),(-0.662095257781165,-0.331862946603753,
0.),.UNSPECIFIED.);
#626=B_SPLINE_CURVE_WITH_KNOTS('',3,(#17394,#17395,#17396,#17397,#17398,
#17399,#17400,#17401,#17402,#17403,#17404,#17405),.UNSPECIFIED.,.F.,.F.,
(4,2,2,2,2,4),(-0.660887316856551,-0.330884876596039,-0.165221392328677,
-0.0825519623367623,-0.0412673951611145,-9.99999991702083E-7),
 .UNSPECIFIED.);
#627=B_SPLINE_CURVE_WITH_KNOTS('',3,(#17409,#17410,#17411,#17412,#17413,
#17414,#17415,#17416,#17417,#17418,#17419,#17420,#17421,#17422),
 .UNSPECIFIED.,.F.,.F.,(4,2,2,2,2,2,4),(-0.662550616898348,-0.62129548086367,
-0.580019388662482,-0.497408726504859,-0.331989034460108,-0.165834990380633,
-1.00000000902156E-6),.UNSPECIFIED.);
#628=B_SPLINE_CURVE_WITH_KNOTS('',3,(#17424,#17425,#17426,#17427,#17428,
#17429),.UNSPECIFIED.,.F.,.F.,(4,2,4),(-0.663826635787024,-0.332807172053626,
-1.00000002301037E-6),.UNSPECIFIED.);
#629=B_SPLINE_CURVE_WITH_KNOTS('',3,(#17434,#17435,#17436,#17437,#17438,
#17439),.UNSPECIFIED.,.F.,.F.,(4,2,4),(-0.662095257781074,-0.331862946603717,
0.),.UNSPECIFIED.);
#630=B_SPLINE_CURVE_WITH_KNOTS('',3,(#17441,#17442,#17443,#17444,#17445,
#17446),.UNSPECIFIED.,.F.,.F.,(4,2,4),(-0.662021637922561,-0.331728159315548,
-1.00000001779232E-6),.UNSPECIFIED.);
#631=B_SPLINE_CURVE_WITH_KNOTS('',3,(#17450,#17451,#17452,#17453,#17454,
#17455,#17456,#17457),.UNSPECIFIED.,.F.,.F.,(4,2,2,4),(-0.663085280601993,
-0.331989035234756,-0.165834990767375,-1.00000000935463E-6),
 .UNSPECIFIED.);
#632=B_SPLINE_CURVE_WITH_KNOTS('',3,(#17459,#17460,#17461,#17462,#17463,
#17464),.UNSPECIFIED.,.F.,.F.,(4,2,4),(-0.663826635786995,-0.332807172053617,
-1.00000001901357E-6),.UNSPECIFIED.);
#633=B_SPLINE_CURVE_WITH_KNOTS('',3,(#17469,#17470,#17471,#17472,#17473,
#17474),.UNSPECIFIED.,.F.,.F.,(4,2,4),(-0.662095257781122,-0.33186294660374,
0.),.UNSPECIFIED.);
#634=B_SPLINE_CURVE_WITH_KNOTS('',3,(#17476,#17477,#17478,#17479,#17480,
#17481),.UNSPECIFIED.,.F.,.F.,(4,2,4),(-0.662021637998179,-0.331728159349608,
-1.0000000176813E-6),.UNSPECIFIED.);
#635=B_SPLINE_CURVE_WITH_KNOTS('',3,(#17485,#17486,#17487,#17488,#17489,
#17490,#17491,#17492,#17493,#17494,#17495,#17496,#17497,#17498),
 .UNSPECIFIED.,.F.,.F.,(4,2,2,2,2,2,4),(-0.662550616895752,-0.621295480861997,
-0.580019388660938,-0.497408726503312,-0.331989034459601,-0.165834990381051,
-1.00000000891054E-6),.UNSPECIFIED.);
#636=B_SPLINE_CURVE_WITH_KNOTS('',3,(#17500,#17501,#17502,#17503,#17504,
#17505),.UNSPECIFIED.,.F.,.F.,(4,2,4),(-0.663826635786914,-0.332807172053552,
-1.00000002090095E-6),.UNSPECIFIED.);
#637=B_SPLINE_CURVE_WITH_KNOTS('',3,(#17510,#17511,#17512,#17513,#17514,
#17515),.UNSPECIFIED.,.F.,.F.,(4,2,4),(-0.662095257781135,-0.331862946603749,
0.),.UNSPECIFIED.);
#638=B_SPLINE_CURVE_WITH_KNOTS('',3,(#17517,#17518,#17519,#17520,#17521,
#17522),.UNSPECIFIED.,.F.,.F.,(4,2,4),(-0.662021637997819,-0.331728159349464,
-1.0000000176813E-6),.UNSPECIFIED.);
#639=B_SPLINE_CURVE_WITH_KNOTS('',3,(#17526,#17527,#17528,#17529,#17530,
#17531,#17532,#17533,#17534,#17535,#17536,#17537,#17538,#17539),
 .UNSPECIFIED.,.F.,.F.,(4,2,2,2,2,2,4),(-0.66255061689952,-0.62129548086583,
-0.58001938866469,-0.497408726506779,-0.331989034460727,-0.165834990380612,
-1.00000000902156E-6),.UNSPECIFIED.);
#640=B_SPLINE_CURVE_WITH_KNOTS('',3,(#17541,#17542,#17543,#17544,#17545,
#17546),.UNSPECIFIED.,.F.,.F.,(4,2,4),(-0.663826635787004,-0.332807172053617,
-1.0000000216781E-6),.UNSPECIFIED.);
#641=B_SPLINE_CURVE_WITH_KNOTS('',3,(#17551,#17552,#17553,#17554,#17555,
#17556),.UNSPECIFIED.,.F.,.F.,(4,2,4),(-0.662095257781009,-0.331862946603692,
0.),.UNSPECIFIED.);
#642=B_SPLINE_CURVE_WITH_KNOTS('',3,(#17558,#17559,#17560,#17561,#17562,
#17563),.UNSPECIFIED.,.F.,.F.,(4,2,4),(-0.662021637880972,-0.331728159296021,
-1.0000000176813E-6),.UNSPECIFIED.);
#643=B_SPLINE_CURVE_WITH_KNOTS('',3,(#17567,#17568,#17569,#17570,#17571,
#17572,#17573,#17574,#17575,#17576,#17577,#17578,#17579,#17580),
 .UNSPECIFIED.,.F.,.F.,(4,2,2,2,2,2,4),(-0.66255061689857,-0.621295480864233,
-0.580019388662843,-0.497408726505221,-0.331989034460455,-0.165834990380495,
-1.00000000813338E-6),.UNSPECIFIED.);
#644=B_SPLINE_CURVE_WITH_KNOTS('',3,(#17582,#17583,#17584,#17585,#17586,
#17587),.UNSPECIFIED.,.F.,.F.,(4,2,4),(-0.66382663578703,-0.332807172053612,
-1.00000001945766E-6),.UNSPECIFIED.);
#645=B_SPLINE_CURVE_WITH_KNOTS('',3,(#17592,#17593,#17594,#17595,#17596,
#17597),.UNSPECIFIED.,.F.,.F.,(4,2,4),(-0.66209525778118,-0.331862946603774,
0.),.UNSPECIFIED.);
#646=B_SPLINE_CURVE_WITH_KNOTS('',3,(#17599,#17600,#17601,#17602,#17603,
#17604),.UNSPECIFIED.,.F.,.F.,(4,2,4),(-0.662021637714287,-0.331728159220456,
-1.00000001745926E-6),.UNSPECIFIED.);
#647=B_SPLINE_CURVE_WITH_KNOTS('',3,(#17608,#17609,#17610,#17611,#17612,
#17613,#17614,#17615,#17616,#17617,#17618,#17619,#17620,#17621),
 .UNSPECIFIED.,.F.,.F.,(4,2,2,2,2,2,4),(-0.662550616897935,-0.621295480863862,
-0.580019388662615,-0.497408726505072,-0.331989034460079,-0.16583499038102,
-1.00000000979872E-6),.UNSPECIFIED.);
#648=B_SPLINE_CURVE_WITH_KNOTS('',3,(#17623,#17624,#17625,#17626,#17627,
#17628),.UNSPECIFIED.,.F.,.F.,(4,2,4),(-0.663826635787039,-0.332807172053655,
-1.00000002345446E-6),.UNSPECIFIED.);
#649=B_SPLINE_CURVE_WITH_KNOTS('',3,(#17633,#17634,#17635,#17636,#17637,
#17638),.UNSPECIFIED.,.F.,.F.,(4,2,4),(-0.662095257781127,-0.331862946603734,
0.),.UNSPECIFIED.);
#650=B_SPLINE_CURVE_WITH_KNOTS('',3,(#17640,#17641,#17642,#17643,#17644,
#17645),.UNSPECIFIED.,.F.,.F.,(4,2,4),(-0.66202163751964,-0.331728159131613,
-1.00000001790335E-6),.UNSPECIFIED.);
#651=B_SPLINE_CURVE_WITH_KNOTS('',3,(#17649,#17650,#17651,#17652,#17653,
#17654,#17655,#17656,#17657,#17658,#17659,#17660,#17661,#17662),
 .UNSPECIFIED.,.F.,.F.,(4,2,2,2,2,2,4),(-0.662550616899407,-0.621295480865396,
-0.580019388664292,-0.497408726506504,-0.33198903446057,-0.165834990380615,
-1.00000000791134E-6),.UNSPECIFIED.);
#652=B_SPLINE_CURVE_WITH_KNOTS('',3,(#17664,#17665,#17666,#17667,#17668,
#17669),.UNSPECIFIED.,.F.,.F.,(4,2,4),(-0.66382663578689,-0.332807172053566,
-1.00000002201117E-6),.UNSPECIFIED.);
#653=B_SPLINE_CURVE_WITH_KNOTS('',3,(#17674,#17675,#17676,#17677,#17678,
#17679),.UNSPECIFIED.,.F.,.F.,(4,2,4),(-0.662095257781152,-0.331862946603746,
0.),.UNSPECIFIED.);
#654=B_SPLINE_CURVE_WITH_KNOTS('',3,(#17681,#17682,#17683,#17684,#17685,
#17686),.UNSPECIFIED.,.F.,.F.,(4,2,4),(-0.662021637368216,-0.331728159062471,
-1.00000001779232E-6),.UNSPECIFIED.);
#655=B_SPLINE_CURVE_WITH_KNOTS('',3,(#17690,#17691,#17692,#17693,#17694,
#17695,#17696,#17697,#17698,#17699,#17700,#17701,#17702,#17703),
 .UNSPECIFIED.,.F.,.F.,(4,2,2,2,2,2,4),(-0.662550616898824,-0.621295480864527,
-0.580019388663592,-0.497408726505791,-0.331989034460403,-0.165834990380775,
-1.00000000935463E-6),.UNSPECIFIED.);
#656=B_SPLINE_CURVE_WITH_KNOTS('',3,(#17705,#17706,#17707,#17708,#17709,
#17710),.UNSPECIFIED.,.F.,.F.,(4,2,4),(-0.663826635787064,-0.332807172053641,
-1.0000000216781E-6),.UNSPECIFIED.);
#657=B_SPLINE_CURVE_WITH_KNOTS('',3,(#17715,#17716,#17717,#17718,#17719,
#17720),.UNSPECIFIED.,.F.,.F.,(4,2,4),(-0.662095257781144,-0.331862946603761,
0.),.UNSPECIFIED.);
#658=B_SPLINE_CURVE_WITH_KNOTS('',3,(#17722,#17723,#17724,#17725,#17726,
#17727),.UNSPECIFIED.,.F.,.F.,(4,2,4),(-0.662021637123029,-0.331728158950561,
-1.00000001779232E-6),.UNSPECIFIED.);
#659=B_SPLINE_CURVE_WITH_KNOTS('',3,(#17731,#17732,#17733,#17734,#17735,
#17736,#17737,#17738,#17739,#17740,#17741,#17742,#17743,#17744),
 .UNSPECIFIED.,.F.,.F.,(4,2,2,2,2,2,4),(-0.662550616899271,-0.621295480864664,
-0.580019388663568,-0.497408726505942,-0.331989034460324,-0.165834990380964,
-1.00000000957667E-6),.UNSPECIFIED.);
#660=B_SPLINE_CURVE_WITH_KNOTS('',3,(#17746,#17747,#17748,#17749,#17750,
#17751),.UNSPECIFIED.,.F.,.F.,(4,2,4),(-0.663826635786987,-0.332807172053595,
-1.00000002278833E-6),.UNSPECIFIED.);
#661=B_SPLINE_CURVE_WITH_KNOTS('',3,(#17756,#17757,#17758,#17759,#17760,
#17761),.UNSPECIFIED.,.F.,.F.,(4,2,4),(-0.662095257780937,-0.331862946603657,
0.),.UNSPECIFIED.);
#662=B_SPLINE_CURVE_WITH_KNOTS('',3,(#17763,#17764,#17765,#17766,#17767,
#17768,#17769,#17770,#17771,#17772,#17773,#17774),.UNSPECIFIED.,.F.,.F.,
(4,2,2,2,2,4),(-0.660887316879566,-0.330884876607085,-0.165221392333038,
-0.0825519623381546,-0.0412673951613865,-9.99999991702083E-7),
 .UNSPECIFIED.);
#663=B_SPLINE_CURVE_WITH_KNOTS('',3,(#17778,#17779,#17780,#17781,#17782,
#17783,#17784,#17785,#17786,#17787,#17788,#17789,#17790,#17791),
 .UNSPECIFIED.,.F.,.F.,(4,2,2,2,2,2,4),(-0.662550616900091,-0.621295480865225,
-0.580019388664242,-0.497408726506713,-0.331989034460346,-0.165834990380543,
-1.00000000913258E-6),.UNSPECIFIED.);
#664=B_SPLINE_CURVE_WITH_KNOTS('',3,(#17793,#17794,#17795,#17796,#17797,
#17798),.UNSPECIFIED.,.F.,.F.,(4,2,4),(-0.663826635786934,-0.332807172053606,
-1.00000002178913E-6),.UNSPECIFIED.);
#665=B_SPLINE_CURVE_WITH_KNOTS('',3,(#17803,#17804,#17805,#17806,#17807,
#17808),.UNSPECIFIED.,.F.,.F.,(4,2,4),(-0.662095257781237,-0.331862946603812,
0.),.UNSPECIFIED.);
#666=B_SPLINE_CURVE_WITH_KNOTS('',3,(#17810,#17811,#17812,#17813,#17814,
#17815),.UNSPECIFIED.,.F.,.F.,(4,2,4),(-0.662021637516076,-0.331728159129799,
-1.00000001790335E-6),.UNSPECIFIED.);
#667=B_SPLINE_CURVE_WITH_KNOTS('',3,(#17819,#17820,#17821,#17822,#17823,
#17824,#17825,#17826),.UNSPECIFIED.,.F.,.F.,(4,2,2,4),(-0.663085280603729,
-0.331989035234337,-0.165834990767195,-1.00000000924361E-6),
 .UNSPECIFIED.);
#668=B_SPLINE_CURVE_WITH_KNOTS('',3,(#17828,#17829,#17830,#17831,#17832,
#17833),.UNSPECIFIED.,.F.,.F.,(4,2,4),(-0.663826635786952,-0.332807172053596,
-1.00000002356548E-6),.UNSPECIFIED.);
#669=B_SPLINE_CURVE_WITH_KNOTS('',3,(#17838,#17839,#17840,#17841,#17842,
#17843),.UNSPECIFIED.,.F.,.F.,(4,2,4),(-0.662095257781154,-0.331862946603771,
0.),.UNSPECIFIED.);
#670=B_SPLINE_CURVE_WITH_KNOTS('',3,(#17845,#17846,#17847,#17848,#17849,
#17850),.UNSPECIFIED.,.F.,.F.,(4,2,4),(-0.662021613149805,-0.331771295733496,
-1.0000000176813E-6),.UNSPECIFIED.);
#671=B_SPLINE_CURVE_WITH_KNOTS('',3,(#17854,#17855,#17856,#17857,#17858,
#17859,#17860,#17861,#17862,#17863,#17864,#17865,#17866,#17867),
 .UNSPECIFIED.,.F.,.F.,(4,2,2,2,2,2,4),(-0.662550616898987,-0.621295480864932,
-0.580019388664009,-0.497408726506264,-0.331989034460189,-0.165834990380972,
-1.00000000990974E-6),.UNSPECIFIED.);
#672=B_SPLINE_CURVE_WITH_KNOTS('',3,(#17869,#17870,#17871,#17872,#17873,
#17874),.UNSPECIFIED.,.F.,.F.,(4,2,4),(-0.663826635786919,-0.332807172053578,
-1.00000002312139E-6),.UNSPECIFIED.);
#673=B_SPLINE_CURVE_WITH_KNOTS('',3,(#17879,#17880,#17881,#17882,#17883,
#17884),.UNSPECIFIED.,.F.,.F.,(4,2,4),(-0.662095257781154,-0.331862946603728,
0.),.UNSPECIFIED.);
#674=B_SPLINE_CURVE_WITH_KNOTS('',3,(#17886,#17887,#17888,#17889,#17890,
#17891),.UNSPECIFIED.,.F.,.F.,(4,2,4),(-0.662021613337153,-0.331771296170992,
-1.00000001779232E-6),.UNSPECIFIED.);
#675=B_SPLINE_CURVE_WITH_KNOTS('',3,(#17895,#17896,#17897,#17898,#17899,
#17900,#17901,#17902,#17903,#17904,#17905,#17906,#17907,#17908),
 .UNSPECIFIED.,.F.,.F.,(4,2,2,2,2,2,4),(-0.662550701757792,-0.621305253813084,
-0.580038858838667,-0.497447618998446,-0.332066833308196,-0.165873822514761,
-1.00000000857747E-6),.UNSPECIFIED.);
#676=B_SPLINE_CURVE_WITH_KNOTS('',3,(#17910,#17911,#17912,#17913,#17914,
#17915),.UNSPECIFIED.,.F.,.F.,(4,2,4),(-0.66382663578696,-0.332807172053593,
-1.00000002312139E-6),.UNSPECIFIED.);
#677=B_SPLINE_CURVE_WITH_KNOTS('',3,(#17920,#17921,#17922,#17923,#17924,
#17925),.UNSPECIFIED.,.F.,.F.,(4,2,4),(-0.662095257781059,-0.331862946603702,
0.),.UNSPECIFIED.);
#678=B_SPLINE_CURVE_WITH_KNOTS('',3,(#17927,#17928,#17929,#17930,#17931,
#17932),.UNSPECIFIED.,.F.,.F.,(4,2,4),(-0.662021613440326,-0.331771295866445,
-1.00000001779232E-6),.UNSPECIFIED.);
#679=B_SPLINE_CURVE_WITH_KNOTS('',3,(#17936,#17937,#17938,#17939,#17940,
#17941,#17942,#17943,#17944,#17945,#17946,#17947,#17948,#17949),
 .UNSPECIFIED.,.F.,.F.,(4,2,2,2,2,2,4),(-0.662550701758225,-0.621305253856284,
-0.580038858924235,-0.497447619168591,-0.332066833647734,-0.165873822684014,
-1.00000000935463E-6),.UNSPECIFIED.);
#680=B_SPLINE_CURVE_WITH_KNOTS('',3,(#17951,#17952,#17953,#17954,#17955,
#17956),.UNSPECIFIED.,.F.,.F.,(4,2,4),(-0.663826635787033,-0.332807172053606,
-1.00000002256628E-6),.UNSPECIFIED.);
#681=B_SPLINE_CURVE_WITH_KNOTS('',3,(#17961,#17962,#17963,#17964,#17965,
#17966),.UNSPECIFIED.,.F.,.F.,(4,2,4),(-0.662095257781069,-0.331862946603717,
0.),.UNSPECIFIED.);
#682=B_SPLINE_CURVE_WITH_KNOTS('',3,(#17968,#17969,#17970,#17971,#17972,
#17973),.UNSPECIFIED.,.F.,.F.,(4,2,4),(-0.662021613427598,-0.331771295860329,
-1.00000001779232E-6),.UNSPECIFIED.);
#683=B_SPLINE_CURVE_WITH_KNOTS('',3,(#17977,#17978,#17979,#17980,#17981,
#17982,#17983,#17984,#17985,#17986,#17987,#17988,#17989,#17990),
 .UNSPECIFIED.,.F.,.F.,(4,2,2,2,2,2,4),(-0.662550701754713,-0.621305253810719,
-0.580038858836423,-0.497447618996478,-0.332066833307539,-0.165873822514765,
-1.00000000891054E-6),.UNSPECIFIED.);
#684=B_SPLINE_CURVE_WITH_KNOTS('',3,(#17992,#17993,#17994,#17995,#17996,
#17997),.UNSPECIFIED.,.F.,.F.,(4,2,4),(-0.663826635786997,-0.332807172053604,
-1.00000002267731E-6),.UNSPECIFIED.);
#685=B_SPLINE_CURVE_WITH_KNOTS('',3,(#18002,#18003,#18004,#18005,#18006,
#18007),.UNSPECIFIED.,.F.,.F.,(4,2,4),(-0.662095257781134,-0.331862946603725,
0.),.UNSPECIFIED.);
#686=B_SPLINE_CURVE_WITH_KNOTS('',3,(#18009,#18010,#18011,#18012,#18013,
#18014),.UNSPECIFIED.,.F.,.F.,(4,2,4),(-0.662021613339374,-0.331771295819707,
-1.00000001779232E-6),.UNSPECIFIED.);
#687=B_SPLINE_CURVE_WITH_KNOTS('',3,(#18018,#18019,#18020,#18021,#18022,
#18023,#18024,#18025,#18026,#18027,#18028,#18029,#18030,#18031),
 .UNSPECIFIED.,.F.,.F.,(4,2,2,2,2,2,4),(-0.662550701759283,-0.62130525381475,
-0.580038858840059,-0.49744761899971,-0.332066833308656,-0.165873822514787,
-1.00000000924361E-6),.UNSPECIFIED.);
#688=B_SPLINE_CURVE_WITH_KNOTS('',3,(#18033,#18034,#18035,#18036,#18037,
#18038),.UNSPECIFIED.,.F.,.F.,(4,2,4),(-0.663826635787049,-0.332807172053624,
-1.00000002012379E-6),.UNSPECIFIED.);
#689=B_SPLINE_CURVE_WITH_KNOTS('',3,(#18043,#18044,#18045,#18046,#18047,
#18048),.UNSPECIFIED.,.F.,.F.,(4,2,4),(-0.662095257776738,-0.331862946601972,
0.),.UNSPECIFIED.);
#690=B_SPLINE_CURVE_WITH_KNOTS('',3,(#18050,#18051,#18052,#18053,#18054,
#18055),.UNSPECIFIED.,.F.,.F.,(4,2,4),(-0.662021613160614,-0.331771295738581,
-1.00000001823641E-6),.UNSPECIFIED.);
#691=B_SPLINE_CURVE_WITH_KNOTS('',3,(#18059,#18060,#18061,#18062,#18063,
#18064,#18065,#18066,#18067,#18068,#18069,#18070,#18071,#18072),
 .UNSPECIFIED.,.F.,.F.,(4,2,2,2,2,2,4),(-0.662550701758829,-0.621305253813552,
-0.580038858838592,-0.497447618998373,-0.332066833308538,-0.165873822514955,
-1.00000000724521E-6),.UNSPECIFIED.);
#692=B_SPLINE_CURVE_WITH_KNOTS('',3,(#18074,#18075,#18076,#18077,#18078,
#18079),.UNSPECIFIED.,.F.,.F.,(4,2,4),(-0.663826635786964,-0.332807172053598,
-1.00000002323242E-6),.UNSPECIFIED.);
#693=B_SPLINE_CURVE_WITH_KNOTS('',3,(#18084,#18085,#18086,#18087,#18088,
#18089),.UNSPECIFIED.,.F.,.F.,(4,2,4),(-0.662095257781233,-0.331862946603775,
0.),.UNSPECIFIED.);
#694=B_SPLINE_CURVE_WITH_KNOTS('',3,(#18091,#18092,#18093,#18094,#18095,
#18096),.UNSPECIFIED.,.F.,.F.,(4,2,4),(-0.662021612957221,-0.331771295645616,
-1.00000001779232E-6),.UNSPECIFIED.);
#695=B_SPLINE_CURVE_WITH_KNOTS('',3,(#18100,#18101,#18102,#18103,#18104,
#18105,#18106,#18107,#18108,#18109,#18110,#18111,#18112,#18113),
 .UNSPECIFIED.,.F.,.F.,(4,2,2,2,2,2,4),(-0.662550701757299,-0.621305253812781,
-0.580038858838426,-0.497447618998266,-0.332066833308142,-0.165873822514797,
-1.00000000835543E-6),.UNSPECIFIED.);
#696=B_SPLINE_CURVE_WITH_KNOTS('',3,(#18115,#18116,#18117,#18118,#18119,
#18120),.UNSPECIFIED.,.F.,.F.,(4,2,4),(-0.663826635786982,-0.332807172053603,
-1.00000002223322E-6),.UNSPECIFIED.);
#697=B_SPLINE_CURVE_WITH_KNOTS('',3,(#18125,#18126,#18127,#18128,#18129,
#18130),.UNSPECIFIED.,.F.,.F.,(4,2,4),(-0.662095257781211,-0.331862946603789,
0.),.UNSPECIFIED.);
#698=B_SPLINE_CURVE_WITH_KNOTS('',3,(#18132,#18133,#18134,#18135,#18136,
#18137),.UNSPECIFIED.,.F.,.F.,(4,2,4),(-0.662021612815302,-0.331771295581121,
-1.00000001779232E-6),.UNSPECIFIED.);
#699=B_SPLINE_CURVE_WITH_KNOTS('',3,(#18141,#18142,#18143,#18144,#18145,
#18146,#18147,#18148,#18149,#18150,#18151,#18152,#18153,#18154),
 .UNSPECIFIED.,.F.,.F.,(4,2,2,2,2,2,4),(-0.662550701758534,-0.621305253813699,
-0.580038858839343,-0.497447618999118,-0.33206683330838,-0.165873822514653,
-1.00000000935463E-6),.UNSPECIFIED.);
#700=B_SPLINE_CURVE_WITH_KNOTS('',3,(#18156,#18157,#18158,#18159,#18160,
#18161),.UNSPECIFIED.,.F.,.F.,(4,2,4),(-0.663826635786954,-0.332807172053568,
-1.00000001945766E-6),.UNSPECIFIED.);
#701=B_SPLINE_CURVE_WITH_KNOTS('',3,(#18166,#18167,#18168,#18169,#18170,
#18171),.UNSPECIFIED.,.F.,.F.,(4,2,4),(-0.662095257781192,-0.331862946603769,
0.),.UNSPECIFIED.);
#702=B_SPLINE_CURVE_WITH_KNOTS('',3,(#18173,#18174,#18175,#18176,#18177,
#18178),.UNSPECIFIED.,.F.,.F.,(4,2,4),(-0.662021612558326,-0.331771295463796,
-1.00000001779232E-6),.UNSPECIFIED.);
#703=B_SPLINE_CURVE_WITH_KNOTS('',3,(#18182,#18183,#18184,#18185,#18186,
#18187,#18188,#18189,#18190,#18191,#18192,#18193,#18194,#18195),
 .UNSPECIFIED.,.F.,.F.,(4,2,2,2,2,2,4),(-0.662550701759507,-0.621305253814335,
-0.580038858839854,-0.497447618999759,-0.332066833308242,-0.165873822514247,
-1.00000001002076E-6),.UNSPECIFIED.);
#704=B_SPLINE_CURVE_WITH_KNOTS('',3,(#18197,#18198,#18199,#18200,#18201,
#18202),.UNSPECIFIED.,.F.,.F.,(4,2,4),(-0.663826635787048,-0.332807172053641,
-1.00000002123402E-6),.UNSPECIFIED.);
#705=B_SPLINE_CURVE_WITH_KNOTS('',3,(#18207,#18208,#18209,#18210,#18211,
#18212),.UNSPECIFIED.,.F.,.F.,(4,2,4),(-0.662095257781137,-0.331862946603746,
0.),.UNSPECIFIED.);
#706=B_SPLINE_CURVE_WITH_KNOTS('',3,(#18214,#18215,#18216,#18217,#18218,
#18219),.UNSPECIFIED.,.F.,.F.,(4,2,4),(-0.662021612804876,-0.331771295576207,
-1.0000000176813E-6),.UNSPECIFIED.);
#707=B_SPLINE_CURVE_WITH_KNOTS('',3,(#18223,#18224,#18225,#18226,#18227,
#18228,#18229,#18230,#18231,#18232,#18233,#18234,#18235,#18236),
 .UNSPECIFIED.,.F.,.F.,(4,2,2,2,2,2,4),(-0.662550701759088,-0.621305253814185,
-0.580038858840118,-0.497447619000064,-0.332066833308297,-0.165873822514322,
-1.000000006246E-6),.UNSPECIFIED.);
#708=B_SPLINE_CURVE_WITH_KNOTS('',3,(#18238,#18239,#18240,#18241,#18242,
#18243),.UNSPECIFIED.,.F.,.F.,(4,2,4),(-0.663826635786971,-0.332807172053609,
-1.00000002334344E-6),.UNSPECIFIED.);
#709=B_SPLINE_CURVE_WITH_KNOTS('',3,(#18248,#18249,#18250,#18251,#18252,
#18253),.UNSPECIFIED.,.F.,.F.,(4,2,4),(-0.662095257781061,-0.331862946603719,
0.),.UNSPECIFIED.);
#710=B_SPLINE_CURVE_WITH_KNOTS('',3,(#18255,#18256,#18257,#18258,#18259,
#18260),.UNSPECIFIED.,.F.,.F.,(4,2,4),(-0.662021612957974,-0.33177129564596,
-1.00000001779232E-6),.UNSPECIFIED.);
#711=B_SPLINE_CURVE_WITH_KNOTS('',3,(#18264,#18265,#18266,#18267,#18268,
#18269,#18270,#18271,#18272,#18273,#18274,#18275,#18276,#18277),
 .UNSPECIFIED.,.F.,.F.,(4,2,2,2,2,2,4),(-0.66255070175906,-0.621305253814359,
-0.580038858840127,-0.49744761899987,-0.332066833308326,-0.165873822514433,
-1.0000000086885E-6),.UNSPECIFIED.);
#712=B_SPLINE_CURVE_WITH_KNOTS('',3,(#18279,#18280,#18281,#18282,#18283,
#18284),.UNSPECIFIED.,.F.,.F.,(4,2,4),(-0.663826635786987,-0.332807172053615,
-1.00000002101197E-6),.UNSPECIFIED.);
#713=B_SPLINE_CURVE_WITH_KNOTS('',3,(#18289,#18290,#18291,#18292,#18293,
#18294),.UNSPECIFIED.,.F.,.F.,(4,2,4),(-0.662095257781128,-0.331862946603748,
0.),.UNSPECIFIED.);
#714=B_SPLINE_CURVE_WITH_KNOTS('',3,(#18296,#18297,#18298,#18299,#18300,
#18301,#18302,#18303,#18304,#18305,#18306,#18307),.UNSPECIFIED.,.F.,.F.,
(4,2,2,2,2,4),(-0.660887065044359,-0.330927753205643,-0.165242782459234,
-0.0825626423163793,-0.0412727318856715,-9.99999991702083E-7),
 .UNSPECIFIED.);
#715=B_SPLINE_CURVE_WITH_KNOTS('',3,(#18311,#18312,#18313,#18314,#18315,
#18316,#18317,#18318,#18319,#18320,#18321,#18322,#18323,#18324),
 .UNSPECIFIED.,.F.,.F.,(4,2,2,2,2,2,4),(-0.662550701758423,-0.621305253813834,
-0.580038858839635,-0.49744761899939,-0.332066833308269,-0.165873822514469,
-1.00000000746725E-6),.UNSPECIFIED.);
#716=B_SPLINE_CURVE_WITH_KNOTS('',3,(#18326,#18327,#18328,#18329,#18330,
#18331),.UNSPECIFIED.,.F.,.F.,(4,2,4),(-0.663826635787052,-0.332807172053646,
-1.00000002023481E-6),.UNSPECIFIED.);
#717=B_SPLINE_CURVE_WITH_KNOTS('',3,(#18336,#18337,#18338,#18339,#18340,
#18341),.UNSPECIFIED.,.F.,.F.,(4,2,4),(-0.662095257781141,-0.331862946603758,
0.),.UNSPECIFIED.);
#718=B_SPLINE_CURVE_WITH_KNOTS('',3,(#18343,#18344,#18345,#18346,#18347,
#18348,#18349,#18350,#18351,#18352,#18353,#18354),.UNSPECIFIED.,.F.,.F.,
(4,2,2,2,2,4),(-0.660887065033929,-0.330927753200197,-0.165242782456535,
-0.0825626423149307,-0.0412727318851053,-9.99999991591061E-7),
 .UNSPECIFIED.);
#719=B_SPLINE_CURVE_WITH_KNOTS('',3,(#18358,#18359,#18360,#18361,#18362,
#18363,#18364,#18365),.UNSPECIFIED.,.F.,.F.,(4,2,2,4),(-0.663084973284213,
-0.332066834082123,-0.165873822900741,-1.00000000902156E-6),
 .UNSPECIFIED.);
#720=B_SPLINE_CURVE_WITH_KNOTS('',3,(#18367,#18368,#18369,#18370,#18371,
#18372),.UNSPECIFIED.,.F.,.F.,(4,2,4),(-0.663826635787002,-0.332807172053626,
-1.0000000206789E-6),.UNSPECIFIED.);
#721=B_SPLINE_CURVE_WITH_KNOTS('',3,(#18377,#18378,#18379,#18380,#18381,
#18382),.UNSPECIFIED.,.F.,.F.,(4,2,4),(-0.662095257781032,-0.331862946603718,
0.),.UNSPECIFIED.);
#722=B_SPLINE_CURVE_WITH_KNOTS('',3,(#18384,#18385,#18386,#18387,#18388,
#18389),.UNSPECIFIED.,.F.,.F.,(4,2,4),(-0.662021613431922,-0.331771295862448,
-1.00000001779232E-6),.UNSPECIFIED.);
#723=B_SPLINE_CURVE_WITH_KNOTS('',3,(#18393,#18394,#18395,#18396,#18397,
#18398,#18399,#18400),.UNSPECIFIED.,.F.,.F.,(4,2,2,4),(-0.663084973280964,
-0.332066834082069,-0.165873822901686,-1.00000000935463E-6),
 .UNSPECIFIED.);
#724=B_SPLINE_CURVE_WITH_KNOTS('',3,(#18402,#18403,#18404,#18405,#18406,
#18407),.UNSPECIFIED.,.F.,.F.,(4,2,4),(-0.663826635787037,-0.33280717205365,
-1.00000002334344E-6),.UNSPECIFIED.);
#725=B_SPLINE_CURVE_WITH_KNOTS('',3,(#18412,#18413,#18414,#18415,#18416,
#18417),.UNSPECIFIED.,.F.,.F.,(4,2,4),(-0.662095257781131,-0.331862946603741,
0.),.UNSPECIFIED.);
#726=B_SPLINE_CURVE_WITH_KNOTS('',3,(#18419,#18420,#18421,#18422,#18423,
#18424),.UNSPECIFIED.,.F.,.F.,(4,2,4),(-0.662021613430381,-0.331771295861564,
-1.00000001779232E-6),.UNSPECIFIED.);
#727=B_SPLINE_CURVE_WITH_KNOTS('',3,(#18428,#18429,#18430,#18431,#18432,
#18433,#18434,#18435,#18436,#18437,#18438,#18439,#18440,#18441),
 .UNSPECIFIED.,.F.,.F.,(4,2,2,2,2,2,4),(-0.662550701756468,-0.62130525381211,
-0.580038858837624,-0.497447618997602,-0.332066833307905,-0.165873822514476,
-1.00000000846645E-6),.UNSPECIFIED.);
#728=B_SPLINE_CURVE_WITH_KNOTS('',3,(#18443,#18444,#18445,#18446,#18447,
#18448),.UNSPECIFIED.,.F.,.F.,(4,2,4),(-0.663826635787072,-0.332807172053659,
-1.00000002223322E-6),.UNSPECIFIED.);
#729=B_SPLINE_CURVE_WITH_KNOTS('',3,(#18453,#18454,#18455,#18456,#18457,
#18458),.UNSPECIFIED.,.F.,.F.,(4,2,4),(-0.662095257781099,-0.331862946603744,
0.),.UNSPECIFIED.);
#730=B_SPLINE_CURVE_WITH_KNOTS('',3,(#18460,#18461,#18462,#18463,#18464,
#18465),.UNSPECIFIED.,.F.,.F.,(4,2,4),(-0.662021613329726,-0.331771295815806,
-1.00000001779232E-6),.UNSPECIFIED.);
#731=B_SPLINE_CURVE_WITH_KNOTS('',3,(#18469,#18470,#18471,#18472,#18473,
#18474,#18475,#18476,#18477,#18478,#18479,#18480,#18481,#18482),
 .UNSPECIFIED.,.F.,.F.,(4,2,2,2,2,2,4),(-0.662550701757085,-0.621305253812491,
-0.580038858837846,-0.497447618997816,-0.332066833308107,-0.165873822514721,
-1.00000000857747E-6),.UNSPECIFIED.);
#732=B_SPLINE_CURVE_WITH_KNOTS('',3,(#18484,#18485,#18486,#18487,#18488,
#18489),.UNSPECIFIED.,.F.,.F.,(4,2,4),(-0.663826635787016,-0.332807172053633,
-1.00000002301037E-6),.UNSPECIFIED.);
#733=B_SPLINE_CURVE_WITH_KNOTS('',3,(#18494,#18495,#18496,#18497,#18498,
#18499),.UNSPECIFIED.,.F.,.F.,(4,2,4),(-0.662095257776784,-0.331862946602006,
0.),.UNSPECIFIED.);
#734=B_SPLINE_CURVE_WITH_KNOTS('',3,(#18501,#18502,#18503,#18504,#18505,
#18506),.UNSPECIFIED.,.F.,.F.,(4,2,4),(-0.662021613154439,-0.331771295735777,
-1.00000001712619E-6),.UNSPECIFIED.);
#735=B_SPLINE_CURVE_WITH_KNOTS('',3,(#18510,#18511,#18512,#18513,#18514,
#18515,#18516,#18517,#18518,#18519,#18520,#18521,#18522,#18523),
 .UNSPECIFIED.,.F.,.F.,(4,2,2,2,2,2,4),(-0.662550701757146,-0.621305253812992,
-0.580038858838693,-0.497447618998531,-0.332066833308134,-0.165873822514585,
-1.00000000902156E-6),.UNSPECIFIED.);
#736=B_SPLINE_CURVE_WITH_KNOTS('',3,(#18525,#18526,#18527,#18528,#18529,
#18530),.UNSPECIFIED.,.F.,.F.,(4,2,4),(-0.663826635786971,-0.332807172053601,
-1.00000002234424E-6),.UNSPECIFIED.);
#737=B_SPLINE_CURVE_WITH_KNOTS('',3,(#18535,#18536,#18537,#18538,#18539,
#18540),.UNSPECIFIED.,.F.,.F.,(4,2,4),(-0.662095257781007,-0.331862946603684,
0.),.UNSPECIFIED.);
#738=B_SPLINE_CURVE_WITH_KNOTS('',3,(#18542,#18543,#18544,#18545,#18546,
#18547),.UNSPECIFIED.,.F.,.F.,(4,2,4),(-0.662021612957012,-0.331771295645723,
-1.00000001779232E-6),.UNSPECIFIED.);
#739=B_SPLINE_CURVE_WITH_KNOTS('',3,(#18551,#18552,#18553,#18554,#18555,
#18556,#18557,#18558,#18559,#18560,#18561,#18562,#18563,#18564),
 .UNSPECIFIED.,.F.,.F.,(4,2,2,2,2,2,4),(-0.66255070175672,-0.621305253812282,
-0.58003885883802,-0.497447618998075,-0.332066833307935,-0.165873822514331,
-1.00000000913258E-6),.UNSPECIFIED.);
#740=B_SPLINE_CURVE_WITH_KNOTS('',3,(#18566,#18567,#18568,#18569,#18570,
#18571),.UNSPECIFIED.,.F.,.F.,(4,2,4),(-0.663826635786866,-0.332807172053519,
-1.00000002145606E-6),.UNSPECIFIED.);
#741=B_SPLINE_CURVE_WITH_KNOTS('',3,(#18576,#18577,#18578,#18579,#18580,
#18581),.UNSPECIFIED.,.F.,.F.,(4,2,4),(-0.662095306120118,-0.331830781965298,
0.),.UNSPECIFIED.);
#742=B_SPLINE_CURVE_WITH_KNOTS('',3,(#18583,#18584,#18585,#18586,#18587,
#18588),.UNSPECIFIED.,.F.,.F.,(4,2,4),(-0.662021612806063,-0.331771295576848,
-1.00000001779232E-6),.UNSPECIFIED.);
#743=B_SPLINE_CURVE_WITH_KNOTS('',3,(#18592,#18593,#18594,#18595,#18596,
#18597,#18598,#18599,#18600,#18601,#18602,#18603,#18604,#18605),
 .UNSPECIFIED.,.F.,.F.,(4,2,2,2,2,2,4),(-0.662550701758247,-0.621305253813676,
-0.580038858839485,-0.497447618999181,-0.332066833308307,-0.165873822514554,
-1.00000000902156E-6),.UNSPECIFIED.);
#744=B_SPLINE_CURVE_WITH_KNOTS('',3,(#18607,#18608,#18609,#18610,#18611,
#18612),.UNSPECIFIED.,.F.,.F.,(4,2,4),(-0.663826635786942,-0.332807172053572,
-1.00000002056788E-6),.UNSPECIFIED.);
#745=B_SPLINE_CURVE_WITH_KNOTS('',3,(#18617,#18618,#18619,#18620,#18621,
#18622),.UNSPECIFIED.,.F.,.F.,(4,2,4),(-0.66209530612013,-0.331830781965309,
0.),.UNSPECIFIED.);
#746=B_SPLINE_CURVE_WITH_KNOTS('',3,(#18624,#18625,#18626,#18627,#18628,
#18629,#18630,#18631,#18632,#18633,#18634,#18635),.UNSPECIFIED.,.F.,.F.,
(4,2,2,2,2,4),(-0.66088706502341,-0.330927753195277,-0.165242782452955,
-0.0825626423128806,-0.0412727318841083,-9.99999991702083E-7),
 .UNSPECIFIED.);
#747=B_SPLINE_CURVE_WITH_KNOTS('',3,(#18639,#18640,#18641,#18642,#18643,
#18644,#18645,#18646,#18647,#18648,#18649,#18650,#18651,#18652),
 .UNSPECIFIED.,.F.,.F.,(4,2,2,2,2,2,4),(-0.662550701758955,-0.621305253813872,
-0.580038858839428,-0.497447618999422,-0.332066833308222,-0.165873822514119,
-1.00000001013179E-6),.UNSPECIFIED.);
#748=B_SPLINE_CURVE_WITH_KNOTS('',3,(#18654,#18655,#18656,#18657,#18658,
#18659),.UNSPECIFIED.,.F.,.F.,(4,2,4),(-0.66382655429936,-0.332732370051042,
-1.00000002123402E-6),.UNSPECIFIED.);
#749=B_SPLINE_CURVE_WITH_KNOTS('',3,(#18664,#18665,#18666,#18667,#18668,
#18669),.UNSPECIFIED.,.F.,.F.,(4,2,4),(-0.662095306120191,-0.33183078196534,
0.),.UNSPECIFIED.);
#750=B_SPLINE_CURVE_WITH_KNOTS('',3,(#18671,#18672,#18673,#18674,#18675,
#18676,#18677,#18678,#18679,#18680,#18681,#18682),.UNSPECIFIED.,.F.,.F.,
(4,2,2,2,2,4),(-0.66088706502611,-0.330927753196476,-0.165242782453738,
-0.0825626423132116,-0.0412727318842448,-9.99999991702083E-7),
 .UNSPECIFIED.);
#751=B_SPLINE_CURVE_WITH_KNOTS('',3,(#18686,#18687,#18688,#18689,#18690,
#18691,#18692,#18693),.UNSPECIFIED.,.F.,.F.,(4,2,2,4),(-0.663084973282026,
-0.332066834082184,-0.165873822900691,-1.00000000946565E-6),
 .UNSPECIFIED.);
#752=B_SPLINE_CURVE_WITH_KNOTS('',3,(#18695,#18696,#18697,#18698,#18699,
#18700),.UNSPECIFIED.,.F.,.F.,(4,2,4),(-0.663826554299285,-0.332732370051009,
-1.0000000216781E-6),.UNSPECIFIED.);
#753=B_SPLINE_CURVE_WITH_KNOTS('',3,(#18705,#18706,#18707,#18708,#18709,
#18710),.UNSPECIFIED.,.F.,.F.,(4,2,4),(-0.662095306120128,-0.331830781965308,
0.),.UNSPECIFIED.);
#754=B_SPLINE_CURVE_WITH_KNOTS('',3,(#18712,#18713,#18714,#18715,#18716,
#18717),.UNSPECIFIED.,.F.,.F.,(4,2,4),(-0.662021612958496,-0.331771295646342,
-1.00000001779232E-6),.UNSPECIFIED.);
#755=B_SPLINE_CURVE_WITH_KNOTS('',3,(#18721,#18722,#18723,#18724,#18725,
#18726,#18727,#18728),.UNSPECIFIED.,.F.,.F.,(4,2,2,4),(-0.663084973281183,
-0.332066834082057,-0.165873822900902,-1.00000000935463E-6),
 .UNSPECIFIED.);
#756=B_SPLINE_CURVE_WITH_KNOTS('',3,(#18730,#18731,#18732,#18733,#18734,
#18735),.UNSPECIFIED.,.F.,.F.,(4,2,4),(-0.663826554299325,-0.332732370051047,
-1.00000002256628E-6),.UNSPECIFIED.);
#757=B_SPLINE_CURVE_WITH_KNOTS('',3,(#18740,#18741,#18742,#18743,#18744,
#18745),.UNSPECIFIED.,.F.,.F.,(4,2,4),(-0.662095306120064,-0.331830781965281,
0.),.UNSPECIFIED.);
#758=B_SPLINE_CURVE_WITH_KNOTS('',3,(#18747,#18748,#18749,#18750,#18751,
#18752),.UNSPECIFIED.,.F.,.F.,(4,2,4),(-0.662021613146791,-0.331771295731921,
-1.00000001679312E-6),.UNSPECIFIED.);
#759=B_SPLINE_CURVE_WITH_KNOTS('',3,(#18756,#18757,#18758,#18759,#18760,
#18761,#18762,#18763,#18764,#18765,#18766,#18767,#18768,#18769),
 .UNSPECIFIED.,.F.,.F.,(4,2,2,2,2,2,4),(-0.662550701759488,-0.621305253814721,
-0.580038858840412,-0.497447619000151,-0.332066833308525,-0.165873822514555,
-1.00000000902156E-6),.UNSPECIFIED.);
#760=B_SPLINE_CURVE_WITH_KNOTS('',3,(#18771,#18772,#18773,#18774,#18775,
#18776),.UNSPECIFIED.,.F.,.F.,(4,2,4),(-0.663826554299435,-0.332732370051088,
-1.00000001990175E-6),.UNSPECIFIED.);
#761=B_SPLINE_CURVE_WITH_KNOTS('',3,(#18781,#18782,#18783,#18784,#18785,
#18786),.UNSPECIFIED.,.F.,.F.,(4,2,4),(-0.662095306120062,-0.331830781965283,
0.),.UNSPECIFIED.);
#762=B_SPLINE_CURVE_WITH_KNOTS('',3,(#18788,#18789,#18790,#18791,#18792,
#18793),.UNSPECIFIED.,.F.,.F.,(4,2,4),(-0.662021613347664,-0.331771296175878,
-1.00000001779232E-6),.UNSPECIFIED.);
#763=B_SPLINE_CURVE_WITH_KNOTS('',3,(#18797,#18798,#18799,#18800,#18801,
#18802,#18803,#18804,#18805,#18806,#18807,#18808,#18809,#18810),
 .UNSPECIFIED.,.F.,.F.,(4,2,2,2,2,2,4),(-0.662550701760095,-0.621305253815354,
-0.580038858840818,-0.497447619000533,-0.332066833308807,-0.165873822514148,
-1.00000001002076E-6),.UNSPECIFIED.);
#764=B_SPLINE_CURVE_WITH_KNOTS('',3,(#18812,#18813,#18814,#18815,#18816,
#18817),.UNSPECIFIED.,.F.,.F.,(4,2,4),(-0.663826554299384,-0.332732370051052,
-1.00000002145606E-6),.UNSPECIFIED.);
#765=B_SPLINE_CURVE_WITH_KNOTS('',3,(#18822,#18823,#18824,#18825,#18826,
#18827),.UNSPECIFIED.,.F.,.F.,(4,2,4),(-0.662095306120294,-0.33183078196538,
0.),.UNSPECIFIED.);
#766=B_SPLINE_CURVE_WITH_KNOTS('',3,(#18829,#18830,#18831,#18832,#18833,
#18834),.UNSPECIFIED.,.F.,.F.,(4,2,4),(-0.662021613433192,-0.331771295862689,
-1.00000001779232E-6),.UNSPECIFIED.);
#767=B_SPLINE_CURVE_WITH_KNOTS('',3,(#18838,#18839,#18840,#18841,#18842,
#18843,#18844,#18845,#18846,#18847,#18848,#18849,#18850,#18851),
 .UNSPECIFIED.,.F.,.F.,(4,2,2,2,2,2,4),(-0.662550701758329,-0.621305253855782,
-0.580038858923311,-0.497447619167824,-0.332066833647579,-0.1658738226846,
-1.00000000935463E-6),.UNSPECIFIED.);
#768=B_SPLINE_CURVE_WITH_KNOTS('',3,(#18853,#18854,#18855,#18856,#18857,
#18858),.UNSPECIFIED.,.F.,.F.,(4,2,4),(-0.663826554299397,-0.33273237005105,
-1.00000002078993E-6),.UNSPECIFIED.);
#769=B_SPLINE_CURVE_WITH_KNOTS('',3,(#18863,#18864,#18865,#18866,#18867,
#18868),.UNSPECIFIED.,.F.,.F.,(4,2,4),(-0.662095306120216,-0.331830781965384,
0.),.UNSPECIFIED.);
#770=B_SPLINE_CURVE_WITH_KNOTS('',3,(#18870,#18871,#18872,#18873,#18874,
#18875),.UNSPECIFIED.,.F.,.F.,(4,2,4),(-0.662021613436443,-0.3317712958642,
-1.0000000176813E-6),.UNSPECIFIED.);
#771=B_SPLINE_CURVE_WITH_KNOTS('',3,(#18879,#18880,#18881,#18882,#18883,
#18884,#18885,#18886,#18887,#18888,#18889,#18890,#18891,#18892),
 .UNSPECIFIED.,.F.,.F.,(4,2,2,2,2,2,4),(-0.662550701759013,-0.621305253814237,
-0.580038858839444,-0.497447618999241,-0.332066833308602,-0.165873822514864,
-1.00000000702316E-6),.UNSPECIFIED.);
#772=B_SPLINE_CURVE_WITH_KNOTS('',3,(#18894,#18895,#18896,#18897,#18898,
#18899),.UNSPECIFIED.,.F.,.F.,(4,2,4),(-0.663826554299459,-0.3327323700511,
-1.00000002112299E-6),.UNSPECIFIED.);
#773=B_SPLINE_CURVE_WITH_KNOTS('',3,(#18904,#18905,#18906,#18907,#18908,
#18909),.UNSPECIFIED.,.F.,.F.,(4,2,4),(-0.662095306120087,-0.331830781965296,
0.),.UNSPECIFIED.);
#774=B_SPLINE_CURVE_WITH_KNOTS('',3,(#18911,#18912,#18913,#18914,#18915,
#18916),.UNSPECIFIED.,.F.,.F.,(4,2,4),(-0.662021613343284,-0.33177129582197,
-1.00000001790335E-6),.UNSPECIFIED.);
#775=B_SPLINE_CURVE_WITH_KNOTS('',3,(#18920,#18921,#18922,#18923,#18924,
#18925,#18926,#18927,#18928,#18929,#18930,#18931,#18932,#18933),
 .UNSPECIFIED.,.F.,.F.,(4,2,2,2,2,2,4),(-0.662550701758145,-0.621305253812989,
-0.580038858838031,-0.497447618997672,-0.33206683330843,-0.165873822514873,
-1.0000000086885E-6),.UNSPECIFIED.);
#776=B_SPLINE_CURVE_WITH_KNOTS('',3,(#18935,#18936,#18937,#18938,#18939,
#18940),.UNSPECIFIED.,.F.,.F.,(4,2,4),(-0.663826554299388,-0.332732370051057,
-1.00000002101197E-6),.UNSPECIFIED.);
#777=B_SPLINE_CURVE_WITH_KNOTS('',3,(#18945,#18946,#18947,#18948,#18949,
#18950),.UNSPECIFIED.,.F.,.F.,(4,2,4),(-0.662095306120114,-0.331830781965322,
0.),.UNSPECIFIED.);
#778=B_SPLINE_CURVE_WITH_KNOTS('',3,(#18952,#18953,#18954,#18955,#18956,
#18957),.UNSPECIFIED.,.F.,.F.,(4,2,4),(-0.662021613164074,-0.331771295740365,
-1.00000001790335E-6),.UNSPECIFIED.);
#779=B_SPLINE_CURVE_WITH_KNOTS('',3,(#18961,#18962,#18963,#18964,#18965,
#18966,#18967,#18968,#18969,#18970,#18971,#18972,#18973,#18974),
 .UNSPECIFIED.,.F.,.F.,(4,2,2,2,2,2,4),(-0.662550701755705,-0.62130525381069,
-0.580038858835955,-0.497447618995727,-0.332066833307856,-0.165873822515044,
-1.00000000857747E-6),.UNSPECIFIED.);
#780=B_SPLINE_CURVE_WITH_KNOTS('',3,(#18976,#18977,#18978,#18979,#18980,
#18981),.UNSPECIFIED.,.F.,.F.,(4,2,4),(-0.663826554299419,-0.332732370051075,
-1.00000002234424E-6),.UNSPECIFIED.);
#781=B_SPLINE_CURVE_WITH_KNOTS('',3,(#18986,#18987,#18988,#18989,#18990,
#18991),.UNSPECIFIED.,.F.,.F.,(4,2,4),(-0.662095306120204,-0.331830781965362,
0.),.UNSPECIFIED.);
#782=B_SPLINE_CURVE_WITH_KNOTS('',3,(#18993,#18994,#18995,#18996,#18997,
#18998),.UNSPECIFIED.,.F.,.F.,(4,2,4),(-0.662021612967814,-0.33177129565058,
-1.00000001779232E-6),.UNSPECIFIED.);
#783=B_SPLINE_CURVE_WITH_KNOTS('',3,(#19002,#19003,#19004,#19005,#19006,
#19007,#19008,#19009,#19010,#19011,#19012,#19013,#19014,#19015),
 .UNSPECIFIED.,.F.,.F.,(4,2,2,2,2,2,4),(-0.662550701757928,-0.621305253812802,
-0.58003885883804,-0.497447618997713,-0.332066833308205,-0.165873822515039,
-1.00000000768929E-6),.UNSPECIFIED.);
#784=B_SPLINE_CURVE_WITH_KNOTS('',3,(#19017,#19018,#19019,#19020,#19021,
#19022),.UNSPECIFIED.,.F.,.F.,(4,2,4),(-0.663826554299339,-0.332732370051032,
-1.00000002134504E-6),.UNSPECIFIED.);
#785=B_SPLINE_CURVE_WITH_KNOTS('',3,(#19027,#19028,#19029,#19030,#19031,
#19032),.UNSPECIFIED.,.F.,.F.,(4,2,4),(-0.662095257781194,-0.331862946603777,
0.),.UNSPECIFIED.);
#786=B_SPLINE_CURVE_WITH_KNOTS('',3,(#19034,#19035,#19036,#19037,#19038,
#19039),.UNSPECIFIED.,.F.,.F.,(4,2,4),(-0.662021612558349,-0.331771295463814,
-1.00000001779232E-6),.UNSPECIFIED.);
#787=B_SPLINE_CURVE_WITH_KNOTS('',3,(#19043,#19044,#19045,#19046,#19047,
#19048,#19049,#19050),.UNSPECIFIED.,.F.,.F.,(4,2,2,4),(-0.663084973281713,
-0.332066834082423,-0.165873822900929,-1.00000000924361E-6),
 .UNSPECIFIED.);
#788=B_SPLINE_CURVE_WITH_KNOTS('',3,(#19052,#19053,#19054,#19055,#19056,
#19057),.UNSPECIFIED.,.F.,.F.,(4,2,4),(-0.663826554299392,-0.332732370051039,
-1.00000002034584E-6),.UNSPECIFIED.);
#789=B_SPLINE_CURVE_WITH_KNOTS('',3,(#19062,#19063,#19064,#19065,#19066,
#19067),.UNSPECIFIED.,.F.,.F.,(4,2,4),(-0.662095306115713,-0.331830781963555,
0.),.UNSPECIFIED.);
#790=B_SPLINE_CURVE_WITH_KNOTS('',3,(#19069,#19070,#19071,#19072,#19073,
#19074,#19075,#19076,#19077,#19078,#19079,#19080),.UNSPECIFIED.,.F.,.F.,
(4,2,2,2,2,4),(-0.660887065032632,-0.330927753199737,-0.165242782455574,
-0.0825626423141882,-0.0412727318846662,-9.99999991702083E-7),
 .UNSPECIFIED.);
#791=B_SPLINE_CURVE_WITH_KNOTS('',3,(#19084,#19085,#19086,#19087,#19088,
#19089,#19090,#19091,#19092,#19093,#19094,#19095,#19096,#19097),
 .UNSPECIFIED.,.F.,.F.,(4,2,2,2,2,2,4),(-0.662550701759551,-0.621305253814749,
-0.58003885884035,-0.497447619000075,-0.332066833308522,-0.1658738225146,
-1.00000000924361E-6),.UNSPECIFIED.);
#792=B_SPLINE_CURVE_WITH_KNOTS('',3,(#19099,#19100,#19101,#19102,#19103,
#19104),.UNSPECIFIED.,.F.,.F.,(4,2,4),(-0.663826554299404,-0.332732370051068,
-1.00000002223322E-6),.UNSPECIFIED.);
#793=B_SPLINE_CURVE_WITH_KNOTS('',3,(#19109,#19110,#19111,#19112,#19113,
#19114,#19115,#19116,#19117,#19118,#19119,#19120),.UNSPECIFIED.,.F.,.F.,
(4,2,2,2,2,4),(-0.260520203475784,-0.209083280006074,-0.154198547441575,
-0.0839662032252584,-0.0407463936727428,0.),.UNSPECIFIED.);
#794=B_SPLINE_CURVE_WITH_KNOTS('',3,(#19122,#19123,#19124,#19125,#19126,
#19127,#19128),.UNSPECIFIED.,.F.,.F.,(4,3,4),(0.,0.000879527967505091,0.00156997524832468),
 .UNSPECIFIED.);
#795=B_SPLINE_CURVE_WITH_KNOTS('',3,(#19132,#19133,#19134,#19135,#19136,
#19137,#19138),.UNSPECIFIED.,.F.,.F.,(4,3,4),(9.85133562538035E-18,0.000871555184780974,
0.00160565474757454),.UNSPECIFIED.);
#796=B_SPLINE_CURVE_WITH_KNOTS('',3,(#19140,#19141,#19142,#19143,#19144,
#19145,#19146,#19147,#19148,#19149),.UNSPECIFIED.,.F.,.F.,(4,2,2,2,4),(-0.260724731519921,
-0.199727802453949,-0.13039083565756,-0.0610645770444107,0.),
 .UNSPECIFIED.);
#797=B_SPLINE_CURVE_WITH_KNOTS('',3,(#19151,#19152,#19153,#19154,#19155,
#19156,#19157),.UNSPECIFIED.,.F.,.F.,(4,3,4),(0.,0.000879527967506278,0.00156997524832335),
 .UNSPECIFIED.);
#798=B_SPLINE_CURVE_WITH_KNOTS('',3,(#19161,#19162,#19163,#19164,#19165,
#19166,#19167),.UNSPECIFIED.,.F.,.F.,(4,3,4),(2.22159771539451E-16,0.000871555185133579,
0.0016056547475732),.UNSPECIFIED.);
#799=B_SPLINE_CURVE_WITH_KNOTS('',3,(#19169,#19170,#19171,#19172,#19173,
#19174,#19175,#19176,#19177,#19178),.UNSPECIFIED.,.F.,.F.,(4,2,2,2,4),(-0.260724731516474,
-0.199727802451461,-0.130390835656149,-0.0610645770440664,0.),
 .UNSPECIFIED.);
#800=B_SPLINE_CURVE_WITH_KNOTS('',3,(#19180,#19181,#19182,#19183,#19184,
#19185,#19186),.UNSPECIFIED.,.F.,.F.,(4,3,4),(0.,0.000879527967497252,0.00156997524832199),
 .UNSPECIFIED.);
#801=B_SPLINE_CURVE_WITH_KNOTS('',3,(#19190,#19191,#19192,#19193,#19194,
#19195,#19196),.UNSPECIFIED.,.F.,.F.,(4,3,4),(3.46944695195361E-18,0.000871555184780109,
0.00160565474757182),.UNSPECIFIED.);
#802=B_SPLINE_CURVE_WITH_KNOTS('',3,(#19198,#19199,#19200,#19201,#19202,
#19203,#19204,#19205,#19206,#19207),.UNSPECIFIED.,.F.,.F.,(4,2,2,2,4),(-0.260724731519922,
-0.199727802453945,-0.130390835657557,-0.0610645770444094,0.),
 .UNSPECIFIED.);
#803=B_SPLINE_CURVE_WITH_KNOTS('',3,(#19209,#19210,#19211,#19212,#19213,
#19214,#19215),.UNSPECIFIED.,.F.,.F.,(4,3,4),(0.,0.000879527967508083,0.00156997524832066),
 .UNSPECIFIED.);
#804=B_SPLINE_CURVE_WITH_KNOTS('',3,(#19219,#19220,#19221,#19222,#19223,
#19224,#19225),.UNSPECIFIED.,.F.,.F.,(4,3,4),(9.34177181294034E-18,0.000871555184785609,
0.00160565474757049),.UNSPECIFIED.);
#805=B_SPLINE_CURVE_WITH_KNOTS('',3,(#19227,#19228,#19229,#19230,#19231,
#19232,#19233,#19234,#19235,#19236),.UNSPECIFIED.,.F.,.F.,(4,2,2,2,4),(-0.260724731519973,
-0.199727802453985,-0.130390835657586,-0.0610645770444184,0.),
 .UNSPECIFIED.);
#806=B_SPLINE_CURVE_WITH_KNOTS('',3,(#19238,#19239,#19240,#19241,#19242,
#19243,#19244),.UNSPECIFIED.,.F.,.F.,(4,3,4),(0.,0.000879527967501964,0.00156997524831932),
 .UNSPECIFIED.);
#807=B_SPLINE_CURVE_WITH_KNOTS('',3,(#19248,#19249,#19250,#19251,#19252,
#19253,#19254),.UNSPECIFIED.,.F.,.F.,(4,3,4),(1.73472347597681E-18,0.00087155518477886,
0.00160565474756914),.UNSPECIFIED.);
#808=B_SPLINE_CURVE_WITH_KNOTS('',3,(#19256,#19257,#19258,#19259,#19260,
#19261,#19262,#19263,#19264,#19265),.UNSPECIFIED.,.F.,.F.,(4,2,2,2,4),(-0.260724731519937,
-0.199727802453964,-0.130390835657569,-0.0610645770444118,0.),
 .UNSPECIFIED.);
#809=B_SPLINE_CURVE_WITH_KNOTS('',3,(#19267,#19268,#19269,#19270,#19271,
#19272,#19273),.UNSPECIFIED.,.F.,.F.,(4,3,4),(0.,0.000879527967645649,0.00156997524831794),
 .UNSPECIFIED.);
#810=B_SPLINE_CURVE_WITH_KNOTS('',3,(#19277,#19278,#19279,#19280,#19281,
#19282,#19283),.UNSPECIFIED.,.F.,.F.,(4,3,4),(2.01474521574067E-16,0.000871555185129347,
0.00160565474756778),.UNSPECIFIED.);
#811=B_SPLINE_CURVE_WITH_KNOTS('',3,(#19285,#19286,#19287,#19288,#19289,
#19290,#19291,#19292,#19293,#19294),.UNSPECIFIED.,.F.,.F.,(4,2,2,2,4),(-0.260724731516495,
-0.199727802451476,-0.130390835656153,-0.0610645770440646,0.),
 .UNSPECIFIED.);
#812=B_SPLINE_CURVE_WITH_KNOTS('',3,(#19296,#19297,#19298,#19299,#19300,
#19301,#19302),.UNSPECIFIED.,.F.,.F.,(4,3,4),(0.,0.000879527967509314,0.00156997524831662),
 .UNSPECIFIED.);
#813=B_SPLINE_CURVE_WITH_KNOTS('',3,(#19306,#19307,#19308,#19309,#19310,
#19311,#19312),.UNSPECIFIED.,.F.,.F.,(4,3,4),(1.56125112837913E-17,0.000871555184791312,
0.00160565474756646),.UNSPECIFIED.);
#814=B_SPLINE_CURVE_WITH_KNOTS('',3,(#19314,#19315,#19316,#19317,#19318,
#19319,#19320,#19321,#19322,#19323),.UNSPECIFIED.,.F.,.F.,(4,2,2,2,4),(-0.260724731519916,
-0.199727802453943,-0.130390835657558,-0.0610645770444119,0.),
 .UNSPECIFIED.);
#815=B_SPLINE_CURVE_WITH_KNOTS('',3,(#19325,#19326,#19327,#19328,#19329,
#19330,#19331),.UNSPECIFIED.,.F.,.F.,(4,3,4),(0.,0.000879527967500359,0.00156997524831529),
 .UNSPECIFIED.);
#816=B_SPLINE_CURVE_WITH_KNOTS('',3,(#19335,#19336,#19337,#19338,#19339,
#19340,#19341),.UNSPECIFIED.,.F.,.F.,(4,3,4),(1.4304896245382E-17,0.000871555184787351,
0.0016056547475651),.UNSPECIFIED.);
#817=B_SPLINE_CURVE_WITH_KNOTS('',3,(#19343,#19344,#19345,#19346,#19347,
#19348,#19349,#19350,#19351,#19352),.UNSPECIFIED.,.F.,.F.,(4,2,2,2,4),(-0.260724731519916,
-0.199727802453942,-0.130390835657559,-0.0610645770444123,0.),
 .UNSPECIFIED.);
#818=B_SPLINE_CURVE_WITH_KNOTS('',3,(#19354,#19355,#19356,#19357,#19358,
#19359,#19360),.UNSPECIFIED.,.F.,.F.,(4,3,4),(0.,0.000879527967502405,0.00156997524831393),
 .UNSPECIFIED.);
#819=B_SPLINE_CURVE_WITH_KNOTS('',3,(#19364,#19365,#19366,#19367,#19368,
#19369,#19370),.UNSPECIFIED.,.F.,.F.,(4,3,4),(1.04083408558608E-17,0.000871555184779143,
0.00160565474756374),.UNSPECIFIED.);
#820=B_SPLINE_CURVE_WITH_KNOTS('',3,(#19372,#19373,#19374,#19375,#19376,
#19377,#19378,#19379,#19380,#19381),.UNSPECIFIED.,.F.,.F.,(4,2,2,2,4),(-0.260724731519971,
-0.199727802453984,-0.130390835657585,-0.061064577044418,0.),
 .UNSPECIFIED.);
#821=B_SPLINE_CURVE_WITH_KNOTS('',3,(#19383,#19384,#19385,#19386,#19387,
#19388,#19389),.UNSPECIFIED.,.F.,.F.,(4,3,4),(0.,0.000879527967498967,0.00156997524831261),
 .UNSPECIFIED.);
#822=B_SPLINE_CURVE_WITH_KNOTS('',3,(#19393,#19394,#19395,#19396,#19397,
#19398,#19399),.UNSPECIFIED.,.F.,.F.,(4,3,4),(3.5762240613455E-18,0.00087155518478463,
0.00160565474756239),.UNSPECIFIED.);
#823=B_SPLINE_CURVE_WITH_KNOTS('',3,(#19401,#19402,#19403,#19404,#19405,
#19406,#19407,#19408,#19409,#19410),.UNSPECIFIED.,.F.,.F.,(4,2,2,2,4),(-0.260724731519967,
-0.199727802453978,-0.130390835657575,-0.0610645770444141,0.),
 .UNSPECIFIED.);
#824=B_SPLINE_CURVE_WITH_KNOTS('',3,(#19412,#19413,#19414,#19415,#19416,
#19417,#19418),.UNSPECIFIED.,.F.,.F.,(4,3,4),(0.,0.000879527967511419,0.00156997524831123),
 .UNSPECIFIED.);
#825=B_SPLINE_CURVE_WITH_KNOTS('',3,(#19422,#19423,#19424,#19425,#19426,
#19427,#19428),.UNSPECIFIED.,.F.,.F.,(4,3,4),(7.81246474747696E-18,0.000871555184784776,
0.00160565474756103),.UNSPECIFIED.);
#826=B_SPLINE_CURVE_WITH_KNOTS('',3,(#19430,#19431,#19432,#19433,#19434,
#19435,#19436,#19437,#19438,#19439),.UNSPECIFIED.,.F.,.F.,(4,2,2,2,4),(-0.260724731519981,
-0.199727802453996,-0.130390835657592,-0.0610645770444198,0.),
 .UNSPECIFIED.);
#827=B_SPLINE_CURVE_WITH_KNOTS('',3,(#19441,#19442,#19443,#19444,#19445,
#19446,#19447),.UNSPECIFIED.,.F.,.F.,(4,3,4),(1.9930455364338E-17,0.00087952796764905,
0.00156997524830989),.UNSPECIFIED.);
#828=B_SPLINE_CURVE_WITH_KNOTS('',3,(#19451,#19452,#19453,#19454,#19455,
#19456,#19457),.UNSPECIFIED.,.F.,.F.,(4,3,4),(1.97026712507607E-17,0.000871555184781697,
0.00160565474757729),.UNSPECIFIED.);
#829=B_SPLINE_CURVE_WITH_KNOTS('',3,(#19459,#19460,#19461,#19462,#19463,
#19464,#19465,#19466,#19467,#19468),.UNSPECIFIED.,.F.,.F.,(4,2,2,2,4),(-0.260724731519855,
-0.199727802453898,-0.130390835657533,-0.0610645770444068,0.),
 .UNSPECIFIED.);
#830=B_SPLINE_CURVE_WITH_KNOTS('',3,(#19470,#19471,#19472,#19473,#19474,
#19475,#19476),.UNSPECIFIED.,.F.,.F.,(4,3,4),(0.,0.000879527967652466,0.00156997524832605),
 .UNSPECIFIED.);
#831=B_SPLINE_CURVE_WITH_KNOTS('',3,(#19480,#19481,#19482,#19483,#19484,
#19485,#19486),.UNSPECIFIED.,.F.,.F.,(4,3,4),(3.46944695195361E-18,0.000871555184779645,
0.00160565474757727),.UNSPECIFIED.);
#832=B_SPLINE_CURVE_WITH_KNOTS('',3,(#19488,#19489,#19490,#19491,#19492,
#19493,#19494,#19495,#19496,#19497),.UNSPECIFIED.,.F.,.F.,(4,2,2,2,4),(-0.260724731519956,
-0.199727802453977,-0.130390835657575,-0.0610645770444154,0.),
 .UNSPECIFIED.);
#833=B_SPLINE_CURVE_WITH_KNOTS('',3,(#19499,#19500,#19501,#19502,#19503,
#19504,#19505),.UNSPECIFIED.,.F.,.F.,(4,3,4),(0.,0.000879527967652087,0.00156997524832604),
 .UNSPECIFIED.);
#834=B_SPLINE_CURVE_WITH_KNOTS('',3,(#19509,#19510,#19511,#19512,#19513,
#19514,#19515),.UNSPECIFIED.,.F.,.F.,(4,3,4),(3.46944695195361E-18,0.000871555184781849,
0.00160565474757726),.UNSPECIFIED.);
#835=B_SPLINE_CURVE_WITH_KNOTS('',3,(#19517,#19518,#19519,#19520,#19521,
#19522,#19523,#19524,#19525,#19526),.UNSPECIFIED.,.F.,.F.,(4,2,2,2,4),(-0.260724731519955,
-0.199727802453976,-0.130390835657579,-0.0610645770444187,0.),
 .UNSPECIFIED.);
#836=B_SPLINE_CURVE_WITH_KNOTS('',3,(#19528,#19529,#19530,#19531,#19532,
#19533,#19534),.UNSPECIFIED.,.F.,.F.,(4,3,4),(0.,0.000879527967511223,0.00156997524832604),
 .UNSPECIFIED.);
#837=B_SPLINE_CURVE_WITH_KNOTS('',3,(#19538,#19539,#19540,#19541,#19542,
#19543,#19544),.UNSPECIFIED.,.F.,.F.,(4,3,4),(2.32821605822755E-16,0.000871555185125512,
0.00160565474757726),.UNSPECIFIED.);
#838=B_SPLINE_CURVE_WITH_KNOTS('',3,(#19546,#19547,#19548,#19549,#19550,
#19551,#19552,#19553,#19554,#19555),.UNSPECIFIED.,.F.,.F.,(4,2,2,2,4),(-0.260724731516488,
-0.199727802451468,-0.130390835656146,-0.0610645770440642,0.),
 .UNSPECIFIED.);
#839=B_SPLINE_CURVE_WITH_KNOTS('',3,(#19557,#19558,#19559,#19560,#19561,
#19562,#19563),.UNSPECIFIED.,.F.,.F.,(4,3,4),(0.,0.000879527967497746,0.00156997524832604),
 .UNSPECIFIED.);
#840=B_SPLINE_CURVE_WITH_KNOTS('',3,(#19567,#19568,#19569,#19570,#19571,
#19572,#19573),.UNSPECIFIED.,.F.,.F.,(4,3,4),(3.46944695195361E-18,0.000871555184784586,
0.00160565474757726),.UNSPECIFIED.);
#841=B_SPLINE_CURVE_WITH_KNOTS('',3,(#19575,#19576,#19577,#19578,#19579,
#19580,#19581,#19582,#19583,#19584),.UNSPECIFIED.,.F.,.F.,(4,2,2,2,4),(-0.2607247315199,
-0.199727802453934,-0.130390835657557,-0.0610645770444129,0.),
 .UNSPECIFIED.);
#842=B_SPLINE_CURVE_WITH_KNOTS('',3,(#19586,#19587,#19588,#19589,#19590,
#19591,#19592),.UNSPECIFIED.,.F.,.F.,(4,3,4),(0.,0.000879527967505927,0.00156997524832604),
 .UNSPECIFIED.);
#843=B_SPLINE_CURVE_WITH_KNOTS('',3,(#19596,#19597,#19598,#19599,#19600,
#19601,#19602),.UNSPECIFIED.,.F.,.F.,(4,3,4),(0.,0.000871555184783887,0.00160565474757725),
 .UNSPECIFIED.);
#844=B_SPLINE_CURVE_WITH_KNOTS('',3,(#19604,#19605,#19606,#19607,#19608,
#19609,#19610,#19611,#19612,#19613),.UNSPECIFIED.,.F.,.F.,(4,2,2,2,4),(-0.26072473151999,
-0.199727802454001,-0.13039083565759,-0.0610645770444177,0.),
 .UNSPECIFIED.);
#845=B_SPLINE_CURVE_WITH_KNOTS('',3,(#19615,#19616,#19617,#19618,#19619,
#19620,#19621),.UNSPECIFIED.,.F.,.F.,(4,3,4),(0.,0.000879527967504626,0.00156997524832606),
 .UNSPECIFIED.);
#846=B_SPLINE_CURVE_WITH_KNOTS('',3,(#19625,#19626,#19627,#19628,#19629,
#19630,#19631),.UNSPECIFIED.,.F.,.F.,(4,3,4),(4.9065389333868E-18,0.000871555184783266,
0.00160565474757725),.UNSPECIFIED.);
#847=B_SPLINE_CURVE_WITH_KNOTS('',3,(#19633,#19634,#19635,#19636,#19637,
#19638,#19639,#19640,#19641,#19642),.UNSPECIFIED.,.F.,.F.,(4,2,2,2,4),(-0.260724731522011,
-0.199727808951148,-0.130390835646158,-0.0610645826755033,0.),
 .UNSPECIFIED.);
#848=B_SPLINE_CURVE_WITH_KNOTS('',3,(#19644,#19645,#19646,#19647,#19648,
#19649,#19650),.UNSPECIFIED.,.F.,.F.,(4,3,4),(0.,0.000879527967507628,0.00156997524832605),
 .UNSPECIFIED.);
#849=B_SPLINE_CURVE_WITH_KNOTS('',3,(#19654,#19655,#19656,#19657,#19658,
#19659,#19660),.UNSPECIFIED.,.F.,.F.,(4,3,4),(2.09578719802802E-16,0.000871555185122462,
0.00160565474757726),.UNSPECIFIED.);
#850=B_SPLINE_CURVE_WITH_KNOTS('',3,(#19662,#19663,#19664,#19665,#19666,
#19667,#19668,#19669,#19670,#19671),.UNSPECIFIED.,.F.,.F.,(4,2,2,2,4),(-0.260724731516458,
-0.199727802451451,-0.130390835656143,-0.0610645770440656,0.),
 .UNSPECIFIED.);
#851=B_SPLINE_CURVE_WITH_KNOTS('',3,(#19673,#19674,#19675,#19676,#19677,
#19678,#19679),.UNSPECIFIED.,.F.,.F.,(4,3,4),(0.,0.000879527967500393,0.00156997524832608),
 .UNSPECIFIED.);
#852=B_SPLINE_CURVE_WITH_KNOTS('',3,(#19683,#19684,#19685,#19686,#19687,
#19688,#19689),.UNSPECIFIED.,.F.,.F.,(4,3,4),(9.34177181294034E-18,0.000871555184782784,
0.00160565474757725),.UNSPECIFIED.);
#853=B_SPLINE_CURVE_WITH_KNOTS('',3,(#19691,#19692,#19693,#19694,#19695,
#19696,#19697,#19698,#19699,#19700),.UNSPECIFIED.,.F.,.F.,(4,2,2,2,4),(-0.260724731519931,
-0.199727802453962,-0.130390835657569,-0.0610645770444118,0.),
 .UNSPECIFIED.);
#854=B_SPLINE_CURVE_WITH_KNOTS('',3,(#19702,#19703,#19704,#19705,#19706,
#19707,#19708),.UNSPECIFIED.,.F.,.F.,(4,3,4),(0.,0.000879527967502687,0.00156997524832604),
 .UNSPECIFIED.);
#855=B_SPLINE_CURVE_WITH_KNOTS('',3,(#19712,#19713,#19714,#19715,#19716,
#19717,#19718),.UNSPECIFIED.,.F.,.F.,(4,3,4),(3.87895961444886E-18,0.000871555184780596,
0.00160565474757726),.UNSPECIFIED.);
#856=B_SPLINE_CURVE_WITH_KNOTS('',3,(#19720,#19721,#19722,#19723,#19724,
#19725,#19726,#19727,#19728,#19729),.UNSPECIFIED.,.F.,.F.,(4,2,2,2,4),(-0.260724731519954,
-0.199727802453973,-0.130390835657584,-0.0610645770444205,0.),
 .UNSPECIFIED.);
#857=B_SPLINE_CURVE_WITH_KNOTS('',3,(#19731,#19732,#19733,#19734,#19735,
#19736,#19737),.UNSPECIFIED.,.F.,.F.,(4,3,4),(0.,0.000879527967508752,0.00156997524832606),
 .UNSPECIFIED.);
#858=B_SPLINE_CURVE_WITH_KNOTS('',3,(#19741,#19742,#19743,#19744,#19745,
#19746,#19747),.UNSPECIFIED.,.F.,.F.,(4,3,4),(7.81246474747696E-18,0.000871555184790998,
0.00160565474757727),.UNSPECIFIED.);
#859=B_SPLINE_CURVE_WITH_KNOTS('',3,(#19749,#19750,#19751,#19752,#19753,
#19754),.UNSPECIFIED.,.F.,.F.,(4,2,4),(0.,0.0407463936727646,0.0482791015350969),
 .UNSPECIFIED.);
#860=B_SPLINE_CURVE_WITH_KNOTS('',3,(#19759,#19760,#19761,#19762,#19763,
#19764,#19765,#19766,#19767,#19768),.UNSPECIFIED.,.F.,.F.,(4,2,2,2,4),(0.0482791015350969,
0.0839662032253167,0.15419854744165,0.209083280006158,0.260520203475897),
 .UNSPECIFIED.);
#861=B_SPLINE_CURVE_WITH_KNOTS('',3,(#19770,#19771,#19772,#19773,#19774,
#19775,#19776),.UNSPECIFIED.,.F.,.F.,(4,3,4),(0.,0.000879527967511759,0.00156997524832607),
 .UNSPECIFIED.);
#862=B_SPLINE_CURVE_WITH_KNOTS('',3,(#19780,#19781,#19782,#19783,#19784,
#19785,#19786),.UNSPECIFIED.,.F.,.F.,(4,3,4),(3.46944695195361E-18,0.000871555184791261,
0.00160565474757729),.UNSPECIFIED.);
#863=B_SPLINE_CURVE_WITH_KNOTS('',3,(#19788,#19789,#19790,#19791,#19792,
#19793,#19794,#19795,#19796,#19797),.UNSPECIFIED.,.F.,.F.,(4,2,2,2,4),(-0.260724731519979,
-0.199727802453994,-0.130390835657588,-0.061064577044418,0.),
 .UNSPECIFIED.);
#864=B_SPLINE_CURVE_WITH_KNOTS('',3,(#19799,#19800,#19801,#19802,#19803,
#19804,#19805),.UNSPECIFIED.,.F.,.F.,(4,3,4),(0.,0.000879527967511587,0.00156997524832605),
 .UNSPECIFIED.);
#865=B_SPLINE_CURVE_WITH_KNOTS('',3,(#19809,#19810,#19811,#19812,#19813,
#19814,#19815),.UNSPECIFIED.,.F.,.F.,(4,3,4),(2.14776701328641E-16,0.000871555185130942,
0.00160565474757727),.UNSPECIFIED.);
#866=B_SPLINE_CURVE_WITH_KNOTS('',3,(#19817,#19818,#19819,#19820,#19821,
#19822,#19823,#19824,#19825,#19826),.UNSPECIFIED.,.F.,.F.,(4,2,2,2,4),(-0.260724731516507,
-0.19972780245148,-0.130390835656155,-0.0610645770440656,0.),
 .UNSPECIFIED.);
#867=B_SPLINE_CURVE_WITH_KNOTS('',3,(#19828,#19829,#19830,#19831,#19832,
#19833,#19834),.UNSPECIFIED.,.F.,.F.,(4,3,4),(0.,0.000879527967649747,0.00156997524832607),
 .UNSPECIFIED.);
#868=B_SPLINE_CURVE_WITH_KNOTS('',3,(#19838,#19839,#19840,#19841,#19842,
#19843,#19844),.UNSPECIFIED.,.F.,.F.,(4,3,4),(1.98214456752023E-16,0.000871555185118887,
0.00160565474757726),.UNSPECIFIED.);
#869=B_SPLINE_CURVE_WITH_KNOTS('',3,(#19846,#19847,#19848,#19849,#19850,
#19851,#19852,#19853,#19854,#19855),.UNSPECIFIED.,.F.,.F.,(4,2,2,2,4),(-0.260724731516436,
-0.199727802451429,-0.130390835656129,-0.0610645770440628,0.),
 .UNSPECIFIED.);
#870=B_SPLINE_CURVE_WITH_KNOTS('',3,(#19857,#19858,#19859,#19860,#19861,
#19862,#19863),.UNSPECIFIED.,.F.,.F.,(4,3,4),(0.,0.000879527967649307,0.00156997524832607),
 .UNSPECIFIED.);
#871=B_SPLINE_CURVE_WITH_KNOTS('',3,(#19867,#19868,#19869,#19870,#19871,
#19872,#19873),.UNSPECIFIED.,.F.,.F.,(4,3,4),(2.04579727988785E-16,0.00087155518513034,
0.00160565474757726),.UNSPECIFIED.);
#872=B_SPLINE_CURVE_WITH_KNOTS('',3,(#19875,#19876,#19877,#19878,#19879,
#19880,#19881,#19882,#19883,#19884),.UNSPECIFIED.,.F.,.F.,(4,2,2,2,4),(-0.260724731516512,
-0.199727802451486,-0.130390835656163,-0.0610645770440718,0.),
 .UNSPECIFIED.);
#873=B_SPLINE_CURVE_WITH_KNOTS('',3,(#19886,#19887,#19888,#19889,#19890,
#19891,#19892),.UNSPECIFIED.,.F.,.F.,(4,3,4),(0.,0.000879527967646912,0.00156997524832608),
 .UNSPECIFIED.);
#874=B_SPLINE_CURVE_WITH_KNOTS('',3,(#19896,#19897,#19898,#19899,#19900,
#19901,#19902),.UNSPECIFIED.,.F.,.F.,(4,3,4),(1.95654969040488E-16,0.000871555185114593,
0.00160565474757726),.UNSPECIFIED.);
#875=B_SPLINE_CURVE_WITH_KNOTS('',3,(#19904,#19905,#19906,#19907,#19908,
#19909,#19910,#19911,#19912,#19913),.UNSPECIFIED.,.F.,.F.,(4,2,2,2,4),(-0.260724731516399,
-0.199727802451402,-0.130390835656104,-0.0610645770440508,0.),
 .UNSPECIFIED.);
#876=B_SPLINE_CURVE_WITH_KNOTS('',3,(#19915,#19916,#19917,#19918,#19919,
#19920,#19921),.UNSPECIFIED.,.F.,.F.,(4,3,4),(0.,0.000879527967647974,0.00156997524832605),
 .UNSPECIFIED.);
#877=B_SPLINE_CURVE_WITH_KNOTS('',3,(#19925,#19926,#19927,#19928,#19929,
#19930,#19931),.UNSPECIFIED.,.F.,.F.,(4,3,4),(1.30968750346023E-17,0.000871555184789597,
0.00160565474757726),.UNSPECIFIED.);
#878=B_SPLINE_CURVE_WITH_KNOTS('',3,(#19933,#19934,#19935,#19936,#19937,
#19938,#19939,#19940,#19941,#19942),.UNSPECIFIED.,.F.,.F.,(4,2,2,2,4),(-0.260724731519943,
-0.199727802453962,-0.130390835657567,-0.0610645770444133,0.),
 .UNSPECIFIED.);
#879=B_SPLINE_CURVE_WITH_KNOTS('',3,(#19944,#19945,#19946,#19947,#19948,
#19949,#19950),.UNSPECIFIED.,.F.,.F.,(4,3,4),(0.,0.000879527967504028,0.00156997524832602),
 .UNSPECIFIED.);
#880=B_SPLINE_CURVE_WITH_KNOTS('',3,(#19954,#19955,#19956,#19957,#19958,
#19959,#19960),.UNSPECIFIED.,.F.,.F.,(4,3,4),(1.73472347597681E-18,0.000871555184776652,
0.00160565474757725),.UNSPECIFIED.);
#881=B_SPLINE_CURVE_WITH_KNOTS('',3,(#19962,#19963,#19964,#19965,#19966,
#19967,#19968,#19969,#19970,#19971),.UNSPECIFIED.,.F.,.F.,(4,2,2,2,4),(-0.260724731519973,
-0.199727802453988,-0.130390835657582,-0.0610645770444168,0.),
 .UNSPECIFIED.);
#882=B_SPLINE_CURVE_WITH_KNOTS('',3,(#19973,#19974,#19975,#19976,#19977,
#19978,#19979),.UNSPECIFIED.,.F.,.F.,(4,3,4),(0.,0.0008795279676465,0.00156997524832604),
 .UNSPECIFIED.);
#883=B_SPLINE_CURVE_WITH_KNOTS('',3,(#19983,#19984,#19985,#19986,#19987,
#19988,#19989),.UNSPECIFIED.,.F.,.F.,(4,3,4),(2.57885184514585E-17,0.000871555184785543,
0.00160565474757727),.UNSPECIFIED.);
#884=B_SPLINE_CURVE_WITH_KNOTS('',3,(#19991,#19992,#19993,#19994,#19995,
#19996,#19997,#19998,#19999,#20000),.UNSPECIFIED.,.F.,.F.,(4,2,2,2,4),(-0.260724731519904,
-0.199727802453939,-0.130390835657553,-0.0610645770444076,0.),
 .UNSPECIFIED.);
#885=B_SPLINE_CURVE_WITH_KNOTS('',3,(#20002,#20003,#20004,#20005,#20006,
#20007,#20008),.UNSPECIFIED.,.F.,.F.,(4,3,4),(0.,0.000879527967654812,0.00156997524832605),
 .UNSPECIFIED.);
#886=B_SPLINE_CURVE_WITH_KNOTS('',3,(#20012,#20013,#20014,#20015,#20016,
#20017,#20018),.UNSPECIFIED.,.F.,.F.,(4,3,4),(1.73472347597681E-18,0.000871555184781887,
0.00160565474757726),.UNSPECIFIED.);
#887=B_SPLINE_CURVE_WITH_KNOTS('',3,(#20020,#20021,#20022,#20023,#20024,
#20025,#20026,#20027,#20028,#20029),.UNSPECIFIED.,.F.,.F.,(4,2,2,2,4),(-0.260724731519953,
-0.19972780245398,-0.130390835657581,-0.0610645770444158,0.),
 .UNSPECIFIED.);
#888=B_SPLINE_CURVE_WITH_KNOTS('',3,(#20031,#20032,#20033,#20034,#20035,
#20036,#20037),.UNSPECIFIED.,.F.,.F.,(4,3,4),(0.,0.000879527967510002,0.00156997524832605),
 .UNSPECIFIED.);
#889=B_SPLINE_CURVE_WITH_KNOTS('',3,(#20041,#20042,#20043,#20044,#20045,
#20046,#20047),.UNSPECIFIED.,.F.,.F.,(4,3,4),(1.01522088571945E-17,0.00087155518478881,
0.00160565474757727),.UNSPECIFIED.);
#890=B_SPLINE_CURVE_WITH_KNOTS('',3,(#20049,#20050,#20051,#20052,#20053,
#20054,#20055,#20056,#20057,#20058),.UNSPECIFIED.,.F.,.F.,(4,2,2,2,4),(-0.260724731519909,
-0.199727802453946,-0.130390835657565,-0.0610645770444126,0.),
 .UNSPECIFIED.);
#891=B_SPLINE_CURVE_WITH_KNOTS('',3,(#20060,#20061,#20062,#20063,#20064,
#20065,#20066),.UNSPECIFIED.,.F.,.F.,(4,3,4),(0.,0.000879527967647106,0.00156997524832605),
 .UNSPECIFIED.);
#892=B_SPLINE_CURVE_WITH_KNOTS('',3,(#20070,#20071,#20072,#20073,#20074,
#20075,#20076),.UNSPECIFIED.,.F.,.F.,(4,3,4),(9.9846720473553E-18,0.000871555184783746,
0.00160565474757726),.UNSPECIFIED.);
#893=B_SPLINE_CURVE_WITH_KNOTS('',3,(#20078,#20079,#20080,#20081,#20082,
#20083,#20084,#20085,#20086,#20087),.UNSPECIFIED.,.F.,.F.,(4,2,2,2,4),(-0.26072473151994,
-0.199727802453954,-0.130390835657562,-0.0610645770444132,0.),
 .UNSPECIFIED.);
#894=B_SPLINE_CURVE_WITH_KNOTS('',3,(#20089,#20090,#20091,#20092,#20093,
#20094,#20095),.UNSPECIFIED.,.F.,.F.,(4,3,4),(0.,0.000879527967650889,0.00156997524832608),
 .UNSPECIFIED.);
#895=B_SPLINE_CURVE_WITH_KNOTS('',3,(#20099,#20100,#20101,#20102,#20103,
#20104,#20105),.UNSPECIFIED.,.F.,.F.,(4,3,4),(3.46944695195361E-18,0.000871555184784394,
0.00160565474757728),.UNSPECIFIED.);
#896=B_SPLINE_CURVE_WITH_KNOTS('',3,(#20107,#20108,#20109,#20110,#20111,
#20112,#20113,#20114,#20115,#20116),.UNSPECIFIED.,.F.,.F.,(4,2,2,2,4),(-0.260724731519926,
-0.19972780245395,-0.130390835657561,-0.061064577044412,0.),
 .UNSPECIFIED.);
#897=B_SPLINE_CURVE_WITH_KNOTS('',3,(#20118,#20119,#20120,#20121,#20122,
#20123,#20124),.UNSPECIFIED.,.F.,.F.,(4,3,4),(0.,0.000879527967499868,0.00156997524832605),
 .UNSPECIFIED.);
#898=B_SPLINE_CURVE_WITH_KNOTS('',3,(#20128,#20129,#20130,#20131,#20132,
#20133,#20134),.UNSPECIFIED.,.F.,.F.,(4,3,4),(1.73472347597681E-18,0.000871555184787591,
0.00160565474757725),.UNSPECIFIED.);
#899=B_SPLINE_CURVE_WITH_KNOTS('',3,(#20136,#20137,#20138,#20139,#20140,
#20141,#20142,#20143,#20144,#20145),.UNSPECIFIED.,.F.,.F.,(4,2,2,2,4),(-0.260724731519915,
-0.199727802453947,-0.130390835657561,-0.0610645770444091,0.),
 .UNSPECIFIED.);
#900=B_SPLINE_CURVE_WITH_KNOTS('',3,(#20147,#20148,#20149,#20150,#20151,
#20152,#20153),.UNSPECIFIED.,.F.,.F.,(4,3,4),(0.,0.000879527967506563,0.00156997524832605),
 .UNSPECIFIED.);
#901=B_SPLINE_CURVE_WITH_KNOTS('',3,(#20157,#20158,#20159,#20160,#20161,
#20162,#20163),.UNSPECIFIED.,.F.,.F.,(4,3,4),(2.09154710985512E-16,0.000871555185128014,
0.00160565474757726),.UNSPECIFIED.);
#902=B_SPLINE_CURVE_WITH_KNOTS('',3,(#20165,#20166,#20167,#20168,#20169,
#20170,#20171,#20172,#20173,#20174),.UNSPECIFIED.,.F.,.F.,(4,2,2,2,4),(-0.260724731516491,
-0.199727802451466,-0.130390835656145,-0.0610645770440631,0.),
 .UNSPECIFIED.);
#903=B_SPLINE_CURVE_WITH_KNOTS('',3,(#20176,#20177,#20178,#20179,#20180,
#20181,#20182),.UNSPECIFIED.,.F.,.F.,(4,3,4),(0.,0.000879527967651056,0.00156997524832606),
 .UNSPECIFIED.);
#904=B_SPLINE_CURVE_WITH_KNOTS('',3,(#20186,#20187,#20188,#20189,#20190,
#20191,#20192),.UNSPECIFIED.,.F.,.F.,(4,3,4),(0.,0.000871555184787238,0.00160565474757725),
 .UNSPECIFIED.);
#905=B_SPLINE_CURVE_WITH_KNOTS('',3,(#20194,#20195,#20196,#20197,#20198,
#20199,#20200,#20201,#20202,#20203),.UNSPECIFIED.,.F.,.F.,(4,2,2,2,4),(-0.260724731519923,
-0.199727802453942,-0.130390835657558,-0.0610645770444118,0.),
 .UNSPECIFIED.);
#906=B_SPLINE_CURVE_WITH_KNOTS('',3,(#20205,#20206,#20207,#20208,#20209,
#20210,#20211),.UNSPECIFIED.,.F.,.F.,(4,3,4),(0.,0.00087952796764459,0.00156997524832608),
 .UNSPECIFIED.);
#907=B_SPLINE_CURVE_WITH_KNOTS('',3,(#20215,#20216,#20217,#20218,#20219,
#20220,#20221),.UNSPECIFIED.,.F.,.F.,(4,3,4),(8.49837472194074E-18,0.000871555184788193,
0.00160565474757728),.UNSPECIFIED.);
#908=B_SPLINE_CURVE_WITH_KNOTS('',3,(#20223,#20224,#20225,#20226,#20227,
#20228,#20229,#20230,#20231,#20232),.UNSPECIFIED.,.F.,.F.,(4,2,2,2,4),(-0.260724731519922,
-0.199727802453952,-0.130390835657565,-0.0610645770444117,0.),
 .UNSPECIFIED.);
#909=B_SPLINE_CURVE_WITH_KNOTS('',3,(#20234,#20235,#20236,#20237,#20238,
#20239,#20240),.UNSPECIFIED.,.F.,.F.,(4,3,4),(0.,0.000879527967508577,0.00156997524832604),
 .UNSPECIFIED.);
#910=B_SPLINE_CURVE_WITH_KNOTS('',3,(#20244,#20245,#20246,#20247,#20248,
#20249,#20250),.UNSPECIFIED.,.F.,.F.,(4,3,4),(2.05935861929181E-16,0.000871555185115414,
0.00160565474757727),.UNSPECIFIED.);
#911=B_SPLINE_CURVE_WITH_KNOTS('',3,(#20252,#20253,#20254,#20255,#20256,
#20257,#20258,#20259,#20260,#20261),.UNSPECIFIED.,.F.,.F.,(4,2,2,2,4),(-0.260724731516467,
-0.199727802451455,-0.130390835656149,-0.0610645770440673,0.),
 .UNSPECIFIED.);
#912=B_SPLINE_CURVE_WITH_KNOTS('',3,(#20263,#20264,#20265,#20266,#20267,
#20268,#20269),.UNSPECIFIED.,.F.,.F.,(4,3,4),(0.,0.000879527967500517,0.00156997524832606),
 .UNSPECIFIED.);
#913=B_SPLINE_CURVE_WITH_KNOTS('',3,(#20273,#20274,#20275,#20276,#20277,
#20278,#20279),.UNSPECIFIED.,.F.,.F.,(4,3,4),(4.9065389333868E-18,0.000871555184783715,
0.00160565474757726),.UNSPECIFIED.);
#914=B_SPLINE_CURVE_WITH_KNOTS('',3,(#20281,#20282,#20283,#20284,#20285,
#20286,#20287,#20288,#20289,#20290),.UNSPECIFIED.,.F.,.F.,(4,2,2,2,4),(-0.260724731521994,
-0.199727808951145,-0.130390835646155,-0.0610645826755003,0.),
 .UNSPECIFIED.);
#915=B_SPLINE_CURVE_WITH_KNOTS('',3,(#20292,#20293,#20294,#20295,#20296,
#20297,#20298),.UNSPECIFIED.,.F.,.F.,(4,3,4),(0.,0.000879527967502014,0.00156997524832605),
 .UNSPECIFIED.);
#916=B_SPLINE_CURVE_WITH_KNOTS('',3,(#20302,#20303,#20304,#20305,#20306,
#20307,#20308),.UNSPECIFIED.,.F.,.F.,(4,3,4),(0.,0.000871555184778678,0.00160565474757727),
 .UNSPECIFIED.);
#917=B_SPLINE_CURVE_WITH_KNOTS('',3,(#20310,#20311,#20312,#20313,#20314,
#20315,#20316,#20317,#20318,#20319),.UNSPECIFIED.,.F.,.F.,(4,2,2,2,4),(-0.260724731519916,
-0.199727802453945,-0.130390835657561,-0.0610645770444109,0.),
 .UNSPECIFIED.);
#918=B_SPLINE_CURVE_WITH_KNOTS('',3,(#20321,#20322,#20323,#20324,#20325,
#20326,#20327),.UNSPECIFIED.,.F.,.F.,(4,3,4),(0.,0.000879527967649045,0.00156997524832605),
 .UNSPECIFIED.);
#919=B_SPLINE_CURVE_WITH_KNOTS('',3,(#20331,#20332,#20333,#20334,#20335,
#20336,#20337),.UNSPECIFIED.,.F.,.F.,(4,3,4),(7.94950163848063E-18,0.000871555184775057,
0.00160565474757727),.UNSPECIFIED.);
#920=B_SPLINE_CURVE_WITH_KNOTS('',3,(#20339,#20340,#20341,#20342,#20343,
#20344,#20345,#20346,#20347,#20348),.UNSPECIFIED.,.F.,.F.,(4,2,2,2,4),(-0.260724731519915,
-0.199727802453944,-0.13039083565756,-0.0610645770444119,0.),
 .UNSPECIFIED.);
#921=B_SPLINE_CURVE_WITH_KNOTS('',3,(#20350,#20351,#20352,#20353,#20354,
#20355,#20356),.UNSPECIFIED.,.F.,.F.,(4,3,4),(0.,0.000879527967640991,0.00156997524832605),
 .UNSPECIFIED.);
#922=B_SPLINE_CURVE_WITH_KNOTS('',3,(#20360,#20361,#20362,#20363,#20364,
#20365,#20366),.UNSPECIFIED.,.F.,.F.,(4,3,4),(0.,0.000871555184782733,0.00160565474757727),
 .UNSPECIFIED.);
#923=B_SPLINE_CURVE_WITH_KNOTS('',3,(#20368,#20369,#20370,#20371,#20372,
#20373,#20374,#20375,#20376,#20377),.UNSPECIFIED.,.F.,.F.,(4,2,2,2,4),(-0.260724731519912,
-0.199727802453946,-0.130390835657566,-0.0610645770444142,0.),
 .UNSPECIFIED.);
#924=B_SPLINE_CURVE_WITH_KNOTS('',3,(#20379,#20380,#20381,#20382,#20383,
#20384,#20385),.UNSPECIFIED.,.F.,.F.,(4,3,4),(0.,0.00087952796764763,0.00156997524832606),
 .UNSPECIFIED.);
#925=B_SPLINE_CURVE_WITH_KNOTS('',3,(#20388,#20389,#20390,#20391,#20392,
#20393,#20394),.UNSPECIFIED.,.F.,.F.,(4,3,4),(7.81246474747696E-18,0.000871555184773631,
0.00160565474757588),.UNSPECIFIED.);
#926=B_SPLINE_CURVE_WITH_KNOTS('',3,(#20407,#20408,#20409,#20410,#20411,
#20412,#20413,#20414,#20415,#20416,#20417,#20418),.UNSPECIFIED.,.F.,.F.,
(4,2,2,2,2,4),(0.,0.0407569430586041,0.0839882141528699,0.154219975171057,
0.209093406724745,0.260520353691867),.UNSPECIFIED.);
#927=B_SPLINE_CURVE_WITH_KNOTS('',3,(#20420,#20421,#20422,#20423,#20424,
#20425,#20426),.UNSPECIFIED.,.F.,.F.,(4,3,4),(1.78811203067275E-18,0.000871811004260026,
0.00160579165132935),.UNSPECIFIED.);
#928=B_SPLINE_CURVE_WITH_KNOTS('',3,(#20430,#20431,#20432,#20433,#20434,
#20435,#20436),.UNSPECIFIED.,.F.,.F.,(4,3,4),(3.69724068824877E-17,0.000879500804028015,
0.00156989029765835),.UNSPECIFIED.);
#929=B_SPLINE_CURVE_WITH_KNOTS('',3,(#20438,#20439,#20440,#20441,#20442,
#20443,#20444,#20445,#20446,#20447),.UNSPECIFIED.,.F.,.F.,(4,2,2,2,4),(-0.260724943430805,
-0.199726494015773,-0.130391022448095,-0.0610665706517605,0.),
 .UNSPECIFIED.);
#930=B_SPLINE_CURVE_WITH_KNOTS('',3,(#20449,#20450,#20451,#20452,#20453,
#20454,#20455),.UNSPECIFIED.,.F.,.F.,(4,3,4),(7.94950163848063E-18,0.000871811004271929,
0.00160579165132327),.UNSPECIFIED.);
#931=B_SPLINE_CURVE_WITH_KNOTS('',3,(#20459,#20460,#20461,#20462,#20463,
#20464,#20465),.UNSPECIFIED.,.F.,.F.,(4,3,4),(2.7097246932071E-17,0.000879500804038936,
0.00156989029765586),.UNSPECIFIED.);
#932=B_SPLINE_CURVE_WITH_KNOTS('',3,(#20467,#20468,#20469,#20470,#20471,
#20472,#20473,#20474,#20475,#20476),.UNSPECIFIED.,.F.,.F.,(4,2,2,2,4),(-0.260724943430658,
-0.199726493772702,-0.130391022195998,-0.0610665704089927,0.),
 .UNSPECIFIED.);
#933=B_SPLINE_CURVE_WITH_KNOTS('',3,(#20478,#20479,#20480,#20481,#20482,
#20483,#20484),.UNSPECIFIED.,.F.,.F.,(4,3,4),(2.91013228173329E-14,0.000871811007982037,
0.00160579165130272),.UNSPECIFIED.);
#934=B_SPLINE_CURVE_WITH_KNOTS('',3,(#20488,#20489,#20490,#20491,#20492,
#20493,#20494),.UNSPECIFIED.,.F.,.F.,(4,3,4),(2.11749985874298E-17,0.000879500804027354,
0.00156989029765845),.UNSPECIFIED.);
#935=B_SPLINE_CURVE_WITH_KNOTS('',3,(#20496,#20497,#20498,#20499,#20500,
#20501,#20502,#20503,#20504,#20505),.UNSPECIFIED.,.F.,.F.,(4,2,2,2,4),(-0.260724943430588,
-0.199726493772793,-0.130391022195965,-0.0610665704088414,0.),
 .UNSPECIFIED.);
#936=B_SPLINE_CURVE_WITH_KNOTS('',3,(#20507,#20508,#20509,#20510,#20511,
#20512,#20513),.UNSPECIFIED.,.F.,.F.,(4,3,4),(2.91023102291187E-14,0.000871811007963625,
0.00160579165130527),.UNSPECIFIED.);
#937=B_SPLINE_CURVE_WITH_KNOTS('',3,(#20517,#20518,#20519,#20520,#20521,
#20522,#20523),.UNSPECIFIED.,.F.,.F.,(4,3,4),(2.32737576866932E-17,0.000879500804022207,
0.00156989029766219),.UNSPECIFIED.);
#938=B_SPLINE_CURVE_WITH_KNOTS('',3,(#20525,#20526,#20527,#20528,#20529,
#20530,#20531,#20532,#20533,#20534),.UNSPECIFIED.,.F.,.F.,(4,2,2,2,4),(-0.260724943430767,
-0.199726493772903,-0.130391022196058,-0.0610665704089389,0.),
 .UNSPECIFIED.);
#939=B_SPLINE_CURVE_WITH_KNOTS('',3,(#20536,#20537,#20538,#20539,#20540,
#20541,#20542),.UNSPECIFIED.,.F.,.F.,(4,3,4),(2.90971702336027E-14,0.000871811007985608,
0.00160579165129744),.UNSPECIFIED.);
#940=B_SPLINE_CURVE_WITH_KNOTS('',3,(#20546,#20547,#20548,#20549,#20550,
#20551,#20552),.UNSPECIFIED.,.F.,.F.,(4,3,4),(3.49106365300398E-17,0.000879500804038357,
0.00156989029766081),.UNSPECIFIED.);
#941=B_SPLINE_CURVE_WITH_KNOTS('',3,(#20554,#20555,#20556,#20557,#20558,
#20559,#20560,#20561,#20562,#20563),.UNSPECIFIED.,.F.,.F.,(4,2,2,2,4),(-0.260724943430475,
-0.199726493772615,-0.130391022195898,-0.061066570408873,0.),
 .UNSPECIFIED.);
#942=B_SPLINE_CURVE_WITH_KNOTS('',3,(#20565,#20566,#20567,#20568,#20569,
#20570,#20571),.UNSPECIFIED.,.F.,.F.,(4,3,4),(2.91265948333354E-14,0.000871811007982302,
0.00160579165130123),.UNSPECIFIED.);
#943=B_SPLINE_CURVE_WITH_KNOTS('',3,(#20575,#20576,#20577,#20578,#20579,
#20580,#20581),.UNSPECIFIED.,.F.,.F.,(4,3,4),(4.06458703981066E-17,0.00087950080403512,
0.00156989029766391),.UNSPECIFIED.);
#944=B_SPLINE_CURVE_WITH_KNOTS('',3,(#20583,#20584,#20585,#20586,#20587,
#20588,#20589,#20590,#20591,#20592),.UNSPECIFIED.,.F.,.F.,(4,2,2,2,4),(-0.26072494343065,
-0.199726493772769,-0.130391022195999,-0.0610665704089316,0.),
 .UNSPECIFIED.);
#945=B_SPLINE_CURVE_WITH_KNOTS('',3,(#20594,#20595,#20596,#20597,#20598,
#20599,#20600),.UNSPECIFIED.,.F.,.F.,(4,3,4),(2.91191625685097E-14,0.000871811007980137,
0.00160579165129441),.UNSPECIFIED.);
#946=B_SPLINE_CURVE_WITH_KNOTS('',3,(#20604,#20605,#20606,#20607,#20608,
#20609,#20610),.UNSPECIFIED.,.F.,.F.,(4,3,4),(2.73734747335474E-17,0.000879500804032835,
0.00156989029766265),.UNSPECIFIED.);
#947=B_SPLINE_CURVE_WITH_KNOTS('',3,(#20612,#20613,#20614,#20615,#20616,
#20617,#20618,#20619,#20620,#20621),.UNSPECIFIED.,.F.,.F.,(4,2,2,2,4),(-0.260724943430845,
-0.199726493772884,-0.130391022196103,-0.061066570409027,0.),
 .UNSPECIFIED.);
#948=B_SPLINE_CURVE_WITH_KNOTS('',3,(#20623,#20624,#20625,#20626,#20627,
#20628,#20629),.UNSPECIFIED.,.F.,.F.,(4,3,4),(2.90751839301751E-14,0.000871811007988348,
0.00160579165129659),.UNSPECIFIED.);
#949=B_SPLINE_CURVE_WITH_KNOTS('',3,(#20633,#20634,#20635,#20636,#20637,
#20638,#20639),.UNSPECIFIED.,.F.,.F.,(4,3,4),(5.18389248106846E-17,0.000879500804056453,
0.00156989029764657),.UNSPECIFIED.);
#950=B_SPLINE_CURVE_WITH_KNOTS('',3,(#20641,#20642,#20643,#20644,#20645,
#20646,#20647,#20648,#20649,#20650),.UNSPECIFIED.,.F.,.F.,(4,2,2,2,4),(-0.260724943430446,
-0.199726493772451,-0.130391022195854,-0.0610665704089763,0.),
 .UNSPECIFIED.);
#951=B_SPLINE_CURVE_WITH_KNOTS('',3,(#20652,#20653,#20654,#20655,#20656,
#20657,#20658),.UNSPECIFIED.,.F.,.F.,(4,3,4),(2.91340106381937E-14,0.00087181100798855,
0.00160579165130922),.UNSPECIFIED.);
#952=B_SPLINE_CURVE_WITH_KNOTS('',3,(#20662,#20663,#20664,#20665,#20666,
#20667,#20668),.UNSPECIFIED.,.F.,.F.,(4,3,4),(5.56194657756796E-17,0.000879500804048824,
0.00156989029765731),.UNSPECIFIED.);
#953=B_SPLINE_CURVE_WITH_KNOTS('',3,(#20670,#20671,#20672,#20673,#20674,
#20675,#20676,#20677,#20678,#20679),.UNSPECIFIED.,.F.,.F.,(4,2,2,2,4),(-0.260724943430608,
-0.199726493772825,-0.130391022195954,-0.0610665704087948,0.),
 .UNSPECIFIED.);
#954=B_SPLINE_CURVE_WITH_KNOTS('',3,(#20681,#20682,#20683,#20684,#20685,
#20686,#20687),.UNSPECIFIED.,.F.,.F.,(4,3,4),(2.90925827778347E-14,0.000871811007964718,
0.00160579165129899),.UNSPECIFIED.);
#955=B_SPLINE_CURVE_WITH_KNOTS('',3,(#20691,#20692,#20693,#20694,#20695,
#20696,#20697),.UNSPECIFIED.,.F.,.F.,(4,3,4),(4.35066434406066E-17,0.000879500804046061,
0.00156989029765632),.UNSPECIFIED.);
#956=B_SPLINE_CURVE_WITH_KNOTS('',3,(#20699,#20700,#20701,#20702,#20703,
#20704,#20705,#20706,#20707,#20708),.UNSPECIFIED.,.F.,.F.,(4,2,2,2,4),(-0.260724943430643,
-0.199726494015738,-0.130391022447992,-0.0610665706515827,0.),
 .UNSPECIFIED.);
#957=B_SPLINE_CURVE_WITH_KNOTS('',3,(#20710,#20711,#20712,#20713,#20714,
#20715,#20716),.UNSPECIFIED.,.F.,.F.,(4,3,4),(3.46944695195361E-18,0.000871811004271182,
0.00160579165132782),.UNSPECIFIED.);
#958=B_SPLINE_CURVE_WITH_KNOTS('',3,(#20720,#20721,#20722,#20723,#20724,
#20725,#20726),.UNSPECIFIED.,.F.,.F.,(4,3,4),(1.27770362542414E-17,0.000879500804024833,
0.00156989029765982),.UNSPECIFIED.);
#959=B_SPLINE_CURVE_WITH_KNOTS('',3,(#20728,#20729,#20730,#20731,#20732,
#20733,#20734,#20735,#20736,#20737),.UNSPECIFIED.,.F.,.F.,(4,2,2,2,4),(-0.260724943430692,
-0.199726493772888,-0.130391022196012,-0.0610665704088243,0.),
 .UNSPECIFIED.);
#960=B_SPLINE_CURVE_WITH_KNOTS('',3,(#20739,#20740,#20741,#20742,#20743,
#20744,#20745),.UNSPECIFIED.,.F.,.F.,(4,3,4),(2.91292484701896E-14,0.000871811007984886,
0.00160579165129793),.UNSPECIFIED.);
#961=B_SPLINE_CURVE_WITH_KNOTS('',3,(#20749,#20750,#20751,#20752,#20753,
#20754,#20755),.UNSPECIFIED.,.F.,.F.,(4,3,4),(1.25393031850254E-17,0.00087950080402042,
0.00156989029765787),.UNSPECIFIED.);
#962=B_SPLINE_CURVE_WITH_KNOTS('',3,(#20757,#20758,#20759,#20760,#20761,
#20762,#20763,#20764,#20765,#20766),.UNSPECIFIED.,.F.,.F.,(4,2,2,2,4),(-0.26072494343069,
-0.199726493772886,-0.130391022196038,-0.0610665704088844,0.),
 .UNSPECIFIED.);
#963=B_SPLINE_CURVE_WITH_KNOTS('',3,(#20768,#20769,#20770,#20771,#20772,
#20773,#20774),.UNSPECIFIED.,.F.,.F.,(4,3,4),(2.90945543471338E-14,0.000871811007981126,
0.00160579165129904),.UNSPECIFIED.);
#964=B_SPLINE_CURVE_WITH_KNOTS('',3,(#20778,#20779,#20780,#20781,#20782,
#20783,#20784),.UNSPECIFIED.,.F.,.F.,(4,3,4),(3.46944695195361E-18,0.000879500804016519,
0.00156989029766726),.UNSPECIFIED.);
#965=B_SPLINE_CURVE_WITH_KNOTS('',3,(#20786,#20787,#20788,#20789,#20790,
#20791,#20792,#20793,#20794,#20795),.UNSPECIFIED.,.F.,.F.,(4,2,2,2,4),(-0.260724943430721,
-0.199726493772798,-0.130391022196058,-0.0610665704090037,0.),
 .UNSPECIFIED.);
#966=B_SPLINE_CURVE_WITH_KNOTS('',3,(#20797,#20798,#20799,#20800,#20801,
#20802,#20803),.UNSPECIFIED.,.F.,.F.,(4,3,4),(2.91013228173329E-14,0.000871811007991177,
0.0016057916512899),.UNSPECIFIED.);
#967=B_SPLINE_CURVE_WITH_KNOTS('',3,(#20807,#20808,#20809,#20810,#20811,
#20812,#20813),.UNSPECIFIED.,.F.,.F.,(4,3,4),(2.11749985874298E-17,0.000879500804033151,
0.00156989029764894),.UNSPECIFIED.);
#968=B_SPLINE_CURVE_WITH_KNOTS('',3,(#20815,#20816,#20817,#20818,#20819,
#20820,#20821,#20822,#20823,#20824),.UNSPECIFIED.,.F.,.F.,(4,2,2,2,4),(-0.26072494343059,
-0.199726494015698,-0.130391022447996,-0.0610665706516228,0.),
 .UNSPECIFIED.);
#969=B_SPLINE_CURVE_WITH_KNOTS('',3,(#20826,#20827,#20828,#20829,#20830,
#20831,#20832),.UNSPECIFIED.,.F.,.F.,(4,3,4),(1.73472347597681E-18,0.000871811004245289,
0.00160579165133993),.UNSPECIFIED.);
#970=B_SPLINE_CURVE_WITH_KNOTS('',3,(#20836,#20837,#20838,#20839,#20840,
#20841,#20842),.UNSPECIFIED.,.F.,.F.,(4,3,4),(1.29814818157976E-17,0.000879500804017423,
0.00156989029766904),.UNSPECIFIED.);
#971=B_SPLINE_CURVE_WITH_KNOTS('',3,(#20844,#20845,#20846,#20847,#20848,
#20849,#20850,#20851,#20852,#20853),.UNSPECIFIED.,.F.,.F.,(4,2,2,2,4),(-0.260724943430682,
-0.199726493772798,-0.130391022196032,-0.0610665704089836,0.),
 .UNSPECIFIED.);
#972=B_SPLINE_CURVE_WITH_KNOTS('',3,(#20855,#20856,#20857,#20858,#20859,
#20860,#20861),.UNSPECIFIED.,.F.,.F.,(4,3,4),(2.91001867197953E-14,0.000871811007999078,
0.00160579165129162),.UNSPECIFIED.);
#973=B_SPLINE_CURVE_WITH_KNOTS('',3,(#20865,#20866,#20867,#20868,#20869,
#20870,#20871),.UNSPECIFIED.,.F.,.F.,(4,3,4),(3.00963274664804E-17,0.000879500804029671,
0.00156989029766195),.UNSPECIFIED.);
#974=B_SPLINE_CURVE_WITH_KNOTS('',3,(#20873,#20874,#20875,#20876,#20877,
#20878,#20879,#20880,#20881,#20882),.UNSPECIFIED.,.F.,.F.,(4,2,2,2,4),(-0.260724943430772,
-0.199726493772819,-0.130391022196083,-0.0610665704090635,0.),
 .UNSPECIFIED.);
#975=B_SPLINE_CURVE_WITH_KNOTS('',3,(#20884,#20885,#20886,#20887,#20888,
#20889,#20890),.UNSPECIFIED.,.F.,.F.,(4,3,4),(2.90982160104274E-14,0.000871811007979976,
0.00160579165129827),.UNSPECIFIED.);
#976=B_SPLINE_CURVE_WITH_KNOTS('',3,(#20894,#20895,#20896,#20897,#20898,
#20899,#20900),.UNSPECIFIED.,.F.,.F.,(4,3,4),(1.30968750346023E-17,0.000879500804031867,
0.00156989029765141),.UNSPECIFIED.);
#977=B_SPLINE_CURVE_WITH_KNOTS('',3,(#20902,#20903,#20904,#20905,#20906,
#20907,#20908,#20909,#20910,#20911),.UNSPECIFIED.,.F.,.F.,(4,2,2,2,4),(-0.260724943430687,
-0.199726493772781,-0.130391022196041,-0.0610665704090031,0.),
 .UNSPECIFIED.);
#978=B_SPLINE_CURVE_WITH_KNOTS('',3,(#20913,#20914,#20915,#20916,#20917,
#20918,#20919),.UNSPECIFIED.,.F.,.F.,(4,3,4),(2.91087637723392E-14,0.000871811007963812,
0.00160579165130534),.UNSPECIFIED.);
#979=B_SPLINE_CURVE_WITH_KNOTS('',3,(#20923,#20924,#20925,#20926,#20927,
#20928,#20929),.UNSPECIFIED.,.F.,.F.,(4,3,4),(1.74337551706054E-17,0.000879500804024546,
0.00156989029766136),.UNSPECIFIED.);
#980=B_SPLINE_CURVE_WITH_KNOTS('',3,(#20931,#20932,#20933,#20934,#20935,
#20936,#20937,#20938,#20939,#20940),.UNSPECIFIED.,.F.,.F.,(4,2,2,2,4),(-0.260724943430695,
-0.199726493772679,-0.130391022195957,-0.0610665704089199,0.),
 .UNSPECIFIED.);
#981=B_SPLINE_CURVE_WITH_KNOTS('',3,(#20942,#20943,#20944,#20945,#20946,
#20947,#20948),.UNSPECIFIED.,.F.,.F.,(4,3,4),(2.91042167107766E-14,0.000871811007980219,
0.00160579165129469),.UNSPECIFIED.);
#982=B_SPLINE_CURVE_WITH_KNOTS('',3,(#20952,#20953,#20954,#20955,#20956,
#20957,#20958),.UNSPECIFIED.,.F.,.F.,(4,3,4),(2.4532694666934E-17,0.000879500804036203,
0.00156989029764486),.UNSPECIFIED.);
#983=B_SPLINE_CURVE_WITH_KNOTS('',3,(#20960,#20961,#20962,#20963,#20964,
#20965,#20966,#20967,#20968,#20969),.UNSPECIFIED.,.F.,.F.,(4,2,2,2,4),(-0.260724943430608,
-0.199726493772553,-0.130391022195942,-0.0610665704090163,0.),
 .UNSPECIFIED.);
#984=B_SPLINE_CURVE_WITH_KNOTS('',3,(#20971,#20972,#20973,#20974,#20975,
#20976,#20977),.UNSPECIFIED.,.F.,.F.,(4,3,4),(2.91014911109026E-14,0.000871811007975891,
0.00160579165131238),.UNSPECIFIED.);
#985=B_SPLINE_CURVE_WITH_KNOTS('',3,(#20981,#20982,#20983,#20984,#20985,
#20986,#20987),.UNSPECIFIED.,.F.,.F.,(4,3,4),(1.35486234660355E-17,0.000879500804022474,
0.00156989029765048),.UNSPECIFIED.);
#986=B_SPLINE_CURVE_WITH_KNOTS('',3,(#20989,#20990,#20991,#20992,#20993,
#20994,#20995,#20996,#20997,#20998),.UNSPECIFIED.,.F.,.F.,(4,2,2,2,4),(-0.260724943430529,
-0.199726493772671,-0.130391022195944,-0.0610665704089295,0.),
 .UNSPECIFIED.);
#987=B_SPLINE_CURVE_WITH_KNOTS('',3,(#21000,#21001,#21002,#21003,#21004,
#21005,#21006),.UNSPECIFIED.,.F.,.F.,(4,3,4),(2.9101180116032E-14,0.000871811007967255,
0.00160579165130327),.UNSPECIFIED.);
#988=B_SPLINE_CURVE_WITH_KNOTS('',3,(#21010,#21011,#21012,#21013,#21014,
#21015,#21016),.UNSPECIFIED.,.F.,.F.,(4,3,4),(1.16368788433466E-17,0.000879500804019555,
0.00156989029765596),.UNSPECIFIED.);
#989=B_SPLINE_CURVE_WITH_KNOTS('',3,(#21018,#21019,#21020,#21021,#21022,
#21023,#21024,#21025,#21026,#21027),.UNSPECIFIED.,.F.,.F.,(4,2,2,2,4),(-0.260724943430678,
-0.199726493772776,-0.130391022196033,-0.0610665704089837,0.),
 .UNSPECIFIED.);
#990=B_SPLINE_CURVE_WITH_KNOTS('',3,(#21029,#21030,#21031,#21032,#21033,
#21034,#21035),.UNSPECIFIED.,.F.,.F.,(4,3,4),(2.91000394628375E-14,0.000871811007976233,
0.00160579165130128),.UNSPECIFIED.);
#991=B_SPLINE_CURVE_WITH_KNOTS('',3,(#21039,#21040,#21041,#21042,#21043,
#21044,#21045),.UNSPECIFIED.,.F.,.F.,(4,3,4),(1.9930455364338E-17,0.000879500804026383,
0.00156989029765913),.UNSPECIFIED.);
#992=B_SPLINE_CURVE_WITH_KNOTS('',3,(#21047,#21048,#21049,#21050,#21051,
#21052,#21053,#21054,#21055,#21056),.UNSPECIFIED.,.F.,.F.,(4,2,2,2,4),(-0.260520353691811,
-0.209093406725458,-0.154219975172592,-0.0839882141543201,-0.0483220958496221),
 .UNSPECIFIED.);
#993=B_SPLINE_CURVE_WITH_KNOTS('',3,(#21061,#21062,#21063,#21064,#21065,
#21066),.UNSPECIFIED.,.F.,.F.,(4,2,4),(-0.0483220958496221,-0.0407569430592836,
0.),.UNSPECIFIED.);
#994=B_SPLINE_CURVE_WITH_KNOTS('',3,(#21068,#21069,#21070,#21071,#21072,
#21073,#21074),.UNSPECIFIED.,.F.,.F.,(4,3,4),(2.90906258208131E-14,0.000871811007977714,
0.00160579165130056),.UNSPECIFIED.);
#995=B_SPLINE_CURVE_WITH_KNOTS('',3,(#21078,#21079,#21080,#21081,#21082,
#21083,#21084),.UNSPECIFIED.,.F.,.F.,(4,3,4),(2.22829265085925E-17,0.000879500804029387,
0.00156989029765885),.UNSPECIFIED.);
#996=B_SPLINE_CURVE_WITH_KNOTS('',3,(#21086,#21087,#21088,#21089,#21090,
#21091,#21092,#21093,#21094,#21095),.UNSPECIFIED.,.F.,.F.,(4,2,2,2,4),(-0.260724943430766,
-0.199726494015728,-0.130391022448065,-0.061066570651741,0.),
 .UNSPECIFIED.);
#997=B_SPLINE_CURVE_WITH_KNOTS('',3,(#21097,#21098,#21099,#21100,#21101,
#21102,#21103),.UNSPECIFIED.,.F.,.F.,(4,3,4),(3.5762240613455E-18,0.00087181100425516,
0.00160579165132772),.UNSPECIFIED.);
#998=B_SPLINE_CURVE_WITH_KNOTS('',3,(#21107,#21108,#21109,#21110,#21111,
#21112,#21113),.UNSPECIFIED.,.F.,.F.,(4,3,4),(1.96261557335472E-17,0.000879500804038629,
0.00156989029765915),.UNSPECIFIED.);
#999=B_SPLINE_CURVE_WITH_KNOTS('',3,(#21115,#21116,#21117,#21118,#21119,
#21120,#21121,#21122,#21123,#21124),.UNSPECIFIED.,.F.,.F.,(4,2,2,2,4),(-0.260724943430666,
-0.199726493772782,-0.130391022196017,-0.0610665704089714,0.),
 .UNSPECIFIED.);
#1000=B_SPLINE_CURVE_WITH_KNOTS('',3,(#21126,#21127,#21128,#21129,#21130,
#21131,#21132),.UNSPECIFIED.,.F.,.F.,(4,3,4),(2.91001126777664E-14,0.000871811007981504,
0.00160579165129883),.UNSPECIFIED.);
#1001=B_SPLINE_CURVE_WITH_KNOTS('',3,(#21136,#21137,#21138,#21139,#21140,
#21141,#21142),.UNSPECIFIED.,.F.,.F.,(4,3,4),(2.7318452618149E-17,0.000879500804037613,
0.00156989029765498),.UNSPECIFIED.);
#1002=B_SPLINE_CURVE_WITH_KNOTS('',3,(#21144,#21145,#21146,#21147,#21148,
#21149,#21150,#21151,#21152,#21153),.UNSPECIFIED.,.F.,.F.,(4,2,2,2,4),(-0.260724943430572,
-0.199726493772594,-0.13039102219594,-0.0610665704089772,0.),
 .UNSPECIFIED.);
#1003=B_SPLINE_CURVE_WITH_KNOTS('',3,(#21155,#21156,#21157,#21158,#21159,
#21160,#21161),.UNSPECIFIED.,.F.,.F.,(4,3,4),(2.91359063697315E-14,0.000871811007969042,
0.00160579165130329),.UNSPECIFIED.);
#1004=B_SPLINE_CURVE_WITH_KNOTS('',3,(#21165,#21166,#21167,#21168,#21169,
#21170,#21171),.UNSPECIFIED.,.F.,.F.,(4,3,4),(2.32737576866932E-17,0.000879500804023078,
0.00156989029766054),.UNSPECIFIED.);
#1005=B_SPLINE_CURVE_WITH_KNOTS('',3,(#21173,#21174,#21175,#21176,#21177,
#21178,#21179,#21180,#21181,#21182),.UNSPECIFIED.,.F.,.F.,(4,2,2,2,4),(-0.260724943430778,
-0.199726493772851,-0.130391022196053,-0.0610665704089545,0.),
 .UNSPECIFIED.);
#1006=B_SPLINE_CURVE_WITH_KNOTS('',3,(#21184,#21185,#21186,#21187,#21188,
#21189,#21190),.UNSPECIFIED.,.F.,.F.,(4,3,4),(2.91132655738402E-14,0.000871811007988041,
0.00160579165129781),.UNSPECIFIED.);
#1007=B_SPLINE_CURVE_WITH_KNOTS('',3,(#21194,#21195,#21196,#21197,#21198,
#21199,#21200),.UNSPECIFIED.,.F.,.F.,(4,3,4),(3.24073089410192E-17,0.000879500804029647,
0.00156989029765669),.UNSPECIFIED.);
#1008=B_SPLINE_CURVE_WITH_KNOTS('',3,(#21202,#21203,#21204,#21205,#21206,
#21207,#21208,#21209,#21210,#21211),.UNSPECIFIED.,.F.,.F.,(4,2,2,2,4),(-0.260724943430862,
-0.199726493772895,-0.130391022196119,-0.0610665704090545,0.),
 .UNSPECIFIED.);
#1009=B_SPLINE_CURVE_WITH_KNOTS('',3,(#21213,#21214,#21215,#21216,#21217,
#21218,#21219),.UNSPECIFIED.,.F.,.F.,(4,3,4),(2.91067438627834E-14,0.0008718110079958,
0.00160579165130139),.UNSPECIFIED.);
#1010=B_SPLINE_CURVE_WITH_KNOTS('',3,(#21223,#21224,#21225,#21226,#21227,
#21228,#21229),.UNSPECIFIED.,.F.,.F.,(4,3,4),(2.92855028701906E-17,0.000879500804033521,
0.00156989029764515),.UNSPECIFIED.);
#1011=B_SPLINE_CURVE_WITH_KNOTS('',3,(#21231,#21232,#21233,#21234,#21235,
#21236,#21237,#21238,#21239,#21240),.UNSPECIFIED.,.F.,.F.,(4,2,2,2,4),(-0.260724943430445,
-0.199726493772613,-0.130391022195896,-0.0610665704088579,0.),
 .UNSPECIFIED.);
#1012=B_SPLINE_CURVE_WITH_KNOTS('',3,(#21242,#21243,#21244,#21245,#21246,
#21247,#21248),.UNSPECIFIED.,.F.,.F.,(4,3,4),(2.91087637723392E-14,0.000871811007984256,
0.00160579165131312),.UNSPECIFIED.);
#1013=B_SPLINE_CURVE_WITH_KNOTS('',3,(#21252,#21253,#21254,#21255,#21256,
#21257,#21258),.UNSPECIFIED.,.F.,.F.,(4,3,4),(3.63878666146591E-17,0.000879500804036169,
0.00156989029767024),.UNSPECIFIED.);
#1014=B_SPLINE_CURVE_WITH_KNOTS('',3,(#21260,#21261,#21262,#21263,#21264,
#21265,#21266,#21267,#21268,#21269),.UNSPECIFIED.,.F.,.F.,(4,2,2,2,4),(-0.26072494343082,
-0.199726493772798,-0.130391022196048,-0.0610665704089677,0.),
 .UNSPECIFIED.);
#1015=B_SPLINE_CURVE_WITH_KNOTS('',3,(#21271,#21272,#21273,#21274,#21275,
#21276,#21277),.UNSPECIFIED.,.F.,.F.,(4,3,4),(2.91241109924099E-14,0.000871811007978442,
0.00160579165128969),.UNSPECIFIED.);
#1016=B_SPLINE_CURVE_WITH_KNOTS('',3,(#21281,#21282,#21283,#21284,#21285,
#21286,#21287),.UNSPECIFIED.,.F.,.F.,(4,3,4),(2.08166817117217E-17,0.000879500804019574,
0.00156989029766826),.UNSPECIFIED.);
#1017=B_SPLINE_CURVE_WITH_KNOTS('',3,(#21289,#21290,#21291,#21292,#21293,
#21294,#21295,#21296,#21297,#21298),.UNSPECIFIED.,.F.,.F.,(4,2,2,2,4),(-0.260724943430785,
-0.199726493772819,-0.130391022196044,-0.0610665704089591,0.),
 .UNSPECIFIED.);
#1018=B_SPLINE_CURVE_WITH_KNOTS('',3,(#21300,#21301,#21302,#21303,#21304,
#21305,#21306),.UNSPECIFIED.,.F.,.F.,(4,3,4),(2.91043716495764E-14,0.000871811007981064,
0.00160579165128749),.UNSPECIFIED.);
#1019=B_SPLINE_CURVE_WITH_KNOTS('',3,(#21310,#21311,#21312,#21313,#21314,
#21315,#21316),.UNSPECIFIED.,.F.,.F.,(4,3,4),(1.97026712507607E-17,0.000879500804023626,
0.00156989029766686),.UNSPECIFIED.);
#1020=B_SPLINE_CURVE_WITH_KNOTS('',3,(#21318,#21319,#21320,#21321,#21322,
#21323,#21324,#21325,#21326,#21327),.UNSPECIFIED.,.F.,.F.,(4,2,2,2,4),(-0.260724943430759,
-0.199726493772798,-0.130391022196069,-0.0610665704090458,0.),
 .UNSPECIFIED.);
#1021=B_SPLINE_CURVE_WITH_KNOTS('',3,(#21329,#21330,#21331,#21332,#21333,
#21334,#21335),.UNSPECIFIED.,.F.,.F.,(4,3,4),(2.90643704185478E-14,0.000871811007973552,
0.00160579165129078),.UNSPECIFIED.);
#1022=B_SPLINE_CURVE_WITH_KNOTS('',3,(#21339,#21340,#21341,#21342,#21343,
#21344,#21345),.UNSPECIFIED.,.F.,.F.,(4,3,4),(3.94435074910981E-17,0.000879500804033538,
0.00156989029765321),.UNSPECIFIED.);
#1023=B_SPLINE_CURVE_WITH_KNOTS('',3,(#21347,#21348,#21349,#21350,#21351,
#21352,#21353,#21354,#21355,#21356),.UNSPECIFIED.,.F.,.F.,(4,2,2,2,4),(-0.260724943430726,
-0.199726493772705,-0.130391022196008,-0.0610665704090159,0.),
 .UNSPECIFIED.);
#1024=B_SPLINE_CURVE_WITH_KNOTS('',3,(#21358,#21359,#21360,#21361,#21362,
#21363,#21364),.UNSPECIFIED.,.F.,.F.,(4,3,4),(2.90938207050466E-14,0.000871811007985816,
0.00160579165130088),.UNSPECIFIED.);
#1025=B_SPLINE_CURVE_WITH_KNOTS('',3,(#21368,#21369,#21370,#21371,#21372,
#21373,#21374),.UNSPECIFIED.,.F.,.F.,(4,3,4),(1.86885762303156E-17,0.000879500804024845,
0.00156989029765983),.UNSPECIFIED.);
#1026=B_SPLINE_CURVE_WITH_KNOTS('',3,(#21376,#21377,#21378,#21379,#21380,
#21381,#21382,#21383,#21384,#21385),.UNSPECIFIED.,.F.,.F.,(4,2,2,2,4),(-0.260724943430608,
-0.199726493772826,-0.130391022195969,-0.0610665704088119,0.),
 .UNSPECIFIED.);
#1027=B_SPLINE_CURVE_WITH_KNOTS('',3,(#21387,#21388,#21389,#21390,#21391,
#21392,#21393),.UNSPECIFIED.,.F.,.F.,(4,3,4),(2.91304865854723E-14,0.000871811007993082,
0.00160579165129793),.UNSPECIFIED.);
#1028=B_SPLINE_CURVE_WITH_KNOTS('',3,(#21397,#21398,#21399,#21400,#21401,
#21402,#21403),.UNSPECIFIED.,.F.,.F.,(4,3,4),(2.22829265085925E-17,0.000879500804025998,
0.00156989029765836),.UNSPECIFIED.);
#1029=B_SPLINE_CURVE_WITH_KNOTS('',3,(#21405,#21406,#21407,#21408,#21409,
#21410,#21411,#21412,#21413,#21414),.UNSPECIFIED.,.F.,.F.,(4,2,2,2,4),(-0.260724943430637,
-0.199726493772782,-0.130391022195983,-0.0610665704088931,0.),
 .UNSPECIFIED.);
#1030=B_SPLINE_CURVE_WITH_KNOTS('',3,(#21416,#21417,#21418,#21419,#21420,
#21421,#21422),.UNSPECIFIED.,.F.,.F.,(4,3,4),(2.91247662370936E-14,0.000871811007979228,
0.00160579165130031),.UNSPECIFIED.);
#1031=B_SPLINE_CURVE_WITH_KNOTS('',3,(#21426,#21427,#21428,#21429,#21430,
#21431,#21432),.UNSPECIFIED.,.F.,.F.,(4,3,4),(2.0888836804026E-17,0.00087950080401925,
0.00156989029766913),.UNSPECIFIED.);
#1032=B_SPLINE_CURVE_WITH_KNOTS('',3,(#21434,#21435,#21436,#21437,#21438,
#21439,#21440,#21441,#21442,#21443),.UNSPECIFIED.,.F.,.F.,(4,2,2,2,4),(-0.26072494343068,
-0.199726493772826,-0.13039102219598,-0.0610665704088353,0.),
 .UNSPECIFIED.);
#1033=B_SPLINE_CURVE_WITH_KNOTS('',3,(#21445,#21446,#21447,#21448,#21449,
#21450,#21451),.UNSPECIFIED.,.F.,.F.,(4,3,4),(2.91135465160192E-14,0.000871811007985186,
0.00160579165128965),.UNSPECIFIED.);
#1034=B_SPLINE_CURVE_WITH_KNOTS('',3,(#21455,#21456,#21457,#21458,#21459,
#21460,#21461),.UNSPECIFIED.,.F.,.F.,(4,3,4),(2.11749985874298E-17,0.000879500804028422,
0.00156989029765732),.UNSPECIFIED.);
#1035=B_SPLINE_CURVE_WITH_KNOTS('',3,(#21463,#21464,#21465,#21466,#21467,
#21468,#21469,#21470,#21471,#21472),.UNSPECIFIED.,.F.,.F.,(4,2,2,2,4),(-0.260724943430486,
-0.199726494015597,-0.130391022447942,-0.0610665706516372,0.),
 .UNSPECIFIED.);
#1036=B_SPLINE_CURVE_WITH_KNOTS('',3,(#21474,#21475,#21476,#21477,#21478,
#21479,#21480),.UNSPECIFIED.,.F.,.F.,(4,3,4),(0.,0.000871811004269854,0.00160579165133273),
 .UNSPECIFIED.);
#1037=B_SPLINE_CURVE_WITH_KNOTS('',3,(#21484,#21485,#21486,#21487,#21488,
#21489,#21490),.UNSPECIFIED.,.F.,.F.,(4,3,4),(3.0245937307082E-17,0.000879500804036986,
0.00156989029766962),.UNSPECIFIED.);
#1038=B_SPLINE_CURVE_WITH_KNOTS('',3,(#21492,#21493,#21494,#21495,#21496,
#21497,#21498,#21499,#21500,#21501),.UNSPECIFIED.,.F.,.F.,(4,2,2,2,4),(-0.260724943430712,
-0.19972649401573,-0.130391022448006,-0.061066570651615,0.),
 .UNSPECIFIED.);
#1039=B_SPLINE_CURVE_WITH_KNOTS('',3,(#21503,#21504,#21505,#21506,#21507,
#21508,#21509),.UNSPECIFIED.,.F.,.F.,(4,3,4),(9.34177181294034E-18,0.000871811004264771,
0.0016057916513195),.UNSPECIFIED.);
#1040=B_SPLINE_CURVE_WITH_KNOTS('',3,(#21513,#21514,#21515,#21516,#21517,
#21518,#21519),.UNSPECIFIED.,.F.,.F.,(4,3,4),(4.16333634234434E-17,0.000879500804025556,
0.00156989029766107),.UNSPECIFIED.);
#1041=B_SPLINE_CURVE_WITH_KNOTS('',3,(#21521,#21522,#21523,#21524,#21525,
#21526,#21527,#21528,#21529,#21530),.UNSPECIFIED.,.F.,.F.,(4,2,2,2,4),(-0.260724943430731,
-0.199726493772769,-0.130391022196028,-0.0610665704089995,0.),
 .UNSPECIFIED.);
#1042=B_SPLINE_CURVE_WITH_KNOTS('',3,(#21532,#21533,#21534,#21535,#21536,
#21537,#21538),.UNSPECIFIED.,.F.,.F.,(4,3,4),(2.9112405365365E-14,0.000871811007989186,
0.00160579165129583),.UNSPECIFIED.);
#1043=B_SPLINE_CURVE_WITH_KNOTS('',3,(#21542,#21543,#21544,#21545,#21546,
#21547,#21548),.UNSPECIFIED.,.F.,.F.,(4,3,4),(3.04442734473391E-17,0.000879500804017925,
0.00156989029765869),.UNSPECIFIED.);
#1044=B_SPLINE_CURVE_WITH_KNOTS('',3,(#21550,#21551,#21552,#21553,#21554,
#21555,#21556,#21557,#21558,#21559),.UNSPECIFIED.,.F.,.F.,(4,2,2,2,4),(-0.260724943430665,
-0.199726493772749,-0.130391022196018,-0.0610665704090143,0.),
 .UNSPECIFIED.);
#1045=B_SPLINE_CURVE_WITH_KNOTS('',3,(#21561,#21562,#21563,#21564,#21565,
#21566,#21567),.UNSPECIFIED.,.F.,.F.,(4,3,4),(2.9097154720412E-14,0.000871811007991494,
0.00160579165130179),.UNSPECIFIED.);
#1046=B_SPLINE_CURVE_WITH_KNOTS('',3,(#21571,#21572,#21573,#21574,#21575,
#21576,#21577),.UNSPECIFIED.,.F.,.F.,(4,3,4),(1.74337551706054E-17,0.000879500804021092,
0.00156989029765673),.UNSPECIFIED.);
#1047=B_SPLINE_CURVE_WITH_KNOTS('',3,(#21579,#21580,#21581,#21582,#21583,
#21584,#21585,#21586,#21587,#21588),.UNSPECIFIED.,.F.,.F.,(4,2,2,2,4),(-0.260724943430631,
-0.199726493772786,-0.130391022195963,-0.0610665704088755,0.),
 .UNSPECIFIED.);
#1048=B_SPLINE_CURVE_WITH_KNOTS('',3,(#21590,#21591,#21592,#21593,#21594,
#21595,#21596),.UNSPECIFIED.,.F.,.F.,(4,3,4),(2.90847295664599E-14,0.000871811007970203,
0.00160579165130329),.UNSPECIFIED.);
#1049=B_SPLINE_CURVE_WITH_KNOTS('',3,(#21600,#21601,#21602,#21603,#21604,
#21605,#21606),.UNSPECIFIED.,.F.,.F.,(4,3,4),(3.87895961444886E-17,0.000879500804034552,
0.00156989029765527),.UNSPECIFIED.);
#1050=B_SPLINE_CURVE_WITH_KNOTS('',3,(#21608,#21609,#21610,#21611,#21612,
#21613,#21614,#21615,#21616,#21617),.UNSPECIFIED.,.F.,.F.,(4,2,2,2,4),(-0.260724943430537,
-0.199726493772744,-0.130391022195923,-0.061066570408807,0.),
 .UNSPECIFIED.);
#1051=B_SPLINE_CURVE_WITH_KNOTS('',3,(#21619,#21620,#21621,#21622,#21623,
#21624,#21625),.UNSPECIFIED.,.F.,.F.,(4,3,4),(2.9092974958669E-14,0.000871811007970566,
0.00160579165130425),.UNSPECIFIED.);
#1052=B_SPLINE_CURVE_WITH_KNOTS('',3,(#21629,#21630,#21631,#21632,#21633,
#21634,#21635),.UNSPECIFIED.,.F.,.F.,(4,3,4),(2.57885184514585E-17,0.00087950080403597,
0.00156989029765865),.UNSPECIFIED.);
#1053=B_SPLINE_CURVE_WITH_KNOTS('',3,(#21637,#21638,#21639,#21640,#21641,
#21642,#21643,#21644,#21645,#21646),.UNSPECIFIED.,.F.,.F.,(4,2,2,2,4),(-0.260724943430618,
-0.199726493772736,-0.130391022195974,-0.0610665704089162,0.),
 .UNSPECIFIED.);
#1054=B_SPLINE_CURVE_WITH_KNOTS('',3,(#21648,#21649,#21650,#21651,#21652,
#21653,#21654),.UNSPECIFIED.,.F.,.F.,(4,3,4),(2.91294464430763E-14,0.000871811007972832,
0.00160579165129869),.UNSPECIFIED.);
#1055=B_SPLINE_CURVE_WITH_KNOTS('',3,(#21658,#21659,#21660,#21661,#21662,
#21663,#21664),.UNSPECIFIED.,.F.,.F.,(4,3,4),(2.32737576866932E-17,0.000879500804029127,
0.0015698902976571),.UNSPECIFIED.);
#1056=B_SPLINE_CURVE_WITH_KNOTS('',3,(#21666,#21667,#21668,#21669,#21670,
#21671,#21672,#21673,#21674,#21675),.UNSPECIFIED.,.F.,.F.,(4,2,2,2,4),(-0.260724943430665,
-0.199726493772715,-0.130391022195962,-0.0610665704089159,0.),
 .UNSPECIFIED.);
#1057=B_SPLINE_CURVE_WITH_KNOTS('',3,(#21677,#21678,#21679,#21680,#21681,
#21682,#21683),.UNSPECIFIED.,.F.,.F.,(4,3,4),(2.90901901300838E-14,0.000871811007981293,
0.00160579165130176),.UNSPECIFIED.);
#1058=B_SPLINE_CURVE_WITH_KNOTS('',3,(#21686,#21687,#21688,#21689,#21690,
#21691,#21692),.UNSPECIFIED.,.F.,.F.,(4,3,4),(1.75413055748779E-17,0.000879500804021358,
0.00156989029765893),.UNSPECIFIED.);
#1059=B_SPLINE_CURVE_WITH_KNOTS('',3,(#21694,#21695,#21696,#21697,#21698,
#21699),.UNSPECIFIED.,.F.,.F.,(4,2,4),(1.00000018525999E-6,0.161245973868135,
0.321302696423032),.UNSPECIFIED.);
#1060=B_SPLINE_CURVE_WITH_KNOTS('',3,(#21700,#21701,#21702,#21703,#21704,
#21705),.UNSPECIFIED.,.F.,.F.,(4,2,4),(1.00000020281465E-6,0.1667794805349,
0.332956960668741),.UNSPECIFIED.);
#1061=B_SPLINE_CURVE_WITH_KNOTS('',3,(#21707,#21708,#21709,#21710,#21711,
#21712),.UNSPECIFIED.,.F.,.F.,(4,2,4),(1.00000020232593E-6,0.166779480533119,
0.33295696066984),.UNSPECIFIED.);
#1062=B_SPLINE_CURVE_WITH_KNOTS('',3,(#21713,#21714,#21715,#21716,#21717,
#21718),.UNSPECIFIED.,.F.,.F.,(4,2,4),(1.00000018558043E-6,0.161245973866302,
0.321302696447619),.UNSPECIFIED.);
#1063=B_SPLINE_CURVE_WITH_KNOTS('',3,(#21720,#21721,#21722,#21723,#21724,
#21725),.UNSPECIFIED.,.F.,.F.,(4,2,4),(1.00000018541071E-6,0.161245467064344,
0.321302696404247),.UNSPECIFIED.);
#1064=B_SPLINE_CURVE_WITH_KNOTS('',3,(#21726,#21727,#21728,#21729,#21730,
#21731),.UNSPECIFIED.,.F.,.F.,(4,2,4),(1.00000020240854E-6,0.1667794805253,
0.332956960639582),.UNSPECIFIED.);
#1065=B_SPLINE_CURVE_WITH_KNOTS('',3,(#21733,#21734,#21735,#21736,#21737,
#21738),.UNSPECIFIED.,.F.,.F.,(4,2,4),(1.00000018516492E-6,0.161245973870214,
0.32130269640169),.UNSPECIFIED.);
#1066=B_SPLINE_CURVE_WITH_KNOTS('',3,(#21739,#21740,#21741,#21742,#21743,
#21744),.UNSPECIFIED.,.F.,.F.,(4,2,4),(1.00000020306044E-6,0.166779480520393,
0.332956960668093),.UNSPECIFIED.);
#1067=B_SPLINE_CURVE_WITH_KNOTS('',3,(#21746,#21747,#21748,#21749,#21750,
#21751),.UNSPECIFIED.,.F.,.F.,(4,2,4),(1.00000018495189E-6,0.161245467061803,
0.321302696480035),.UNSPECIFIED.);
#1068=B_SPLINE_CURVE_WITH_KNOTS('',3,(#21752,#21753,#21754,#21755,#21756,
#21757),.UNSPECIFIED.,.F.,.F.,(4,2,4),(1.00000020291508E-6,0.166779480527622,
0.332956960694064),.UNSPECIFIED.);
#1069=B_SPLINE_CURVE_WITH_KNOTS('',3,(#21759,#21760,#21761,#21762,#21763,
#21764),.UNSPECIFIED.,.F.,.F.,(4,2,4),(1.00000018524296E-6,0.161245467067315,
0.321302696528087),.UNSPECIFIED.);
#1070=B_SPLINE_CURVE_WITH_KNOTS('',3,(#21765,#21766,#21767,#21768,#21769,
#21770),.UNSPECIFIED.,.F.,.F.,(4,2,4),(1.00000020251295E-6,0.166779480532976,
0.332956960702249),.UNSPECIFIED.);
#1071=B_SPLINE_CURVE_WITH_KNOTS('',3,(#21772,#21773,#21774,#21775,#21776,
#21777),.UNSPECIFIED.,.F.,.F.,(4,2,4),(1.00000018551213E-6,0.161245467070566,
0.321302696524444),.UNSPECIFIED.);
#1072=B_SPLINE_CURVE_WITH_KNOTS('',3,(#21778,#21779,#21780,#21781,#21782,
#21783),.UNSPECIFIED.,.F.,.F.,(4,2,4),(1.00000020265717E-6,0.166779480531078,
0.332956960668084),.UNSPECIFIED.);
#1073=B_SPLINE_CURVE_WITH_KNOTS('',3,(#21785,#21786,#21787,#21788,#21789,
#21790),.UNSPECIFIED.,.F.,.F.,(4,2,4),(1.00000018518735E-6,0.161245467061048,
0.321302696421221),.UNSPECIFIED.);
#1074=B_SPLINE_CURVE_WITH_KNOTS('',3,(#21791,#21792,#21793,#21794,#21795,
#21796),.UNSPECIFIED.,.F.,.F.,(4,2,4),(1.000000202362E-6,0.166779480540548,
0.332956960686337),.UNSPECIFIED.);
#1075=B_SPLINE_CURVE_WITH_KNOTS('',3,(#21798,#21799,#21800,#21801,#21802,
#21803),.UNSPECIFIED.,.F.,.F.,(4,2,4),(1.00000018537216E-6,0.161245973869415,
0.321302696413987),.UNSPECIFIED.);
#1076=B_SPLINE_CURVE_WITH_KNOTS('',3,(#21804,#21805,#21806,#21807,#21808,
#21809),.UNSPECIFIED.,.F.,.F.,(4,2,4),(1.00000020298589E-6,0.166779480532959,
0.332956960659601),.UNSPECIFIED.);
#1077=B_SPLINE_CURVE_WITH_KNOTS('',3,(#21811,#21812,#21813,#21814,#21815,
#21816),.UNSPECIFIED.,.F.,.F.,(4,2,4),(1.00000018494672E-6,0.161245973865759,
0.321302696389016),.UNSPECIFIED.);
#1078=B_SPLINE_CURVE_WITH_KNOTS('',3,(#21817,#21818,#21819,#21820,#21821,
#21822),.UNSPECIFIED.,.F.,.F.,(4,2,4),(1.00000020269192E-6,0.166779480525868,
0.332956960672747),.UNSPECIFIED.);
#1079=B_SPLINE_CURVE_WITH_KNOTS('',3,(#21824,#21825,#21826,#21827,#21828,
#21829),.UNSPECIFIED.,.F.,.F.,(4,2,4),(1.00000018523224E-6,0.161245467065664,
0.321302696484184),.UNSPECIFIED.);
#1080=B_SPLINE_CURVE_WITH_KNOTS('',3,(#21830,#21831,#21832,#21833,#21834,
#21835),.UNSPECIFIED.,.F.,.F.,(4,2,4),(1.00000020265587E-6,0.166779480529505,
0.332956960668596),.UNSPECIFIED.);
#1081=B_SPLINE_CURVE_WITH_KNOTS('',3,(#21837,#21838,#21839,#21840,#21841,
#21842),.UNSPECIFIED.,.F.,.F.,(4,2,4),(1.00000018523152E-6,0.161245973866936,
0.321302696434055),.UNSPECIFIED.);
#1082=B_SPLINE_CURVE_WITH_KNOTS('',3,(#21843,#21844,#21845,#21846,#21847,
#21848),.UNSPECIFIED.,.F.,.F.,(4,2,4),(1.00000020282499E-6,0.16677948053055,
0.332956960655279),.UNSPECIFIED.);
#1083=B_SPLINE_CURVE_WITH_KNOTS('',3,(#21850,#21851,#21852,#21853,#21854,
#21855),.UNSPECIFIED.,.F.,.F.,(4,2,4),(1.00000018488197E-6,0.161245467060642,
0.321302696386487),.UNSPECIFIED.);
#1084=B_SPLINE_CURVE_WITH_KNOTS('',3,(#21856,#21857,#21858,#21859,#21860,
#21861),.UNSPECIFIED.,.F.,.F.,(4,2,4),(1.00000020310365E-6,0.16677948052756,
0.332956960677708),.UNSPECIFIED.);
#1085=B_SPLINE_CURVE_WITH_KNOTS('',3,(#21863,#21864,#21865,#21866,#21867,
#21868),.UNSPECIFIED.,.F.,.F.,(4,2,4),(1.00000018517987E-6,0.161245973870067,
0.321302696479206),.UNSPECIFIED.);
#1086=B_SPLINE_CURVE_WITH_KNOTS('',3,(#21869,#21870,#21871,#21872,#21873,
#21874),.UNSPECIFIED.,.F.,.F.,(4,2,4),(1.00000020285339E-6,0.166779480523092,
0.332956960656032),.UNSPECIFIED.);
#1087=B_SPLINE_CURVE_WITH_KNOTS('',3,(#21876,#21877,#21878,#21879,#21880,
#21881),.UNSPECIFIED.,.F.,.F.,(4,2,4),(1.00000018502563E-6,0.161245467059883,
0.321302696428097),.UNSPECIFIED.);
#1088=B_SPLINE_CURVE_WITH_KNOTS('',3,(#21882,#21883,#21884,#21885,#21886,
#21887),.UNSPECIFIED.,.F.,.F.,(4,2,4),(1.00000020277303E-6,0.166779480528052,
0.33295696065521),.UNSPECIFIED.);
#1089=B_SPLINE_CURVE_WITH_KNOTS('',3,(#21889,#21890,#21891,#21892,#21893,
#21894),.UNSPECIFIED.,.F.,.F.,(4,2,4),(1.00000018537403E-6,0.161245467061688,
0.321302696397048),.UNSPECIFIED.);
#1090=B_SPLINE_CURVE_WITH_KNOTS('',3,(#21895,#21896,#21897,#21898,#21899,
#21900),.UNSPECIFIED.,.F.,.F.,(4,2,4),(1.00000020322115E-6,0.166779480526764,
0.332956960619472),.UNSPECIFIED.);
#1091=B_SPLINE_CURVE_WITH_KNOTS('',3,(#21902,#21903,#21904,#21905,#21906,
#21907),.UNSPECIFIED.,.F.,.F.,(4,2,4),(1.00000018531336E-6,0.161245467045064,
0.321302696266755),.UNSPECIFIED.);
#1092=B_SPLINE_CURVE_WITH_KNOTS('',3,(#21908,#21909,#21910,#21911,#21912,
#21913),.UNSPECIFIED.,.F.,.F.,(4,2,4),(1.00000020262015E-6,0.166779480521345,
0.332956960659132),.UNSPECIFIED.);
#1093=B_SPLINE_CURVE_WITH_KNOTS('',3,(#21915,#21916,#21917,#21918,#21919,
#21920),.UNSPECIFIED.,.F.,.F.,(4,2,4),(1.00000018504582E-6,0.161245467060812,
0.321302696456924),.UNSPECIFIED.);
#1094=B_SPLINE_CURVE_WITH_KNOTS('',3,(#21921,#21922,#21923,#21924,#21925,
#21926),.UNSPECIFIED.,.F.,.F.,(4,2,4),(1.00000020282842E-6,0.166779480527225,
0.332956960704414),.UNSPECIFIED.);
#1095=B_SPLINE_CURVE_WITH_KNOTS('',3,(#21928,#21929,#21930,#21931,#21932,
#21933),.UNSPECIFIED.,.F.,.F.,(4,2,4),(1.00000018543154E-6,0.161245973871395,
0.321302696554539),.UNSPECIFIED.);
#1096=B_SPLINE_CURVE_WITH_KNOTS('',3,(#21934,#21935,#21936,#21937,#21938,
#21939),.UNSPECIFIED.,.F.,.F.,(4,2,4),(1.00000020267848E-6,0.166779480528834,
0.332956960646251),.UNSPECIFIED.);
#1097=B_SPLINE_CURVE_WITH_KNOTS('',3,(#21941,#21942,#21943,#21944,#21945,
#21946),.UNSPECIFIED.,.F.,.F.,(4,2,4),(1.00000018528204E-6,0.161245973862908,
0.321302696370201),.UNSPECIFIED.);
#1098=B_SPLINE_CURVE_WITH_KNOTS('',3,(#21947,#21948,#21949,#21950,#21951,
#21952),.UNSPECIFIED.,.F.,.F.,(4,2,4),(1.00000020243982E-6,0.166779480529185,
0.332956960704068),.UNSPECIFIED.);
#1099=B_SPLINE_CURVE_WITH_KNOTS('',3,(#21954,#21955,#21956,#21957,#21958,
#21959),.UNSPECIFIED.,.F.,.F.,(4,2,4),(1.0000001851793E-6,0.161245467065769,
0.32130269653859),.UNSPECIFIED.);
#1100=B_SPLINE_CURVE_WITH_KNOTS('',3,(#21960,#21961,#21962,#21963,#21964,
#21965),.UNSPECIFIED.,.F.,.F.,(4,2,4),(1.00000020281741E-6,0.166779480531347,
0.33295696066664),.UNSPECIFIED.);
#1101=B_SPLINE_CURVE_WITH_KNOTS('',3,(#21967,#21968,#21969,#21970,#21971,
#21972),.UNSPECIFIED.,.F.,.F.,(4,2,4),(1.00000018530067E-6,0.161245973867389,
0.321302696417749),.UNSPECIFIED.);
#1102=B_SPLINE_CURVE_WITH_KNOTS('',3,(#21973,#21974,#21975,#21976,#21977,
#21978),.UNSPECIFIED.,.F.,.F.,(4,2,4),(1.00000020264041E-6,0.166779480527634,
0.332956960670351),.UNSPECIFIED.);
#1103=B_SPLINE_CURVE_WITH_KNOTS('',3,(#21980,#21981,#21982,#21983,#21984,
#21985),.UNSPECIFIED.,.F.,.F.,(4,2,4),(1.00000018506015E-6,0.161245973866292,
0.321302696447615),.UNSPECIFIED.);
#1104=B_SPLINE_CURVE_WITH_KNOTS('',3,(#21986,#21987,#21988,#21989,#21990,
#21991),.UNSPECIFIED.,.F.,.F.,(4,2,4),(1.00000020278924E-6,0.166779480531265,
0.332956960653417),.UNSPECIFIED.);
#1105=B_SPLINE_CURVE_WITH_KNOTS('',3,(#21993,#21994,#21995,#21996,#21997,
#21998),.UNSPECIFIED.,.F.,.F.,(4,2,4),(1.00000018471263E-6,0.161245973865716,
0.321302696384943),.UNSPECIFIED.);
#1106=B_SPLINE_CURVE_WITH_KNOTS('',3,(#21999,#22000,#22001,#22002,#22003,
#22004),.UNSPECIFIED.,.F.,.F.,(4,2,4),(1.00000020287686E-6,0.166779480530013,
0.33295696070179),.UNSPECIFIED.);
#1107=B_SPLINE_CURVE_WITH_KNOTS('',3,(#22006,#22007,#22008,#22009,#22010,
#22011),.UNSPECIFIED.,.F.,.F.,(4,2,4),(1.00000018567777E-6,0.161245467067852,
0.321302696531001),.UNSPECIFIED.);
#1108=B_SPLINE_CURVE_WITH_KNOTS('',3,(#22012,#22013,#22014,#22015,#22016,
#22017),.UNSPECIFIED.,.F.,.F.,(4,2,4),(1.00000020307531E-6,0.166779480520602,
0.332956960698483),.UNSPECIFIED.);
#1109=B_SPLINE_CURVE_WITH_KNOTS('',3,(#22019,#22020,#22021,#22022,#22023,
#22024),.UNSPECIFIED.,.F.,.F.,(4,2,4),(1.00000018514608E-6,0.161245467067323,
0.321302696582733),.UNSPECIFIED.);
#1110=B_SPLINE_CURVE_WITH_KNOTS('',3,(#22025,#22026,#22027,#22028,#22029,
#22030),.UNSPECIFIED.,.F.,.F.,(4,2,4),(1.00000020271264E-6,0.166779480532087,
0.33295696071809),.UNSPECIFIED.);
#1111=B_SPLINE_CURVE_WITH_KNOTS('',3,(#22032,#22033,#22034,#22035,#22036,
#22037),.UNSPECIFIED.,.F.,.F.,(4,2,4),(1.00000018490616E-6,0.161245467070947,
0.32130269657138),.UNSPECIFIED.);
#1112=B_SPLINE_CURVE_WITH_KNOTS('',3,(#22038,#22039,#22040,#22041,#22042,
#22043),.UNSPECIFIED.,.F.,.F.,(4,2,4),(1.00000020260949E-6,0.166779480540914,
0.332956960617602),.UNSPECIFIED.);
#1113=B_SPLINE_CURVE_WITH_KNOTS('',3,(#22045,#22046,#22047,#22048,#22049,
#22050),.UNSPECIFIED.,.F.,.F.,(4,2,4),(1.00000018495762E-6,0.161245973857737,
0.321302696209486),.UNSPECIFIED.);
#1114=B_SPLINE_CURVE_WITH_KNOTS('',3,(#22051,#22052,#22053,#22054,#22055,
#22056),.UNSPECIFIED.,.F.,.F.,(4,2,4),(1.00000020240665E-6,0.166779480518083,
0.33295696063765),.UNSPECIFIED.);
#1115=B_SPLINE_CURVE_WITH_KNOTS('',3,(#22058,#22059,#22060,#22061,#22062,
#22063),.UNSPECIFIED.,.F.,.F.,(4,2,4),(1.00000018539525E-6,0.161245467056979,
0.3213026964032),.UNSPECIFIED.);
#1116=B_SPLINE_CURVE_WITH_KNOTS('',3,(#22064,#22065,#22066,#22067,#22068,
#22069),.UNSPECIFIED.,.F.,.F.,(4,2,4),(1.00000020243603E-6,0.166779480530758,
0.332956960667656),.UNSPECIFIED.);
#1117=B_SPLINE_CURVE_WITH_KNOTS('',3,(#22071,#22072,#22073,#22074,#22075,
#22076),.UNSPECIFIED.,.F.,.F.,(4,2,4),(1.00000018564707E-6,0.161245973864463,
0.321302696409748),.UNSPECIFIED.);
#1118=B_SPLINE_CURVE_WITH_KNOTS('',3,(#22077,#22078,#22079,#22080,#22081,
#22082),.UNSPECIFIED.,.F.,.F.,(4,2,4),(1.00000020289556E-6,0.166779480530644,
0.332956960665992),.UNSPECIFIED.);
#1119=B_SPLINE_CURVE_WITH_KNOTS('',3,(#22084,#22085,#22086,#22087,#22088,
#22089),.UNSPECIFIED.,.F.,.F.,(4,2,4),(1.00000018538887E-6,0.161245467065029,
0.321302696435402),.UNSPECIFIED.);
#1120=B_SPLINE_CURVE_WITH_KNOTS('',3,(#22090,#22091,#22092,#22093,#22094,
#22095),.UNSPECIFIED.,.F.,.F.,(4,2,4),(1.00000020280345E-6,0.166779480528368,
0.332956960671687),.UNSPECIFIED.);
#1121=B_SPLINE_CURVE_WITH_KNOTS('',3,(#22097,#22098,#22099,#22100,#22101,
#22102),.UNSPECIFIED.,.F.,.F.,(4,2,4),(1.00000018531322E-6,0.16124597386755,
0.32130269645182),.UNSPECIFIED.);
#1122=B_SPLINE_CURVE_WITH_KNOTS('',3,(#22103,#22104,#22105,#22106,#22107,
#22108),.UNSPECIFIED.,.F.,.F.,(4,2,4),(1.00000020245141E-6,0.166779480529231,
0.332956960669946),.UNSPECIFIED.);
#1123=B_SPLINE_CURVE_WITH_KNOTS('',3,(#22110,#22111,#22112,#22113,#22114,
#22115),.UNSPECIFIED.,.F.,.F.,(4,2,4),(1.00000018554594E-6,0.16124546706305,
0.321302696441769),.UNSPECIFIED.);
#1124=B_SPLINE_CURVE_WITH_KNOTS('',3,(#22116,#22117,#22118,#22119,#22120,
#22121),.UNSPECIFIED.,.F.,.F.,(4,2,4),(1.00000020288612E-6,0.166779480527922,
0.332956960667366),.UNSPECIFIED.);
#1125=B_SPLINE_CURVE_WITH_KNOTS('',3,(#22123,#22124,#22125,#22126,#22127,
#22128),.UNSPECIFIED.,.F.,.F.,(4,2,4),(1.00000018525775E-6,0.161245973865254,
0.32130269643526),.UNSPECIFIED.);
#1126=B_SPLINE_CURVE_WITH_KNOTS('',3,(#22129,#22130,#22131,#22132,#22133,
#22134),.UNSPECIFIED.,.F.,.F.,(4,2,4),(1.00000020267844E-6,0.166779480525132,
0.332956960648716),.UNSPECIFIED.);
#1127=B_SPLINE_CURVE_WITH_KNOTS('',3,(#22136,#22137,#22138,#22139,#22140,
#22141),.UNSPECIFIED.,.F.,.F.,(4,2,4),(1.00000018542923E-6,0.161245467060377,
0.321302696403438),.UNSPECIFIED.);
#1128=B_SPLINE_CURVE_WITH_KNOTS('',3,(#22142,#22143,#22144,#22145,#22146,
#22147),.UNSPECIFIED.,.F.,.F.,(4,2,4),(1.00000020266136E-6,0.166779480530653,
0.332956960655275),.UNSPECIFIED.);
#1129=B_SPLINE_CURVE_WITH_KNOTS('',3,(#22149,#22150,#22151,#22152,#22153,
#22154),.UNSPECIFIED.,.F.,.F.,(4,2,4),(1.00000018510516E-6,0.161245973869074,
0.321302696406845),.UNSPECIFIED.);
#1130=B_SPLINE_CURVE_WITH_KNOTS('',3,(#22155,#22156,#22157,#22158,#22159,
#22160),.UNSPECIFIED.,.F.,.F.,(4,2,4),(1.00000020266632E-6,0.166779480533638,
0.332956960627681),.UNSPECIFIED.);
#1131=B_SPLINE_CURVE_WITH_KNOTS('',3,(#22162,#22163,#22164,#22165,#22166,
#22167),.UNSPECIFIED.,.F.,.F.,(4,2,4),(1.00000018510568E-6,0.161245973864822,
0.321302696292674),.UNSPECIFIED.);
#1132=B_SPLINE_CURVE_WITH_KNOTS('',3,(#22168,#22169,#22170,#22171,#22172,
#22173),.UNSPECIFIED.,.F.,.F.,(4,2,4),(1.00000020272525E-6,0.166779480521084,
0.332956960672202),.UNSPECIFIED.);
#1133=B_SPLINE_CURVE_WITH_KNOTS('',3,(#22175,#22176,#22177,#22178,#22179,
#22180),.UNSPECIFIED.,.F.,.F.,(4,2,4),(1.00000018522469E-6,0.161245467066401,
0.321302696507321),.UNSPECIFIED.);
#1134=B_SPLINE_CURVE_WITH_KNOTS('',3,(#22181,#22182,#22183,#22184,#22185,
#22186),.UNSPECIFIED.,.F.,.F.,(4,2,4),(1.0000002026673E-6,0.166779480534649,
0.332956960655979),.UNSPECIFIED.);
#1135=B_SPLINE_CURVE_WITH_KNOTS('',3,(#22188,#22189,#22190,#22191,#22192,
#22193),.UNSPECIFIED.,.F.,.F.,(4,2,4),(1.00000018545856E-6,0.16124546705897,
0.321302696360171),.UNSPECIFIED.);
#1136=B_SPLINE_CURVE_WITH_KNOTS('',3,(#22194,#22195,#22196,#22197,#22198,
#22199),.UNSPECIFIED.,.F.,.F.,(4,2,4),(1.00000020277335E-6,0.166779480534565,
0.332956960695636),.UNSPECIFIED.);
#1137=B_SPLINE_CURVE_WITH_KNOTS('',3,(#22201,#22202,#22203,#22204,#22205,
#22206),.UNSPECIFIED.,.F.,.F.,(4,2,4),(1.00000018536716E-6,0.161245467067694,
0.321302696478807),.UNSPECIFIED.);
#1138=B_SPLINE_CURVE_WITH_KNOTS('',3,(#22207,#22208,#22209,#22210,#22211,
#22212),.UNSPECIFIED.,.F.,.F.,(4,2,4),(1.00000020264012E-6,0.166779480514383,
0.332956960670406),.UNSPECIFIED.);
#1139=B_SPLINE_CURVE_WITH_KNOTS('',3,(#22214,#22215,#22216,#22217,#22218,
#22219),.UNSPECIFIED.,.F.,.F.,(4,2,4),(1.00000018542659E-6,0.161245973863339,
0.321302696520851),.UNSPECIFIED.);
#1140=B_SPLINE_CURVE_WITH_KNOTS('',3,(#22220,#22221,#22222,#22223,#22224,
#22225),.UNSPECIFIED.,.F.,.F.,(4,2,4),(1.000000202736E-6,0.166779480527173,
0.332956960649766),.UNSPECIFIED.);
#1141=B_SPLINE_CURVE_WITH_KNOTS('',3,(#22227,#22228,#22229,#22230,#22231,
#22232),.UNSPECIFIED.,.F.,.F.,(4,2,4),(1.00000018528858E-6,0.161245467063617,
0.321302696399603),.UNSPECIFIED.);
#1142=B_SPLINE_CURVE_WITH_KNOTS('',3,(#22233,#22234,#22235,#22236,#22237,
#22238),.UNSPECIFIED.,.F.,.F.,(4,2,4),(1.00000020289104E-6,0.16677948052314,
0.332956960694236),.UNSPECIFIED.);
#1143=B_SPLINE_CURVE_WITH_KNOTS('',3,(#22240,#22241,#22242,#22243,#22244,
#22245),.UNSPECIFIED.,.F.,.F.,(4,2,4),(1.00000018486152E-6,0.161245467066123,
0.321302696553676),.UNSPECIFIED.);
#1144=B_SPLINE_CURVE_WITH_KNOTS('',3,(#22246,#22247,#22248,#22249,#22250,
#22251),.UNSPECIFIED.,.F.,.F.,(4,2,4),(1.00000020272568E-6,0.166779480527199,
0.332956960661804),.UNSPECIFIED.);
#1145=B_SPLINE_CURVE_WITH_KNOTS('',3,(#22253,#22254,#22255,#22256,#22257,
#22258),.UNSPECIFIED.,.F.,.F.,(4,2,4),(1.00000018559864E-6,0.161245973866835,
0.321302696434928),.UNSPECIFIED.);
#1146=B_SPLINE_CURVE_WITH_KNOTS('',3,(#22259,#22260,#22261,#22262,#22263,
#22264),.UNSPECIFIED.,.F.,.F.,(4,2,4),(1.00000020252041E-6,0.166779480527667,
0.332956960670414),.UNSPECIFIED.);
#1147=B_SPLINE_CURVE_WITH_KNOTS('',3,(#22266,#22267,#22268,#22269,#22270,
#22271),.UNSPECIFIED.,.F.,.F.,(4,2,4),(1.00000022065418E-6,0.167102971345719,
0.334149753299976),.UNSPECIFIED.);
#1148=B_SPLINE_CURVE_WITH_KNOTS('',3,(#22272,#22273,#22274,#22275,#22276,
#22277),.UNSPECIFIED.,.F.,.F.,(4,2,4),(1.00000012092585E-6,0.161160399905657,
0.32316760723809),.UNSPECIFIED.);
#1149=B_SPLINE_CURVE_WITH_KNOTS('',3,(#22279,#22280,#22281,#22282,#22283,
#22284),.UNSPECIFIED.,.F.,.F.,(4,2,4),(1.00000012028406E-6,0.161160399904698,
0.323167607237289),.UNSPECIFIED.);
#1150=B_SPLINE_CURVE_WITH_KNOTS('',3,(#22285,#22286,#22287,#22288,#22289,
#22290),.UNSPECIFIED.,.F.,.F.,(4,2,4),(1.00000022034966E-6,0.1671029713458,
0.334149753300162),.UNSPECIFIED.);
#1151=B_SPLINE_CURVE_WITH_KNOTS('',3,(#22292,#22293,#22294,#22295,#22296,
#22297),.UNSPECIFIED.,.F.,.F.,(4,2,4),(1.00000012065005E-6,0.161160399904619,
0.323167607236669),.UNSPECIFIED.);
#1152=B_SPLINE_CURVE_WITH_KNOTS('',3,(#22298,#22299,#22300,#22301,#22302,
#22303),.UNSPECIFIED.,.F.,.F.,(4,2,4),(1.00000022013381E-6,0.167102971345785,
0.334149753300176),.UNSPECIFIED.);
#1153=B_SPLINE_CURVE_WITH_KNOTS('',3,(#22305,#22306,#22307,#22308,#22309,
#22310),.UNSPECIFIED.,.F.,.F.,(4,2,4),(1.00000012096186E-6,0.161160399904608,
0.323167607236878),.UNSPECIFIED.);
#1154=B_SPLINE_CURVE_WITH_KNOTS('',3,(#22311,#22312,#22313,#22314,#22315,
#22316),.UNSPECIFIED.,.F.,.F.,(4,2,4),(1.00000022094295E-6,0.167102971345706,
0.334149753300038),.UNSPECIFIED.);
#1155=B_SPLINE_CURVE_WITH_KNOTS('',3,(#22318,#22319,#22320,#22321,#22322,
#22323),.UNSPECIFIED.,.F.,.F.,(4,2,4),(1.00000012019619E-6,0.161160399904656,
0.323167607236991),.UNSPECIFIED.);
#1156=B_SPLINE_CURVE_WITH_KNOTS('',3,(#22324,#22325,#22326,#22327,#22328,
#22329),.UNSPECIFIED.,.F.,.F.,(4,2,4),(1.00000022083162E-6,0.167102971345771,
0.334149753300189),.UNSPECIFIED.);
#1157=B_SPLINE_CURVE_WITH_KNOTS('',3,(#22331,#22332,#22333,#22334,#22335,
#22336),.UNSPECIFIED.,.F.,.F.,(4,2,4),(1.00000012046609E-6,0.16115988960677,
0.323167607237021),.UNSPECIFIED.);
#1158=B_SPLINE_CURVE_WITH_KNOTS('',3,(#22337,#22338,#22339,#22340,#22341,
#22342),.UNSPECIFIED.,.F.,.F.,(4,2,4),(1.00000022058697E-6,0.1671029713457,
0.334149753299905),.UNSPECIFIED.);
#1159=B_SPLINE_CURVE_WITH_KNOTS('',3,(#22344,#22345,#22346,#22347,#22348,
#22349),.UNSPECIFIED.,.F.,.F.,(4,2,4),(1.00000012068149E-6,0.161159889606763,
0.323167607237227),.UNSPECIFIED.);
#1160=B_SPLINE_CURVE_WITH_KNOTS('',3,(#22350,#22351,#22352,#22353,#22354,
#22355),.UNSPECIFIED.,.F.,.F.,(4,2,4),(1.00000022093697E-6,0.167102971345751,
0.334149753300017),.UNSPECIFIED.);
#1161=B_SPLINE_CURVE_WITH_KNOTS('',3,(#22357,#22358,#22359,#22360,#22361,
#22362),.UNSPECIFIED.,.F.,.F.,(4,2,4),(1.00000012055824E-6,0.161160399904627,
0.323167607236808),.UNSPECIFIED.);
#1162=B_SPLINE_CURVE_WITH_KNOTS('',3,(#22363,#22364,#22365,#22366,#22367,
#22368),.UNSPECIFIED.,.F.,.F.,(4,2,4),(1.00000022101565E-6,0.167102971345646,
0.334149753299828),.UNSPECIFIED.);
#1163=B_SPLINE_CURVE_WITH_KNOTS('',3,(#22370,#22371,#22372,#22373,#22374,
#22375),.UNSPECIFIED.,.F.,.F.,(4,2,4),(1.00000012064667E-6,0.16116039990467,
0.323167607237047),.UNSPECIFIED.);
#1164=B_SPLINE_CURVE_WITH_KNOTS('',3,(#22376,#22377,#22378,#22379,#22380,
#22381),.UNSPECIFIED.,.F.,.F.,(4,2,4),(1.00000022025054E-6,0.16710297134573,
0.334149753300021),.UNSPECIFIED.);
#1165=B_SPLINE_CURVE_WITH_KNOTS('',3,(#22383,#22384,#22385,#22386,#22387,
#22388),.UNSPECIFIED.,.F.,.F.,(4,2,4),(1.00000012080846E-6,0.161160399904661,
0.323167607236932),.UNSPECIFIED.);
#1166=B_SPLINE_CURVE_WITH_KNOTS('',3,(#22389,#22390,#22391,#22392,#22393,
#22394),.UNSPECIFIED.,.F.,.F.,(4,2,4),(1.00000022119352E-6,0.167102971345721,
0.334149753299959),.UNSPECIFIED.);
#1167=B_SPLINE_CURVE_WITH_KNOTS('',3,(#22396,#22397,#22398,#22399,#22400,
#22401),.UNSPECIFIED.,.F.,.F.,(4,2,4),(1.00000012038514E-6,0.161160399904662,
0.323167607237004),.UNSPECIFIED.);
#1168=B_SPLINE_CURVE_WITH_KNOTS('',3,(#22402,#22403,#22404,#22405,#22406,
#22407),.UNSPECIFIED.,.F.,.F.,(4,2,4),(1.00000022107472E-6,0.167102971345737,
0.33414975330002),.UNSPECIFIED.);
#1169=B_SPLINE_CURVE_WITH_KNOTS('',3,(#22409,#22410,#22411,#22412,#22413,
#22414),.UNSPECIFIED.,.F.,.F.,(4,2,4),(1.00000012039255E-6,0.161160399904654,
0.323167607237),.UNSPECIFIED.);
#1170=B_SPLINE_CURVE_WITH_KNOTS('',3,(#22415,#22416,#22417,#22418,#22419,
#22420),.UNSPECIFIED.,.F.,.F.,(4,2,4),(1.00000022054453E-6,0.167102971345693,
0.334149753299904),.UNSPECIFIED.);
#1171=B_SPLINE_CURVE_WITH_KNOTS('',3,(#22422,#22423,#22424,#22425,#22426,
#22427),.UNSPECIFIED.,.F.,.F.,(4,2,4),(1.00000012058307E-6,0.161159889606735,
0.323167607236912),.UNSPECIFIED.);
#1172=B_SPLINE_CURVE_WITH_KNOTS('',3,(#22428,#22429,#22430,#22431,#22432,
#22433),.UNSPECIFIED.,.F.,.F.,(4,2,4),(1.00000022069235E-6,0.167102971345655,
0.334149753299868),.UNSPECIFIED.);
#1173=B_SPLINE_CURVE_WITH_KNOTS('',3,(#22435,#22436,#22437,#22438,#22439,
#22440),.UNSPECIFIED.,.F.,.F.,(4,2,4),(1.00000012093059E-6,0.161160399904649,
0.323167607236986),.UNSPECIFIED.);
#1174=B_SPLINE_CURVE_WITH_KNOTS('',3,(#22441,#22442,#22443,#22444,#22445,
#22446),.UNSPECIFIED.,.F.,.F.,(4,2,4),(1.00000022078288E-6,0.167102971345831,
0.334149753300156),.UNSPECIFIED.);
#1175=B_SPLINE_CURVE_WITH_KNOTS('',3,(#22448,#22449,#22450,#22451,#22452,
#22453),.UNSPECIFIED.,.F.,.F.,(4,2,4),(1.00000012057364E-6,0.161160399904675,
0.323167607237077),.UNSPECIFIED.);
#1176=B_SPLINE_CURVE_WITH_KNOTS('',3,(#22454,#22455,#22456,#22457,#22458,
#22459),.UNSPECIFIED.,.F.,.F.,(4,2,4),(1.000000220711E-6,0.167102971345943,
0.334149753300391),.UNSPECIFIED.);
#1177=B_SPLINE_CURVE_WITH_KNOTS('',3,(#22461,#22462,#22463,#22464,#22465,
#22466),.UNSPECIFIED.,.F.,.F.,(4,2,4),(1.00000012058037E-6,0.161160399904651,
0.323167607236874),.UNSPECIFIED.);
#1178=B_SPLINE_CURVE_WITH_KNOTS('',3,(#22467,#22468,#22469,#22470,#22471,
#22472),.UNSPECIFIED.,.F.,.F.,(4,2,4),(1.00000022031051E-6,0.167102971345854,
0.334149753300263),.UNSPECIFIED.);
#1179=B_SPLINE_CURVE_WITH_KNOTS('',3,(#22474,#22475,#22476,#22477,#22478,
#22479),.UNSPECIFIED.,.F.,.F.,(4,2,4),(1.00000012055685E-6,0.161160399904695,
0.323167607237214),.UNSPECIFIED.);
#1180=B_SPLINE_CURVE_WITH_KNOTS('',3,(#22480,#22481,#22482,#22483,#22484,
#22485),.UNSPECIFIED.,.F.,.F.,(4,2,4),(1.00000022029865E-6,0.167102971345825,
0.334149753300157),.UNSPECIFIED.);
#1181=B_SPLINE_CURVE_WITH_KNOTS('',3,(#22487,#22488,#22489,#22490,#22491,
#22492),.UNSPECIFIED.,.F.,.F.,(4,2,4),(1.00000012053579E-6,0.161160399904707,
0.323167607237315),.UNSPECIFIED.);
#1182=B_SPLINE_CURVE_WITH_KNOTS('',3,(#22493,#22494,#22495,#22496,#22497,
#22498),.UNSPECIFIED.,.F.,.F.,(4,2,4),(1.00000022063479E-6,0.167102971345967,
0.334149753300421),.UNSPECIFIED.);
#1183=B_SPLINE_CURVE_WITH_KNOTS('',3,(#22500,#22501,#22502,#22503,#22504,
#22505),.UNSPECIFIED.,.F.,.F.,(4,2,4),(1.00000012093733E-6,0.161160399904629,
0.323167607236834),.UNSPECIFIED.);
#1184=B_SPLINE_CURVE_WITH_KNOTS('',3,(#22506,#22507,#22508,#22509,#22510,
#22511),.UNSPECIFIED.,.F.,.F.,(4,2,4),(1.0000002205328E-6,0.16710297134574,
0.334149753300078),.UNSPECIFIED.);
#1185=B_SPLINE_CURVE_WITH_KNOTS('',3,(#22513,#22514,#22515,#22516,#22517,
#22518),.UNSPECIFIED.,.F.,.F.,(4,2,4),(1.00000012048169E-6,0.161159889606741,
0.323167607237064),.UNSPECIFIED.);
#1186=B_SPLINE_CURVE_WITH_KNOTS('',3,(#22519,#22520,#22521,#22522,#22523,
#22524),.UNSPECIFIED.,.F.,.F.,(4,2,4),(1.00000022062917E-6,0.167102971345646,
0.334149753299816),.UNSPECIFIED.);
#1187=B_SPLINE_CURVE_WITH_KNOTS('',3,(#22526,#22527,#22528,#22529,#22530,
#22531),.UNSPECIFIED.,.F.,.F.,(4,2,4),(1.00000012032585E-6,0.16116039990466,
0.323167607237033),.UNSPECIFIED.);
#1188=B_SPLINE_CURVE_WITH_KNOTS('',3,(#22532,#22533,#22534,#22535,#22536,
#22537),.UNSPECIFIED.,.F.,.F.,(4,2,4),(1.00000022065021E-6,0.167102971345787,
0.334149753300079),.UNSPECIFIED.);
#1189=B_SPLINE_CURVE_WITH_KNOTS('',3,(#22539,#22540,#22541,#22542,#22543,
#22544),.UNSPECIFIED.,.F.,.F.,(4,2,4),(1.00000012068184E-6,0.16115988960672,
0.323167607236954),.UNSPECIFIED.);
#1190=B_SPLINE_CURVE_WITH_KNOTS('',3,(#22545,#22546,#22547,#22548,#22549,
#22550),.UNSPECIFIED.,.F.,.F.,(4,2,4),(1.0000002207771E-6,0.167102971345759,
0.334149753300061),.UNSPECIFIED.);
#1191=B_SPLINE_CURVE_WITH_KNOTS('',3,(#22552,#22553,#22554,#22555,#22556,
#22557),.UNSPECIFIED.,.F.,.F.,(4,2,4),(1.00000012044603E-6,0.161160399904649,
0.323167607237023),.UNSPECIFIED.);
#1192=B_SPLINE_CURVE_WITH_KNOTS('',3,(#22558,#22559,#22560,#22561,#22562,
#22563),.UNSPECIFIED.,.F.,.F.,(4,2,4),(1.00000022079248E-6,0.1671029713458,
0.33414975330013),.UNSPECIFIED.);
#1193=B_SPLINE_CURVE_WITH_KNOTS('',3,(#22565,#22566,#22567,#22568,#22569,
#22570),.UNSPECIFIED.,.F.,.F.,(4,2,4),(1.00000012037424E-6,0.161160399904647,
0.323167607237001),.UNSPECIFIED.);
#1194=B_SPLINE_CURVE_WITH_KNOTS('',3,(#22571,#22572,#22573,#22574,#22575,
#22576),.UNSPECIFIED.,.F.,.F.,(4,2,4),(1.00000022090657E-6,0.167102971345759,
0.334149753300051),.UNSPECIFIED.);
#1195=B_SPLINE_CURVE_WITH_KNOTS('',3,(#22578,#22579,#22580,#22581,#22582,
#22583),.UNSPECIFIED.,.F.,.F.,(4,2,4),(1.00000012028251E-6,0.161160399904642,
0.323167607236946),.UNSPECIFIED.);
#1196=B_SPLINE_CURVE_WITH_KNOTS('',3,(#22584,#22585,#22586,#22587,#22588,
#22589),.UNSPECIFIED.,.F.,.F.,(4,2,4),(1.00000022075346E-6,0.167102971345758,
0.334149753300091),.UNSPECIFIED.);
#1197=B_SPLINE_CURVE_WITH_KNOTS('',3,(#22591,#22592,#22593,#22594,#22595,
#22596),.UNSPECIFIED.,.F.,.F.,(4,2,4),(1.00000012045161E-6,0.161160399904678,
0.323167607237292),.UNSPECIFIED.);
#1198=B_SPLINE_CURVE_WITH_KNOTS('',3,(#22597,#22598,#22599,#22600,#22601,
#22602),.UNSPECIFIED.,.F.,.F.,(4,2,4),(1.00000022071781E-6,0.167102971346066,
0.334149753300729),.UNSPECIFIED.);
#1199=B_SPLINE_CURVE_WITH_KNOTS('',3,(#22604,#22605,#22606,#22607,#22608,
#22609),.UNSPECIFIED.,.F.,.F.,(4,2,4),(1.00000012085704E-6,0.161160399904647,
0.323167607236899),.UNSPECIFIED.);
#1200=B_SPLINE_CURVE_WITH_KNOTS('',3,(#22610,#22611,#22612,#22613,#22614,
#22615),.UNSPECIFIED.,.F.,.F.,(4,2,4),(1.00000022074304E-6,0.167102971345757,
0.334149753300087),.UNSPECIFIED.);
#1201=B_SPLINE_CURVE_WITH_KNOTS('',3,(#22617,#22618,#22619,#22620,#22621,
#22622),.UNSPECIFIED.,.F.,.F.,(4,2,4),(1.00000012006173E-6,0.161160399904691,
0.323167607237029),.UNSPECIFIED.);
#1202=B_SPLINE_CURVE_WITH_KNOTS('',3,(#22623,#22624,#22625,#22626,#22627,
#22628),.UNSPECIFIED.,.F.,.F.,(4,2,4),(1.00000022083549E-6,0.167102971345888,
0.334149753300255),.UNSPECIFIED.);
#1203=B_SPLINE_CURVE_WITH_KNOTS('',3,(#22630,#22631,#22632,#22633,#22634,
#22635),.UNSPECIFIED.,.F.,.F.,(4,2,4),(1.00000012064762E-6,0.161160399904703,
0.323167607237272),.UNSPECIFIED.);
#1204=B_SPLINE_CURVE_WITH_KNOTS('',3,(#22636,#22637,#22638,#22639,#22640,
#22641),.UNSPECIFIED.,.F.,.F.,(4,2,4),(1.00000022088092E-6,0.167102971345646,
0.33414975329985),.UNSPECIFIED.);
#1205=B_SPLINE_CURVE_WITH_KNOTS('',3,(#22643,#22644,#22645,#22646,#22647,
#22648),.UNSPECIFIED.,.F.,.F.,(4,2,4),(1.00000012096778E-6,0.161160399904595,
0.323167607236728),.UNSPECIFIED.);
#1206=B_SPLINE_CURVE_WITH_KNOTS('',3,(#22649,#22650,#22651,#22652,#22653,
#22654),.UNSPECIFIED.,.F.,.F.,(4,2,4),(1.00000022064523E-6,0.167102971345871,
0.334149753300307),.UNSPECIFIED.);
#1207=B_SPLINE_CURVE_WITH_KNOTS('',3,(#22656,#22657,#22658,#22659,#22660,
#22661),.UNSPECIFIED.,.F.,.F.,(4,2,4),(1.00000012057745E-6,0.161160399904619,
0.32316760723675),.UNSPECIFIED.);
#1208=B_SPLINE_CURVE_WITH_KNOTS('',3,(#22662,#22663,#22664,#22665,#22666,
#22667),.UNSPECIFIED.,.F.,.F.,(4,2,4),(1.00000022078269E-6,0.167102971345806,
0.334149753300164),.UNSPECIFIED.);
#1209=B_SPLINE_CURVE_WITH_KNOTS('',3,(#22669,#22670,#22671,#22672,#22673,
#22674),.UNSPECIFIED.,.F.,.F.,(4,2,4),(1.00000012048116E-6,0.16116039990468,
0.323167607237172),.UNSPECIFIED.);
#1210=B_SPLINE_CURVE_WITH_KNOTS('',3,(#22675,#22676,#22677,#22678,#22679,
#22680),.UNSPECIFIED.,.F.,.F.,(4,2,4),(1.00000022054791E-6,0.167102971345839,
0.334149753300197),.UNSPECIFIED.);
#1211=B_SPLINE_CURVE_WITH_KNOTS('',3,(#22682,#22683,#22684,#22685,#22686,
#22687),.UNSPECIFIED.,.F.,.F.,(4,2,4),(1.00000012048408E-6,0.161159889606746,
0.323167607237105),.UNSPECIFIED.);
#1212=B_SPLINE_CURVE_WITH_KNOTS('',3,(#22688,#22689,#22690,#22691,#22692,
#22693),.UNSPECIFIED.,.F.,.F.,(4,2,4),(1.00000022061624E-6,0.16710297134579,
0.3341497533002),.UNSPECIFIED.);
#1213=B_SPLINE_CURVE_WITH_KNOTS('',3,(#22695,#22696,#22697,#22698,#22699,
#22700),.UNSPECIFIED.,.F.,.F.,(4,2,4),(1.00000012060288E-6,0.161159889606819,
0.32316760723714),.UNSPECIFIED.);
#1214=B_SPLINE_CURVE_WITH_KNOTS('',3,(#22701,#22702,#22703,#22704,#22705,
#22706),.UNSPECIFIED.,.F.,.F.,(4,2,4),(1.00000022039092E-6,0.16710297134578,
0.334149753300241),.UNSPECIFIED.);
#1215=B_SPLINE_CURVE_WITH_KNOTS('',3,(#22708,#22709,#22710,#22711,#22712,
#22713),.UNSPECIFIED.,.F.,.F.,(4,2,4),(1.00000012039262E-6,0.161159889606932,
0.323167607237268),.UNSPECIFIED.);
#1216=B_SPLINE_CURVE_WITH_KNOTS('',3,(#22714,#22715,#22716,#22717,#22718,
#22719),.UNSPECIFIED.,.F.,.F.,(4,2,4),(1.00000022068054E-6,0.167102971345753,
0.334149753300243),.UNSPECIFIED.);
#1217=B_SPLINE_CURVE_WITH_KNOTS('',3,(#22721,#22722,#22723,#22724,#22725,
#22726),.UNSPECIFIED.,.F.,.F.,(4,2,4),(1.00000012008432E-6,0.161160399904884,
0.323167607237139),.UNSPECIFIED.);
#1218=B_SPLINE_CURVE_WITH_KNOTS('',3,(#22727,#22728,#22729,#22730,#22731,
#22732),.UNSPECIFIED.,.F.,.F.,(4,2,4),(1.00000022061894E-6,0.167102971345809,
0.334149753300514),.UNSPECIFIED.);
#1219=B_SPLINE_CURVE_WITH_KNOTS('',3,(#22734,#22735,#22736,#22737,#22738,
#22739),.UNSPECIFIED.,.F.,.F.,(4,2,4),(1.00000012081545E-6,0.161160399905061,
0.323167607237863),.UNSPECIFIED.);
#1220=B_SPLINE_CURVE_WITH_KNOTS('',3,(#22740,#22741,#22742,#22743,#22744,
#22745),.UNSPECIFIED.,.F.,.F.,(4,2,4),(1.00000022055009E-6,0.16710297134578,
0.334149753300514),.UNSPECIFIED.);
#1221=B_SPLINE_CURVE_WITH_KNOTS('',3,(#22747,#22748,#22749,#22750,#22751,
#22752),.UNSPECIFIED.,.F.,.F.,(4,2,4),(1.00000012031008E-6,0.161160399905076,
0.323167607237676),.UNSPECIFIED.);
#1222=B_SPLINE_CURVE_WITH_KNOTS('',3,(#22753,#22754,#22755,#22756,#22757,
#22758),.UNSPECIFIED.,.F.,.F.,(4,2,4),(1.00000022063654E-6,0.167102971345982,
0.334149753301056),.UNSPECIFIED.);
#1223=B_SPLINE_CURVE_WITH_KNOTS('',3,(#22760,#22761,#22762,#22763,#22764,
#22765),.UNSPECIFIED.,.F.,.F.,(4,2,4),(1.00000012057795E-6,0.161159889607266,
0.323167607237755),.UNSPECIFIED.);
#1224=B_SPLINE_CURVE_WITH_KNOTS('',3,(#22766,#22767,#22768,#22769,#22770,
#22771),.UNSPECIFIED.,.F.,.F.,(4,2,4),(1.00000022038566E-6,0.167102971345924,
0.334149753300952),.UNSPECIFIED.);
#1225=B_SPLINE_CURVE_WITH_KNOTS('',3,(#22773,#22774,#22775,#22776,#22777,
#22778),.UNSPECIFIED.,.F.,.F.,(4,2,4),(1.00000012035839E-6,0.161160399905228,
0.323167607237738),.UNSPECIFIED.);
#1226=B_SPLINE_CURVE_WITH_KNOTS('',3,(#22779,#22780,#22781,#22782,#22783,
#22784),.UNSPECIFIED.,.F.,.F.,(4,2,4),(1.00000022108953E-6,0.167102971345621,
0.334149753300335),.UNSPECIFIED.);
#1227=B_SPLINE_CURVE_WITH_KNOTS('',3,(#22786,#22787,#22788,#22789,#22790,
#22791),.UNSPECIFIED.,.F.,.F.,(4,2,4),(1.00000011994104E-6,0.161159889607422,
0.323167607237808),.UNSPECIFIED.);
#1228=B_SPLINE_CURVE_WITH_KNOTS('',3,(#22792,#22793,#22794,#22795,#22796,
#22797),.UNSPECIFIED.,.F.,.F.,(4,2,4),(1.00000022079877E-6,0.167102971345911,
0.334149753301048),.UNSPECIFIED.);
#1229=B_SPLINE_CURVE_WITH_KNOTS('',3,(#22799,#22800,#22801,#22802,#22803,
#22804),.UNSPECIFIED.,.F.,.F.,(4,2,4),(1.00000012034089E-6,0.161160399905409,
0.323167607237919),.UNSPECIFIED.);
#1230=B_SPLINE_CURVE_WITH_KNOTS('',3,(#22805,#22806,#22807,#22808,#22809,
#22810),.UNSPECIFIED.,.F.,.F.,(4,2,4),(1.0000002204628E-6,0.167102971345718,
0.334149753300732),.UNSPECIFIED.);
#1231=B_SPLINE_CURVE_WITH_KNOTS('',3,(#22812,#22813,#22814,#22815,#22816,
#22817),.UNSPECIFIED.,.F.,.F.,(4,2,4),(1.00000011993139E-6,0.161159889607588,
0.323167607237936),.UNSPECIFIED.);
#1232=B_SPLINE_CURVE_WITH_KNOTS('',3,(#22818,#22819,#22820,#22821,#22822,
#22823),.UNSPECIFIED.,.F.,.F.,(4,2,4),(1.00000022104047E-6,0.167102971345937,
0.334149753301223),.UNSPECIFIED.);
#1233=B_SPLINE_CURVE_WITH_KNOTS('',3,(#22825,#22826,#22827,#22828,#22829,
#22830),.UNSPECIFIED.,.F.,.F.,(4,2,4),(1.00000012050061E-6,0.161160399905562,
0.323167607237955),.UNSPECIFIED.);
#1234=B_SPLINE_CURVE_WITH_KNOTS('',3,(#22831,#22832,#22833,#22834,#22835,
#22836),.UNSPECIFIED.,.F.,.F.,(4,2,4),(1.00000022052091E-6,0.167102971345926,
0.334149753301295),.UNSPECIFIED.);
#1235=B_SPLINE_CURVE_WITH_KNOTS('',3,(#22891,#22892,#22893,#22894,#22895,
#22896,#22897,#22898,#22899,#22900,#22901,#22902,#22903,#22904,#22905,#22906,
#22907,#22908,#22909,#22910,#22911,#22912,#22913,#22914,#22915,#22916,#22917,
#22918,#22919,#22920,#22921,#22922,#22923,#22924,#22925,#22926,#22927,#22928,
#22929,#22930,#22931,#22932,#22933,#22934,#22935,#22936,#22937,#22938,#22939,
#22940,#22941,#22942),.UNSPECIFIED.,.F.,.F.,(4,3,3,3,3,3,3,3,3,3,3,3,3,
3,3,3,3,4),(0.,0.0290398589546445,0.0579843816831971,0.0868853129795454,
0.115761457357984,0.144631560789434,0.173538323016997,0.202474581669382,
0.2314954385994,0.249999999943001,0.279015696481342,0.30796588845617,0.336869516660747,
0.365745410793947,0.394622693781268,0.423510570114902,0.452445568558316,
0.460808762537663),.UNSPECIFIED.);
#1236=B_SPLINE_CURVE_WITH_KNOTS('',3,(#23074,#23075,#23076,#23077,#23078,
#23079,#23080,#23081),.UNSPECIFIED.,.F.,.F.,(4,2,2,4),(0.0783698293107414,
0.308777371982556,0.539184914655036,0.562623084473123),.UNSPECIFIED.);
#1237=B_SPLINE_CURVE_WITH_KNOTS('',3,(#23224,#23225,#23226,#23227,#23228,
#23229,#23230,#23231,#23232,#23233,#23234,#23235,#23236,#23237,#23238,#23239,
#23240,#23241,#23242,#23243,#23244,#23245,#23246,#23247,#23248,#23249,#23250,
#23251,#23252,#23253,#23254,#23255,#23256,#23257,#23258,#23259,#23260,#23261,
#23262,#23263,#23264,#23265,#23266,#23267,#23268,#23269,#23270,#23271,#23272,
#23273,#23274,#23275),.UNSPECIFIED.,.F.,.F.,(4,3,3,3,3,3,3,3,3,3,3,3,3,
3,3,3,3,4),(0.,0.0290398589545971,0.0579843816831279,0.0868853129794532,
0.115761457357872,0.144631560789305,0.173538323016845,0.202474581669205,
0.231495438599207,0.249999999943415,0.279015696481713,0.307965888456488,
0.336869516660988,0.365745410794182,0.394622693781447,0.423510570114973,
0.45244556855835,0.460808762537663),.UNSPECIFIED.);
#1238=B_SPLINE_CURVE_WITH_KNOTS('',3,(#23396,#23397,#23398,#23399,#23400,
#23401,#23402,#23403,#23404,#23405,#23406,#23407,#23408,#23409,#23410,#23411,
#23412,#23413,#23414,#23415,#23416,#23417,#23418,#23419,#23420,#23421,#23422,
#23423,#23424,#23425,#23426,#23427,#23428,#23429,#23430,#23431,#23432,#23433,
#23434,#23435,#23436,#23437,#23438,#23439,#23440,#23441,#23442,#23443,#23444,
#23445,#23446,#23447),.UNSPECIFIED.,.F.,.F.,(4,3,3,3,3,3,3,3,3,3,3,3,3,
3,3,3,3,4),(0.,0.029039858954596,0.0579843816831248,0.0868853129794533,
0.115761457357877,0.144631560789305,0.173538323016854,0.202474581669227,
0.231495438599218,0.249999999943415,0.279015696481708,0.307965888456495,
0.336869516661002,0.365745410794122,0.394622693781374,0.423510570114958,
0.452445568558351,0.460808762537663),.UNSPECIFIED.);
#1239=B_SPLINE_CURVE_WITH_KNOTS('',3,(#23693,#23694,#23695,#23696,#23697,
#23698,#23699,#23700,#23701,#23702,#23703,#23704,#23705,#23706,#23707,#23708,
#23709,#23710,#23711,#23712,#23713,#23714,#23715,#23716,#23717,#23718,#23719,
#23720,#23721,#23722,#23723,#23724,#23725,#23726,#23727,#23728,#23729,#23730,
#23731,#23732,#23733,#23734,#23735,#23736,#23737,#23738,#23739,#23740,#23741,
#23742,#23743,#23744),.UNSPECIFIED.,.F.,.F.,(4,3,3,3,3,3,3,3,3,3,3,3,3,
3,3,3,3,4),(0.,0.0290398589546279,0.0579843816831548,0.086885312979481,
0.115761457357894,0.14463156078933,0.173538323016879,0.202474581669232,
0.231495438599223,0.249999999943415,0.279015696481706,0.307965888456492,
0.336869516661009,0.365745410794138,0.394622693781402,0.423510570114935,
0.452445568558275,0.460808762537663),.UNSPECIFIED.);
#1240=B_SPLINE_CURVE_WITH_KNOTS('',3,(#23865,#23866,#23867,#23868,#23869,
#23870,#23871,#23872,#23873,#23874,#23875,#23876,#23877,#23878,#23879,#23880,
#23881,#23882,#23883,#23884,#23885,#23886,#23887,#23888,#23889,#23890,#23891,
#23892,#23893,#23894,#23895,#23896,#23897,#23898,#23899,#23900,#23901,#23902,
#23903,#23904,#23905,#23906,#23907,#23908,#23909,#23910,#23911,#23912,#23913,
#23914,#23915,#23916),.UNSPECIFIED.,.F.,.F.,(4,3,3,3,3,3,3,3,3,3,3,3,3,
3,3,3,3,4),(0.,0.0290398589546199,0.0579843816831478,0.0868853129794725,
0.11576145735789,0.144631560789328,0.17353832301687,0.202474581669228,0.231495438599226,
0.249999999943415,0.279015696481709,0.307965888456473,0.336869516660979,
0.365745410794135,0.394622693781407,0.423510570114972,0.452445568558348,
0.460808762537948),.UNSPECIFIED.);
#1241=B_SPLINE_CURVE_WITH_KNOTS('',3,(#24037,#24038,#24039,#24040,#24041,
#24042,#24043,#24044,#24045,#24046,#24047,#24048,#24049,#24050,#24051,#24052,
#24053,#24054,#24055,#24056,#24057,#24058,#24059,#24060,#24061,#24062,#24063,
#24064,#24065,#24066,#24067,#24068,#24069,#24070,#24071,#24072,#24073,#24074,
#24075,#24076,#24077,#24078,#24079,#24080,#24081,#24082,#24083,#24084,#24085,
#24086,#24087,#24088),.UNSPECIFIED.,.F.,.F.,(4,3,3,3,3,3,3,3,3,3,3,3,3,
3,3,3,3,4),(0.,0.0290398589546317,0.0579843816831625,0.0868853129794868,
0.115761457357901,0.144631560789317,0.173538323016866,0.202474581669238,
0.231495438599229,0.249999999943415,0.279015696481706,0.307965888456485,
0.336869516660966,0.365745410794117,0.394622693781377,0.423510570114936,
0.452445568558318,0.460808762537663),.UNSPECIFIED.);
#1242=B_SPLINE_CURVE_WITH_KNOTS('',3,(#24209,#24210,#24211,#24212,#24213,
#24214,#24215,#24216,#24217,#24218,#24219,#24220,#24221,#24222,#24223,#24224,
#24225,#24226,#24227,#24228,#24229,#24230,#24231,#24232,#24233,#24234,#24235,
#24236,#24237,#24238,#24239,#24240,#24241,#24242,#24243,#24244,#24245,#24246,
#24247,#24248,#24249,#24250,#24251,#24252,#24253,#24254,#24255,#24256,#24257,
#24258,#24259,#24260),.UNSPECIFIED.,.F.,.F.,(4,3,3,3,3,3,3,3,3,3,3,3,3,
3,3,3,3,4),(0.,0.0290398589545938,0.0579843816831263,0.0868853129794523,
0.115761457357861,0.144631560789281,0.173538323016826,0.202474581669178,
0.231495438599186,0.249999999943415,0.279015696481703,0.307965888456488,
0.336869516660999,0.365745410794192,0.394622693781458,0.423510570115037,
0.452445568558385,0.460808762537663),.UNSPECIFIED.);
#1243=B_SPLINE_CURVE_WITH_KNOTS('',3,(#24381,#24382,#24383,#24384,#24385,
#24386,#24387,#24388,#24389,#24390,#24391,#24392,#24393,#24394,#24395,#24396,
#24397,#24398,#24399,#24400,#24401,#24402,#24403,#24404,#24405,#24406,#24407,
#24408,#24409,#24410,#24411,#24412,#24413,#24414,#24415,#24416,#24417,#24418,
#24419,#24420,#24421,#24422,#24423,#24424,#24425,#24426,#24427,#24428,#24429,
#24430,#24431,#24432),.UNSPECIFIED.,.F.,.F.,(4,3,3,3,3,3,3,3,3,3,3,3,3,
3,3,3,3,4),(0.,0.029039858954607,0.057984381683134,0.0868853129794584,0.115761457357883,
0.144631560789343,0.173538323016891,0.202474581669253,0.23149543859925,
0.249999999943415,0.279015696481708,0.307965888456493,0.336869516661006,
0.365745410794227,0.39462269378149,0.423510570115083,0.452445568558457,
0.460808762537663),.UNSPECIFIED.);
#1244=B_SPLINE_CURVE_WITH_KNOTS('',3,(#24553,#24554,#24555,#24556,#24557,
#24558,#24559,#24560,#24561,#24562,#24563,#24564,#24565,#24566,#24567,#24568,
#24569,#24570,#24571,#24572,#24573,#24574,#24575,#24576,#24577,#24578,#24579,
#24580,#24581,#24582,#24583,#24584,#24585,#24586,#24587,#24588,#24589,#24590,
#24591,#24592,#24593,#24594,#24595,#24596,#24597,#24598,#24599,#24600,#24601,
#24602,#24603,#24604),.UNSPECIFIED.,.F.,.F.,(4,3,3,3,3,3,3,3,3,3,3,3,3,
3,3,3,3,4),(0.,0.029039858954619,0.0579843816831522,0.0868853129794786,
0.115761457357895,0.144631560789334,0.17353832301688,0.202474581669239,
0.23149543859923,0.249999999943415,0.279015696481715,0.307965888456487,
0.336869516660996,0.365745410794131,0.394622693781399,0.423510570114902,
0.452445568558267,0.460808762537948),.UNSPECIFIED.);
#1245=B_SPLINE_CURVE_WITH_KNOTS('',3,(#24725,#24726,#24727,#24728,#24729,
#24730,#24731,#24732,#24733,#24734,#24735,#24736,#24737,#24738,#24739,#24740,
#24741,#24742,#24743,#24744,#24745,#24746,#24747,#24748,#24749,#24750,#24751,
#24752,#24753,#24754,#24755,#24756,#24757,#24758,#24759,#24760,#24761,#24762,
#24763,#24764,#24765,#24766,#24767,#24768,#24769,#24770,#24771,#24772,#24773,
#24774,#24775,#24776),.UNSPECIFIED.,.F.,.F.,(4,3,3,3,3,3,3,3,3,3,3,3,3,
3,3,3,3,4),(0.,0.0290398589546166,0.0579843816831443,0.0868853129794682,
0.115761457357876,0.144631560789308,0.173538323016849,0.202474581669216,
0.231495438599206,0.249999999943415,0.279015696481708,0.307965888456497,
0.336869516660995,0.365745410794177,0.394622693781448,0.423510570114999,
0.452445568558359,0.460808762537663),.UNSPECIFIED.);
#1246=B_SPLINE_CURVE_WITH_KNOTS('',3,(#24897,#24898,#24899,#24900,#24901,
#24902,#24903,#24904,#24905,#24906,#24907,#24908,#24909,#24910,#24911,#24912,
#24913,#24914,#24915,#24916,#24917,#24918,#24919,#24920,#24921,#24922,#24923,
#24924,#24925,#24926,#24927,#24928,#24929,#24930,#24931,#24932,#24933,#24934,
#24935,#24936,#24937,#24938,#24939,#24940,#24941,#24942,#24943,#24944,#24945,
#24946,#24947,#24948),.UNSPECIFIED.,.F.,.F.,(4,3,3,3,3,3,3,3,3,3,3,3,3,
3,3,3,3,4),(0.,0.0290398589545852,0.0579843816831127,0.0868853129794385,
0.115761457357852,0.144631560789294,0.173538323016838,0.202474581669212,
0.231495438599219,0.249999999943415,0.279015696481717,0.307965888456499,
0.336869516661014,0.365745410794191,0.394622693781443,0.423510570114999,
0.452445568558387,0.460808762537663),.UNSPECIFIED.);
#1247=B_SPLINE_CURVE_WITH_KNOTS('',3,(#25194,#25195,#25196,#25197,#25198,
#25199,#25200,#25201,#25202,#25203,#25204,#25205,#25206,#25207,#25208,#25209,
#25210,#25211,#25212,#25213,#25214,#25215,#25216,#25217,#25218,#25219,#25220,
#25221,#25222,#25223,#25224,#25225,#25226,#25227,#25228,#25229,#25230,#25231,
#25232,#25233,#25234,#25235,#25236,#25237,#25238,#25239,#25240,#25241,#25242,
#25243,#25244,#25245),.UNSPECIFIED.,.F.,.F.,(4,3,3,3,3,3,3,3,3,3,3,3,3,
3,3,3,3,4),(0.,0.0290398589546215,0.0579843816831506,0.0868853129794766,
0.115761457357889,0.144631560789315,0.173538323016858,0.202474581669225,
0.23149543859923,0.249999999943415,0.279015696481707,0.307965888456492,
0.336869516660998,0.365745410794129,0.394622693781395,0.423510570114959,
0.452445568558335,0.460808762537663),.UNSPECIFIED.);
#1248=B_SPLINE_CURVE_WITH_KNOTS('',3,(#25366,#25367,#25368,#25369,#25370,
#25371,#25372,#25373,#25374,#25375,#25376,#25377,#25378,#25379,#25380,#25381,
#25382,#25383,#25384,#25385,#25386,#25387,#25388,#25389,#25390,#25391,#25392,
#25393,#25394,#25395,#25396,#25397,#25398,#25399,#25400,#25401,#25402,#25403,
#25404,#25405,#25406,#25407,#25408,#25409,#25410,#25411,#25412,#25413,#25414,
#25415,#25416,#25417),.UNSPECIFIED.,.F.,.F.,(4,3,3,3,3,3,3,3,3,3,3,3,3,
3,3,3,3,4),(0.,0.0290398589546135,0.0579843816831423,0.0868853129794702,
0.115761457357887,0.144631560789319,0.17353832301686,0.202474581669214,
0.231495438599214,0.249999999943415,0.27901569648171,0.307965888456478,
0.33686951666102,0.365745410794196,0.394622693781435,0.42351057011498,0.452445568558357,
0.460808762537663),.UNSPECIFIED.);
#1249=B_SPLINE_CURVE_WITH_KNOTS('',3,(#25663,#25664,#25665,#25666,#25667,
#25668,#25669,#25670,#25671,#25672,#25673,#25674,#25675,#25676,#25677,#25678,
#25679,#25680,#25681,#25682,#25683,#25684,#25685,#25686,#25687,#25688,#25689,
#25690,#25691,#25692,#25693,#25694,#25695,#25696,#25697,#25698,#25699,#25700,
#25701,#25702,#25703,#25704,#25705,#25706,#25707,#25708,#25709,#25710,#25711,
#25712,#25713,#25714),.UNSPECIFIED.,.F.,.F.,(4,3,3,3,3,3,3,3,3,3,3,3,3,
3,3,3,3,4),(0.,0.029039858954608,0.0579843816831391,0.0868853129794618,
0.11576145735788,0.144631560789298,0.173538323016834,0.202474581669206,
0.231495438599219,0.249999999943415,0.279015696481705,0.307965888456485,
0.336869516660995,0.365745410794133,0.394622693781401,0.423510570114937,
0.452445568558294,0.460808762537949),.UNSPECIFIED.);
#1250=B_SPLINE_CURVE_WITH_KNOTS('',3,(#25835,#25836,#25837,#25838,#25839,
#25840,#25841,#25842,#25843,#25844,#25845,#25846,#25847,#25848,#25849,#25850,
#25851,#25852,#25853,#25854,#25855,#25856,#25857,#25858,#25859,#25860,#25861,
#25862,#25863,#25864,#25865,#25866,#25867,#25868,#25869,#25870,#25871,#25872,
#25873,#25874,#25875,#25876,#25877,#25878,#25879,#25880,#25881,#25882,#25883,
#25884,#25885,#25886),.UNSPECIFIED.,.F.,.F.,(4,3,3,3,3,3,3,3,3,3,3,3,3,
3,3,3,3,4),(0.,0.0290398589545822,0.0579843816831122,0.0868853129794408,
0.115761457357852,0.144631560789278,0.17353832301682,0.202474581669178,
0.231495438599178,0.249999999943415,0.279015696481709,0.307965888456482,
0.336869516660988,0.365745410794173,0.394622693781441,0.423510570115002,
0.45244556855839,0.460808762537663),.UNSPECIFIED.);
#1251=B_SPLINE_CURVE_WITH_KNOTS('',3,(#26007,#26008,#26009,#26010,#26011,
#26012,#26013,#26014,#26015,#26016,#26017,#26018,#26019,#26020,#26021,#26022,
#26023,#26024,#26025,#26026,#26027,#26028,#26029,#26030,#26031,#26032,#26033,
#26034,#26035,#26036,#26037,#26038,#26039,#26040,#26041,#26042,#26043,#26044,
#26045,#26046,#26047,#26048,#26049,#26050,#26051,#26052,#26053,#26054,#26055,
#26056,#26057,#26058),.UNSPECIFIED.,.F.,.F.,(4,3,3,3,3,3,3,3,3,3,3,3,3,
3,3,3,3,4),(0.,0.0290398589545848,0.057984381683115,0.0868853129794429,
0.115761457357857,0.144631560789289,0.173538323016833,0.202474581669208,
0.231495438599203,0.249999999943415,0.279015696481713,0.307965888456485,
0.33686951666099,0.365745410794146,0.394622693781407,0.423510570114923,
0.452445568558284,0.460808762537663),.UNSPECIFIED.);
#1252=B_SPLINE_CURVE_WITH_KNOTS('',3,(#26179,#26180,#26181,#26182,#26183,
#26184,#26185,#26186,#26187,#26188,#26189,#26190,#26191,#26192,#26193,#26194,
#26195,#26196,#26197,#26198,#26199,#26200,#26201,#26202,#26203,#26204,#26205,
#26206,#26207,#26208,#26209,#26210,#26211,#26212,#26213,#26214,#26215,#26216,
#26217,#26218,#26219,#26220,#26221,#26222,#26223,#26224,#26225,#26226,#26227,
#26228,#26229,#26230),.UNSPECIFIED.,.F.,.F.,(4,3,3,3,3,3,3,3,3,3,3,3,3,
3,3,3,3,4),(0.,0.0290398589546297,0.0579843816831633,0.0868853129794911,
0.115761457357903,0.144631560789311,0.173538323016857,0.202474581669236,
0.231495438599235,0.249999999943415,0.279015696481717,0.307965888456498,
0.33686951666101,0.3657454107942,0.394622693781471,0.423510570115025,0.452445568558387,
0.460808762537948),.UNSPECIFIED.);
#1253=B_SPLINE_CURVE_WITH_KNOTS('',3,(#26351,#26352,#26353,#26354,#26355,
#26356,#26357,#26358,#26359,#26360,#26361,#26362,#26363,#26364,#26365,#26366,
#26367,#26368,#26369,#26370,#26371,#26372,#26373,#26374,#26375,#26376,#26377,
#26378,#26379,#26380,#26381,#26382,#26383,#26384,#26385,#26386,#26387,#26388,
#26389,#26390,#26391,#26392,#26393,#26394,#26395,#26396,#26397,#26398,#26399,
#26400,#26401,#26402),.UNSPECIFIED.,.F.,.F.,(4,3,3,3,3,3,3,3,3,3,3,3,3,
3,3,3,3,4),(0.,0.0290398589546329,0.0579843816831612,0.0868853129794864,
0.115761457357903,0.144631560789325,0.173538323016875,0.202474581669236,
0.231495438599232,0.249999999943415,0.279015696481708,0.307965888456492,
0.336869516660998,0.365745410794162,0.394622693781427,0.423510570114935,
0.452445568558293,0.460808762537663),.UNSPECIFIED.);
#1254=B_SPLINE_CURVE_WITH_KNOTS('',3,(#26523,#26524,#26525,#26526,#26527,
#26528,#26529,#26530,#26531,#26532,#26533,#26534,#26535,#26536,#26537,#26538,
#26539,#26540,#26541,#26542,#26543,#26544,#26545,#26546,#26547,#26548,#26549,
#26550,#26551,#26552,#26553,#26554,#26555,#26556,#26557,#26558,#26559,#26560,
#26561,#26562,#26563,#26564,#26565,#26566,#26567,#26568,#26569,#26570,#26571,
#26572,#26573,#26574),.UNSPECIFIED.,.F.,.F.,(4,3,3,3,3,3,3,3,3,3,3,3,3,
3,3,3,3,4),(0.,0.0290398589545988,0.0579843816831278,0.0868853129794553,
0.115761457357868,0.144631560789295,0.173538323016838,0.202474581669197,
0.231495438599194,0.249999999943415,0.279015696481713,0.307965888456485,
0.336869516660974,0.365745410794115,0.394622693781377,0.423510570114947,
0.452445568558327,0.460808762537662),.UNSPECIFIED.);
#1255=B_SPLINE_CURVE_WITH_KNOTS('',3,(#26695,#26696,#26697,#26698,#26699,
#26700,#26701,#26702,#26703,#26704,#26705,#26706,#26707,#26708,#26709,#26710,
#26711,#26712,#26713,#26714,#26715,#26716,#26717,#26718,#26719,#26720,#26721,
#26722,#26723,#26724,#26725,#26726,#26727,#26728,#26729,#26730,#26731,#26732,
#26733,#26734,#26735,#26736,#26737,#26738,#26739,#26740,#26741,#26742,#26743,
#26744,#26745,#26746),.UNSPECIFIED.,.F.,.F.,(4,3,3,3,3,3,3,3,3,3,3,3,3,
3,3,3,3,4),(0.,0.0290398589546069,0.0579843816831384,0.0868853129794673,
0.115761457357882,0.144631560789308,0.173538323016854,0.202474581669225,
0.231495438599218,0.249999999943415,0.279015696481714,0.30796588845649,
0.336869516661014,0.365745410794146,0.394622693781409,0.423510570114946,
0.45244556855833,0.460808762537664),.UNSPECIFIED.);
#1256=B_SPLINE_CURVE_WITH_KNOTS('',3,(#26867,#26868,#26869,#26870,#26871,
#26872,#26873,#26874,#26875,#26876,#26877,#26878,#26879,#26880,#26881,#26882,
#26883,#26884,#26885,#26886,#26887,#26888,#26889,#26890,#26891,#26892,#26893,
#26894,#26895,#26896,#26897,#26898,#26899,#26900,#26901,#26902,#26903,#26904,
#26905,#26906,#26907,#26908,#26909,#26910,#26911,#26912,#26913,#26914,#26915,
#26916,#26917,#26918),.UNSPECIFIED.,.F.,.F.,(4,3,3,3,3,3,3,3,3,3,3,3,3,
3,3,3,3,4),(0.,0.0290398589546067,0.0579843816831386,0.0868853129794601,
0.115761457357869,0.144631560789311,0.173538323016853,0.202474581669217,
0.231495438599211,0.249999999943415,0.279015696481709,0.307965888456493,
0.336869516660981,0.365745410794142,0.394622693781412,0.423510570114967,
0.452445568558324,0.460808762537663),.UNSPECIFIED.);
#1257=B_SPLINE_CURVE_WITH_KNOTS('',3,(#27039,#27040,#27041,#27042,#27043,
#27044,#27045,#27046,#27047,#27048,#27049,#27050,#27051,#27052,#27053,#27054,
#27055,#27056,#27057,#27058,#27059,#27060,#27061,#27062,#27063,#27064,#27065,
#27066,#27067,#27068,#27069,#27070,#27071,#27072,#27073,#27074,#27075,#27076,
#27077,#27078,#27079,#27080,#27081,#27082,#27083,#27084,#27085,#27086,#27087,
#27088,#27089,#27090),.UNSPECIFIED.,.F.,.F.,(4,3,3,3,3,3,3,3,3,3,3,3,3,
3,3,3,3,4),(0.,0.0290398589546235,0.0579843816831504,0.0868853129794786,
0.115761457357899,0.144631560789329,0.173538323016875,0.202474581669235,
0.231495438599228,0.249999999943415,0.279015696481717,0.307965888456488,
0.336869516661017,0.365745410794157,0.394622693781428,0.423510570114982,
0.452445568558358,0.460808762537662),.UNSPECIFIED.);
#1258=B_SPLINE_CURVE_WITH_KNOTS('',3,(#27461,#27462,#27463,#27464,#27465,
#27466,#27467,#27468,#27469,#27470,#27471,#27472,#27473,#27474,#27475,#27476,
#27477,#27478,#27479,#27480,#27481,#27482,#27483,#27484,#27485,#27486,#27487,
#27488,#27489,#27490,#27491,#27492,#27493,#27494,#27495,#27496,#27497,#27498,
#27499,#27500,#27501,#27502,#27503,#27504,#27505,#27506,#27507,#27508,#27509,
#27510,#27511,#27512),.UNSPECIFIED.,.F.,.F.,(4,3,3,3,3,3,3,3,3,3,3,3,3,
3,3,3,3,4),(0.,0.0290398589545856,0.0579843816831171,0.0868853129794436,
0.115761457357868,0.144631560789292,0.173538323016835,0.202474581669204,
0.2314954385992,0.249999999943414,0.27901569648171,0.307965888456488,0.336869516660999,
0.365745410794178,0.394622693781442,0.423510570114995,0.452445568558389,
0.460808762537663),.UNSPECIFIED.);
#1259=B_SPLINE_CURVE_WITH_KNOTS('',3,(#27633,#27634,#27635,#27636,#27637,
#27638,#27639,#27640,#27641,#27642,#27643,#27644,#27645,#27646,#27647,#27648,
#27649,#27650,#27651,#27652,#27653,#27654,#27655,#27656,#27657,#27658,#27659,
#27660,#27661,#27662,#27663,#27664,#27665,#27666,#27667,#27668,#27669,#27670,
#27671,#27672,#27673,#27674,#27675,#27676,#27677,#27678,#27679,#27680,#27681,
#27682,#27683,#27684),.UNSPECIFIED.,.F.,.F.,(4,3,3,3,3,3,3,3,3,3,3,3,3,
3,3,3,3,4),(0.,0.0290398589546211,0.0579843816831511,0.0868853129794771,
0.115761457357895,0.144631560789324,0.173538323016875,0.202474581669245,
0.231495438599253,0.249999999943415,0.279015696481702,0.307965888456477,
0.336869516660978,0.365745410794173,0.39462269378144,0.423510570114968,
0.452445568558341,0.460808762537949),.UNSPECIFIED.);
#1260=B_SPLINE_CURVE_WITH_KNOTS('',3,(#27805,#27806,#27807,#27808,#27809,
#27810,#27811,#27812,#27813,#27814,#27815,#27816,#27817,#27818,#27819,#27820,
#27821,#27822,#27823,#27824,#27825,#27826,#27827,#27828,#27829,#27830,#27831,
#27832,#27833,#27834,#27835,#27836,#27837,#27838,#27839,#27840,#27841,#27842,
#27843,#27844,#27845,#27846,#27847,#27848,#27849,#27850,#27851,#27852,#27853,
#27854,#27855,#27856),.UNSPECIFIED.,.F.,.F.,(4,3,3,3,3,3,3,3,3,3,3,3,3,
3,3,3,3,4),(0.,0.0290398589545922,0.0579843816831198,0.0868853129794405,
0.115761457357857,0.144631560789285,0.173538323016824,0.202474581669182,
0.231495438599174,0.249999999943415,0.279015696481716,0.307965888456492,
0.336869516661011,0.365745410794209,0.394622693781464,0.42351057011501,
0.452445568558355,0.460808762537948),.UNSPECIFIED.);
#1261=B_SPLINE_CURVE_WITH_KNOTS('',3,(#27977,#27978,#27979,#27980,#27981,
#27982,#27983,#27984,#27985,#27986,#27987,#27988,#27989,#27990,#27991,#27992,
#27993,#27994,#27995,#27996,#27997,#27998,#27999,#28000,#28001,#28002,#28003,
#28004,#28005,#28006,#28007,#28008,#28009,#28010,#28011,#28012,#28013,#28014,
#28015,#28016,#28017,#28018,#28019,#28020,#28021,#28022,#28023,#28024,#28025,
#28026,#28027,#28028),.UNSPECIFIED.,.F.,.F.,(4,3,3,3,3,3,3,3,3,3,3,3,3,
3,3,3,3,4),(0.,0.0290398589546412,0.0579843816831699,0.0868853129794985,
0.115761457357923,0.144631560789358,0.173538323016903,0.202474581669269,
0.231495438599259,0.249999999943415,0.279015696481711,0.307965888456494,
0.336869516660983,0.365745410794105,0.394622693781363,0.423510570114903,
0.452445568558268,0.460808762537948),.UNSPECIFIED.);
#1262=B_SPLINE_CURVE_WITH_KNOTS('',3,(#28149,#28150,#28151,#28152,#28153,
#28154,#28155,#28156,#28157,#28158,#28159,#28160,#28161,#28162,#28163,#28164,
#28165,#28166,#28167,#28168,#28169,#28170,#28171,#28172,#28173,#28174,#28175,
#28176,#28177,#28178,#28179,#28180,#28181,#28182,#28183,#28184,#28185,#28186,
#28187,#28188,#28189,#28190,#28191,#28192,#28193,#28194,#28195,#28196,#28197,
#28198,#28199,#28200),.UNSPECIFIED.,.F.,.F.,(4,3,3,3,3,3,3,3,3,3,3,3,3,
3,3,3,3,4),(0.,0.0290398589546109,0.0579843816831413,0.0868853129794694,
0.115761457357886,0.144631560789337,0.173538323016872,0.202474581669243,
0.231495438599242,0.249999999943415,0.279015696481705,0.307965888456473,
0.336869516660985,0.365745410794155,0.394622693781409,0.423510570114964,
0.452445568558341,0.460808762537948),.UNSPECIFIED.);
#1263=B_SPLINE_CURVE_WITH_KNOTS('',3,(#28321,#28322,#28323,#28324,#28325,
#28326,#28327,#28328,#28329,#28330,#28331,#28332,#28333,#28334,#28335,#28336,
#28337,#28338,#28339,#28340,#28341,#28342,#28343,#28344,#28345,#28346,#28347,
#28348,#28349,#28350,#28351,#28352,#28353,#28354,#28355,#28356,#28357,#28358,
#28359,#28360,#28361,#28362,#28363,#28364,#28365,#28366,#28367,#28368,#28369,
#28370,#28371,#28372),.UNSPECIFIED.,.F.,.F.,(4,3,3,3,3,3,3,3,3,3,3,3,3,
3,3,3,3,4),(0.,0.0290398589546184,0.0579843816831456,0.0868853129794708,
0.115761457357885,0.144631560789321,0.173538323016869,0.202474581669233,
0.231495438599223,0.249999999943415,0.279015696481714,0.307965888456492,
0.33686951666099,0.365745410794174,0.394622693781447,0.423510570115006,
0.452445568558363,0.460808762537662),.UNSPECIFIED.);
#1264=B_SPLINE_CURVE_WITH_KNOTS('',3,(#28743,#28744,#28745,#28746,#28747,
#28748,#28749,#28750,#28751,#28752,#28753,#28754,#28755,#28756,#28757,#28758,
#28759,#28760,#28761,#28762,#28763,#28764,#28765,#28766,#28767,#28768,#28769,
#28770,#28771,#28772,#28773,#28774,#28775,#28776,#28777,#28778,#28779,#28780,
#28781,#28782,#28783,#28784,#28785,#28786,#28787,#28788,#28789,#28790,#28791,
#28792,#28793,#28794),.UNSPECIFIED.,.F.,.F.,(4,3,3,3,3,3,3,3,3,3,3,3,3,
3,3,3,3,4),(0.,0.0290398589546294,0.0579843816831567,0.0868853129794856,
0.115761457357898,0.144631560789333,0.17353832301688,0.202474581669258,
0.231495438599254,0.249999999943415,0.279015696481708,0.307965888456474,
0.336869516660986,0.365745410794101,0.394622693781369,0.423510570114902,
0.45244556855825,0.460808762537663),.UNSPECIFIED.);
#1265=B_SPLINE_CURVE_WITH_KNOTS('',3,(#28915,#28916,#28917,#28918,#28919,
#28920,#28921,#28922,#28923,#28924,#28925,#28926,#28927,#28928,#28929,#28930,
#28931,#28932,#28933,#28934,#28935,#28936,#28937,#28938,#28939,#28940,#28941,
#28942,#28943,#28944,#28945,#28946,#28947,#28948,#28949,#28950,#28951,#28952,
#28953,#28954,#28955,#28956,#28957,#28958,#28959,#28960,#28961,#28962,#28963,
#28964,#28965,#28966),.UNSPECIFIED.,.F.,.F.,(4,3,3,3,3,3,3,3,3,3,3,3,3,
3,3,3,3,4),(0.,0.0290398589546234,0.0579843816831522,0.0868853129794782,
0.115761457357893,0.144631560789316,0.173538323016863,0.202474581669234,
0.231495438599237,0.249999999943415,0.27901569648171,0.307965888456479,
0.336869516660982,0.365745410794167,0.394622693781427,0.42351057011498,
0.452445568558371,0.460808762537948),.UNSPECIFIED.);
#1266=B_SPLINE_CURVE_WITH_KNOTS('',3,(#29212,#29213,#29214,#29215,#29216,
#29217,#29218,#29219,#29220,#29221,#29222,#29223,#29224,#29225,#29226,#29227,
#29228,#29229,#29230,#29231,#29232,#29233,#29234,#29235,#29236,#29237,#29238,
#29239,#29240,#29241,#29242,#29243,#29244,#29245,#29246,#29247,#29248,#29249,
#29250,#29251,#29252,#29253,#29254,#29255,#29256,#29257,#29258,#29259,#29260,
#29261,#29262,#29263),.UNSPECIFIED.,.F.,.F.,(4,3,3,3,3,3,3,3,3,3,3,3,3,
3,3,3,3,4),(0.,0.0290398589546338,0.0579843816831629,0.0868853129794867,
0.115761457357902,0.14463156078933,0.173538323016871,0.202474581669241,
0.231495438599246,0.249999999943414,0.279015696481711,0.307965888456466,
0.336869516660969,0.365745410794144,0.39462269378141,0.423510570114948,
0.452445568558332,0.460808762537663),.UNSPECIFIED.);
#1267=B_SPLINE_CURVE_WITH_KNOTS('',3,(#29384,#29385,#29386,#29387,#29388,
#29389,#29390,#29391,#29392,#29393,#29394,#29395,#29396,#29397,#29398,#29399,
#29400,#29401,#29402,#29403,#29404,#29405,#29406,#29407,#29408,#29409,#29410,
#29411,#29412,#29413,#29414,#29415,#29416,#29417,#29418,#29419,#29420,#29421,
#29422,#29423,#29424,#29425,#29426,#29427,#29428,#29429,#29430,#29431,#29432,
#29433,#29434,#29435),.UNSPECIFIED.,.F.,.F.,(4,3,3,3,3,3,3,3,3,3,3,3,3,
3,3,3,3,4),(0.,0.0290398589546154,0.0579843816831472,0.0868853129794752,
0.115761457357892,0.144631560789324,0.173538323016871,0.202474581669217,
0.231495438599219,0.249999999943415,0.27901569648171,0.307965888456471,
0.336869516660976,0.36574541079416,0.394622693781427,0.423510570115009,
0.452445568558392,0.460808762537663),.UNSPECIFIED.);
#1268=B_SPLINE_CURVE_WITH_KNOTS('',3,(#29556,#29557,#29558,#29559,#29560,
#29561,#29562,#29563,#29564,#29565,#29566,#29567,#29568,#29569,#29570,#29571,
#29572,#29573,#29574,#29575,#29576,#29577,#29578,#29579,#29580,#29581,#29582,
#29583,#29584,#29585,#29586,#29587,#29588,#29589,#29590,#29591,#29592,#29593,
#29594,#29595,#29596,#29597,#29598,#29599,#29600,#29601,#29602,#29603,#29604,
#29605,#29606,#29607),.UNSPECIFIED.,.F.,.F.,(4,3,3,3,3,3,3,3,3,3,3,3,3,
3,3,3,3,4),(0.,0.0290398589545966,0.0579843816831232,0.0868853129794503,
0.115761457357871,0.144631560789306,0.173538323016847,0.202474581669227,
0.231495438599228,0.249999999943415,0.279015696481708,0.307965888456479,
0.336869516660994,0.365745410794156,0.394622693781412,0.423510570114948,
0.452445568558316,0.460808762537949),.UNSPECIFIED.);
#1269=B_SPLINE_CURVE_WITH_KNOTS('',3,(#29728,#29729,#29730,#29731,#29732,
#29733,#29734,#29735,#29736,#29737,#29738,#29739,#29740,#29741,#29742,#29743,
#29744,#29745,#29746,#29747,#29748,#29749,#29750,#29751,#29752,#29753,#29754,
#29755,#29756,#29757,#29758,#29759,#29760,#29761,#29762,#29763,#29764,#29765,
#29766,#29767,#29768,#29769,#29770,#29771,#29772,#29773,#29774,#29775,#29776,
#29777,#29778,#29779),.UNSPECIFIED.,.F.,.F.,(4,3,3,3,3,3,3,3,3,3,3,3,3,
3,3,3,3,4),(0.,0.0290398589546008,0.0579843816831334,0.0868853129794548,
0.115761457357876,0.144631560789317,0.173538323016859,0.202474581669222,
0.231495438599218,0.249999999943415,0.279015696481709,0.307965888456467,
0.336869516660974,0.365745410794129,0.394622693781389,0.423510570114927,
0.452445568558316,0.460808762537663),.UNSPECIFIED.);
#1270=B_SPLINE_CURVE_WITH_KNOTS('',3,(#29900,#29901,#29902,#29903,#29904,
#29905,#29906,#29907,#29908,#29909,#29910,#29911,#29912,#29913,#29914,#29915,
#29916,#29917,#29918,#29919,#29920,#29921,#29922,#29923,#29924,#29925,#29926,
#29927,#29928,#29929,#29930,#29931,#29932,#29933,#29934,#29935,#29936,#29937,
#29938,#29939,#29940,#29941,#29942,#29943,#29944,#29945,#29946,#29947,#29948,
#29949,#29950,#29951),.UNSPECIFIED.,.F.,.F.,(4,3,3,3,3,3,3,3,3,3,3,3,3,
3,3,3,3,4),(0.,0.0290398589546263,0.0579843816831578,0.0868853129794855,
0.115761457357901,0.144631560789329,0.173538323016871,0.202474581669257,
0.231495438599254,0.249999999943415,0.279015696481705,0.307965888456485,
0.336869516661016,0.365745410794173,0.394622693781439,0.423510570114975,
0.452445568558338,0.460808762537663),.UNSPECIFIED.);
#1271=B_SPLINE_CURVE_WITH_KNOTS('',3,(#30207,#30208,#30209,#30210,#30211,
#30212,#30213,#30214),.UNSPECIFIED.,.F.,.F.,(4,2,2,4),(0.0783698352504338,
0.308777376437326,0.539184917624882,0.562623087291958),.UNSPECIFIED.);
#1272=B_SPLINE_CURVE_WITH_KNOTS('',3,(#30367,#30368,#30369,#30370,#30371,
#30372,#30373,#30374),.UNSPECIFIED.,.F.,.F.,(4,2,2,4),(0.0783698388401175,
0.308777379129589,0.539184919419725,0.562623088995283),.UNSPECIFIED.);
#1273=B_SPLINE_CURVE_WITH_KNOTS('',3,(#30535,#30536,#30537,#30538,#30539,
#30540,#30541,#30542),.UNSPECIFIED.,.F.,.F.,(4,2,2,4),(0.0783698437311044,
0.308777382797829,0.539184921865218,0.562623091316491),.UNSPECIFIED.);
#1274=B_SPLINE_CURVE_WITH_KNOTS('',3,(#30543,#30544,#30545,#30546,#30547,
#30548,#30549,#30550,#30551,#30552),.UNSPECIFIED.,.F.,.F.,(4,3,3,4),(0.078369843932103,
0.308777382798096,0.539184921865232,0.563918785527715),.UNSPECIFIED.);
#1275=B_SPLINE_CURVE_WITH_KNOTS('',3,(#30713,#30714,#30715,#30716,#30717,
#30718,#30719,#30720),.UNSPECIFIED.,.F.,.F.,(4,2,2,4),(0.0783698481609191,
0.30877738612019,0.539184924080125,0.5626230934188),.UNSPECIFIED.);
#1276=B_SPLINE_CURVE_WITH_KNOTS('',3,(#30873,#30874,#30875,#30876,#30877,
#30878,#30879,#30880),.UNSPECIFIED.,.F.,.F.,(4,2,2,4),(0.0783698504851113,
0.308777387863334,0.539184925242222,0.562623094521722),.UNSPECIFIED.);
#1277=B_SPLINE_CURVE_WITH_KNOTS('',3,(#31033,#31034,#31035,#31036,#31037,
#31038,#31039,#31040),.UNSPECIFIED.,.F.,.F.,(4,2,2,4),(0.0783698504851048,
0.308777387863329,0.539184925242218,0.562623094521906),.UNSPECIFIED.);
#1278=B_SPLINE_CURVE_WITH_KNOTS('',3,(#31193,#31194,#31195,#31196,#31197,
#31198,#31199,#31200),.UNSPECIFIED.,.F.,.F.,(4,2,2,4),(0.0783698481609166,
0.308777386120188,0.539184924080124,0.562623093418605),.UNSPECIFIED.);
#1279=B_SPLINE_CURVE_WITH_KNOTS('',3,(#31353,#31354,#31355,#31356,#31357,
#31358,#31359,#31360),.UNSPECIFIED.,.F.,.F.,(4,2,2,4),(0.0783698437311068,
0.308777382797831,0.539184921865219,0.56262309131643),.UNSPECIFIED.);
#1280=B_SPLINE_CURVE_WITH_KNOTS('',3,(#31513,#31514,#31515,#31516,#31517,
#31518,#31519,#31520),.UNSPECIFIED.,.F.,.F.,(4,2,2,4),(0.0783698388401241,
0.308777379129594,0.539184919419728,0.562623088995254),.UNSPECIFIED.);
#1281=B_SPLINE_CURVE_WITH_KNOTS('',3,(#31673,#31674,#31675,#31676,#31677,
#31678,#31679,#31680),.UNSPECIFIED.,.F.,.F.,(4,2,2,4),(0.0783698352504275,
0.308777376437321,0.539184917624879,0.562623087291614),.UNSPECIFIED.);
#1282=B_SPLINE_CURVE_WITH_KNOTS('',3,(#31833,#31834,#31835,#31836,#31837,
#31838,#31839,#31840),.UNSPECIFIED.,.F.,.F.,(4,2,2,4),(0.0783698293107417,
0.308777371982557,0.539184914655036,0.562623084473152),.UNSPECIFIED.);
#1283=B_SPLINE_CURVE_WITH_KNOTS('',3,(#32001,#32002,#32003,#32004,#32005,
#32006,#32007,#32008),.UNSPECIFIED.,.F.,.F.,(4,2,2,4),(0.0783698352504225,
0.308777376437317,0.539184917624877,0.562623087291754),.UNSPECIFIED.);
#1284=B_SPLINE_CURVE_WITH_KNOTS('',3,(#32009,#32010,#32011,#32012,#32013,
#32014,#32015,#32016,#32017,#32018),.UNSPECIFIED.,.F.,.F.,(4,3,3,4),(0.0783698354514212,
0.308777376437563,0.53918491762485,0.563918781514903),.UNSPECIFIED.);
#1285=B_SPLINE_CURVE_WITH_KNOTS('',3,(#32179,#32180,#32181,#32182,#32183,
#32184,#32185,#32186),.UNSPECIFIED.,.F.,.F.,(4,2,2,4),(0.0783698388401176,
0.308777379129589,0.539184919419725,0.562623088995512),.UNSPECIFIED.);
#1286=B_SPLINE_CURVE_WITH_KNOTS('',3,(#32339,#32340,#32341,#32342,#32343,
#32344,#32345,#32346),.UNSPECIFIED.,.F.,.F.,(4,2,2,4),(0.078369843731106,
0.30877738279783,0.539184921865219,0.56262309131667),.UNSPECIFIED.);
#1287=B_SPLINE_CURVE_WITH_KNOTS('',3,(#32555,#32556,#32557,#32558,#32559,
#32560,#32561,#32562),.UNSPECIFIED.,.F.,.F.,(4,2,2,4),(0.0783698481609151,
0.308777386120187,0.539184924080123,0.562623093418658),.UNSPECIFIED.);
#1288=B_SPLINE_CURVE_WITH_KNOTS('',3,(#32659,#32660,#32661,#32662,#32663,
#32664,#32665,#32666),.UNSPECIFIED.,.F.,.F.,(4,2,2,4),(0.0783698504851104,
0.308777387863333,0.539184925242221,0.562623094521848),.UNSPECIFIED.);
#1289=B_SPLINE_CURVE_WITH_KNOTS('',3,(#32819,#32820,#32821,#32822,#32823,
#32824,#32825,#32826),.UNSPECIFIED.,.F.,.F.,(4,2,2,4),(0.0783698504851007,
0.308777387863326,0.539184925242216,0.562623094521626),.UNSPECIFIED.);
#1290=B_SPLINE_CURVE_WITH_KNOTS('',3,(#32979,#32980,#32981,#32982,#32983,
#32984,#32985,#32986),.UNSPECIFIED.,.F.,.F.,(4,2,2,4),(0.0783698481609159,
0.308777386120187,0.539184924080124,0.562623093418695),.UNSPECIFIED.);
#1291=B_SPLINE_CURVE_WITH_KNOTS('',3,(#33139,#33140,#33141,#33142,#33143,
#33144,#33145,#33146),.UNSPECIFIED.,.F.,.F.,(4,2,2,4),(0.0783698437310911,
0.308777382797819,0.539184921865211,0.562623091316394),.UNSPECIFIED.);
#1292=B_SPLINE_CURVE_WITH_KNOTS('',3,(#33299,#33300,#33301,#33302,#33303,
#33304,#33305,#33306),.UNSPECIFIED.,.F.,.F.,(4,2,2,4),(0.0783698388401225,
0.308777379129592,0.539184919419727,0.562623088994977),.UNSPECIFIED.);
#1293=B_SPLINE_CURVE_WITH_KNOTS('',3,(#33459,#33460,#33461,#33462,#33463,
#33464,#33465,#33466),.UNSPECIFIED.,.F.,.F.,(4,2,2,4),(0.0783698352504349,
0.308777376437327,0.539184917624883,0.562623087291856),.UNSPECIFIED.);
#1294=B_SPLINE_CURVE_WITH_KNOTS('',3,(#33619,#33620,#33621,#33622,#33623,
#33624,#33625,#33626),.UNSPECIFIED.,.F.,.F.,(4,2,2,4),(0.0783698293107414,
0.308777371982556,0.539184914655036,0.562623084473124),.UNSPECIFIED.);
#1295=B_SPLINE_CURVE_WITH_KNOTS('',3,(#33779,#33780,#33781,#33782,#33783,
#33784,#33785,#33786),.UNSPECIFIED.,.F.,.F.,(4,2,2,4),(0.0783698352504222,
0.308777376437317,0.539184917624877,0.562623087291584),.UNSPECIFIED.);
#1296=B_SPLINE_CURVE_WITH_KNOTS('',3,(#33939,#33940,#33941,#33942,#33943,
#33944,#33945,#33946),.UNSPECIFIED.,.F.,.F.,(4,2,2,4),(0.078369838840123,
0.308777379129593,0.539184919419728,0.562623088995037),.UNSPECIFIED.);
#1297=B_SPLINE_CURVE_WITH_KNOTS('',3,(#34107,#34108,#34109,#34110,#34111,
#34112,#34113,#34114),.UNSPECIFIED.,.F.,.F.,(4,2,2,4),(0.0783698437311085,
0.308777382797832,0.53918492186522,0.562623091316454),.UNSPECIFIED.);
#1298=B_SPLINE_CURVE_WITH_KNOTS('',3,(#34115,#34116,#34117,#34118,#34119,
#34120,#34121,#34122,#34123,#34124),.UNSPECIFIED.,.F.,.F.,(4,3,3,4),(0.078369843932107,
0.308777382798091,0.539184921865221,0.563918785527689),.UNSPECIFIED.);
#1299=B_SPLINE_CURVE_WITH_KNOTS('',3,(#34293,#34294,#34295,#34296,#34297,
#34298,#34299,#34300),.UNSPECIFIED.,.F.,.F.,(4,2,2,4),(0.078369848160917,
0.308777386120188,0.539184924080124,0.562623093418646),.UNSPECIFIED.);
#1300=B_SPLINE_CURVE_WITH_KNOTS('',3,(#34301,#34302,#34303,#34304,#34305,
#34306,#34307,#34308,#34309,#34310),.UNSPECIFIED.,.F.,.F.,(4,3,3,4),(0.0783698483619153,
0.308777386120433,0.539184924080096,0.563918787623678),.UNSPECIFIED.);
#1301=B_SPLINE_CURVE_WITH_KNOTS('',3,(#34471,#34472,#34473,#34474,#34475,
#34476,#34477,#34478),.UNSPECIFIED.,.F.,.F.,(4,2,2,4),(0.0783698504850856,
0.308777387863315,0.539184925242209,0.56262309452169),.UNSPECIFIED.);
#1302=B_SPLINE_CURVE_WITH_KNOTS('',3,(#34631,#34632,#34633,#34634,#34635,
#34636,#34637,#34638),.UNSPECIFIED.,.F.,.F.,(4,2,2,4),(0.0783698504851055,
0.30877738786333,0.539184925242219,0.562623094521574),.UNSPECIFIED.);
#1303=B_SPLINE_CURVE_WITH_KNOTS('',3,(#34791,#34792,#34793,#34794,#34795,
#34796,#34797,#34798),.UNSPECIFIED.,.F.,.F.,(4,2,2,4),(0.0783698481609001,
0.308777386120176,0.539184924080116,0.562623093418498),.UNSPECIFIED.);
#1304=B_SPLINE_CURVE_WITH_KNOTS('',3,(#34951,#34952,#34953,#34954,#34955,
#34956,#34957,#34958),.UNSPECIFIED.,.F.,.F.,(4,2,2,4),(0.0783698437310988,
0.308777382797825,0.539184921865215,0.562623091316541),.UNSPECIFIED.);
#1305=B_SPLINE_CURVE_WITH_KNOTS('',3,(#35111,#35112,#35113,#35114,#35115,
#35116,#35117,#35118),.UNSPECIFIED.,.F.,.F.,(4,2,2,4),(0.0783698388401159,
0.308777379129587,0.539184919419724,0.562623088995074),.UNSPECIFIED.);
#1306=B_SPLINE_CURVE_WITH_KNOTS('',3,(#35271,#35272,#35273,#35274,#35275,
#35276,#35277,#35278),.UNSPECIFIED.,.F.,.F.,(4,2,2,4),(0.0783698352504283,
0.308777376437322,0.53918491762488,0.562623087291795),.UNSPECIFIED.);
#1307=B_SPLINE_CURVE_WITH_KNOTS('',3,(#35439,#35440,#35441,#35442,#35443,
#35444,#35445,#35446),.UNSPECIFIED.,.F.,.F.,(4,2,2,4),(0.0783698293107271,
0.308777371982546,0.53918491465503,0.562623084473022),.UNSPECIFIED.);
#1308=B_SPLINE_CURVE_WITH_KNOTS('',3,(#35447,#35448,#35449,#35450,#35451,
#35452,#35453,#35454,#35455,#35456),.UNSPECIFIED.,.F.,.F.,(4,3,3,4),(0.0783698295117259,
0.308777371982838,0.539184914655095,0.563918778704584),.UNSPECIFIED.);
#1309=B_SPLINE_CURVE_WITH_KNOTS('',3,(#35625,#35626,#35627,#35628,#35629,
#35630,#35631,#35632),.UNSPECIFIED.,.F.,.F.,(4,2,2,4),(0.0783698352504227,
0.308777376437317,0.539184917624878,0.56262308729164),.UNSPECIFIED.);
#1310=B_SPLINE_CURVE_WITH_KNOTS('',3,(#35633,#35634,#35635,#35636,#35637,
#35638,#35639,#35640,#35641,#35642),.UNSPECIFIED.,.F.,.F.,(4,3,3,4),(0.0783698354514214,
0.308777376437584,0.539184917624891,0.563918781514891),.UNSPECIFIED.);
#1311=B_SPLINE_CURVE_WITH_KNOTS('',3,(#35803,#35804,#35805,#35806,#35807,
#35808,#35809,#35810),.UNSPECIFIED.,.F.,.F.,(4,2,2,4),(0.078369838840114,
0.308777379129586,0.539184919419723,0.562623088995413),.UNSPECIFIED.);
#1312=B_SPLINE_CURVE_WITH_KNOTS('',3,(#35963,#35964,#35965,#35966,#35967,
#35968,#35969,#35970),.UNSPECIFIED.,.F.,.F.,(4,2,2,4),(0.078369843731106,
0.30877738279783,0.539184921865219,0.562623091316345),.UNSPECIFIED.);
#1313=B_SPLINE_CURVE_WITH_KNOTS('',3,(#36179,#36180,#36181,#36182,#36183,
#36184,#36185,#36186),.UNSPECIFIED.,.F.,.F.,(4,2,2,4),(0.0783698481609172,
0.308777386120188,0.539184924080125,0.562623093418633),.UNSPECIFIED.);
#1314=B_SPLINE_CURVE_WITH_KNOTS('',3,(#36283,#36284,#36285,#36286,#36287,
#36288,#36289,#36290),.UNSPECIFIED.,.F.,.F.,(4,2,2,4),(0.0783698504850854,
0.308777387863314,0.539184925242208,0.562623094521865),.UNSPECIFIED.);
#1315=B_SPLINE_CURVE_WITH_KNOTS('',3,(#36443,#36444,#36445,#36446,#36447,
#36448,#36449,#36450),.UNSPECIFIED.,.F.,.F.,(4,2,2,4),(0.0783698504851049,
0.308777387863329,0.539184925242218,0.562623094521782),.UNSPECIFIED.);
#1316=B_SPLINE_CURVE_WITH_KNOTS('',3,(#36603,#36604,#36605,#36606,#36607,
#36608,#36609,#36610),.UNSPECIFIED.,.F.,.F.,(4,2,2,4),(0.0783698481609187,
0.30877738612019,0.539184924080125,0.562623093418547),.UNSPECIFIED.);
#1317=B_SPLINE_CURVE_WITH_KNOTS('',3,(#36763,#36764,#36765,#36766,#36767,
#36768,#36769,#36770),.UNSPECIFIED.,.F.,.F.,(4,2,2,4),(0.0783698437311104,
0.308777382797833,0.539184921865221,0.562623091316399),.UNSPECIFIED.);
#1318=B_SPLINE_CURVE_WITH_KNOTS('',3,(#36923,#36924,#36925,#36926,#36927,
#36928,#36929,#36930),.UNSPECIFIED.,.F.,.F.,(4,2,2,4),(0.0783698388401129,
0.308777379129585,0.539184919419723,0.562623088995376),.UNSPECIFIED.);
#1319=B_SPLINE_CURVE_WITH_KNOTS('',3,(#37091,#37092,#37093,#37094,#37095,
#37096,#37097,#37098),.UNSPECIFIED.,.F.,.F.,(4,2,2,4),(0.0783698352504293,
0.308777376437322,0.53918491762488,0.562623087291725),.UNSPECIFIED.);
#1320=B_SPLINE_CURVE_WITH_KNOTS('',3,(#37099,#37100,#37101,#37102,#37103,
#37104,#37105,#37106,#37107,#37108),.UNSPECIFIED.,.F.,.F.,(4,3,3,4),(0.078369835451428,
0.308777376437561,0.539184917624838,0.563918781514903),.UNSPECIFIED.);
#1324=SHAPE_REPRESENTATION_RELATIONSHIP('SRR','None',#37957,#1336);
#1336=ADVANCED_BREP_SHAPE_REPRESENTATION('',(#1360),#37872);
#1348=STYLED_ITEM('',(#38023),#1360);
#1360=MANIFOLD_SOLID_BREP('Body1',#10822);
#1405=FACE_BOUND('',#2421,.T.);
#1406=FACE_BOUND('',#2423,.T.);
#1504=PLANE('',#11426);
#1505=PLANE('',#11427);
#1506=PLANE('',#11428);
#1507=PLANE('',#11429);
#1508=PLANE('',#11430);
#1648=FACE_OUTER_BOUND('',#2285,.T.);
#1649=FACE_OUTER_BOUND('',#2286,.T.);
#1650=FACE_OUTER_BOUND('',#2287,.T.);
#1651=FACE_OUTER_BOUND('',#2288,.T.);
#1652=FACE_OUTER_BOUND('',#2289,.T.);
#1653=FACE_OUTER_BOUND('',#2290,.T.);
#1654=FACE_OUTER_BOUND('',#2291,.T.);
#1655=FACE_OUTER_BOUND('',#2292,.T.);
#1656=FACE_OUTER_BOUND('',#2293,.T.);
#1657=FACE_OUTER_BOUND('',#2294,.T.);
#1658=FACE_OUTER_BOUND('',#2295,.T.);
#1659=FACE_OUTER_BOUND('',#2296,.T.);
#1660=FACE_OUTER_BOUND('',#2297,.T.);
#1661=FACE_OUTER_BOUND('',#2298,.T.);
#1662=FACE_OUTER_BOUND('',#2299,.T.);
#1663=FACE_OUTER_BOUND('',#2300,.T.);
#1664=FACE_OUTER_BOUND('',#2301,.T.);
#1665=FACE_OUTER_BOUND('',#2302,.T.);
#1666=FACE_OUTER_BOUND('',#2303,.T.);
#1667=FACE_OUTER_BOUND('',#2304,.T.);
#1668=FACE_OUTER_BOUND('',#2305,.T.);
#1669=FACE_OUTER_BOUND('',#2306,.T.);
#1670=FACE_OUTER_BOUND('',#2307,.T.);
#1671=FACE_OUTER_BOUND('',#2308,.T.);
#1672=FACE_OUTER_BOUND('',#2309,.T.);
#1673=FACE_OUTER_BOUND('',#2310,.T.);
#1674=FACE_OUTER_BOUND('',#2311,.T.);
#1675=FACE_OUTER_BOUND('',#2312,.T.);
#1676=FACE_OUTER_BOUND('',#2313,.T.);
#1677=FACE_OUTER_BOUND('',#2314,.T.);
#1678=FACE_OUTER_BOUND('',#2315,.T.);
#1679=FACE_OUTER_BOUND('',#2316,.T.);
#1680=FACE_OUTER_BOUND('',#2317,.T.);
#1681=FACE_OUTER_BOUND('',#2318,.T.);
#1682=FACE_OUTER_BOUND('',#2319,.T.);
#1683=FACE_OUTER_BOUND('',#2320,.T.);
#1684=FACE_OUTER_BOUND('',#2321,.T.);
#1685=FACE_OUTER_BOUND('',#2322,.T.);
#1686=FACE_OUTER_BOUND('',#2323,.T.);
#1687=FACE_OUTER_BOUND('',#2324,.T.);
#1688=FACE_OUTER_BOUND('',#2325,.T.);
#1689=FACE_OUTER_BOUND('',#2326,.T.);
#1690=FACE_OUTER_BOUND('',#2327,.T.);
#1691=FACE_OUTER_BOUND('',#2328,.T.);
#1692=FACE_OUTER_BOUND('',#2329,.T.);
#1693=FACE_OUTER_BOUND('',#2330,.T.);
#1694=FACE_OUTER_BOUND('',#2331,.T.);
#1695=FACE_OUTER_BOUND('',#2332,.T.);
#1696=FACE_OUTER_BOUND('',#2333,.T.);
#1697=FACE_OUTER_BOUND('',#2334,.T.);
#1698=FACE_OUTER_BOUND('',#2335,.T.);
#1699=FACE_OUTER_BOUND('',#2336,.T.);
#1700=FACE_OUTER_BOUND('',#2337,.T.);
#1701=FACE_OUTER_BOUND('',#2338,.T.);
#1702=FACE_OUTER_BOUND('',#2339,.T.);
#1703=FACE_OUTER_BOUND('',#2340,.T.);
#1704=FACE_OUTER_BOUND('',#2341,.T.);
#1705=FACE_OUTER_BOUND('',#2342,.T.);
#1706=FACE_OUTER_BOUND('',#2343,.T.);
#1707=FACE_OUTER_BOUND('',#2344,.T.);
#1708=FACE_OUTER_BOUND('',#2345,.T.);
#1709=FACE_OUTER_BOUND('',#2346,.T.);
#1710=FACE_OUTER_BOUND('',#2347,.T.);
#1711=FACE_OUTER_BOUND('',#2348,.T.);
#1712=FACE_OUTER_BOUND('',#2349,.T.);
#1713=FACE_OUTER_BOUND('',#2350,.T.);
#1714=FACE_OUTER_BOUND('',#2351,.T.);
#1715=FACE_OUTER_BOUND('',#2352,.T.);
#1716=FACE_OUTER_BOUND('',#2353,.T.);
#1717=FACE_OUTER_BOUND('',#2354,.T.);
#1718=FACE_OUTER_BOUND('',#2355,.T.);
#1719=FACE_OUTER_BOUND('',#2356,.T.);
#1720=FACE_OUTER_BOUND('',#2357,.T.);
#1721=FACE_OUTER_BOUND('',#2358,.T.);
#1722=FACE_OUTER_BOUND('',#2359,.T.);
#1723=FACE_OUTER_BOUND('',#2360,.T.);
#1724=FACE_OUTER_BOUND('',#2361,.T.);
#1725=FACE_OUTER_BOUND('',#2362,.T.);
#1726=FACE_OUTER_BOUND('',#2363,.T.);
#1727=FACE_OUTER_BOUND('',#2364,.T.);
#1728=FACE_OUTER_BOUND('',#2365,.T.);
#1729=FACE_OUTER_BOUND('',#2366,.T.);
#1730=FACE_OUTER_BOUND('',#2367,.T.);
#1731=FACE_OUTER_BOUND('',#2368,.T.);
#1732=FACE_OUTER_BOUND('',#2369,.T.);
#1733=FACE_OUTER_BOUND('',#2370,.T.);
#1734=FACE_OUTER_BOUND('',#2371,.T.);
#1735=FACE_OUTER_BOUND('',#2372,.T.);
#1736=FACE_OUTER_BOUND('',#2373,.T.);
#1737=FACE_OUTER_BOUND('',#2374,.T.);
#1738=FACE_OUTER_BOUND('',#2375,.T.);
#1739=FACE_OUTER_BOUND('',#2376,.T.);
#1740=FACE_OUTER_BOUND('',#2377,.T.);
#1741=FACE_OUTER_BOUND('',#2378,.T.);
#1742=FACE_OUTER_BOUND('',#2379,.T.);
#1743=FACE_OUTER_BOUND('',#2380,.T.);
#1744=FACE_OUTER_BOUND('',#2381,.T.);
#1745=FACE_OUTER_BOUND('',#2382,.T.);
#1746=FACE_OUTER_BOUND('',#2383,.T.);
#1747=FACE_OUTER_BOUND('',#2384,.T.);
#1748=FACE_OUTER_BOUND('',#2385,.T.);
#1749=FACE_OUTER_BOUND('',#2386,.T.);
#1750=FACE_OUTER_BOUND('',#2387,.T.);
#1751=FACE_OUTER_BOUND('',#2388,.T.);
#1752=FACE_OUTER_BOUND('',#2389,.T.);
#1753=FACE_OUTER_BOUND('',#2390,.T.);
#1754=FACE_OUTER_BOUND('',#2391,.T.);
#1755=FACE_OUTER_BOUND('',#2392,.T.);
#1756=FACE_OUTER_BOUND('',#2393,.T.);
#1757=FACE_OUTER_BOUND('',#2394,.T.);
#1758=FACE_OUTER_BOUND('',#2395,.T.);
#1759=FACE_OUTER_BOUND('',#2396,.T.);
#1760=FACE_OUTER_BOUND('',#2397,.T.);
#1761=FACE_OUTER_BOUND('',#2398,.T.);
#1762=FACE_OUTER_BOUND('',#2399,.T.);
#1763=FACE_OUTER_BOUND('',#2400,.T.);
#1764=FACE_OUTER_BOUND('',#2401,.T.);
#1765=FACE_OUTER_BOUND('',#2402,.T.);
#1766=FACE_OUTER_BOUND('',#2403,.T.);
#1767=FACE_OUTER_BOUND('',#2404,.T.);
#1768=FACE_OUTER_BOUND('',#2405,.T.);
#1769=FACE_OUTER_BOUND('',#2406,.T.);
#1770=FACE_OUTER_BOUND('',#2407,.T.);
#1771=FACE_OUTER_BOUND('',#2408,.T.);
#1772=FACE_OUTER_BOUND('',#2409,.T.);
#1773=FACE_OUTER_BOUND('',#2410,.T.);
#1774=FACE_OUTER_BOUND('',#2411,.T.);
#1775=FACE_OUTER_BOUND('',#2412,.T.);
#1776=FACE_OUTER_BOUND('',#2413,.T.);
#1777=FACE_OUTER_BOUND('',#2414,.T.);
#1778=FACE_OUTER_BOUND('',#2415,.T.);
#1779=FACE_OUTER_BOUND('',#2416,.T.);
#1780=FACE_OUTER_BOUND('',#2417,.T.);
#1781=FACE_OUTER_BOUND('',#2418,.T.);
#1782=FACE_OUTER_BOUND('',#2419,.T.);
#1783=FACE_OUTER_BOUND('',#2420,.T.);
#1784=FACE_OUTER_BOUND('',#2422,.T.);
#1785=FACE_OUTER_BOUND('',#2424,.T.);
#1786=FACE_OUTER_BOUND('',#2425,.T.);
#1787=FACE_OUTER_BOUND('',#2426,.T.);
#1788=FACE_OUTER_BOUND('',#2427,.T.);
#1789=FACE_OUTER_BOUND('',#2428,.T.);
#1790=FACE_OUTER_BOUND('',#2429,.T.);
#1791=FACE_OUTER_BOUND('',#2430,.T.);
#1792=FACE_OUTER_BOUND('',#2431,.T.);
#1793=FACE_OUTER_BOUND('',#2432,.T.);
#1794=FACE_OUTER_BOUND('',#2433,.T.);
#1795=FACE_OUTER_BOUND('',#2434,.T.);
#1796=FACE_OUTER_BOUND('',#2435,.T.);
#1797=FACE_OUTER_BOUND('',#2436,.T.);
#1798=FACE_OUTER_BOUND('',#2437,.T.);
#1799=FACE_OUTER_BOUND('',#2438,.T.);
#1800=FACE_OUTER_BOUND('',#2439,.T.);
#1801=FACE_OUTER_BOUND('',#2440,.T.);
#1802=FACE_OUTER_BOUND('',#2441,.T.);
#1803=FACE_OUTER_BOUND('',#2442,.T.);
#1804=FACE_OUTER_BOUND('',#2443,.T.);
#1805=FACE_OUTER_BOUND('',#2444,.T.);
#1806=FACE_OUTER_BOUND('',#2445,.T.);
#1807=FACE_OUTER_BOUND('',#2446,.T.);
#1808=FACE_OUTER_BOUND('',#2447,.T.);
#1809=FACE_OUTER_BOUND('',#2448,.T.);
#1810=FACE_OUTER_BOUND('',#2449,.T.);
#1811=FACE_OUTER_BOUND('',#2450,.T.);
#1812=FACE_OUTER_BOUND('',#2451,.T.);
#1813=FACE_OUTER_BOUND('',#2452,.T.);
#1814=FACE_OUTER_BOUND('',#2453,.T.);
#1815=FACE_OUTER_BOUND('',#2454,.T.);
#1816=FACE_OUTER_BOUND('',#2455,.T.);
#1817=FACE_OUTER_BOUND('',#2456,.T.);
#1818=FACE_OUTER_BOUND('',#2457,.T.);
#1819=FACE_OUTER_BOUND('',#2458,.T.);
#1820=FACE_OUTER_BOUND('',#2459,.T.);
#1821=FACE_OUTER_BOUND('',#2460,.T.);
#1822=FACE_OUTER_BOUND('',#2461,.T.);
#1823=FACE_OUTER_BOUND('',#2462,.T.);
#1824=FACE_OUTER_BOUND('',#2463,.T.);
#1825=FACE_OUTER_BOUND('',#2464,.T.);
#1826=FACE_OUTER_BOUND('',#2465,.T.);
#1827=FACE_OUTER_BOUND('',#2466,.T.);
#1828=FACE_OUTER_BOUND('',#2467,.T.);
#1829=FACE_OUTER_BOUND('',#2468,.T.);
#1830=FACE_OUTER_BOUND('',#2469,.T.);
#1831=FACE_OUTER_BOUND('',#2470,.T.);
#1832=FACE_OUTER_BOUND('',#2471,.T.);
#1833=FACE_OUTER_BOUND('',#2472,.T.);
#1834=FACE_OUTER_BOUND('',#2473,.T.);
#1835=FACE_OUTER_BOUND('',#2474,.T.);
#1836=FACE_OUTER_BOUND('',#2475,.T.);
#1837=FACE_OUTER_BOUND('',#2476,.T.);
#1838=FACE_OUTER_BOUND('',#2477,.T.);
#1839=FACE_OUTER_BOUND('',#2478,.T.);
#1840=FACE_OUTER_BOUND('',#2479,.T.);
#1841=FACE_OUTER_BOUND('',#2480,.T.);
#1842=FACE_OUTER_BOUND('',#2481,.T.);
#1843=FACE_OUTER_BOUND('',#2482,.T.);
#1844=FACE_OUTER_BOUND('',#2483,.T.);
#1845=FACE_OUTER_BOUND('',#2484,.T.);
#1846=FACE_OUTER_BOUND('',#2485,.T.);
#1847=FACE_OUTER_BOUND('',#2486,.T.);
#1848=FACE_OUTER_BOUND('',#2487,.T.);
#1849=FACE_OUTER_BOUND('',#2488,.T.);
#1850=FACE_OUTER_BOUND('',#2489,.T.);
#1851=FACE_OUTER_BOUND('',#2490,.T.);
#1852=FACE_OUTER_BOUND('',#2491,.T.);
#1853=FACE_OUTER_BOUND('',#2492,.T.);
#1854=FACE_OUTER_BOUND('',#2493,.T.);
#1855=FACE_OUTER_BOUND('',#2494,.T.);
#1856=FACE_OUTER_BOUND('',#2495,.T.);
#1857=FACE_OUTER_BOUND('',#2496,.T.);
#1858=FACE_OUTER_BOUND('',#2497,.T.);
#1859=FACE_OUTER_BOUND('',#2498,.T.);
#1860=FACE_OUTER_BOUND('',#2499,.T.);
#1861=FACE_OUTER_BOUND('',#2500,.T.);
#1862=FACE_OUTER_BOUND('',#2501,.T.);
#1863=FACE_OUTER_BOUND('',#2502,.T.);
#1864=FACE_OUTER_BOUND('',#2503,.T.);
#1865=FACE_OUTER_BOUND('',#2504,.T.);
#1866=FACE_OUTER_BOUND('',#2505,.T.);
#1867=FACE_OUTER_BOUND('',#2506,.T.);
#1868=FACE_OUTER_BOUND('',#2507,.T.);
#1869=FACE_OUTER_BOUND('',#2508,.T.);
#1870=FACE_OUTER_BOUND('',#2509,.T.);
#1871=FACE_OUTER_BOUND('',#2510,.T.);
#1872=FACE_OUTER_BOUND('',#2511,.T.);
#1873=FACE_OUTER_BOUND('',#2512,.T.);
#1874=FACE_OUTER_BOUND('',#2513,.T.);
#1875=FACE_OUTER_BOUND('',#2514,.T.);
#1876=FACE_OUTER_BOUND('',#2515,.T.);
#1877=FACE_OUTER_BOUND('',#2516,.T.);
#1878=FACE_OUTER_BOUND('',#2517,.T.);
#1879=FACE_OUTER_BOUND('',#2518,.T.);
#1880=FACE_OUTER_BOUND('',#2519,.T.);
#1881=FACE_OUTER_BOUND('',#2520,.T.);
#1882=FACE_OUTER_BOUND('',#2521,.T.);
#1883=FACE_OUTER_BOUND('',#2522,.T.);
#1884=FACE_OUTER_BOUND('',#2523,.T.);
#1885=FACE_OUTER_BOUND('',#2524,.T.);
#1886=FACE_OUTER_BOUND('',#2525,.T.);
#1887=FACE_OUTER_BOUND('',#2526,.T.);
#1888=FACE_OUTER_BOUND('',#2527,.T.);
#1889=FACE_OUTER_BOUND('',#2528,.T.);
#1890=FACE_OUTER_BOUND('',#2529,.T.);
#1891=FACE_OUTER_BOUND('',#2530,.T.);
#1892=FACE_OUTER_BOUND('',#2531,.T.);
#1893=FACE_OUTER_BOUND('',#2532,.T.);
#1894=FACE_OUTER_BOUND('',#2533,.T.);
#1895=FACE_OUTER_BOUND('',#2534,.T.);
#1896=FACE_OUTER_BOUND('',#2535,.T.);
#1897=FACE_OUTER_BOUND('',#2536,.T.);
#1898=FACE_OUTER_BOUND('',#2537,.T.);
#1899=FACE_OUTER_BOUND('',#2538,.T.);
#1900=FACE_OUTER_BOUND('',#2539,.T.);
#1901=FACE_OUTER_BOUND('',#2540,.T.);
#1902=FACE_OUTER_BOUND('',#2541,.T.);
#1903=FACE_OUTER_BOUND('',#2542,.T.);
#1904=FACE_OUTER_BOUND('',#2543,.T.);
#1905=FACE_OUTER_BOUND('',#2544,.T.);
#1906=FACE_OUTER_BOUND('',#2545,.T.);
#1907=FACE_OUTER_BOUND('',#2546,.T.);
#1908=FACE_OUTER_BOUND('',#2547,.T.);
#1909=FACE_OUTER_BOUND('',#2548,.T.);
#1910=FACE_OUTER_BOUND('',#2549,.T.);
#1911=FACE_OUTER_BOUND('',#2550,.T.);
#1912=FACE_OUTER_BOUND('',#2551,.T.);
#1913=FACE_OUTER_BOUND('',#2552,.T.);
#1914=FACE_OUTER_BOUND('',#2553,.T.);
#1915=FACE_OUTER_BOUND('',#2554,.T.);
#1916=FACE_OUTER_BOUND('',#2555,.T.);
#1917=FACE_OUTER_BOUND('',#2556,.T.);
#1918=FACE_OUTER_BOUND('',#2557,.T.);
#1919=FACE_OUTER_BOUND('',#2558,.T.);
#1920=FACE_OUTER_BOUND('',#2559,.T.);
#1921=FACE_OUTER_BOUND('',#2560,.T.);
#1922=FACE_OUTER_BOUND('',#2561,.T.);
#1923=FACE_OUTER_BOUND('',#2562,.T.);
#1924=FACE_OUTER_BOUND('',#2563,.T.);
#1925=FACE_OUTER_BOUND('',#2564,.T.);
#1926=FACE_OUTER_BOUND('',#2565,.T.);
#1927=FACE_OUTER_BOUND('',#2566,.T.);
#1928=FACE_OUTER_BOUND('',#2567,.T.);
#1929=FACE_OUTER_BOUND('',#2568,.T.);
#1930=FACE_OUTER_BOUND('',#2569,.T.);
#1931=FACE_OUTER_BOUND('',#2570,.T.);
#1932=FACE_OUTER_BOUND('',#2571,.T.);
#1933=FACE_OUTER_BOUND('',#2572,.T.);
#1934=FACE_OUTER_BOUND('',#2573,.T.);
#1935=FACE_OUTER_BOUND('',#2574,.T.);
#1936=FACE_OUTER_BOUND('',#2575,.T.);
#1937=FACE_OUTER_BOUND('',#2576,.T.);
#1938=FACE_OUTER_BOUND('',#2577,.T.);
#1939=FACE_OUTER_BOUND('',#2578,.T.);
#1940=FACE_OUTER_BOUND('',#2579,.T.);
#1941=FACE_OUTER_BOUND('',#2580,.T.);
#1942=FACE_OUTER_BOUND('',#2581,.T.);
#1943=FACE_OUTER_BOUND('',#2582,.T.);
#1944=FACE_OUTER_BOUND('',#2583,.T.);
#1945=FACE_OUTER_BOUND('',#2584,.T.);
#1946=FACE_OUTER_BOUND('',#2585,.T.);
#1947=FACE_OUTER_BOUND('',#2586,.T.);
#1948=FACE_OUTER_BOUND('',#2587,.T.);
#1949=FACE_OUTER_BOUND('',#2588,.T.);
#1950=FACE_OUTER_BOUND('',#2589,.T.);
#1951=FACE_OUTER_BOUND('',#2590,.T.);
#1952=FACE_OUTER_BOUND('',#2591,.T.);
#1953=FACE_OUTER_BOUND('',#2592,.T.);
#1954=FACE_OUTER_BOUND('',#2593,.T.);
#1955=FACE_OUTER_BOUND('',#2594,.T.);
#1956=FACE_OUTER_BOUND('',#2595,.T.);
#1957=FACE_OUTER_BOUND('',#2596,.T.);
#1958=FACE_OUTER_BOUND('',#2597,.T.);
#1959=FACE_OUTER_BOUND('',#2598,.T.);
#1960=FACE_OUTER_BOUND('',#2599,.T.);
#1961=FACE_OUTER_BOUND('',#2600,.T.);
#1962=FACE_OUTER_BOUND('',#2601,.T.);
#1963=FACE_OUTER_BOUND('',#2602,.T.);
#1964=FACE_OUTER_BOUND('',#2603,.T.);
#1965=FACE_OUTER_BOUND('',#2604,.T.);
#1966=FACE_OUTER_BOUND('',#2605,.T.);
#1967=FACE_OUTER_BOUND('',#2606,.T.);
#1968=FACE_OUTER_BOUND('',#2607,.T.);
#1969=FACE_OUTER_BOUND('',#2608,.T.);
#1970=FACE_OUTER_BOUND('',#2609,.T.);
#1971=FACE_OUTER_BOUND('',#2610,.T.);
#1972=FACE_OUTER_BOUND('',#2611,.T.);
#1973=FACE_OUTER_BOUND('',#2612,.T.);
#1974=FACE_OUTER_BOUND('',#2613,.T.);
#1975=FACE_OUTER_BOUND('',#2614,.T.);
#1976=FACE_OUTER_BOUND('',#2615,.T.);
#1977=FACE_OUTER_BOUND('',#2616,.T.);
#1978=FACE_OUTER_BOUND('',#2617,.T.);
#1979=FACE_OUTER_BOUND('',#2618,.T.);
#1980=FACE_OUTER_BOUND('',#2619,.T.);
#1981=FACE_OUTER_BOUND('',#2620,.T.);
#1982=FACE_OUTER_BOUND('',#2621,.T.);
#1983=FACE_OUTER_BOUND('',#2622,.T.);
#1984=FACE_OUTER_BOUND('',#2623,.T.);
#1985=FACE_OUTER_BOUND('',#2624,.T.);
#1986=FACE_OUTER_BOUND('',#2625,.T.);
#1987=FACE_OUTER_BOUND('',#2626,.T.);
#1988=FACE_OUTER_BOUND('',#2627,.T.);
#1989=FACE_OUTER_BOUND('',#2628,.T.);
#1990=FACE_OUTER_BOUND('',#2629,.T.);
#1991=FACE_OUTER_BOUND('',#2630,.T.);
#1992=FACE_OUTER_BOUND('',#2631,.T.);
#1993=FACE_OUTER_BOUND('',#2632,.T.);
#1994=FACE_OUTER_BOUND('',#2633,.T.);
#1995=FACE_OUTER_BOUND('',#2634,.T.);
#1996=FACE_OUTER_BOUND('',#2635,.T.);
#1997=FACE_OUTER_BOUND('',#2636,.T.);
#1998=FACE_OUTER_BOUND('',#2637,.T.);
#1999=FACE_OUTER_BOUND('',#2638,.T.);
#2000=FACE_OUTER_BOUND('',#2639,.T.);
#2001=FACE_OUTER_BOUND('',#2640,.T.);
#2002=FACE_OUTER_BOUND('',#2641,.T.);
#2003=FACE_OUTER_BOUND('',#2642,.T.);
#2004=FACE_OUTER_BOUND('',#2643,.T.);
#2005=FACE_OUTER_BOUND('',#2644,.T.);
#2006=FACE_OUTER_BOUND('',#2645,.T.);
#2007=FACE_OUTER_BOUND('',#2646,.T.);
#2008=FACE_OUTER_BOUND('',#2647,.T.);
#2009=FACE_OUTER_BOUND('',#2648,.T.);
#2010=FACE_OUTER_BOUND('',#2649,.T.);
#2011=FACE_OUTER_BOUND('',#2650,.T.);
#2012=FACE_OUTER_BOUND('',#2651,.T.);
#2013=FACE_OUTER_BOUND('',#2652,.T.);
#2014=FACE_OUTER_BOUND('',#2653,.T.);
#2015=FACE_OUTER_BOUND('',#2654,.T.);
#2016=FACE_OUTER_BOUND('',#2655,.T.);
#2017=FACE_OUTER_BOUND('',#2656,.T.);
#2018=FACE_OUTER_BOUND('',#2657,.T.);
#2019=FACE_OUTER_BOUND('',#2658,.T.);
#2020=FACE_OUTER_BOUND('',#2659,.T.);
#2021=FACE_OUTER_BOUND('',#2660,.T.);
#2022=FACE_OUTER_BOUND('',#2661,.T.);
#2023=FACE_OUTER_BOUND('',#2662,.T.);
#2024=FACE_OUTER_BOUND('',#2663,.T.);
#2025=FACE_OUTER_BOUND('',#2664,.T.);
#2026=FACE_OUTER_BOUND('',#2665,.T.);
#2027=FACE_OUTER_BOUND('',#2666,.T.);
#2028=FACE_OUTER_BOUND('',#2667,.T.);
#2029=FACE_OUTER_BOUND('',#2668,.T.);
#2030=FACE_OUTER_BOUND('',#2669,.T.);
#2031=FACE_OUTER_BOUND('',#2670,.T.);
#2032=FACE_OUTER_BOUND('',#2671,.T.);
#2033=FACE_OUTER_BOUND('',#2672,.T.);
#2034=FACE_OUTER_BOUND('',#2673,.T.);
#2035=FACE_OUTER_BOUND('',#2674,.T.);
#2036=FACE_OUTER_BOUND('',#2675,.T.);
#2037=FACE_OUTER_BOUND('',#2676,.T.);
#2038=FACE_OUTER_BOUND('',#2677,.T.);
#2039=FACE_OUTER_BOUND('',#2678,.T.);
#2040=FACE_OUTER_BOUND('',#2679,.T.);
#2041=FACE_OUTER_BOUND('',#2680,.T.);
#2042=FACE_OUTER_BOUND('',#2681,.T.);
#2043=FACE_OUTER_BOUND('',#2682,.T.);
#2044=FACE_OUTER_BOUND('',#2683,.T.);
#2045=FACE_OUTER_BOUND('',#2684,.T.);
#2046=FACE_OUTER_BOUND('',#2685,.T.);
#2047=FACE_OUTER_BOUND('',#2686,.T.);
#2048=FACE_OUTER_BOUND('',#2687,.T.);
#2049=FACE_OUTER_BOUND('',#2688,.T.);
#2050=FACE_OUTER_BOUND('',#2689,.T.);
#2051=FACE_OUTER_BOUND('',#2690,.T.);
#2285=EDGE_LOOP('',(#7139,#7140,#7141,#7142,#7143,#7144));
#2286=EDGE_LOOP('',(#7145,#7146,#7147,#7148,#7149,#7150));
#2287=EDGE_LOOP('',(#7151,#7152,#7153,#7154,#7155,#7156));
#2288=EDGE_LOOP('',(#7157,#7158,#7159,#7160,#7161,#7162));
#2289=EDGE_LOOP('',(#7163,#7164,#7165,#7166,#7167,#7168));
#2290=EDGE_LOOP('',(#7169,#7170,#7171,#7172,#7173,#7174));
#2291=EDGE_LOOP('',(#7175,#7176,#7177,#7178,#7179,#7180));
#2292=EDGE_LOOP('',(#7181,#7182,#7183,#7184,#7185,#7186));
#2293=EDGE_LOOP('',(#7187,#7188,#7189,#7190,#7191,#7192));
#2294=EDGE_LOOP('',(#7193,#7194,#7195,#7196,#7197,#7198));
#2295=EDGE_LOOP('',(#7199,#7200,#7201,#7202,#7203,#7204));
#2296=EDGE_LOOP('',(#7205,#7206,#7207,#7208,#7209,#7210));
#2297=EDGE_LOOP('',(#7211,#7212,#7213,#7214,#7215,#7216));
#2298=EDGE_LOOP('',(#7217,#7218,#7219,#7220,#7221,#7222));
#2299=EDGE_LOOP('',(#7223,#7224,#7225,#7226,#7227,#7228));
#2300=EDGE_LOOP('',(#7229,#7230,#7231,#7232,#7233,#7234));
#2301=EDGE_LOOP('',(#7235,#7236,#7237,#7238,#7239,#7240));
#2302=EDGE_LOOP('',(#7241,#7242,#7243,#7244,#7245,#7246));
#2303=EDGE_LOOP('',(#7247,#7248,#7249,#7250,#7251,#7252));
#2304=EDGE_LOOP('',(#7253,#7254,#7255,#7256,#7257,#7258));
#2305=EDGE_LOOP('',(#7259,#7260,#7261,#7262,#7263,#7264));
#2306=EDGE_LOOP('',(#7265,#7266,#7267,#7268,#7269,#7270));
#2307=EDGE_LOOP('',(#7271,#7272,#7273,#7274,#7275,#7276));
#2308=EDGE_LOOP('',(#7277,#7278,#7279,#7280,#7281,#7282));
#2309=EDGE_LOOP('',(#7283,#7284,#7285,#7286,#7287,#7288));
#2310=EDGE_LOOP('',(#7289,#7290,#7291,#7292,#7293,#7294));
#2311=EDGE_LOOP('',(#7295,#7296,#7297,#7298,#7299,#7300));
#2312=EDGE_LOOP('',(#7301,#7302,#7303,#7304,#7305,#7306));
#2313=EDGE_LOOP('',(#7307,#7308,#7309,#7310,#7311,#7312));
#2314=EDGE_LOOP('',(#7313,#7314,#7315,#7316,#7317,#7318));
#2315=EDGE_LOOP('',(#7319,#7320,#7321,#7322,#7323,#7324));
#2316=EDGE_LOOP('',(#7325,#7326,#7327,#7328,#7329,#7330));
#2317=EDGE_LOOP('',(#7331,#7332,#7333,#7334,#7335,#7336));
#2318=EDGE_LOOP('',(#7337,#7338,#7339,#7340,#7341,#7342));
#2319=EDGE_LOOP('',(#7343,#7344,#7345,#7346,#7347,#7348));
#2320=EDGE_LOOP('',(#7349,#7350,#7351,#7352,#7353,#7354));
#2321=EDGE_LOOP('',(#7355,#7356,#7357,#7358,#7359,#7360));
#2322=EDGE_LOOP('',(#7361,#7362,#7363,#7364,#7365,#7366));
#2323=EDGE_LOOP('',(#7367,#7368,#7369,#7370,#7371,#7372));
#2324=EDGE_LOOP('',(#7373,#7374,#7375,#7376,#7377,#7378));
#2325=EDGE_LOOP('',(#7379,#7380,#7381,#7382,#7383,#7384));
#2326=EDGE_LOOP('',(#7385,#7386,#7387,#7388,#7389,#7390));
#2327=EDGE_LOOP('',(#7391,#7392,#7393,#7394,#7395,#7396));
#2328=EDGE_LOOP('',(#7397,#7398,#7399,#7400,#7401,#7402));
#2329=EDGE_LOOP('',(#7403,#7404,#7405,#7406,#7407,#7408,#7409,#7410,#7411,
#7412,#7413,#7414,#7415,#7416,#7417,#7418,#7419,#7420,#7421,#7422,#7423,
#7424,#7425,#7426,#7427,#7428,#7429,#7430,#7431,#7432,#7433,#7434,#7435,
#7436,#7437,#7438,#7439,#7440,#7441,#7442,#7443,#7444,#7445,#7446,#7447,
#7448,#7449,#7450,#7451,#7452,#7453,#7454,#7455,#7456,#7457,#7458,#7459,
#7460,#7461,#7462,#7463,#7464,#7465,#7466,#7467,#7468,#7469,#7470,#7471,
#7472,#7473,#7474,#7475,#7476,#7477,#7478,#7479,#7480,#7481,#7482,#7483,
#7484,#7485,#7486,#7487,#7488,#7489,#7490,#7491,#7492,#7493,#7494,#7495,
#7496,#7497,#7498,#7499,#7500,#7501,#7502,#7503,#7504,#7505,#7506,#7507,
#7508,#7509,#7510,#7511,#7512,#7513,#7514,#7515,#7516,#7517,#7518,#7519,
#7520,#7521,#7522,#7523,#7524,#7525,#7526,#7527,#7528,#7529,#7530,#7531,
#7532,#7533,#7534,#7535,#7536,#7537,#7538,#7539,#7540,#7541,#7542,#7543,
#7544,#7545,#7546,#7547,#7548,#7549,#7550,#7551,#7552,#7553,#7554,#7555,
#7556,#7557,#7558,#7559,#7560,#7561,#7562,#7563,#7564,#7565,#7566,#7567,
#7568,#7569,#7570,#7571,#7572,#7573,#7574,#7575,#7576,#7577,#7578,#7579,
#7580,#7581,#7582));
#2330=EDGE_LOOP('',(#7583,#7584,#7585,#7586));
#2331=EDGE_LOOP('',(#7587,#7588,#7589,#7590,#7591,#7592,#7593,#7594,#7595,
#7596,#7597,#7598,#7599,#7600,#7601,#7602,#7603,#7604,#7605,#7606,#7607,
#7608,#7609,#7610,#7611,#7612,#7613,#7614,#7615,#7616,#7617,#7618,#7619,
#7620,#7621,#7622,#7623,#7624,#7625,#7626,#7627,#7628,#7629,#7630,#7631,
#7632,#7633,#7634,#7635,#7636,#7637,#7638,#7639,#7640,#7641,#7642,#7643,
#7644,#7645,#7646,#7647,#7648,#7649,#7650,#7651,#7652,#7653,#7654,#7655,
#7656,#7657,#7658,#7659,#7660,#7661,#7662,#7663,#7664,#7665,#7666,#7667,
#7668,#7669,#7670,#7671,#7672,#7673,#7674,#7675,#7676,#7677,#7678,#7679,
#7680,#7681,#7682,#7683,#7684,#7685,#7686,#7687,#7688,#7689,#7690,#7691,
#7692,#7693,#7694,#7695,#7696,#7697,#7698,#7699,#7700,#7701,#7702,#7703,
#7704,#7705,#7706,#7707,#7708,#7709,#7710,#7711,#7712,#7713,#7714,#7715,
#7716,#7717,#7718,#7719,#7720,#7721,#7722,#7723,#7724,#7725,#7726,#7727,
#7728,#7729,#7730,#7731,#7732,#7733,#7734,#7735,#7736,#7737,#7738,#7739,
#7740,#7741,#7742,#7743,#7744,#7745,#7746,#7747,#7748,#7749,#7750,#7751,
#7752,#7753,#7754,#7755,#7756,#7757,#7758,#7759,#7760,#7761,#7762,#7763,
#7764,#7765,#7766));
#2332=EDGE_LOOP('',(#7767,#7768,#7769,#7770));
#2333=EDGE_LOOP('',(#7771,#7772,#7773,#7774));
#2334=EDGE_LOOP('',(#7775,#7776,#7777,#7778));
#2335=EDGE_LOOP('',(#7779,#7780,#7781,#7782));
#2336=EDGE_LOOP('',(#7783,#7784,#7785,#7786));
#2337=EDGE_LOOP('',(#7787,#7788,#7789,#7790));
#2338=EDGE_LOOP('',(#7791,#7792,#7793,#7794));
#2339=EDGE_LOOP('',(#7795,#7796,#7797,#7798));
#2340=EDGE_LOOP('',(#7799,#7800,#7801,#7802));
#2341=EDGE_LOOP('',(#7803,#7804,#7805,#7806));
#2342=EDGE_LOOP('',(#7807,#7808,#7809,#7810));
#2343=EDGE_LOOP('',(#7811,#7812,#7813,#7814));
#2344=EDGE_LOOP('',(#7815,#7816,#7817,#7818));
#2345=EDGE_LOOP('',(#7819,#7820,#7821,#7822));
#2346=EDGE_LOOP('',(#7823,#7824,#7825,#7826));
#2347=EDGE_LOOP('',(#7827,#7828,#7829,#7830));
#2348=EDGE_LOOP('',(#7831,#7832,#7833,#7834));
#2349=EDGE_LOOP('',(#7835,#7836,#7837,#7838));
#2350=EDGE_LOOP('',(#7839,#7840,#7841,#7842));
#2351=EDGE_LOOP('',(#7843,#7844,#7845,#7846));
#2352=EDGE_LOOP('',(#7847,#7848,#7849,#7850));
#2353=EDGE_LOOP('',(#7851,#7852,#7853,#7854));
#2354=EDGE_LOOP('',(#7855,#7856,#7857,#7858));
#2355=EDGE_LOOP('',(#7859,#7860,#7861,#7862));
#2356=EDGE_LOOP('',(#7863,#7864,#7865,#7866));
#2357=EDGE_LOOP('',(#7867,#7868,#7869,#7870));
#2358=EDGE_LOOP('',(#7871,#7872,#7873,#7874));
#2359=EDGE_LOOP('',(#7875,#7876,#7877,#7878));
#2360=EDGE_LOOP('',(#7879,#7880,#7881,#7882));
#2361=EDGE_LOOP('',(#7883,#7884,#7885,#7886));
#2362=EDGE_LOOP('',(#7887,#7888,#7889,#7890));
#2363=EDGE_LOOP('',(#7891,#7892,#7893,#7894));
#2364=EDGE_LOOP('',(#7895,#7896,#7897,#7898));
#2365=EDGE_LOOP('',(#7899,#7900,#7901,#7902));
#2366=EDGE_LOOP('',(#7903,#7904,#7905,#7906));
#2367=EDGE_LOOP('',(#7907,#7908,#7909,#7910));
#2368=EDGE_LOOP('',(#7911,#7912,#7913,#7914));
#2369=EDGE_LOOP('',(#7915,#7916,#7917,#7918));
#2370=EDGE_LOOP('',(#7919,#7920,#7921,#7922));
#2371=EDGE_LOOP('',(#7923,#7924,#7925,#7926));
#2372=EDGE_LOOP('',(#7927,#7928,#7929,#7930));
#2373=EDGE_LOOP('',(#7931,#7932,#7933,#7934));
#2374=EDGE_LOOP('',(#7935,#7936,#7937,#7938));
#2375=EDGE_LOOP('',(#7939,#7940,#7941,#7942));
#2376=EDGE_LOOP('',(#7943,#7944,#7945,#7946));
#2377=EDGE_LOOP('',(#7947,#7948,#7949,#7950));
#2378=EDGE_LOOP('',(#7951,#7952,#7953,#7954));
#2379=EDGE_LOOP('',(#7955,#7956,#7957,#7958));
#2380=EDGE_LOOP('',(#7959,#7960,#7961,#7962));
#2381=EDGE_LOOP('',(#7963,#7964,#7965,#7966));
#2382=EDGE_LOOP('',(#7967,#7968,#7969,#7970));
#2383=EDGE_LOOP('',(#7971,#7972,#7973,#7974));
#2384=EDGE_LOOP('',(#7975,#7976,#7977,#7978));
#2385=EDGE_LOOP('',(#7979,#7980,#7981,#7982));
#2386=EDGE_LOOP('',(#7983,#7984,#7985,#7986));
#2387=EDGE_LOOP('',(#7987,#7988,#7989,#7990));
#2388=EDGE_LOOP('',(#7991,#7992,#7993,#7994));
#2389=EDGE_LOOP('',(#7995,#7996,#7997,#7998));
#2390=EDGE_LOOP('',(#7999,#8000,#8001,#8002));
#2391=EDGE_LOOP('',(#8003,#8004,#8005,#8006));
#2392=EDGE_LOOP('',(#8007,#8008,#8009,#8010));
#2393=EDGE_LOOP('',(#8011,#8012,#8013,#8014));
#2394=EDGE_LOOP('',(#8015,#8016,#8017,#8018));
#2395=EDGE_LOOP('',(#8019,#8020,#8021,#8022));
#2396=EDGE_LOOP('',(#8023,#8024,#8025,#8026));
#2397=EDGE_LOOP('',(#8027,#8028,#8029,#8030));
#2398=EDGE_LOOP('',(#8031,#8032,#8033,#8034));
#2399=EDGE_LOOP('',(#8035,#8036,#8037,#8038));
#2400=EDGE_LOOP('',(#8039,#8040,#8041,#8042));
#2401=EDGE_LOOP('',(#8043,#8044,#8045,#8046));
#2402=EDGE_LOOP('',(#8047,#8048,#8049,#8050));
#2403=EDGE_LOOP('',(#8051,#8052,#8053,#8054));
#2404=EDGE_LOOP('',(#8055,#8056,#8057,#8058));
#2405=EDGE_LOOP('',(#8059,#8060,#8061,#8062));
#2406=EDGE_LOOP('',(#8063,#8064,#8065,#8066));
#2407=EDGE_LOOP('',(#8067,#8068,#8069,#8070));
#2408=EDGE_LOOP('',(#8071,#8072,#8073,#8074));
#2409=EDGE_LOOP('',(#8075,#8076,#8077,#8078));
#2410=EDGE_LOOP('',(#8079,#8080,#8081,#8082));
#2411=EDGE_LOOP('',(#8083,#8084,#8085,#8086));
#2412=EDGE_LOOP('',(#8087,#8088,#8089,#8090));
#2413=EDGE_LOOP('',(#8091,#8092,#8093,#8094));
#2414=EDGE_LOOP('',(#8095,#8096,#8097,#8098));
#2415=EDGE_LOOP('',(#8099,#8100,#8101,#8102));
#2416=EDGE_LOOP('',(#8103,#8104,#8105,#8106));
#2417=EDGE_LOOP('',(#8107,#8108,#8109,#8110));
#2418=EDGE_LOOP('',(#8111,#8112,#8113,#8114));
#2419=EDGE_LOOP('',(#8115,#8116,#8117,#8118));
#2420=EDGE_LOOP('',(#8119));
#2421=EDGE_LOOP('',(#8120,#8121,#8122,#8123));
#2422=EDGE_LOOP('',(#8124));
#2423=EDGE_LOOP('',(#8125,#8126,#8127,#8128));
#2424=EDGE_LOOP('',(#8129,#8130,#8131,#8132));
#2425=EDGE_LOOP('',(#8133,#8134,#8135,#8136));
#2426=EDGE_LOOP('',(#8137,#8138,#8139,#8140));
#2427=EDGE_LOOP('',(#8141,#8142,#8143,#8144,#8145));
#2428=EDGE_LOOP('',(#8146,#8147,#8148,#8149,#8150));
#2429=EDGE_LOOP('',(#8151,#8152,#8153,#8154,#8155));
#2430=EDGE_LOOP('',(#8156,#8157,#8158,#8159,#8160));
#2431=EDGE_LOOP('',(#8161,#8162,#8163,#8164,#8165));
#2432=EDGE_LOOP('',(#8166,#8167,#8168,#8169,#8170));
#2433=EDGE_LOOP('',(#8171,#8172,#8173,#8174,#8175));
#2434=EDGE_LOOP('',(#8176,#8177,#8178,#8179,#8180));
#2435=EDGE_LOOP('',(#8181,#8182,#8183,#8184,#8185));
#2436=EDGE_LOOP('',(#8186,#8187,#8188,#8189,#8190));
#2437=EDGE_LOOP('',(#8191,#8192,#8193,#8194,#8195));
#2438=EDGE_LOOP('',(#8196,#8197,#8198,#8199,#8200));
#2439=EDGE_LOOP('',(#8201,#8202,#8203,#8204,#8205));
#2440=EDGE_LOOP('',(#8206,#8207,#8208,#8209,#8210));
#2441=EDGE_LOOP('',(#8211,#8212,#8213,#8214,#8215));
#2442=EDGE_LOOP('',(#8216,#8217,#8218,#8219,#8220));
#2443=EDGE_LOOP('',(#8221,#8222,#8223,#8224,#8225));
#2444=EDGE_LOOP('',(#8226,#8227,#8228,#8229,#8230));
#2445=EDGE_LOOP('',(#8231,#8232,#8233,#8234,#8235));
#2446=EDGE_LOOP('',(#8236,#8237,#8238,#8239,#8240));
#2447=EDGE_LOOP('',(#8241,#8242,#8243,#8244,#8245));
#2448=EDGE_LOOP('',(#8246,#8247,#8248,#8249,#8250));
#2449=EDGE_LOOP('',(#8251,#8252,#8253,#8254,#8255));
#2450=EDGE_LOOP('',(#8256,#8257,#8258,#8259,#8260));
#2451=EDGE_LOOP('',(#8261,#8262,#8263,#8264,#8265));
#2452=EDGE_LOOP('',(#8266,#8267,#8268,#8269,#8270));
#2453=EDGE_LOOP('',(#8271,#8272,#8273,#8274,#8275));
#2454=EDGE_LOOP('',(#8276,#8277,#8278,#8279,#8280));
#2455=EDGE_LOOP('',(#8281,#8282,#8283,#8284,#8285));
#2456=EDGE_LOOP('',(#8286,#8287,#8288,#8289,#8290));
#2457=EDGE_LOOP('',(#8291,#8292,#8293,#8294,#8295));
#2458=EDGE_LOOP('',(#8296,#8297,#8298,#8299,#8300));
#2459=EDGE_LOOP('',(#8301,#8302,#8303,#8304,#8305));
#2460=EDGE_LOOP('',(#8306,#8307,#8308,#8309,#8310));
#2461=EDGE_LOOP('',(#8311,#8312,#8313,#8314,#8315));
#2462=EDGE_LOOP('',(#8316,#8317,#8318,#8319,#8320));
#2463=EDGE_LOOP('',(#8321,#8322,#8323,#8324,#8325));
#2464=EDGE_LOOP('',(#8326,#8327,#8328,#8329,#8330));
#2465=EDGE_LOOP('',(#8331,#8332,#8333,#8334,#8335));
#2466=EDGE_LOOP('',(#8336,#8337,#8338,#8339,#8340));
#2467=EDGE_LOOP('',(#8341,#8342,#8343,#8344,#8345));
#2468=EDGE_LOOP('',(#8346,#8347,#8348,#8349,#8350));
#2469=EDGE_LOOP('',(#8351,#8352,#8353,#8354,#8355));
#2470=EDGE_LOOP('',(#8356,#8357,#8358,#8359,#8360));
#2471=EDGE_LOOP('',(#8361,#8362,#8363,#8364,#8365));
#2472=EDGE_LOOP('',(#8366,#8367,#8368,#8369,#8370));
#2473=EDGE_LOOP('',(#8371,#8372,#8373,#8374,#8375));
#2474=EDGE_LOOP('',(#8376,#8377,#8378,#8379,#8380));
#2475=EDGE_LOOP('',(#8381,#8382,#8383,#8384,#8385));
#2476=EDGE_LOOP('',(#8386,#8387,#8388,#8389,#8390));
#2477=EDGE_LOOP('',(#8391,#8392,#8393,#8394,#8395));
#2478=EDGE_LOOP('',(#8396,#8397,#8398,#8399,#8400));
#2479=EDGE_LOOP('',(#8401,#8402,#8403,#8404,#8405));
#2480=EDGE_LOOP('',(#8406,#8407,#8408,#8409,#8410));
#2481=EDGE_LOOP('',(#8411,#8412,#8413,#8414,#8415));
#2482=EDGE_LOOP('',(#8416,#8417,#8418,#8419,#8420));
#2483=EDGE_LOOP('',(#8421,#8422,#8423,#8424,#8425));
#2484=EDGE_LOOP('',(#8426,#8427,#8428,#8429,#8430));
#2485=EDGE_LOOP('',(#8431,#8432,#8433,#8434,#8435));
#2486=EDGE_LOOP('',(#8436,#8437,#8438,#8439,#8440));
#2487=EDGE_LOOP('',(#8441,#8442,#8443,#8444,#8445));
#2488=EDGE_LOOP('',(#8446,#8447,#8448,#8449,#8450));
#2489=EDGE_LOOP('',(#8451,#8452,#8453,#8454,#8455));
#2490=EDGE_LOOP('',(#8456,#8457,#8458,#8459,#8460));
#2491=EDGE_LOOP('',(#8461,#8462,#8463,#8464,#8465));
#2492=EDGE_LOOP('',(#8466,#8467,#8468,#8469,#8470));
#2493=EDGE_LOOP('',(#8471,#8472,#8473,#8474,#8475));
#2494=EDGE_LOOP('',(#8476,#8477,#8478,#8479,#8480));
#2495=EDGE_LOOP('',(#8481,#8482,#8483,#8484,#8485));
#2496=EDGE_LOOP('',(#8486,#8487,#8488,#8489,#8490));
#2497=EDGE_LOOP('',(#8491,#8492,#8493,#8494,#8495));
#2498=EDGE_LOOP('',(#8496,#8497,#8498,#8499,#8500));
#2499=EDGE_LOOP('',(#8501,#8502,#8503,#8504,#8505));
#2500=EDGE_LOOP('',(#8506,#8507,#8508,#8509,#8510));
#2501=EDGE_LOOP('',(#8511,#8512,#8513,#8514,#8515));
#2502=EDGE_LOOP('',(#8516,#8517,#8518,#8519,#8520));
#2503=EDGE_LOOP('',(#8521,#8522,#8523,#8524,#8525));
#2504=EDGE_LOOP('',(#8526,#8527,#8528,#8529,#8530));
#2505=EDGE_LOOP('',(#8531,#8532,#8533,#8534,#8535));
#2506=EDGE_LOOP('',(#8536,#8537,#8538,#8539,#8540));
#2507=EDGE_LOOP('',(#8541,#8542,#8543,#8544,#8545));
#2508=EDGE_LOOP('',(#8546,#8547,#8548,#8549,#8550));
#2509=EDGE_LOOP('',(#8551,#8552,#8553,#8554,#8555));
#2510=EDGE_LOOP('',(#8556,#8557,#8558,#8559,#8560));
#2511=EDGE_LOOP('',(#8561,#8562,#8563,#8564,#8565));
#2512=EDGE_LOOP('',(#8566,#8567,#8568,#8569,#8570));
#2513=EDGE_LOOP('',(#8571,#8572,#8573,#8574,#8575));
#2514=EDGE_LOOP('',(#8576,#8577,#8578,#8579,#8580));
#2515=EDGE_LOOP('',(#8581,#8582,#8583,#8584,#8585));
#2516=EDGE_LOOP('',(#8586,#8587,#8588,#8589,#8590));
#2517=EDGE_LOOP('',(#8591,#8592,#8593,#8594,#8595));
#2518=EDGE_LOOP('',(#8596,#8597,#8598,#8599,#8600));
#2519=EDGE_LOOP('',(#8601,#8602,#8603,#8604,#8605));
#2520=EDGE_LOOP('',(#8606,#8607,#8608,#8609,#8610));
#2521=EDGE_LOOP('',(#8611,#8612,#8613,#8614,#8615));
#2522=EDGE_LOOP('',(#8616,#8617,#8618,#8619,#8620));
#2523=EDGE_LOOP('',(#8621,#8622,#8623,#8624,#8625));
#2524=EDGE_LOOP('',(#8626,#8627,#8628,#8629,#8630));
#2525=EDGE_LOOP('',(#8631,#8632,#8633,#8634,#8635));
#2526=EDGE_LOOP('',(#8636,#8637,#8638,#8639,#8640));
#2527=EDGE_LOOP('',(#8641,#8642,#8643,#8644,#8645));
#2528=EDGE_LOOP('',(#8646,#8647,#8648,#8649,#8650));
#2529=EDGE_LOOP('',(#8651,#8652,#8653,#8654,#8655));
#2530=EDGE_LOOP('',(#8656,#8657,#8658,#8659,#8660));
#2531=EDGE_LOOP('',(#8661,#8662,#8663,#8664,#8665,#8666));
#2532=EDGE_LOOP('',(#8667,#8668,#8669,#8670,#8671));
#2533=EDGE_LOOP('',(#8672,#8673,#8674,#8675,#8676));
#2534=EDGE_LOOP('',(#8677,#8678,#8679,#8680,#8681));
#2535=EDGE_LOOP('',(#8682,#8683,#8684,#8685,#8686));
#2536=EDGE_LOOP('',(#8687,#8688,#8689,#8690,#8691));
#2537=EDGE_LOOP('',(#8692,#8693,#8694,#8695,#8696));
#2538=EDGE_LOOP('',(#8697,#8698,#8699,#8700,#8701));
#2539=EDGE_LOOP('',(#8702,#8703,#8704,#8705,#8706));
#2540=EDGE_LOOP('',(#8707,#8708,#8709,#8710,#8711));
#2541=EDGE_LOOP('',(#8712,#8713,#8714,#8715,#8716));
#2542=EDGE_LOOP('',(#8717,#8718,#8719,#8720,#8721));
#2543=EDGE_LOOP('',(#8722,#8723,#8724,#8725,#8726));
#2544=EDGE_LOOP('',(#8727,#8728,#8729,#8730,#8731));
#2545=EDGE_LOOP('',(#8732,#8733,#8734,#8735,#8736));
#2546=EDGE_LOOP('',(#8737,#8738,#8739,#8740,#8741));
#2547=EDGE_LOOP('',(#8742,#8743,#8744,#8745,#8746));
#2548=EDGE_LOOP('',(#8747,#8748,#8749,#8750,#8751));
#2549=EDGE_LOOP('',(#8752,#8753,#8754,#8755,#8756));
#2550=EDGE_LOOP('',(#8757,#8758,#8759,#8760,#8761));
#2551=EDGE_LOOP('',(#8762,#8763,#8764,#8765,#8766));
#2552=EDGE_LOOP('',(#8767,#8768,#8769,#8770,#8771));
#2553=EDGE_LOOP('',(#8772,#8773,#8774,#8775,#8776));
#2554=EDGE_LOOP('',(#8777,#8778,#8779,#8780,#8781));
#2555=EDGE_LOOP('',(#8782,#8783,#8784,#8785,#8786));
#2556=EDGE_LOOP('',(#8787,#8788,#8789,#8790,#8791));
#2557=EDGE_LOOP('',(#8792,#8793,#8794,#8795,#8796));
#2558=EDGE_LOOP('',(#8797,#8798,#8799,#8800,#8801));
#2559=EDGE_LOOP('',(#8802,#8803,#8804,#8805,#8806));
#2560=EDGE_LOOP('',(#8807,#8808,#8809,#8810,#8811));
#2561=EDGE_LOOP('',(#8812,#8813,#8814,#8815,#8816));
#2562=EDGE_LOOP('',(#8817,#8818,#8819,#8820,#8821));
#2563=EDGE_LOOP('',(#8822,#8823,#8824,#8825,#8826));
#2564=EDGE_LOOP('',(#8827,#8828,#8829,#8830,#8831));
#2565=EDGE_LOOP('',(#8832,#8833,#8834,#8835,#8836));
#2566=EDGE_LOOP('',(#8837,#8838,#8839,#8840,#8841));
#2567=EDGE_LOOP('',(#8842,#8843,#8844,#8845,#8846));
#2568=EDGE_LOOP('',(#8847,#8848,#8849,#8850,#8851));
#2569=EDGE_LOOP('',(#8852,#8853,#8854,#8855,#8856));
#2570=EDGE_LOOP('',(#8857,#8858,#8859,#8860,#8861));
#2571=EDGE_LOOP('',(#8862,#8863,#8864,#8865,#8866));
#2572=EDGE_LOOP('',(#8867,#8868,#8869,#8870,#8871));
#2573=EDGE_LOOP('',(#8872,#8873,#8874,#8875,#8876));
#2574=EDGE_LOOP('',(#8877,#8878,#8879,#8880,#8881));
#2575=EDGE_LOOP('',(#8882,#8883,#8884,#8885,#8886));
#2576=EDGE_LOOP('',(#8887,#8888,#8889,#8890,#8891));
#2577=EDGE_LOOP('',(#8892,#8893,#8894,#8895,#8896));
#2578=EDGE_LOOP('',(#8897,#8898,#8899,#8900,#8901));
#2579=EDGE_LOOP('',(#8902,#8903,#8904,#8905,#8906));
#2580=EDGE_LOOP('',(#8907,#8908,#8909,#8910,#8911));
#2581=EDGE_LOOP('',(#8912,#8913,#8914,#8915,#8916));
#2582=EDGE_LOOP('',(#8917,#8918,#8919,#8920,#8921));
#2583=EDGE_LOOP('',(#8922,#8923,#8924,#8925,#8926));
#2584=EDGE_LOOP('',(#8927,#8928,#8929,#8930,#8931));
#2585=EDGE_LOOP('',(#8932,#8933,#8934,#8935,#8936));
#2586=EDGE_LOOP('',(#8937,#8938,#8939,#8940,#8941));
#2587=EDGE_LOOP('',(#8942,#8943,#8944,#8945,#8946));
#2588=EDGE_LOOP('',(#8947,#8948,#8949,#8950,#8951));
#2589=EDGE_LOOP('',(#8952,#8953,#8954,#8955,#8956));
#2590=EDGE_LOOP('',(#8957,#8958,#8959,#8960,#8961));
#2591=EDGE_LOOP('',(#8962,#8963,#8964,#8965,#8966));
#2592=EDGE_LOOP('',(#8967,#8968,#8969,#8970,#8971,#8972));
#2593=EDGE_LOOP('',(#8973,#8974,#8975,#8976,#8977));
#2594=EDGE_LOOP('',(#8978,#8979,#8980,#8981,#8982));
#2595=EDGE_LOOP('',(#8983,#8984,#8985,#8986,#8987));
#2596=EDGE_LOOP('',(#8988,#8989,#8990,#8991,#8992));
#2597=EDGE_LOOP('',(#8993,#8994,#8995,#8996,#8997));
#2598=EDGE_LOOP('',(#8998,#8999,#9000,#9001,#9002));
#2599=EDGE_LOOP('',(#9003,#9004,#9005,#9006,#9007));
#2600=EDGE_LOOP('',(#9008,#9009,#9010,#9011,#9012));
#2601=EDGE_LOOP('',(#9013,#9014,#9015,#9016,#9017));
#2602=EDGE_LOOP('',(#9018,#9019,#9020,#9021,#9022));
#2603=EDGE_LOOP('',(#9023,#9024,#9025,#9026,#9027));
#2604=EDGE_LOOP('',(#9028,#9029,#9030,#9031,#9032));
#2605=EDGE_LOOP('',(#9033,#9034,#9035,#9036,#9037));
#2606=EDGE_LOOP('',(#9038,#9039,#9040,#9041,#9042));
#2607=EDGE_LOOP('',(#9043,#9044,#9045,#9046,#9047));
#2608=EDGE_LOOP('',(#9048,#9049,#9050,#9051,#9052));
#2609=EDGE_LOOP('',(#9053,#9054,#9055,#9056,#9057));
#2610=EDGE_LOOP('',(#9058,#9059,#9060,#9061,#9062));
#2611=EDGE_LOOP('',(#9063,#9064,#9065,#9066,#9067));
#2612=EDGE_LOOP('',(#9068,#9069,#9070,#9071,#9072));
#2613=EDGE_LOOP('',(#9073,#9074,#9075,#9076,#9077));
#2614=EDGE_LOOP('',(#9078,#9079,#9080,#9081,#9082));
#2615=EDGE_LOOP('',(#9083,#9084,#9085,#9086,#9087));
#2616=EDGE_LOOP('',(#9088,#9089,#9090,#9091,#9092));
#2617=EDGE_LOOP('',(#9093,#9094,#9095,#9096,#9097));
#2618=EDGE_LOOP('',(#9098,#9099,#9100,#9101,#9102));
#2619=EDGE_LOOP('',(#9103,#9104,#9105,#9106,#9107));
#2620=EDGE_LOOP('',(#9108,#9109,#9110,#9111,#9112));
#2621=EDGE_LOOP('',(#9113,#9114,#9115,#9116,#9117));
#2622=EDGE_LOOP('',(#9118,#9119,#9120,#9121,#9122));
#2623=EDGE_LOOP('',(#9123,#9124,#9125,#9126,#9127));
#2624=EDGE_LOOP('',(#9128,#9129,#9130,#9131,#9132));
#2625=EDGE_LOOP('',(#9133,#9134,#9135,#9136,#9137));
#2626=EDGE_LOOP('',(#9138,#9139,#9140,#9141,#9142));
#2627=EDGE_LOOP('',(#9143,#9144,#9145,#9146,#9147));
#2628=EDGE_LOOP('',(#9148,#9149,#9150,#9151,#9152));
#2629=EDGE_LOOP('',(#9153,#9154,#9155,#9156,#9157));
#2630=EDGE_LOOP('',(#9158,#9159,#9160,#9161,#9162));
#2631=EDGE_LOOP('',(#9163,#9164,#9165,#9166,#9167));
#2632=EDGE_LOOP('',(#9168,#9169,#9170,#9171,#9172));
#2633=EDGE_LOOP('',(#9173,#9174,#9175,#9176,#9177));
#2634=EDGE_LOOP('',(#9178,#9179,#9180,#9181,#9182));
#2635=EDGE_LOOP('',(#9183,#9184,#9185,#9186,#9187));
#2636=EDGE_LOOP('',(#9188,#9189,#9190,#9191,#9192));
#2637=EDGE_LOOP('',(#9193,#9194,#9195,#9196,#9197));
#2638=EDGE_LOOP('',(#9198,#9199,#9200,#9201,#9202));
#2639=EDGE_LOOP('',(#9203,#9204,#9205,#9206,#9207));
#2640=EDGE_LOOP('',(#9208,#9209,#9210,#9211,#9212));
#2641=EDGE_LOOP('',(#9213,#9214,#9215,#9216,#9217));
#2642=EDGE_LOOP('',(#9218,#9219,#9220,#9221,#9222));
#2643=EDGE_LOOP('',(#9223,#9224,#9225,#9226,#9227));
#2644=EDGE_LOOP('',(#9228,#9229,#9230,#9231,#9232));
#2645=EDGE_LOOP('',(#9233,#9234,#9235,#9236,#9237));
#2646=EDGE_LOOP('',(#9238,#9239,#9240,#9241,#9242));
#2647=EDGE_LOOP('',(#9243,#9244,#9245,#9246,#9247));
#2648=EDGE_LOOP('',(#9248,#9249,#9250,#9251,#9252));
#2649=EDGE_LOOP('',(#9253,#9254,#9255,#9256,#9257));
#2650=EDGE_LOOP('',(#9258,#9259,#9260,#9261,#9262));
#2651=EDGE_LOOP('',(#9263,#9264,#9265,#9266,#9267));
#2652=EDGE_LOOP('',(#9268,#9269,#9270,#9271,#9272));
#2653=EDGE_LOOP('',(#9273,#9274,#9275,#9276,#9277));
#2654=EDGE_LOOP('',(#9278,#9279,#9280,#9281,#9282));
#2655=EDGE_LOOP('',(#9283,#9284,#9285,#9286,#9287));
#2656=EDGE_LOOP('',(#9288,#9289,#9290,#9291,#9292));
#2657=EDGE_LOOP('',(#9293,#9294,#9295,#9296,#9297));
#2658=EDGE_LOOP('',(#9298,#9299,#9300,#9301,#9302));
#2659=EDGE_LOOP('',(#9303,#9304,#9305,#9306,#9307));
#2660=EDGE_LOOP('',(#9308,#9309,#9310,#9311,#9312));
#2661=EDGE_LOOP('',(#9313,#9314,#9315,#9316,#9317));
#2662=EDGE_LOOP('',(#9318,#9319,#9320,#9321,#9322));
#2663=EDGE_LOOP('',(#9323,#9324,#9325,#9326,#9327));
#2664=EDGE_LOOP('',(#9328,#9329,#9330,#9331,#9332));
#2665=EDGE_LOOP('',(#9333,#9334,#9335,#9336,#9337));
#2666=EDGE_LOOP('',(#9338,#9339,#9340,#9341,#9342));
#2667=EDGE_LOOP('',(#9343,#9344,#9345,#9346,#9347));
#2668=EDGE_LOOP('',(#9348,#9349,#9350,#9351,#9352));
#2669=EDGE_LOOP('',(#9353,#9354,#9355,#9356,#9357));
#2670=EDGE_LOOP('',(#9358,#9359,#9360,#9361,#9362));
#2671=EDGE_LOOP('',(#9363,#9364,#9365,#9366,#9367));
#2672=EDGE_LOOP('',(#9368,#9369,#9370,#9371,#9372));
#2673=EDGE_LOOP('',(#9373,#9374,#9375,#9376,#9377));
#2674=EDGE_LOOP('',(#9378,#9379,#9380,#9381,#9382));
#2675=EDGE_LOOP('',(#9383,#9384,#9385,#9386,#9387));
#2676=EDGE_LOOP('',(#9388,#9389,#9390,#9391,#9392));
#2677=EDGE_LOOP('',(#9393,#9394,#9395,#9396,#9397));
#2678=EDGE_LOOP('',(#9398,#9399,#9400,#9401,#9402));
#2679=EDGE_LOOP('',(#9403,#9404,#9405,#9406,#9407));
#2680=EDGE_LOOP('',(#9408,#9409,#9410,#9411,#9412));
#2681=EDGE_LOOP('',(#9413,#9414,#9415,#9416,#9417));
#2682=EDGE_LOOP('',(#9418,#9419,#9420,#9421,#9422));
#2683=EDGE_LOOP('',(#9423,#9424,#9425,#9426,#9427));
#2684=EDGE_LOOP('',(#9428,#9429,#9430,#9431,#9432));
#2685=EDGE_LOOP('',(#9433,#9434,#9435,#9436,#9437));
#2686=EDGE_LOOP('',(#9438,#9439,#9440,#9441,#9442));
#2687=EDGE_LOOP('',(#9443,#9444,#9445,#9446,#9447));
#2688=EDGE_LOOP('',(#9448,#9449,#9450,#9451,#9452));
#2689=EDGE_LOOP('',(#9453,#9454,#9455,#9456,#9457));
#2690=EDGE_LOOP('',(#9458,#9459,#9460,#9461,#9462));
#2989=LINE('',#19756,#3290);
#2990=LINE('',#20400,#3291);
#2991=LINE('',#20403,#3292);
#2992=LINE('',#21058,#3293);
#2993=LINE('',#22839,#3294);
#2994=LINE('',#22841,#3295);
#2995=LINE('',#22842,#3296);
#2996=LINE('',#22845,#3297);
#2997=LINE('',#22847,#3298);
#2998=LINE('',#22848,#3299);
#2999=LINE('',#22850,#3300);
#3000=LINE('',#22852,#3301);
#3290=VECTOR('',#12612,41.5);
#3291=VECTOR('',#12663,1000.);
#3292=VECTOR('',#12666,1000.);
#3293=VECTOR('',#12713,43.5);
#3294=VECTOR('',#12938,1000.);
#3295=VECTOR('',#12939,1000.);
#3296=VECTOR('',#12940,1000.);
#3297=VECTOR('',#12943,1000.);
#3298=VECTOR('',#12944,1000.);
#3299=VECTOR('',#12945,1000.);
#3300=VECTOR('',#12948,1000.);
#3301=VECTOR('',#12951,1000.);
#3534=CIRCLE('',#11112,43.5);
#3535=CIRCLE('',#11113,43.5);
#3536=CIRCLE('',#11115,43.5);
#3537=CIRCLE('',#11116,43.5);
#3538=CIRCLE('',#11118,43.5);
#3539=CIRCLE('',#11119,43.5);
#3540=CIRCLE('',#11121,43.5);
#3541=CIRCLE('',#11122,43.5);
#3542=CIRCLE('',#11124,43.5);
#3543=CIRCLE('',#11125,43.5);
#3544=CIRCLE('',#11127,43.5);
#3545=CIRCLE('',#11128,43.5);
#3546=CIRCLE('',#11130,43.5);
#3547=CIRCLE('',#11131,43.5);
#3548=CIRCLE('',#11133,43.5);
#3549=CIRCLE('',#11134,43.5);
#3550=CIRCLE('',#11136,43.5);
#3551=CIRCLE('',#11137,43.5);
#3552=CIRCLE('',#11139,43.5);
#3553=CIRCLE('',#11140,43.5);
#3554=CIRCLE('',#11142,43.5);
#3555=CIRCLE('',#11143,43.5);
#3556=CIRCLE('',#11145,43.5);
#3557=CIRCLE('',#11146,43.5);
#3558=CIRCLE('',#11148,43.5);
#3559=CIRCLE('',#11149,43.5);
#3560=CIRCLE('',#11151,43.5);
#3561=CIRCLE('',#11152,43.5);
#3562=CIRCLE('',#11154,43.5);
#3563=CIRCLE('',#11155,43.5);
#3564=CIRCLE('',#11157,43.5);
#3565=CIRCLE('',#11158,43.5);
#3566=CIRCLE('',#11160,43.5);
#3567=CIRCLE('',#11161,43.5);
#3568=CIRCLE('',#11163,43.5);
#3569=CIRCLE('',#11164,43.5);
#3570=CIRCLE('',#11166,43.5);
#3571=CIRCLE('',#11167,43.5);
#3572=CIRCLE('',#11169,43.5);
#3573=CIRCLE('',#11170,43.5);
#3574=CIRCLE('',#11172,43.5);
#3575=CIRCLE('',#11173,43.5);
#3576=CIRCLE('',#11175,43.5);
#3577=CIRCLE('',#11176,43.5);
#3578=CIRCLE('',#11178,43.5);
#3579=CIRCLE('',#11179,43.5);
#3580=CIRCLE('',#11181,43.5);
#3581=CIRCLE('',#11182,43.5);
#3582=CIRCLE('',#11184,43.5);
#3583=CIRCLE('',#11185,43.5);
#3584=CIRCLE('',#11187,43.5);
#3585=CIRCLE('',#11188,43.5);
#3586=CIRCLE('',#11190,43.5);
#3587=CIRCLE('',#11191,43.5);
#3588=CIRCLE('',#11193,43.5);
#3589=CIRCLE('',#11194,43.5);
#3590=CIRCLE('',#11196,43.5);
#3591=CIRCLE('',#11197,43.5);
#3592=CIRCLE('',#11199,43.5);
#3593=CIRCLE('',#11200,43.5);
#3594=CIRCLE('',#11202,43.5);
#3595=CIRCLE('',#11203,43.5);
#3596=CIRCLE('',#11205,43.5);
#3597=CIRCLE('',#11206,43.5);
#3598=CIRCLE('',#11208,43.5);
#3599=CIRCLE('',#11209,43.5);
#3600=CIRCLE('',#11211,43.5);
#3601=CIRCLE('',#11212,43.5);
#3602=CIRCLE('',#11214,43.5);
#3603=CIRCLE('',#11215,43.5);
#3604=CIRCLE('',#11217,43.5);
#3605=CIRCLE('',#11218,43.5);
#3606=CIRCLE('',#11220,43.5);
#3607=CIRCLE('',#11221,43.5);
#3608=CIRCLE('',#11223,43.5);
#3609=CIRCLE('',#11224,43.5);
#3610=CIRCLE('',#11226,43.5);
#3611=CIRCLE('',#11227,43.5);
#3612=CIRCLE('',#11229,43.5);
#3613=CIRCLE('',#11230,43.5);
#3614=CIRCLE('',#11232,43.5);
#3615=CIRCLE('',#11233,43.5);
#3616=CIRCLE('',#11235,43.5);
#3617=CIRCLE('',#11236,43.5);
#3618=CIRCLE('',#11238,43.5);
#3619=CIRCLE('',#11239,43.5);
#3620=CIRCLE('',#11241,43.5);
#3621=CIRCLE('',#11242,43.5);
#3622=CIRCLE('',#11244,43.5);
#3623=CIRCLE('',#11245,43.5);
#3624=CIRCLE('',#11246,43.5);
#3625=CIRCLE('',#11247,43.5);
#3626=CIRCLE('',#11248,43.5);
#3627=CIRCLE('',#11249,43.5);
#3628=CIRCLE('',#11250,43.5);
#3629=CIRCLE('',#11251,43.5);
#3630=CIRCLE('',#11252,43.5);
#3631=CIRCLE('',#11253,43.5);
#3632=CIRCLE('',#11254,43.5);
#3633=CIRCLE('',#11255,43.5);
#3634=CIRCLE('',#11256,43.5);
#3635=CIRCLE('',#11257,43.5);
#3636=CIRCLE('',#11258,43.5);
#3637=CIRCLE('',#11259,43.5);
#3638=CIRCLE('',#11260,43.5);
#3639=CIRCLE('',#11261,43.5);
#3640=CIRCLE('',#11262,43.5);
#3641=CIRCLE('',#11263,43.5);
#3642=CIRCLE('',#11264,43.5);
#3643=CIRCLE('',#11265,43.5);
#3644=CIRCLE('',#11266,41.5);
#3645=CIRCLE('',#11267,43.5);
#3646=CIRCLE('',#11268,43.5);
#3647=CIRCLE('',#11269,43.5);
#3648=CIRCLE('',#11270,43.5);
#3649=CIRCLE('',#11271,43.5);
#3650=CIRCLE('',#11272,43.5);
#3651=CIRCLE('',#11273,43.5);
#3652=CIRCLE('',#11274,43.5);
#3653=CIRCLE('',#11275,43.5);
#3654=CIRCLE('',#11276,43.5);
#3655=CIRCLE('',#11277,43.5);
#3656=CIRCLE('',#11278,43.5);
#3657=CIRCLE('',#11279,43.5);
#3658=CIRCLE('',#11280,43.5);
#3659=CIRCLE('',#11281,43.5);
#3660=CIRCLE('',#11282,43.5);
#3661=CIRCLE('',#11283,43.5);
#3662=CIRCLE('',#11284,43.5);
#3663=CIRCLE('',#11285,43.5);
#3664=CIRCLE('',#11286,43.5);
#3665=CIRCLE('',#11287,43.5);
#3666=CIRCLE('',#11288,43.5);
#3667=CIRCLE('',#11290,15.);
#3668=CIRCLE('',#11291,15.);
#3669=CIRCLE('',#11293,43.5);
#3670=CIRCLE('',#11294,43.5);
#3671=CIRCLE('',#11295,43.5);
#3672=CIRCLE('',#11296,43.5);
#3673=CIRCLE('',#11297,43.5);
#3674=CIRCLE('',#11298,43.5);
#3675=CIRCLE('',#11299,43.5);
#3676=CIRCLE('',#11300,43.5);
#3677=CIRCLE('',#11301,43.5);
#3678=CIRCLE('',#11302,43.5);
#3679=CIRCLE('',#11303,43.5);
#3680=CIRCLE('',#11304,43.5);
#3681=CIRCLE('',#11305,43.5);
#3682=CIRCLE('',#11306,43.5);
#3683=CIRCLE('',#11307,43.5);
#3684=CIRCLE('',#11308,43.5);
#3685=CIRCLE('',#11309,43.5);
#3686=CIRCLE('',#11310,43.5);
#3687=CIRCLE('',#11311,43.5);
#3688=CIRCLE('',#11312,43.5);
#3689=CIRCLE('',#11313,43.5);
#3690=CIRCLE('',#11314,43.5);
#3691=CIRCLE('',#11315,41.5);
#3692=CIRCLE('',#11316,43.5);
#3693=CIRCLE('',#11317,43.5);
#3694=CIRCLE('',#11318,43.5);
#3695=CIRCLE('',#11319,43.5);
#3696=CIRCLE('',#11320,43.5);
#3697=CIRCLE('',#11321,43.5);
#3698=CIRCLE('',#11322,43.5);
#3699=CIRCLE('',#11323,43.5);
#3700=CIRCLE('',#11324,43.5);
#3701=CIRCLE('',#11325,43.5);
#3702=CIRCLE('',#11326,43.5);
#3703=CIRCLE('',#11327,43.5);
#3704=CIRCLE('',#11328,43.5);
#3705=CIRCLE('',#11329,43.5);
#3706=CIRCLE('',#11330,43.5);
#3707=CIRCLE('',#11331,43.5);
#3708=CIRCLE('',#11332,43.5);
#3709=CIRCLE('',#11333,43.5);
#3710=CIRCLE('',#11334,43.5);
#3711=CIRCLE('',#11335,43.5);
#3712=CIRCLE('',#11336,43.5);
#3713=CIRCLE('',#11337,43.5);
#3714=CIRCLE('',#11431,1.8);
#3715=CIRCLE('',#11432,1.8);
#3716=CIRCLE('',#11433,18.);
#3717=CIRCLE('',#11434,18.);
#3718=CIRCLE('',#11435,18.);
#3719=CIRCLE('',#11436,18.);
#3720=CIRCLE('',#11437,1.8);
#3721=CIRCLE('',#11438,1.8);
#3722=CIRCLE('',#11439,18.);
#3723=CIRCLE('',#11440,18.);
#3724=CIRCLE('',#11441,1.8);
#3725=CIRCLE('',#11442,1.8);
#3726=CIRCLE('',#11443,18.);
#3727=CIRCLE('',#11444,18.);
#3728=CIRCLE('',#11445,1.8);
#3729=CIRCLE('',#11446,1.8);
#3730=CIRCLE('',#11447,18.);
#3731=CIRCLE('',#11448,18.);
#3732=CIRCLE('',#11449,1.8);
#3733=CIRCLE('',#11450,1.8);
#3734=CIRCLE('',#11451,18.);
#3735=CIRCLE('',#11452,18.);
#3736=CIRCLE('',#11453,1.8);
#3737=CIRCLE('',#11454,1.8);
#3738=CIRCLE('',#11455,18.);
#3739=CIRCLE('',#11456,18.);
#3740=CIRCLE('',#11457,1.8);
#3741=CIRCLE('',#11458,1.8);
#3742=CIRCLE('',#11459,18.);
#3743=CIRCLE('',#11460,18.);
#3744=CIRCLE('',#11461,1.8);
#3745=CIRCLE('',#11462,1.8);
#3746=CIRCLE('',#11463,18.);
#3747=CIRCLE('',#11464,18.);
#3748=CIRCLE('',#11465,1.8);
#3749=CIRCLE('',#11466,1.8);
#3750=CIRCLE('',#11467,18.);
#3751=CIRCLE('',#11468,18.);
#3752=CIRCLE('',#11469,1.8);
#3753=CIRCLE('',#11470,1.8);
#3754=CIRCLE('',#11471,18.);
#3755=CIRCLE('',#11472,18.);
#3756=CIRCLE('',#11473,1.8);
#3757=CIRCLE('',#11474,1.8);
#3758=CIRCLE('',#11475,18.);
#3759=CIRCLE('',#11476,18.);
#3760=CIRCLE('',#11477,1.8);
#3761=CIRCLE('',#11478,1.8);
#3762=CIRCLE('',#11479,18.);
#3763=CIRCLE('',#11480,18.);
#3764=CIRCLE('',#11481,1.8);
#3765=CIRCLE('',#11482,1.8);
#3766=CIRCLE('',#11483,18.);
#3767=CIRCLE('',#11484,18.);
#3768=CIRCLE('',#11485,1.8);
#3769=CIRCLE('',#11486,1.8);
#3770=CIRCLE('',#11487,18.);
#3771=CIRCLE('',#11488,18.);
#3772=CIRCLE('',#11489,1.8);
#3773=CIRCLE('',#11490,1.8);
#3774=CIRCLE('',#11491,18.);
#3775=CIRCLE('',#11492,17.9999999999999);
#3776=CIRCLE('',#11493,1.80000000000001);
#3777=CIRCLE('',#11494,1.80000000000001);
#3778=CIRCLE('',#11495,18.);
#3779=CIRCLE('',#11496,18.);
#3780=CIRCLE('',#11497,1.8);
#3781=CIRCLE('',#11498,1.8);
#3782=CIRCLE('',#11499,18.);
#3783=CIRCLE('',#11500,18.);
#3784=CIRCLE('',#11501,1.8);
#3785=CIRCLE('',#11502,1.8);
#3786=CIRCLE('',#11503,18.);
#3787=CIRCLE('',#11504,18.);
#3788=CIRCLE('',#11505,1.8);
#3789=CIRCLE('',#11506,1.8);
#3790=CIRCLE('',#11507,18.);
#3791=CIRCLE('',#11508,18.);
#3792=CIRCLE('',#11509,1.8);
#3793=CIRCLE('',#11510,1.8);
#3794=CIRCLE('',#11511,18.);
#3795=CIRCLE('',#11512,18.);
#3796=CIRCLE('',#11513,1.8);
#3797=CIRCLE('',#11514,1.8);
#3798=CIRCLE('',#11515,18.);
#3799=CIRCLE('',#11516,18.);
#3800=CIRCLE('',#11517,1.8);
#3801=CIRCLE('',#11518,1.8);
#3802=CIRCLE('',#11519,18.);
#3803=CIRCLE('',#11520,18.);
#3804=CIRCLE('',#11521,1.8);
#3805=CIRCLE('',#11522,1.8);
#3806=CIRCLE('',#11523,18.);
#3807=CIRCLE('',#11524,18.);
#3808=CIRCLE('',#11525,1.8);
#3809=CIRCLE('',#11526,1.8);
#3810=CIRCLE('',#11527,18.);
#3811=CIRCLE('',#11528,18.);
#3812=CIRCLE('',#11529,1.8);
#3813=CIRCLE('',#11530,1.8);
#3814=CIRCLE('',#11531,18.);
#3815=CIRCLE('',#11532,18.);
#3816=CIRCLE('',#11533,1.8);
#3817=CIRCLE('',#11534,1.8);
#3818=CIRCLE('',#11535,18.);
#3819=CIRCLE('',#11536,18.);
#3820=CIRCLE('',#11537,1.8);
#3821=CIRCLE('',#11538,1.8);
#3822=CIRCLE('',#11539,18.);
#3823=CIRCLE('',#11540,18.);
#3824=CIRCLE('',#11541,1.8);
#3825=CIRCLE('',#11542,1.8);
#3826=CIRCLE('',#11543,18.);
#3827=CIRCLE('',#11544,18.);
#3828=CIRCLE('',#11545,1.8);
#3829=CIRCLE('',#11546,1.8);
#3830=CIRCLE('',#11547,18.);
#3831=CIRCLE('',#11548,18.);
#3832=CIRCLE('',#11549,1.8);
#3833=CIRCLE('',#11550,1.8);
#3834=CIRCLE('',#11551,18.);
#3835=CIRCLE('',#11552,18.);
#3836=CIRCLE('',#11553,1.8);
#3837=CIRCLE('',#11554,1.8);
#3838=CIRCLE('',#11555,18.);
#3839=CIRCLE('',#11556,18.);
#3840=CIRCLE('',#11557,1.8);
#3841=CIRCLE('',#11558,1.8);
#3842=CIRCLE('',#11559,18.);
#3843=CIRCLE('',#11560,18.);
#3844=CIRCLE('',#11561,1.8);
#3845=CIRCLE('',#11562,1.8);
#3846=CIRCLE('',#11563,18.);
#3847=CIRCLE('',#11564,18.);
#3848=CIRCLE('',#11565,1.8);
#3849=CIRCLE('',#11566,1.8);
#3850=CIRCLE('',#11567,18.);
#3851=CIRCLE('',#11568,18.);
#3852=CIRCLE('',#11569,1.8);
#3853=CIRCLE('',#11570,1.8);
#3854=CIRCLE('',#11571,18.);
#3855=CIRCLE('',#11572,18.);
#3856=CIRCLE('',#11573,1.8);
#3857=CIRCLE('',#11574,1.8);
#3858=CIRCLE('',#11575,18.);
#3859=CIRCLE('',#11576,18.);
#3860=CIRCLE('',#11577,1.8);
#3861=CIRCLE('',#11578,1.8);
#3862=CIRCLE('',#11579,17.9999999999999);
#3863=CIRCLE('',#11580,18.);
#3864=CIRCLE('',#11581,1.8);
#3865=CIRCLE('',#11582,1.8);
#3866=CIRCLE('',#11583,18.);
#3867=CIRCLE('',#11584,18.);
#3868=CIRCLE('',#11585,1.8);
#3869=CIRCLE('',#11586,1.8);
#3870=CIRCLE('',#11587,18.);
#3871=CIRCLE('',#11588,18.);
#3872=CIRCLE('',#11589,1.8);
#3873=CIRCLE('',#11590,1.8);
#3874=CIRCLE('',#11591,18.);
#3875=CIRCLE('',#11592,18.);
#3876=CIRCLE('',#11593,1.8);
#3877=CIRCLE('',#11594,1.8);
#3878=CIRCLE('',#11595,18.);
#3879=CIRCLE('',#11596,18.);
#3880=CIRCLE('',#11597,1.8);
#3881=CIRCLE('',#11598,1.8);
#3882=CIRCLE('',#11599,18.);
#3883=CIRCLE('',#11600,18.);
#3884=CIRCLE('',#11601,1.8);
#3885=CIRCLE('',#11602,1.8);
#3886=CIRCLE('',#11603,18.);
#3887=CIRCLE('',#11604,18.);
#3888=CIRCLE('',#11605,1.8);
#3889=CIRCLE('',#11606,1.8);
#4134=VERTEX_POINT('',#17303);
#4135=VERTEX_POINT('',#17304);
#4136=VERTEX_POINT('',#17311);
#4137=VERTEX_POINT('',#17318);
#4138=VERTEX_POINT('',#17320);
#4139=VERTEX_POINT('',#17335);
#4140=VERTEX_POINT('',#17344);
#4141=VERTEX_POINT('',#17345);
#4142=VERTEX_POINT('',#17352);
#4143=VERTEX_POINT('',#17359);
#4144=VERTEX_POINT('',#17361);
#4145=VERTEX_POINT('',#17376);
#4146=VERTEX_POINT('',#17385);
#4147=VERTEX_POINT('',#17386);
#4148=VERTEX_POINT('',#17393);
#4149=VERTEX_POINT('',#17406);
#4150=VERTEX_POINT('',#17408);
#4151=VERTEX_POINT('',#17423);
#4152=VERTEX_POINT('',#17432);
#4153=VERTEX_POINT('',#17433);
#4154=VERTEX_POINT('',#17440);
#4155=VERTEX_POINT('',#17447);
#4156=VERTEX_POINT('',#17449);
#4157=VERTEX_POINT('',#17458);
#4158=VERTEX_POINT('',#17467);
#4159=VERTEX_POINT('',#17468);
#4160=VERTEX_POINT('',#17475);
#4161=VERTEX_POINT('',#17482);
#4162=VERTEX_POINT('',#17484);
#4163=VERTEX_POINT('',#17499);
#4164=VERTEX_POINT('',#17508);
#4165=VERTEX_POINT('',#17509);
#4166=VERTEX_POINT('',#17516);
#4167=VERTEX_POINT('',#17523);
#4168=VERTEX_POINT('',#17525);
#4169=VERTEX_POINT('',#17540);
#4170=VERTEX_POINT('',#17549);
#4171=VERTEX_POINT('',#17550);
#4172=VERTEX_POINT('',#17557);
#4173=VERTEX_POINT('',#17564);
#4174=VERTEX_POINT('',#17566);
#4175=VERTEX_POINT('',#17581);
#4176=VERTEX_POINT('',#17590);
#4177=VERTEX_POINT('',#17591);
#4178=VERTEX_POINT('',#17598);
#4179=VERTEX_POINT('',#17605);
#4180=VERTEX_POINT('',#17607);
#4181=VERTEX_POINT('',#17622);
#4182=VERTEX_POINT('',#17631);
#4183=VERTEX_POINT('',#17632);
#4184=VERTEX_POINT('',#17639);
#4185=VERTEX_POINT('',#17646);
#4186=VERTEX_POINT('',#17648);
#4187=VERTEX_POINT('',#17663);
#4188=VERTEX_POINT('',#17672);
#4189=VERTEX_POINT('',#17673);
#4190=VERTEX_POINT('',#17680);
#4191=VERTEX_POINT('',#17687);
#4192=VERTEX_POINT('',#17689);
#4193=VERTEX_POINT('',#17704);
#4194=VERTEX_POINT('',#17713);
#4195=VERTEX_POINT('',#17714);
#4196=VERTEX_POINT('',#17721);
#4197=VERTEX_POINT('',#17728);
#4198=VERTEX_POINT('',#17730);
#4199=VERTEX_POINT('',#17745);
#4200=VERTEX_POINT('',#17754);
#4201=VERTEX_POINT('',#17755);
#4202=VERTEX_POINT('',#17762);
#4203=VERTEX_POINT('',#17775);
#4204=VERTEX_POINT('',#17777);
#4205=VERTEX_POINT('',#17792);
#4206=VERTEX_POINT('',#17801);
#4207=VERTEX_POINT('',#17802);
#4208=VERTEX_POINT('',#17809);
#4209=VERTEX_POINT('',#17816);
#4210=VERTEX_POINT('',#17818);
#4211=VERTEX_POINT('',#17827);
#4212=VERTEX_POINT('',#17836);
#4213=VERTEX_POINT('',#17837);
#4214=VERTEX_POINT('',#17844);
#4215=VERTEX_POINT('',#17851);
#4216=VERTEX_POINT('',#17853);
#4217=VERTEX_POINT('',#17868);
#4218=VERTEX_POINT('',#17877);
#4219=VERTEX_POINT('',#17878);
#4220=VERTEX_POINT('',#17885);
#4221=VERTEX_POINT('',#17892);
#4222=VERTEX_POINT('',#17894);
#4223=VERTEX_POINT('',#17909);
#4224=VERTEX_POINT('',#17918);
#4225=VERTEX_POINT('',#17919);
#4226=VERTEX_POINT('',#17926);
#4227=VERTEX_POINT('',#17933);
#4228=VERTEX_POINT('',#17935);
#4229=VERTEX_POINT('',#17950);
#4230=VERTEX_POINT('',#17959);
#4231=VERTEX_POINT('',#17960);
#4232=VERTEX_POINT('',#17967);
#4233=VERTEX_POINT('',#17974);
#4234=VERTEX_POINT('',#17976);
#4235=VERTEX_POINT('',#17991);
#4236=VERTEX_POINT('',#18000);
#4237=VERTEX_POINT('',#18001);
#4238=VERTEX_POINT('',#18008);
#4239=VERTEX_POINT('',#18015);
#4240=VERTEX_POINT('',#18017);
#4241=VERTEX_POINT('',#18032);
#4242=VERTEX_POINT('',#18041);
#4243=VERTEX_POINT('',#18042);
#4244=VERTEX_POINT('',#18049);
#4245=VERTEX_POINT('',#18056);
#4246=VERTEX_POINT('',#18058);
#4247=VERTEX_POINT('',#18073);
#4248=VERTEX_POINT('',#18082);
#4249=VERTEX_POINT('',#18083);
#4250=VERTEX_POINT('',#18090);
#4251=VERTEX_POINT('',#18097);
#4252=VERTEX_POINT('',#18099);
#4253=VERTEX_POINT('',#18114);
#4254=VERTEX_POINT('',#18123);
#4255=VERTEX_POINT('',#18124);
#4256=VERTEX_POINT('',#18131);
#4257=VERTEX_POINT('',#18138);
#4258=VERTEX_POINT('',#18140);
#4259=VERTEX_POINT('',#18155);
#4260=VERTEX_POINT('',#18164);
#4261=VERTEX_POINT('',#18165);
#4262=VERTEX_POINT('',#18172);
#4263=VERTEX_POINT('',#18179);
#4264=VERTEX_POINT('',#18181);
#4265=VERTEX_POINT('',#18196);
#4266=VERTEX_POINT('',#18205);
#4267=VERTEX_POINT('',#18206);
#4268=VERTEX_POINT('',#18213);
#4269=VERTEX_POINT('',#18220);
#4270=VERTEX_POINT('',#18222);
#4271=VERTEX_POINT('',#18237);
#4272=VERTEX_POINT('',#18246);
#4273=VERTEX_POINT('',#18247);
#4274=VERTEX_POINT('',#18254);
#4275=VERTEX_POINT('',#18261);
#4276=VERTEX_POINT('',#18263);
#4277=VERTEX_POINT('',#18278);
#4278=VERTEX_POINT('',#18287);
#4279=VERTEX_POINT('',#18288);
#4280=VERTEX_POINT('',#18295);
#4281=VERTEX_POINT('',#18308);
#4282=VERTEX_POINT('',#18310);
#4283=VERTEX_POINT('',#18325);
#4284=VERTEX_POINT('',#18334);
#4285=VERTEX_POINT('',#18335);
#4286=VERTEX_POINT('',#18342);
#4287=VERTEX_POINT('',#18355);
#4288=VERTEX_POINT('',#18357);
#4289=VERTEX_POINT('',#18366);
#4290=VERTEX_POINT('',#18375);
#4291=VERTEX_POINT('',#18376);
#4292=VERTEX_POINT('',#18383);
#4293=VERTEX_POINT('',#18390);
#4294=VERTEX_POINT('',#18392);
#4295=VERTEX_POINT('',#18401);
#4296=VERTEX_POINT('',#18410);
#4297=VERTEX_POINT('',#18411);
#4298=VERTEX_POINT('',#18418);
#4299=VERTEX_POINT('',#18425);
#4300=VERTEX_POINT('',#18427);
#4301=VERTEX_POINT('',#18442);
#4302=VERTEX_POINT('',#18451);
#4303=VERTEX_POINT('',#18452);
#4304=VERTEX_POINT('',#18459);
#4305=VERTEX_POINT('',#18466);
#4306=VERTEX_POINT('',#18468);
#4307=VERTEX_POINT('',#18483);
#4308=VERTEX_POINT('',#18492);
#4309=VERTEX_POINT('',#18493);
#4310=VERTEX_POINT('',#18500);
#4311=VERTEX_POINT('',#18507);
#4312=VERTEX_POINT('',#18509);
#4313=VERTEX_POINT('',#18524);
#4314=VERTEX_POINT('',#18533);
#4315=VERTEX_POINT('',#18534);
#4316=VERTEX_POINT('',#18541);
#4317=VERTEX_POINT('',#18548);
#4318=VERTEX_POINT('',#18550);
#4319=VERTEX_POINT('',#18565);
#4320=VERTEX_POINT('',#18574);
#4321=VERTEX_POINT('',#18575);
#4322=VERTEX_POINT('',#18582);
#4323=VERTEX_POINT('',#18589);
#4324=VERTEX_POINT('',#18591);
#4325=VERTEX_POINT('',#18606);
#4326=VERTEX_POINT('',#18615);
#4327=VERTEX_POINT('',#18616);
#4328=VERTEX_POINT('',#18623);
#4329=VERTEX_POINT('',#18636);
#4330=VERTEX_POINT('',#18638);
#4331=VERTEX_POINT('',#18653);
#4332=VERTEX_POINT('',#18662);
#4333=VERTEX_POINT('',#18663);
#4334=VERTEX_POINT('',#18670);
#4335=VERTEX_POINT('',#18683);
#4336=VERTEX_POINT('',#18685);
#4337=VERTEX_POINT('',#18694);
#4338=VERTEX_POINT('',#18703);
#4339=VERTEX_POINT('',#18704);
#4340=VERTEX_POINT('',#18711);
#4341=VERTEX_POINT('',#18718);
#4342=VERTEX_POINT('',#18720);
#4343=VERTEX_POINT('',#18729);
#4344=VERTEX_POINT('',#18738);
#4345=VERTEX_POINT('',#18739);
#4346=VERTEX_POINT('',#18746);
#4347=VERTEX_POINT('',#18753);
#4348=VERTEX_POINT('',#18755);
#4349=VERTEX_POINT('',#18770);
#4350=VERTEX_POINT('',#18779);
#4351=VERTEX_POINT('',#18780);
#4352=VERTEX_POINT('',#18787);
#4353=VERTEX_POINT('',#18794);
#4354=VERTEX_POINT('',#18796);
#4355=VERTEX_POINT('',#18811);
#4356=VERTEX_POINT('',#18820);
#4357=VERTEX_POINT('',#18821);
#4358=VERTEX_POINT('',#18828);
#4359=VERTEX_POINT('',#18835);
#4360=VERTEX_POINT('',#18837);
#4361=VERTEX_POINT('',#18852);
#4362=VERTEX_POINT('',#18861);
#4363=VERTEX_POINT('',#18862);
#4364=VERTEX_POINT('',#18869);
#4365=VERTEX_POINT('',#18876);
#4366=VERTEX_POINT('',#18878);
#4367=VERTEX_POINT('',#18893);
#4368=VERTEX_POINT('',#18902);
#4369=VERTEX_POINT('',#18903);
#4370=VERTEX_POINT('',#18910);
#4371=VERTEX_POINT('',#18917);
#4372=VERTEX_POINT('',#18919);
#4373=VERTEX_POINT('',#18934);
#4374=VERTEX_POINT('',#18943);
#4375=VERTEX_POINT('',#18944);
#4376=VERTEX_POINT('',#18951);
#4377=VERTEX_POINT('',#18958);
#4378=VERTEX_POINT('',#18960);
#4379=VERTEX_POINT('',#18975);
#4380=VERTEX_POINT('',#18984);
#4381=VERTEX_POINT('',#18985);
#4382=VERTEX_POINT('',#18992);
#4383=VERTEX_POINT('',#18999);
#4384=VERTEX_POINT('',#19001);
#4385=VERTEX_POINT('',#19016);
#4386=VERTEX_POINT('',#19025);
#4387=VERTEX_POINT('',#19026);
#4388=VERTEX_POINT('',#19033);
#4389=VERTEX_POINT('',#19040);
#4390=VERTEX_POINT('',#19042);
#4391=VERTEX_POINT('',#19051);
#4392=VERTEX_POINT('',#19060);
#4393=VERTEX_POINT('',#19061);
#4394=VERTEX_POINT('',#19068);
#4395=VERTEX_POINT('',#19081);
#4396=VERTEX_POINT('',#19083);
#4397=VERTEX_POINT('',#19098);
#4398=VERTEX_POINT('',#19107);
#4399=VERTEX_POINT('',#19108);
#4400=VERTEX_POINT('',#19121);
#4401=VERTEX_POINT('',#19129);
#4402=VERTEX_POINT('',#19131);
#4403=VERTEX_POINT('',#19139);
#4404=VERTEX_POINT('',#19150);
#4405=VERTEX_POINT('',#19158);
#4406=VERTEX_POINT('',#19160);
#4407=VERTEX_POINT('',#19168);
#4408=VERTEX_POINT('',#19179);
#4409=VERTEX_POINT('',#19187);
#4410=VERTEX_POINT('',#19189);
#4411=VERTEX_POINT('',#19197);
#4412=VERTEX_POINT('',#19208);
#4413=VERTEX_POINT('',#19216);
#4414=VERTEX_POINT('',#19218);
#4415=VERTEX_POINT('',#19226);
#4416=VERTEX_POINT('',#19237);
#4417=VERTEX_POINT('',#19245);
#4418=VERTEX_POINT('',#19247);
#4419=VERTEX_POINT('',#19255);
#4420=VERTEX_POINT('',#19266);
#4421=VERTEX_POINT('',#19274);
#4422=VERTEX_POINT('',#19276);
#4423=VERTEX_POINT('',#19284);
#4424=VERTEX_POINT('',#19295);
#4425=VERTEX_POINT('',#19303);
#4426=VERTEX_POINT('',#19305);
#4427=VERTEX_POINT('',#19313);
#4428=VERTEX_POINT('',#19324);
#4429=VERTEX_POINT('',#19332);
#4430=VERTEX_POINT('',#19334);
#4431=VERTEX_POINT('',#19342);
#4432=VERTEX_POINT('',#19353);
#4433=VERTEX_POINT('',#19361);
#4434=VERTEX_POINT('',#19363);
#4435=VERTEX_POINT('',#19371);
#4436=VERTEX_POINT('',#19382);
#4437=VERTEX_POINT('',#19390);
#4438=VERTEX_POINT('',#19392);
#4439=VERTEX_POINT('',#19400);
#4440=VERTEX_POINT('',#19411);
#4441=VERTEX_POINT('',#19419);
#4442=VERTEX_POINT('',#19421);
#4443=VERTEX_POINT('',#19429);
#4444=VERTEX_POINT('',#19440);
#4445=VERTEX_POINT('',#19448);
#4446=VERTEX_POINT('',#19450);
#4447=VERTEX_POINT('',#19458);
#4448=VERTEX_POINT('',#19469);
#4449=VERTEX_POINT('',#19477);
#4450=VERTEX_POINT('',#19479);
#4451=VERTEX_POINT('',#19487);
#4452=VERTEX_POINT('',#19498);
#4453=VERTEX_POINT('',#19506);
#4454=VERTEX_POINT('',#19508);
#4455=VERTEX_POINT('',#19516);
#4456=VERTEX_POINT('',#19527);
#4457=VERTEX_POINT('',#19535);
#4458=VERTEX_POINT('',#19537);
#4459=VERTEX_POINT('',#19545);
#4460=VERTEX_POINT('',#19556);
#4461=VERTEX_POINT('',#19564);
#4462=VERTEX_POINT('',#19566);
#4463=VERTEX_POINT('',#19574);
#4464=VERTEX_POINT('',#19585);
#4465=VERTEX_POINT('',#19593);
#4466=VERTEX_POINT('',#19595);
#4467=VERTEX_POINT('',#19603);
#4468=VERTEX_POINT('',#19614);
#4469=VERTEX_POINT('',#19622);
#4470=VERTEX_POINT('',#19624);
#4471=VERTEX_POINT('',#19632);
#4472=VERTEX_POINT('',#19643);
#4473=VERTEX_POINT('',#19651);
#4474=VERTEX_POINT('',#19653);
#4475=VERTEX_POINT('',#19661);
#4476=VERTEX_POINT('',#19672);
#4477=VERTEX_POINT('',#19680);
#4478=VERTEX_POINT('',#19682);
#4479=VERTEX_POINT('',#19690);
#4480=VERTEX_POINT('',#19701);
#4481=VERTEX_POINT('',#19709);
#4482=VERTEX_POINT('',#19711);
#4483=VERTEX_POINT('',#19719);
#4484=VERTEX_POINT('',#19730);
#4485=VERTEX_POINT('',#19738);
#4486=VERTEX_POINT('',#19740);
#4487=VERTEX_POINT('',#19748);
#4488=VERTEX_POINT('',#19755);
#4489=VERTEX_POINT('',#19758);
#4490=VERTEX_POINT('',#19769);
#4491=VERTEX_POINT('',#19777);
#4492=VERTEX_POINT('',#19779);
#4493=VERTEX_POINT('',#19787);
#4494=VERTEX_POINT('',#19798);
#4495=VERTEX_POINT('',#19806);
#4496=VERTEX_POINT('',#19808);
#4497=VERTEX_POINT('',#19816);
#4498=VERTEX_POINT('',#19827);
#4499=VERTEX_POINT('',#19835);
#4500=VERTEX_POINT('',#19837);
#4501=VERTEX_POINT('',#19845);
#4502=VERTEX_POINT('',#19856);
#4503=VERTEX_POINT('',#19864);
#4504=VERTEX_POINT('',#19866);
#4505=VERTEX_POINT('',#19874);
#4506=VERTEX_POINT('',#19885);
#4507=VERTEX_POINT('',#19893);
#4508=VERTEX_POINT('',#19895);
#4509=VERTEX_POINT('',#19903);
#4510=VERTEX_POINT('',#19914);
#4511=VERTEX_POINT('',#19922);
#4512=VERTEX_POINT('',#19924);
#4513=VERTEX_POINT('',#19932);
#4514=VERTEX_POINT('',#19943);
#4515=VERTEX_POINT('',#19951);
#4516=VERTEX_POINT('',#19953);
#4517=VERTEX_POINT('',#19961);
#4518=VERTEX_POINT('',#19972);
#4519=VERTEX_POINT('',#19980);
#4520=VERTEX_POINT('',#19982);
#4521=VERTEX_POINT('',#19990);
#4522=VERTEX_POINT('',#20001);
#4523=VERTEX_POINT('',#20009);
#4524=VERTEX_POINT('',#20011);
#4525=VERTEX_POINT('',#20019);
#4526=VERTEX_POINT('',#20030);
#4527=VERTEX_POINT('',#20038);
#4528=VERTEX_POINT('',#20040);
#4529=VERTEX_POINT('',#20048);
#4530=VERTEX_POINT('',#20059);
#4531=VERTEX_POINT('',#20067);
#4532=VERTEX_POINT('',#20069);
#4533=VERTEX_POINT('',#20077);
#4534=VERTEX_POINT('',#20088);
#4535=VERTEX_POINT('',#20096);
#4536=VERTEX_POINT('',#20098);
#4537=VERTEX_POINT('',#20106);
#4538=VERTEX_POINT('',#20117);
#4539=VERTEX_POINT('',#20125);
#4540=VERTEX_POINT('',#20127);
#4541=VERTEX_POINT('',#20135);
#4542=VERTEX_POINT('',#20146);
#4543=VERTEX_POINT('',#20154);
#4544=VERTEX_POINT('',#20156);
#4545=VERTEX_POINT('',#20164);
#4546=VERTEX_POINT('',#20175);
#4547=VERTEX_POINT('',#20183);
#4548=VERTEX_POINT('',#20185);
#4549=VERTEX_POINT('',#20193);
#4550=VERTEX_POINT('',#20204);
#4551=VERTEX_POINT('',#20212);
#4552=VERTEX_POINT('',#20214);
#4553=VERTEX_POINT('',#20222);
#4554=VERTEX_POINT('',#20233);
#4555=VERTEX_POINT('',#20241);
#4556=VERTEX_POINT('',#20243);
#4557=VERTEX_POINT('',#20251);
#4558=VERTEX_POINT('',#20262);
#4559=VERTEX_POINT('',#20270);
#4560=VERTEX_POINT('',#20272);
#4561=VERTEX_POINT('',#20280);
#4562=VERTEX_POINT('',#20291);
#4563=VERTEX_POINT('',#20299);
#4564=VERTEX_POINT('',#20301);
#4565=VERTEX_POINT('',#20309);
#4566=VERTEX_POINT('',#20320);
#4567=VERTEX_POINT('',#20328);
#4568=VERTEX_POINT('',#20330);
#4569=VERTEX_POINT('',#20338);
#4570=VERTEX_POINT('',#20349);
#4571=VERTEX_POINT('',#20357);
#4572=VERTEX_POINT('',#20359);
#4573=VERTEX_POINT('',#20367);
#4574=VERTEX_POINT('',#20378);
#4575=VERTEX_POINT('',#20386);
#4576=VERTEX_POINT('',#20396);
#4577=VERTEX_POINT('',#20397);
#4578=VERTEX_POINT('',#20399);
#4579=VERTEX_POINT('',#20401);
#4580=VERTEX_POINT('',#20405);
#4581=VERTEX_POINT('',#20406);
#4582=VERTEX_POINT('',#20419);
#4583=VERTEX_POINT('',#20427);
#4584=VERTEX_POINT('',#20429);
#4585=VERTEX_POINT('',#20437);
#4586=VERTEX_POINT('',#20448);
#4587=VERTEX_POINT('',#20456);
#4588=VERTEX_POINT('',#20458);
#4589=VERTEX_POINT('',#20466);
#4590=VERTEX_POINT('',#20477);
#4591=VERTEX_POINT('',#20485);
#4592=VERTEX_POINT('',#20487);
#4593=VERTEX_POINT('',#20495);
#4594=VERTEX_POINT('',#20506);
#4595=VERTEX_POINT('',#20514);
#4596=VERTEX_POINT('',#20516);
#4597=VERTEX_POINT('',#20524);
#4598=VERTEX_POINT('',#20535);
#4599=VERTEX_POINT('',#20543);
#4600=VERTEX_POINT('',#20545);
#4601=VERTEX_POINT('',#20553);
#4602=VERTEX_POINT('',#20564);
#4603=VERTEX_POINT('',#20572);
#4604=VERTEX_POINT('',#20574);
#4605=VERTEX_POINT('',#20582);
#4606=VERTEX_POINT('',#20593);
#4607=VERTEX_POINT('',#20601);
#4608=VERTEX_POINT('',#20603);
#4609=VERTEX_POINT('',#20611);
#4610=VERTEX_POINT('',#20622);
#4611=VERTEX_POINT('',#20630);
#4612=VERTEX_POINT('',#20632);
#4613=VERTEX_POINT('',#20640);
#4614=VERTEX_POINT('',#20651);
#4615=VERTEX_POINT('',#20659);
#4616=VERTEX_POINT('',#20661);
#4617=VERTEX_POINT('',#20669);
#4618=VERTEX_POINT('',#20680);
#4619=VERTEX_POINT('',#20688);
#4620=VERTEX_POINT('',#20690);
#4621=VERTEX_POINT('',#20698);
#4622=VERTEX_POINT('',#20709);
#4623=VERTEX_POINT('',#20717);
#4624=VERTEX_POINT('',#20719);
#4625=VERTEX_POINT('',#20727);
#4626=VERTEX_POINT('',#20738);
#4627=VERTEX_POINT('',#20746);
#4628=VERTEX_POINT('',#20748);
#4629=VERTEX_POINT('',#20756);
#4630=VERTEX_POINT('',#20767);
#4631=VERTEX_POINT('',#20775);
#4632=VERTEX_POINT('',#20777);
#4633=VERTEX_POINT('',#20785);
#4634=VERTEX_POINT('',#20796);
#4635=VERTEX_POINT('',#20804);
#4636=VERTEX_POINT('',#20806);
#4637=VERTEX_POINT('',#20814);
#4638=VERTEX_POINT('',#20825);
#4639=VERTEX_POINT('',#20833);
#4640=VERTEX_POINT('',#20835);
#4641=VERTEX_POINT('',#20843);
#4642=VERTEX_POINT('',#20854);
#4643=VERTEX_POINT('',#20862);
#4644=VERTEX_POINT('',#20864);
#4645=VERTEX_POINT('',#20872);
#4646=VERTEX_POINT('',#20883);
#4647=VERTEX_POINT('',#20891);
#4648=VERTEX_POINT('',#20893);
#4649=VERTEX_POINT('',#20901);
#4650=VERTEX_POINT('',#20912);
#4651=VERTEX_POINT('',#20920);
#4652=VERTEX_POINT('',#20922);
#4653=VERTEX_POINT('',#20930);
#4654=VERTEX_POINT('',#20941);
#4655=VERTEX_POINT('',#20949);
#4656=VERTEX_POINT('',#20951);
#4657=VERTEX_POINT('',#20959);
#4658=VERTEX_POINT('',#20970);
#4659=VERTEX_POINT('',#20978);
#4660=VERTEX_POINT('',#20980);
#4661=VERTEX_POINT('',#20988);
#4662=VERTEX_POINT('',#20999);
#4663=VERTEX_POINT('',#21007);
#4664=VERTEX_POINT('',#21009);
#4665=VERTEX_POINT('',#21017);
#4666=VERTEX_POINT('',#21028);
#4667=VERTEX_POINT('',#21036);
#4668=VERTEX_POINT('',#21038);
#4669=VERTEX_POINT('',#21046);
#4670=VERTEX_POINT('',#21057);
#4671=VERTEX_POINT('',#21060);
#4672=VERTEX_POINT('',#21067);
#4673=VERTEX_POINT('',#21075);
#4674=VERTEX_POINT('',#21077);
#4675=VERTEX_POINT('',#21085);
#4676=VERTEX_POINT('',#21096);
#4677=VERTEX_POINT('',#21104);
#4678=VERTEX_POINT('',#21106);
#4679=VERTEX_POINT('',#21114);
#4680=VERTEX_POINT('',#21125);
#4681=VERTEX_POINT('',#21133);
#4682=VERTEX_POINT('',#21135);
#4683=VERTEX_POINT('',#21143);
#4684=VERTEX_POINT('',#21154);
#4685=VERTEX_POINT('',#21162);
#4686=VERTEX_POINT('',#21164);
#4687=VERTEX_POINT('',#21172);
#4688=VERTEX_POINT('',#21183);
#4689=VERTEX_POINT('',#21191);
#4690=VERTEX_POINT('',#21193);
#4691=VERTEX_POINT('',#21201);
#4692=VERTEX_POINT('',#21212);
#4693=VERTEX_POINT('',#21220);
#4694=VERTEX_POINT('',#21222);
#4695=VERTEX_POINT('',#21230);
#4696=VERTEX_POINT('',#21241);
#4697=VERTEX_POINT('',#21249);
#4698=VERTEX_POINT('',#21251);
#4699=VERTEX_POINT('',#21259);
#4700=VERTEX_POINT('',#21270);
#4701=VERTEX_POINT('',#21278);
#4702=VERTEX_POINT('',#21280);
#4703=VERTEX_POINT('',#21288);
#4704=VERTEX_POINT('',#21299);
#4705=VERTEX_POINT('',#21307);
#4706=VERTEX_POINT('',#21309);
#4707=VERTEX_POINT('',#21317);
#4708=VERTEX_POINT('',#21328);
#4709=VERTEX_POINT('',#21336);
#4710=VERTEX_POINT('',#21338);
#4711=VERTEX_POINT('',#21346);
#4712=VERTEX_POINT('',#21357);
#4713=VERTEX_POINT('',#21365);
#4714=VERTEX_POINT('',#21367);
#4715=VERTEX_POINT('',#21375);
#4716=VERTEX_POINT('',#21386);
#4717=VERTEX_POINT('',#21394);
#4718=VERTEX_POINT('',#21396);
#4719=VERTEX_POINT('',#21404);
#4720=VERTEX_POINT('',#21415);
#4721=VERTEX_POINT('',#21423);
#4722=VERTEX_POINT('',#21425);
#4723=VERTEX_POINT('',#21433);
#4724=VERTEX_POINT('',#21444);
#4725=VERTEX_POINT('',#21452);
#4726=VERTEX_POINT('',#21454);
#4727=VERTEX_POINT('',#21462);
#4728=VERTEX_POINT('',#21473);
#4729=VERTEX_POINT('',#21481);
#4730=VERTEX_POINT('',#21483);
#4731=VERTEX_POINT('',#21491);
#4732=VERTEX_POINT('',#21502);
#4733=VERTEX_POINT('',#21510);
#4734=VERTEX_POINT('',#21512);
#4735=VERTEX_POINT('',#21520);
#4736=VERTEX_POINT('',#21531);
#4737=VERTEX_POINT('',#21539);
#4738=VERTEX_POINT('',#21541);
#4739=VERTEX_POINT('',#21549);
#4740=VERTEX_POINT('',#21560);
#4741=VERTEX_POINT('',#21568);
#4742=VERTEX_POINT('',#21570);
#4743=VERTEX_POINT('',#21578);
#4744=VERTEX_POINT('',#21589);
#4745=VERTEX_POINT('',#21597);
#4746=VERTEX_POINT('',#21599);
#4747=VERTEX_POINT('',#21607);
#4748=VERTEX_POINT('',#21618);
#4749=VERTEX_POINT('',#21626);
#4750=VERTEX_POINT('',#21628);
#4751=VERTEX_POINT('',#21636);
#4752=VERTEX_POINT('',#21647);
#4753=VERTEX_POINT('',#21655);
#4754=VERTEX_POINT('',#21657);
#4755=VERTEX_POINT('',#21665);
#4756=VERTEX_POINT('',#21676);
#4757=VERTEX_POINT('',#21684);
#4758=VERTEX_POINT('',#22838);
#4759=VERTEX_POINT('',#22840);
#4760=VERTEX_POINT('',#22844);
#4761=VERTEX_POINT('',#22846);
#4762=VERTEX_POINT('',#22890);
#4763=VERTEX_POINT('',#22943);
#4764=VERTEX_POINT('',#22945);
#4765=VERTEX_POINT('',#23222);
#4766=VERTEX_POINT('',#23312);
#4767=VERTEX_POINT('',#23355);
#4768=VERTEX_POINT('',#23394);
#4769=VERTEX_POINT('',#23484);
#4770=VERTEX_POINT('',#23527);
#4771=VERTEX_POINT('',#23566);
#4772=VERTEX_POINT('',#23609);
#4773=VERTEX_POINT('',#23652);
#4774=VERTEX_POINT('',#23691);
#4775=VERTEX_POINT('',#23781);
#4776=VERTEX_POINT('',#23824);
#4777=VERTEX_POINT('',#23863);
#4778=VERTEX_POINT('',#23953);
#4779=VERTEX_POINT('',#23996);
#4780=VERTEX_POINT('',#24035);
#4781=VERTEX_POINT('',#24125);
#4782=VERTEX_POINT('',#24168);
#4783=VERTEX_POINT('',#24207);
#4784=VERTEX_POINT('',#24297);
#4785=VERTEX_POINT('',#24340);
#4786=VERTEX_POINT('',#24379);
#4787=VERTEX_POINT('',#24469);
#4788=VERTEX_POINT('',#24512);
#4789=VERTEX_POINT('',#24551);
#4790=VERTEX_POINT('',#24641);
#4791=VERTEX_POINT('',#24684);
#4792=VERTEX_POINT('',#24723);
#4793=VERTEX_POINT('',#24813);
#4794=VERTEX_POINT('',#24856);
#4795=VERTEX_POINT('',#24895);
#4796=VERTEX_POINT('',#24985);
#4797=VERTEX_POINT('',#25028);
#4798=VERTEX_POINT('',#25067);
#4799=VERTEX_POINT('',#25110);
#4800=VERTEX_POINT('',#25153);
#4801=VERTEX_POINT('',#25192);
#4802=VERTEX_POINT('',#25282);
#4803=VERTEX_POINT('',#25325);
#4804=VERTEX_POINT('',#25364);
#4805=VERTEX_POINT('',#25454);
#4806=VERTEX_POINT('',#25497);
#4807=VERTEX_POINT('',#25536);
#4808=VERTEX_POINT('',#25579);
#4809=VERTEX_POINT('',#25622);
#4810=VERTEX_POINT('',#25661);
#4811=VERTEX_POINT('',#25751);
#4812=VERTEX_POINT('',#25794);
#4813=VERTEX_POINT('',#25833);
#4814=VERTEX_POINT('',#25923);
#4815=VERTEX_POINT('',#25966);
#4816=VERTEX_POINT('',#26005);
#4817=VERTEX_POINT('',#26095);
#4818=VERTEX_POINT('',#26138);
#4819=VERTEX_POINT('',#26177);
#4820=VERTEX_POINT('',#26267);
#4821=VERTEX_POINT('',#26310);
#4822=VERTEX_POINT('',#26349);
#4823=VERTEX_POINT('',#26439);
#4824=VERTEX_POINT('',#26482);
#4825=VERTEX_POINT('',#26521);
#4826=VERTEX_POINT('',#26611);
#4827=VERTEX_POINT('',#26654);
#4828=VERTEX_POINT('',#26693);
#4829=VERTEX_POINT('',#26783);
#4830=VERTEX_POINT('',#26826);
#4831=VERTEX_POINT('',#26865);
#4832=VERTEX_POINT('',#26955);
#4833=VERTEX_POINT('',#26998);
#4834=VERTEX_POINT('',#27037);
#4835=VERTEX_POINT('',#27127);
#4836=VERTEX_POINT('',#27170);
#4837=VERTEX_POINT('',#27209);
#4838=VERTEX_POINT('',#27252);
#4839=VERTEX_POINT('',#27295);
#4840=VERTEX_POINT('',#27334);
#4841=VERTEX_POINT('',#27377);
#4842=VERTEX_POINT('',#27420);
#4843=VERTEX_POINT('',#27459);
#4844=VERTEX_POINT('',#27549);
#4845=VERTEX_POINT('',#27592);
#4846=VERTEX_POINT('',#27631);
#4847=VERTEX_POINT('',#27721);
#4848=VERTEX_POINT('',#27764);
#4849=VERTEX_POINT('',#27803);
#4850=VERTEX_POINT('',#27893);
#4851=VERTEX_POINT('',#27936);
#4852=VERTEX_POINT('',#27975);
#4853=VERTEX_POINT('',#28065);
#4854=VERTEX_POINT('',#28108);
#4855=VERTEX_POINT('',#28147);
#4856=VERTEX_POINT('',#28237);
#4857=VERTEX_POINT('',#28280);
#4858=VERTEX_POINT('',#28319);
#4859=VERTEX_POINT('',#28409);
#4860=VERTEX_POINT('',#28452);
#4861=VERTEX_POINT('',#28491);
#4862=VERTEX_POINT('',#28534);
#4863=VERTEX_POINT('',#28577);
#4864=VERTEX_POINT('',#28616);
#4865=VERTEX_POINT('',#28659);
#4866=VERTEX_POINT('',#28702);
#4867=VERTEX_POINT('',#28741);
#4868=VERTEX_POINT('',#28831);
#4869=VERTEX_POINT('',#28874);
#4870=VERTEX_POINT('',#28913);
#4871=VERTEX_POINT('',#29003);
#4872=VERTEX_POINT('',#29046);
#4873=VERTEX_POINT('',#29085);
#4874=VERTEX_POINT('',#29128);
#4875=VERTEX_POINT('',#29171);
#4876=VERTEX_POINT('',#29210);
#4877=VERTEX_POINT('',#29300);
#4878=VERTEX_POINT('',#29343);
#4879=VERTEX_POINT('',#29382);
#4880=VERTEX_POINT('',#29472);
#4881=VERTEX_POINT('',#29515);
#4882=VERTEX_POINT('',#29554);
#4883=VERTEX_POINT('',#29644);
#4884=VERTEX_POINT('',#29687);
#4885=VERTEX_POINT('',#29726);
#4886=VERTEX_POINT('',#29816);
#4887=VERTEX_POINT('',#29859);
#4888=VERTEX_POINT('',#29898);
#4889=VERTEX_POINT('',#29988);
#4890=VERTEX_POINT('',#30031);
#4891=VERTEX_POINT('',#30070);
#4892=VERTEX_POINT('',#30113);
#4893=VERTEX_POINT('',#30156);
#5280=EDGE_CURVE('',#4134,#4135,#617,.T.);
#5281=EDGE_CURVE('',#4136,#4135,#618,.T.);
#5282=EDGE_CURVE('',#4137,#4136,#3534,.T.);
#5283=EDGE_CURVE('',#4138,#4137,#619,.T.);
#5284=EDGE_CURVE('',#4138,#4139,#620,.T.);
#5285=EDGE_CURVE('',#4134,#4139,#3535,.T.);
#5286=EDGE_CURVE('',#4140,#4141,#621,.T.);
#5287=EDGE_CURVE('',#4142,#4141,#622,.T.);
#5288=EDGE_CURVE('',#4143,#4142,#3536,.T.);
#5289=EDGE_CURVE('',#4144,#4143,#623,.T.);
#5290=EDGE_CURVE('',#4144,#4145,#624,.T.);
#5291=EDGE_CURVE('',#4140,#4145,#3537,.T.);
#5292=EDGE_CURVE('',#4146,#4147,#625,.T.);
#5293=EDGE_CURVE('',#4148,#4147,#626,.T.);
#5294=EDGE_CURVE('',#4149,#4148,#3538,.T.);
#5295=EDGE_CURVE('',#4150,#4149,#627,.T.);
#5296=EDGE_CURVE('',#4150,#4151,#628,.T.);
#5297=EDGE_CURVE('',#4146,#4151,#3539,.T.);
#5298=EDGE_CURVE('',#4152,#4153,#629,.T.);
#5299=EDGE_CURVE('',#4154,#4153,#630,.T.);
#5300=EDGE_CURVE('',#4155,#4154,#3540,.T.);
#5301=EDGE_CURVE('',#4156,#4155,#631,.T.);
#5302=EDGE_CURVE('',#4156,#4157,#632,.T.);
#5303=EDGE_CURVE('',#4152,#4157,#3541,.T.);
#5304=EDGE_CURVE('',#4158,#4159,#633,.T.);
#5305=EDGE_CURVE('',#4160,#4159,#634,.T.);
#5306=EDGE_CURVE('',#4161,#4160,#3542,.T.);
#5307=EDGE_CURVE('',#4162,#4161,#635,.T.);
#5308=EDGE_CURVE('',#4162,#4163,#636,.T.);
#5309=EDGE_CURVE('',#4158,#4163,#3543,.T.);
#5310=EDGE_CURVE('',#4164,#4165,#637,.T.);
#5311=EDGE_CURVE('',#4166,#4165,#638,.T.);
#5312=EDGE_CURVE('',#4167,#4166,#3544,.T.);
#5313=EDGE_CURVE('',#4168,#4167,#639,.T.);
#5314=EDGE_CURVE('',#4168,#4169,#640,.T.);
#5315=EDGE_CURVE('',#4164,#4169,#3545,.T.);
#5316=EDGE_CURVE('',#4170,#4171,#641,.T.);
#5317=EDGE_CURVE('',#4172,#4171,#642,.T.);
#5318=EDGE_CURVE('',#4173,#4172,#3546,.T.);
#5319=EDGE_CURVE('',#4174,#4173,#643,.T.);
#5320=EDGE_CURVE('',#4174,#4175,#644,.T.);
#5321=EDGE_CURVE('',#4170,#4175,#3547,.T.);
#5322=EDGE_CURVE('',#4176,#4177,#645,.T.);
#5323=EDGE_CURVE('',#4178,#4177,#646,.T.);
#5324=EDGE_CURVE('',#4179,#4178,#3548,.T.);
#5325=EDGE_CURVE('',#4180,#4179,#647,.T.);
#5326=EDGE_CURVE('',#4180,#4181,#648,.T.);
#5327=EDGE_CURVE('',#4176,#4181,#3549,.T.);
#5328=EDGE_CURVE('',#4182,#4183,#649,.T.);
#5329=EDGE_CURVE('',#4184,#4183,#650,.T.);
#5330=EDGE_CURVE('',#4185,#4184,#3550,.T.);
#5331=EDGE_CURVE('',#4186,#4185,#651,.T.);
#5332=EDGE_CURVE('',#4186,#4187,#652,.T.);
#5333=EDGE_CURVE('',#4182,#4187,#3551,.T.);
#5334=EDGE_CURVE('',#4188,#4189,#653,.T.);
#5335=EDGE_CURVE('',#4190,#4189,#654,.T.);
#5336=EDGE_CURVE('',#4191,#4190,#3552,.T.);
#5337=EDGE_CURVE('',#4192,#4191,#655,.T.);
#5338=EDGE_CURVE('',#4192,#4193,#656,.T.);
#5339=EDGE_CURVE('',#4188,#4193,#3553,.T.);
#5340=EDGE_CURVE('',#4194,#4195,#657,.T.);
#5341=EDGE_CURVE('',#4196,#4195,#658,.T.);
#5342=EDGE_CURVE('',#4197,#4196,#3554,.T.);
#5343=EDGE_CURVE('',#4198,#4197,#659,.T.);
#5344=EDGE_CURVE('',#4198,#4199,#660,.T.);
#5345=EDGE_CURVE('',#4194,#4199,#3555,.T.);
#5346=EDGE_CURVE('',#4200,#4201,#661,.T.);
#5347=EDGE_CURVE('',#4202,#4201,#662,.T.);
#5348=EDGE_CURVE('',#4203,#4202,#3556,.T.);
#5349=EDGE_CURVE('',#4204,#4203,#663,.T.);
#5350=EDGE_CURVE('',#4204,#4205,#664,.T.);
#5351=EDGE_CURVE('',#4200,#4205,#3557,.T.);
#5352=EDGE_CURVE('',#4206,#4207,#665,.T.);
#5353=EDGE_CURVE('',#4208,#4207,#666,.T.);
#5354=EDGE_CURVE('',#4209,#4208,#3558,.T.);
#5355=EDGE_CURVE('',#4210,#4209,#667,.T.);
#5356=EDGE_CURVE('',#4210,#4211,#668,.T.);
#5357=EDGE_CURVE('',#4206,#4211,#3559,.T.);
#5358=EDGE_CURVE('',#4212,#4213,#669,.T.);
#5359=EDGE_CURVE('',#4214,#4213,#670,.T.);
#5360=EDGE_CURVE('',#4215,#4214,#3560,.T.);
#5361=EDGE_CURVE('',#4216,#4215,#671,.T.);
#5362=EDGE_CURVE('',#4216,#4217,#672,.T.);
#5363=EDGE_CURVE('',#4212,#4217,#3561,.T.);
#5364=EDGE_CURVE('',#4218,#4219,#673,.T.);
#5365=EDGE_CURVE('',#4220,#4219,#674,.T.);
#5366=EDGE_CURVE('',#4221,#4220,#3562,.T.);
#5367=EDGE_CURVE('',#4222,#4221,#675,.T.);
#5368=EDGE_CURVE('',#4222,#4223,#676,.T.);
#5369=EDGE_CURVE('',#4218,#4223,#3563,.T.);
#5370=EDGE_CURVE('',#4224,#4225,#677,.T.);
#5371=EDGE_CURVE('',#4226,#4225,#678,.T.);
#5372=EDGE_CURVE('',#4227,#4226,#3564,.T.);
#5373=EDGE_CURVE('',#4228,#4227,#679,.T.);
#5374=EDGE_CURVE('',#4228,#4229,#680,.T.);
#5375=EDGE_CURVE('',#4224,#4229,#3565,.T.);
#5376=EDGE_CURVE('',#4230,#4231,#681,.T.);
#5377=EDGE_CURVE('',#4232,#4231,#682,.T.);
#5378=EDGE_CURVE('',#4233,#4232,#3566,.T.);
#5379=EDGE_CURVE('',#4234,#4233,#683,.T.);
#5380=EDGE_CURVE('',#4234,#4235,#684,.T.);
#5381=EDGE_CURVE('',#4230,#4235,#3567,.T.);
#5382=EDGE_CURVE('',#4236,#4237,#685,.T.);
#5383=EDGE_CURVE('',#4238,#4237,#686,.T.);
#5384=EDGE_CURVE('',#4239,#4238,#3568,.T.);
#5385=EDGE_CURVE('',#4240,#4239,#687,.T.);
#5386=EDGE_CURVE('',#4240,#4241,#688,.T.);
#5387=EDGE_CURVE('',#4236,#4241,#3569,.T.);
#5388=EDGE_CURVE('',#4242,#4243,#689,.T.);
#5389=EDGE_CURVE('',#4244,#4243,#690,.T.);
#5390=EDGE_CURVE('',#4245,#4244,#3570,.T.);
#5391=EDGE_CURVE('',#4246,#4245,#691,.T.);
#5392=EDGE_CURVE('',#4246,#4247,#692,.T.);
#5393=EDGE_CURVE('',#4242,#4247,#3571,.T.);
#5394=EDGE_CURVE('',#4248,#4249,#693,.T.);
#5395=EDGE_CURVE('',#4250,#4249,#694,.T.);
#5396=EDGE_CURVE('',#4251,#4250,#3572,.T.);
#5397=EDGE_CURVE('',#4252,#4251,#695,.T.);
#5398=EDGE_CURVE('',#4252,#4253,#696,.T.);
#5399=EDGE_CURVE('',#4248,#4253,#3573,.T.);
#5400=EDGE_CURVE('',#4254,#4255,#697,.T.);
#5401=EDGE_CURVE('',#4256,#4255,#698,.T.);
#5402=EDGE_CURVE('',#4257,#4256,#3574,.T.);
#5403=EDGE_CURVE('',#4258,#4257,#699,.T.);
#5404=EDGE_CURVE('',#4258,#4259,#700,.T.);
#5405=EDGE_CURVE('',#4254,#4259,#3575,.T.);
#5406=EDGE_CURVE('',#4260,#4261,#701,.T.);
#5407=EDGE_CURVE('',#4262,#4261,#702,.T.);
#5408=EDGE_CURVE('',#4263,#4262,#3576,.T.);
#5409=EDGE_CURVE('',#4264,#4263,#703,.T.);
#5410=EDGE_CURVE('',#4264,#4265,#704,.T.);
#5411=EDGE_CURVE('',#4260,#4265,#3577,.T.);
#5412=EDGE_CURVE('',#4266,#4267,#705,.T.);
#5413=EDGE_CURVE('',#4268,#4267,#706,.T.);
#5414=EDGE_CURVE('',#4269,#4268,#3578,.T.);
#5415=EDGE_CURVE('',#4270,#4269,#707,.T.);
#5416=EDGE_CURVE('',#4270,#4271,#708,.T.);
#5417=EDGE_CURVE('',#4266,#4271,#3579,.T.);
#5418=EDGE_CURVE('',#4272,#4273,#709,.T.);
#5419=EDGE_CURVE('',#4274,#4273,#710,.T.);
#5420=EDGE_CURVE('',#4275,#4274,#3580,.T.);
#5421=EDGE_CURVE('',#4276,#4275,#711,.T.);
#5422=EDGE_CURVE('',#4276,#4277,#712,.T.);
#5423=EDGE_CURVE('',#4272,#4277,#3581,.T.);
#5424=EDGE_CURVE('',#4278,#4279,#713,.T.);
#5425=EDGE_CURVE('',#4280,#4279,#714,.T.);
#5426=EDGE_CURVE('',#4281,#4280,#3582,.T.);
#5427=EDGE_CURVE('',#4282,#4281,#715,.T.);
#5428=EDGE_CURVE('',#4282,#4283,#716,.T.);
#5429=EDGE_CURVE('',#4278,#4283,#3583,.T.);
#5430=EDGE_CURVE('',#4284,#4285,#717,.T.);
#5431=EDGE_CURVE('',#4286,#4285,#718,.T.);
#5432=EDGE_CURVE('',#4287,#4286,#3584,.T.);
#5433=EDGE_CURVE('',#4288,#4287,#719,.T.);
#5434=EDGE_CURVE('',#4288,#4289,#720,.T.);
#5435=EDGE_CURVE('',#4284,#4289,#3585,.T.);
#5436=EDGE_CURVE('',#4290,#4291,#721,.T.);
#5437=EDGE_CURVE('',#4292,#4291,#722,.T.);
#5438=EDGE_CURVE('',#4293,#4292,#3586,.T.);
#5439=EDGE_CURVE('',#4294,#4293,#723,.T.);
#5440=EDGE_CURVE('',#4294,#4295,#724,.T.);
#5441=EDGE_CURVE('',#4290,#4295,#3587,.T.);
#5442=EDGE_CURVE('',#4296,#4297,#725,.T.);
#5443=EDGE_CURVE('',#4298,#4297,#726,.T.);
#5444=EDGE_CURVE('',#4299,#4298,#3588,.T.);
#5445=EDGE_CURVE('',#4300,#4299,#727,.T.);
#5446=EDGE_CURVE('',#4300,#4301,#728,.T.);
#5447=EDGE_CURVE('',#4296,#4301,#3589,.T.);
#5448=EDGE_CURVE('',#4302,#4303,#729,.T.);
#5449=EDGE_CURVE('',#4304,#4303,#730,.T.);
#5450=EDGE_CURVE('',#4305,#4304,#3590,.T.);
#5451=EDGE_CURVE('',#4306,#4305,#731,.T.);
#5452=EDGE_CURVE('',#4306,#4307,#732,.T.);
#5453=EDGE_CURVE('',#4302,#4307,#3591,.T.);
#5454=EDGE_CURVE('',#4308,#4309,#733,.T.);
#5455=EDGE_CURVE('',#4310,#4309,#734,.T.);
#5456=EDGE_CURVE('',#4311,#4310,#3592,.T.);
#5457=EDGE_CURVE('',#4312,#4311,#735,.T.);
#5458=EDGE_CURVE('',#4312,#4313,#736,.T.);
#5459=EDGE_CURVE('',#4308,#4313,#3593,.T.);
#5460=EDGE_CURVE('',#4314,#4315,#737,.T.);
#5461=EDGE_CURVE('',#4316,#4315,#738,.T.);
#5462=EDGE_CURVE('',#4317,#4316,#3594,.T.);
#5463=EDGE_CURVE('',#4318,#4317,#739,.T.);
#5464=EDGE_CURVE('',#4318,#4319,#740,.T.);
#5465=EDGE_CURVE('',#4314,#4319,#3595,.T.);
#5466=EDGE_CURVE('',#4320,#4321,#741,.T.);
#5467=EDGE_CURVE('',#4322,#4321,#742,.T.);
#5468=EDGE_CURVE('',#4323,#4322,#3596,.T.);
#5469=EDGE_CURVE('',#4324,#4323,#743,.T.);
#5470=EDGE_CURVE('',#4324,#4325,#744,.T.);
#5471=EDGE_CURVE('',#4320,#4325,#3597,.T.);
#5472=EDGE_CURVE('',#4326,#4327,#745,.T.);
#5473=EDGE_CURVE('',#4328,#4327,#746,.T.);
#5474=EDGE_CURVE('',#4329,#4328,#3598,.T.);
#5475=EDGE_CURVE('',#4330,#4329,#747,.T.);
#5476=EDGE_CURVE('',#4330,#4331,#748,.T.);
#5477=EDGE_CURVE('',#4326,#4331,#3599,.T.);
#5478=EDGE_CURVE('',#4332,#4333,#749,.T.);
#5479=EDGE_CURVE('',#4334,#4333,#750,.T.);
#5480=EDGE_CURVE('',#4335,#4334,#3600,.T.);
#5481=EDGE_CURVE('',#4336,#4335,#751,.T.);
#5482=EDGE_CURVE('',#4336,#4337,#752,.T.);
#5483=EDGE_CURVE('',#4332,#4337,#3601,.T.);
#5484=EDGE_CURVE('',#4338,#4339,#753,.T.);
#5485=EDGE_CURVE('',#4340,#4339,#754,.T.);
#5486=EDGE_CURVE('',#4341,#4340,#3602,.T.);
#5487=EDGE_CURVE('',#4342,#4341,#755,.T.);
#5488=EDGE_CURVE('',#4342,#4343,#756,.T.);
#5489=EDGE_CURVE('',#4338,#4343,#3603,.T.);
#5490=EDGE_CURVE('',#4344,#4345,#757,.T.);
#5491=EDGE_CURVE('',#4346,#4345,#758,.T.);
#5492=EDGE_CURVE('',#4347,#4346,#3604,.T.);
#5493=EDGE_CURVE('',#4348,#4347,#759,.T.);
#5494=EDGE_CURVE('',#4348,#4349,#760,.T.);
#5495=EDGE_CURVE('',#4344,#4349,#3605,.T.);
#5496=EDGE_CURVE('',#4350,#4351,#761,.T.);
#5497=EDGE_CURVE('',#4352,#4351,#762,.T.);
#5498=EDGE_CURVE('',#4353,#4352,#3606,.T.);
#5499=EDGE_CURVE('',#4354,#4353,#763,.T.);
#5500=EDGE_CURVE('',#4354,#4355,#764,.T.);
#5501=EDGE_CURVE('',#4350,#4355,#3607,.T.);
#5502=EDGE_CURVE('',#4356,#4357,#765,.T.);
#5503=EDGE_CURVE('',#4358,#4357,#766,.T.);
#5504=EDGE_CURVE('',#4359,#4358,#3608,.T.);
#5505=EDGE_CURVE('',#4360,#4359,#767,.T.);
#5506=EDGE_CURVE('',#4360,#4361,#768,.T.);
#5507=EDGE_CURVE('',#4356,#4361,#3609,.T.);
#5508=EDGE_CURVE('',#4362,#4363,#769,.T.);
#5509=EDGE_CURVE('',#4364,#4363,#770,.T.);
#5510=EDGE_CURVE('',#4365,#4364,#3610,.T.);
#5511=EDGE_CURVE('',#4366,#4365,#771,.T.);
#5512=EDGE_CURVE('',#4366,#4367,#772,.T.);
#5513=EDGE_CURVE('',#4362,#4367,#3611,.T.);
#5514=EDGE_CURVE('',#4368,#4369,#773,.T.);
#5515=EDGE_CURVE('',#4370,#4369,#774,.T.);
#5516=EDGE_CURVE('',#4371,#4370,#3612,.T.);
#5517=EDGE_CURVE('',#4372,#4371,#775,.T.);
#5518=EDGE_CURVE('',#4372,#4373,#776,.T.);
#5519=EDGE_CURVE('',#4368,#4373,#3613,.T.);
#5520=EDGE_CURVE('',#4374,#4375,#777,.T.);
#5521=EDGE_CURVE('',#4376,#4375,#778,.T.);
#5522=EDGE_CURVE('',#4377,#4376,#3614,.T.);
#5523=EDGE_CURVE('',#4378,#4377,#779,.T.);
#5524=EDGE_CURVE('',#4378,#4379,#780,.T.);
#5525=EDGE_CURVE('',#4374,#4379,#3615,.T.);
#5526=EDGE_CURVE('',#4380,#4381,#781,.T.);
#5527=EDGE_CURVE('',#4382,#4381,#782,.T.);
#5528=EDGE_CURVE('',#4383,#4382,#3616,.T.);
#5529=EDGE_CURVE('',#4384,#4383,#783,.T.);
#5530=EDGE_CURVE('',#4384,#4385,#784,.T.);
#5531=EDGE_CURVE('',#4380,#4385,#3617,.T.);
#5532=EDGE_CURVE('',#4386,#4387,#785,.T.);
#5533=EDGE_CURVE('',#4388,#4387,#786,.T.);
#5534=EDGE_CURVE('',#4389,#4388,#3618,.T.);
#5535=EDGE_CURVE('',#4390,#4389,#787,.T.);
#5536=EDGE_CURVE('',#4390,#4391,#788,.T.);
#5537=EDGE_CURVE('',#4386,#4391,#3619,.T.);
#5538=EDGE_CURVE('',#4392,#4393,#789,.T.);
#5539=EDGE_CURVE('',#4394,#4393,#790,.T.);
#5540=EDGE_CURVE('',#4395,#4394,#3620,.T.);
#5541=EDGE_CURVE('',#4396,#4395,#791,.T.);
#5542=EDGE_CURVE('',#4396,#4397,#792,.T.);
#5543=EDGE_CURVE('',#4392,#4397,#3621,.T.);
#5544=EDGE_CURVE('',#4398,#4399,#793,.T.);
#5545=EDGE_CURVE('',#4400,#4398,#794,.T.);
#5546=EDGE_CURVE('',#4401,#4400,#3622,.T.);
#5547=EDGE_CURVE('',#4402,#4401,#795,.T.);
#5548=EDGE_CURVE('',#4403,#4402,#796,.T.);
#5549=EDGE_CURVE('',#4404,#4403,#797,.T.);
#5550=EDGE_CURVE('',#4405,#4404,#3623,.T.);
#5551=EDGE_CURVE('',#4406,#4405,#798,.T.);
#5552=EDGE_CURVE('',#4407,#4406,#799,.T.);
#5553=EDGE_CURVE('',#4408,#4407,#800,.T.);
#5554=EDGE_CURVE('',#4409,#4408,#3624,.T.);
#5555=EDGE_CURVE('',#4410,#4409,#801,.T.);
#5556=EDGE_CURVE('',#4411,#4410,#802,.T.);
#5557=EDGE_CURVE('',#4412,#4411,#803,.T.);
#5558=EDGE_CURVE('',#4413,#4412,#3625,.T.);
#5559=EDGE_CURVE('',#4414,#4413,#804,.T.);
#5560=EDGE_CURVE('',#4415,#4414,#805,.T.);
#5561=EDGE_CURVE('',#4416,#4415,#806,.T.);
#5562=EDGE_CURVE('',#4417,#4416,#3626,.T.);
#5563=EDGE_CURVE('',#4418,#4417,#807,.T.);
#5564=EDGE_CURVE('',#4419,#4418,#808,.T.);
#5565=EDGE_CURVE('',#4420,#4419,#809,.T.);
#5566=EDGE_CURVE('',#4421,#4420,#3627,.T.);
#5567=EDGE_CURVE('',#4422,#4421,#810,.T.);
#5568=EDGE_CURVE('',#4423,#4422,#811,.T.);
#5569=EDGE_CURVE('',#4424,#4423,#812,.T.);
#5570=EDGE_CURVE('',#4425,#4424,#3628,.T.);
#5571=EDGE_CURVE('',#4426,#4425,#813,.T.);
#5572=EDGE_CURVE('',#4427,#4426,#814,.T.);
#5573=EDGE_CURVE('',#4428,#4427,#815,.T.);
#5574=EDGE_CURVE('',#4429,#4428,#3629,.T.);
#5575=EDGE_CURVE('',#4430,#4429,#816,.T.);
#5576=EDGE_CURVE('',#4431,#4430,#817,.T.);
#5577=EDGE_CURVE('',#4432,#4431,#818,.T.);
#5578=EDGE_CURVE('',#4433,#4432,#3630,.T.);
#5579=EDGE_CURVE('',#4434,#4433,#819,.T.);
#5580=EDGE_CURVE('',#4435,#4434,#820,.T.);
#5581=EDGE_CURVE('',#4436,#4435,#821,.T.);
#5582=EDGE_CURVE('',#4437,#4436,#3631,.T.);
#5583=EDGE_CURVE('',#4438,#4437,#822,.T.);
#5584=EDGE_CURVE('',#4439,#4438,#823,.T.);
#5585=EDGE_CURVE('',#4440,#4439,#824,.T.);
#5586=EDGE_CURVE('',#4441,#4440,#3632,.T.);
#5587=EDGE_CURVE('',#4442,#4441,#825,.T.);
#5588=EDGE_CURVE('',#4443,#4442,#826,.T.);
#5589=EDGE_CURVE('',#4444,#4443,#827,.T.);
#5590=EDGE_CURVE('',#4445,#4444,#3633,.T.);
#5591=EDGE_CURVE('',#4446,#4445,#828,.T.);
#5592=EDGE_CURVE('',#4447,#4446,#829,.T.);
#5593=EDGE_CURVE('',#4448,#4447,#830,.T.);
#5594=EDGE_CURVE('',#4449,#4448,#3634,.T.);
#5595=EDGE_CURVE('',#4450,#4449,#831,.T.);
#5596=EDGE_CURVE('',#4451,#4450,#832,.T.);
#5597=EDGE_CURVE('',#4452,#4451,#833,.T.);
#5598=EDGE_CURVE('',#4453,#4452,#3635,.T.);
#5599=EDGE_CURVE('',#4454,#4453,#834,.T.);
#5600=EDGE_CURVE('',#4455,#4454,#835,.T.);
#5601=EDGE_CURVE('',#4456,#4455,#836,.T.);
#5602=EDGE_CURVE('',#4457,#4456,#3636,.T.);
#5603=EDGE_CURVE('',#4458,#4457,#837,.T.);
#5604=EDGE_CURVE('',#4459,#4458,#838,.T.);
#5605=EDGE_CURVE('',#4460,#4459,#839,.T.);
#5606=EDGE_CURVE('',#4461,#4460,#3637,.T.);
#5607=EDGE_CURVE('',#4462,#4461,#840,.T.);
#5608=EDGE_CURVE('',#4463,#4462,#841,.T.);
#5609=EDGE_CURVE('',#4464,#4463,#842,.T.);
#5610=EDGE_CURVE('',#4465,#4464,#3638,.T.);
#5611=EDGE_CURVE('',#4466,#4465,#843,.T.);
#5612=EDGE_CURVE('',#4467,#4466,#844,.T.);
#5613=EDGE_CURVE('',#4468,#4467,#845,.T.);
#5614=EDGE_CURVE('',#4469,#4468,#3639,.T.);
#5615=EDGE_CURVE('',#4470,#4469,#846,.T.);
#5616=EDGE_CURVE('',#4471,#4470,#847,.T.);
#5617=EDGE_CURVE('',#4472,#4471,#848,.T.);
#5618=EDGE_CURVE('',#4473,#4472,#3640,.T.);
#5619=EDGE_CURVE('',#4474,#4473,#849,.T.);
#5620=EDGE_CURVE('',#4475,#4474,#850,.T.);
#5621=EDGE_CURVE('',#4476,#4475,#851,.T.);
#5622=EDGE_CURVE('',#4477,#4476,#3641,.T.);
#5623=EDGE_CURVE('',#4478,#4477,#852,.T.);
#5624=EDGE_CURVE('',#4479,#4478,#853,.T.);
#5625=EDGE_CURVE('',#4480,#4479,#854,.T.);
#5626=EDGE_CURVE('',#4481,#4480,#3642,.T.);
#5627=EDGE_CURVE('',#4482,#4481,#855,.T.);
#5628=EDGE_CURVE('',#4483,#4482,#856,.T.);
#5629=EDGE_CURVE('',#4484,#4483,#857,.T.);
#5630=EDGE_CURVE('',#4485,#4484,#3643,.T.);
#5631=EDGE_CURVE('',#4486,#4485,#858,.T.);
#5632=EDGE_CURVE('',#4487,#4486,#859,.F.);
#5633=EDGE_CURVE('',#4487,#4488,#2989,.T.);
#5634=EDGE_CURVE('',#4488,#4488,#3644,.T.);
#5635=EDGE_CURVE('',#4489,#4487,#860,.F.);
#5636=EDGE_CURVE('',#4490,#4489,#861,.T.);
#5637=EDGE_CURVE('',#4491,#4490,#3645,.T.);
#5638=EDGE_CURVE('',#4492,#4491,#862,.T.);
#5639=EDGE_CURVE('',#4493,#4492,#863,.T.);
#5640=EDGE_CURVE('',#4494,#4493,#864,.T.);
#5641=EDGE_CURVE('',#4495,#4494,#3646,.T.);
#5642=EDGE_CURVE('',#4496,#4495,#865,.T.);
#5643=EDGE_CURVE('',#4497,#4496,#866,.T.);
#5644=EDGE_CURVE('',#4498,#4497,#867,.T.);
#5645=EDGE_CURVE('',#4499,#4498,#3647,.T.);
#5646=EDGE_CURVE('',#4500,#4499,#868,.T.);
#5647=EDGE_CURVE('',#4501,#4500,#869,.T.);
#5648=EDGE_CURVE('',#4502,#4501,#870,.T.);
#5649=EDGE_CURVE('',#4503,#4502,#3648,.T.);
#5650=EDGE_CURVE('',#4504,#4503,#871,.T.);
#5651=EDGE_CURVE('',#4505,#4504,#872,.T.);
#5652=EDGE_CURVE('',#4506,#4505,#873,.T.);
#5653=EDGE_CURVE('',#4507,#4506,#3649,.T.);
#5654=EDGE_CURVE('',#4508,#4507,#874,.T.);
#5655=EDGE_CURVE('',#4509,#4508,#875,.T.);
#5656=EDGE_CURVE('',#4510,#4509,#876,.T.);
#5657=EDGE_CURVE('',#4511,#4510,#3650,.T.);
#5658=EDGE_CURVE('',#4512,#4511,#877,.T.);
#5659=EDGE_CURVE('',#4513,#4512,#878,.T.);
#5660=EDGE_CURVE('',#4514,#4513,#879,.T.);
#5661=EDGE_CURVE('',#4515,#4514,#3651,.T.);
#5662=EDGE_CURVE('',#4516,#4515,#880,.T.);
#5663=EDGE_CURVE('',#4517,#4516,#881,.T.);
#5664=EDGE_CURVE('',#4518,#4517,#882,.T.);
#5665=EDGE_CURVE('',#4519,#4518,#3652,.T.);
#5666=EDGE_CURVE('',#4520,#4519,#883,.T.);
#5667=EDGE_CURVE('',#4521,#4520,#884,.T.);
#5668=EDGE_CURVE('',#4522,#4521,#885,.T.);
#5669=EDGE_CURVE('',#4523,#4522,#3653,.T.);
#5670=EDGE_CURVE('',#4524,#4523,#886,.T.);
#5671=EDGE_CURVE('',#4525,#4524,#887,.T.);
#5672=EDGE_CURVE('',#4526,#4525,#888,.T.);
#5673=EDGE_CURVE('',#4527,#4526,#3654,.T.);
#5674=EDGE_CURVE('',#4528,#4527,#889,.T.);
#5675=EDGE_CURVE('',#4529,#4528,#890,.T.);
#5676=EDGE_CURVE('',#4530,#4529,#891,.T.);
#5677=EDGE_CURVE('',#4531,#4530,#3655,.T.);
#5678=EDGE_CURVE('',#4532,#4531,#892,.T.);
#5679=EDGE_CURVE('',#4533,#4532,#893,.T.);
#5680=EDGE_CURVE('',#4534,#4533,#894,.T.);
#5681=EDGE_CURVE('',#4535,#4534,#3656,.T.);
#5682=EDGE_CURVE('',#4536,#4535,#895,.T.);
#5683=EDGE_CURVE('',#4537,#4536,#896,.T.);
#5684=EDGE_CURVE('',#4538,#4537,#897,.T.);
#5685=EDGE_CURVE('',#4539,#4538,#3657,.T.);
#5686=EDGE_CURVE('',#4540,#4539,#898,.T.);
#5687=EDGE_CURVE('',#4541,#4540,#899,.T.);
#5688=EDGE_CURVE('',#4542,#4541,#900,.T.);
#5689=EDGE_CURVE('',#4543,#4542,#3658,.T.);
#5690=EDGE_CURVE('',#4544,#4543,#901,.T.);
#5691=EDGE_CURVE('',#4545,#4544,#902,.T.);
#5692=EDGE_CURVE('',#4546,#4545,#903,.T.);
#5693=EDGE_CURVE('',#4547,#4546,#3659,.T.);
#5694=EDGE_CURVE('',#4548,#4547,#904,.T.);
#5695=EDGE_CURVE('',#4549,#4548,#905,.T.);
#5696=EDGE_CURVE('',#4550,#4549,#906,.T.);
#5697=EDGE_CURVE('',#4551,#4550,#3660,.T.);
#5698=EDGE_CURVE('',#4552,#4551,#907,.T.);
#5699=EDGE_CURVE('',#4553,#4552,#908,.T.);
#5700=EDGE_CURVE('',#4554,#4553,#909,.T.);
#5701=EDGE_CURVE('',#4555,#4554,#3661,.T.);
#5702=EDGE_CURVE('',#4556,#4555,#910,.T.);
#5703=EDGE_CURVE('',#4557,#4556,#911,.T.);
#5704=EDGE_CURVE('',#4558,#4557,#912,.T.);
#5705=EDGE_CURVE('',#4559,#4558,#3662,.T.);
#5706=EDGE_CURVE('',#4560,#4559,#913,.T.);
#5707=EDGE_CURVE('',#4561,#4560,#914,.T.);
#5708=EDGE_CURVE('',#4562,#4561,#915,.T.);
#5709=EDGE_CURVE('',#4563,#4562,#3663,.T.);
#5710=EDGE_CURVE('',#4564,#4563,#916,.T.);
#5711=EDGE_CURVE('',#4565,#4564,#917,.T.);
#5712=EDGE_CURVE('',#4566,#4565,#918,.T.);
#5713=EDGE_CURVE('',#4567,#4566,#3664,.T.);
#5714=EDGE_CURVE('',#4568,#4567,#919,.T.);
#5715=EDGE_CURVE('',#4569,#4568,#920,.T.);
#5716=EDGE_CURVE('',#4570,#4569,#921,.T.);
#5717=EDGE_CURVE('',#4571,#4570,#3665,.T.);
#5718=EDGE_CURVE('',#4572,#4571,#922,.T.);
#5719=EDGE_CURVE('',#4573,#4572,#923,.T.);
#5720=EDGE_CURVE('',#4574,#4573,#924,.T.);
#5721=EDGE_CURVE('',#4575,#4574,#3666,.T.);
#5722=EDGE_CURVE('',#4399,#4575,#925,.T.);
#5723=EDGE_CURVE('',#4576,#4577,#3667,.T.);
#5724=EDGE_CURVE('',#4577,#4578,#2990,.T.);
#5725=EDGE_CURVE('',#4579,#4578,#3668,.T.);
#5726=EDGE_CURVE('',#4576,#4579,#2991,.T.);
#5727=EDGE_CURVE('',#4580,#4581,#926,.F.);
#5728=EDGE_CURVE('',#4581,#4582,#927,.T.);
#5729=EDGE_CURVE('',#4583,#4582,#3669,.T.);
#5730=EDGE_CURVE('',#4583,#4584,#928,.T.);
#5731=EDGE_CURVE('',#4584,#4585,#929,.T.);
#5732=EDGE_CURVE('',#4585,#4586,#930,.T.);
#5733=EDGE_CURVE('',#4587,#4586,#3670,.T.);
#5734=EDGE_CURVE('',#4587,#4588,#931,.T.);
#5735=EDGE_CURVE('',#4588,#4589,#932,.T.);
#5736=EDGE_CURVE('',#4589,#4590,#933,.T.);
#5737=EDGE_CURVE('',#4591,#4590,#3671,.T.);
#5738=EDGE_CURVE('',#4591,#4592,#934,.T.);
#5739=EDGE_CURVE('',#4592,#4593,#935,.T.);
#5740=EDGE_CURVE('',#4593,#4594,#936,.T.);
#5741=EDGE_CURVE('',#4595,#4594,#3672,.T.);
#5742=EDGE_CURVE('',#4595,#4596,#937,.T.);
#5743=EDGE_CURVE('',#4596,#4597,#938,.T.);
#5744=EDGE_CURVE('',#4597,#4598,#939,.T.);
#5745=EDGE_CURVE('',#4599,#4598,#3673,.T.);
#5746=EDGE_CURVE('',#4599,#4600,#940,.T.);
#5747=EDGE_CURVE('',#4600,#4601,#941,.T.);
#5748=EDGE_CURVE('',#4601,#4602,#942,.T.);
#5749=EDGE_CURVE('',#4603,#4602,#3674,.T.);
#5750=EDGE_CURVE('',#4603,#4604,#943,.T.);
#5751=EDGE_CURVE('',#4604,#4605,#944,.T.);
#5752=EDGE_CURVE('',#4605,#4606,#945,.T.);
#5753=EDGE_CURVE('',#4607,#4606,#3675,.T.);
#5754=EDGE_CURVE('',#4607,#4608,#946,.T.);
#5755=EDGE_CURVE('',#4608,#4609,#947,.T.);
#5756=EDGE_CURVE('',#4609,#4610,#948,.T.);
#5757=EDGE_CURVE('',#4611,#4610,#3676,.T.);
#5758=EDGE_CURVE('',#4611,#4612,#949,.T.);
#5759=EDGE_CURVE('',#4612,#4613,#950,.T.);
#5760=EDGE_CURVE('',#4613,#4614,#951,.T.);
#5761=EDGE_CURVE('',#4615,#4614,#3677,.T.);
#5762=EDGE_CURVE('',#4615,#4616,#952,.T.);
#5763=EDGE_CURVE('',#4616,#4617,#953,.T.);
#5764=EDGE_CURVE('',#4617,#4618,#954,.T.);
#5765=EDGE_CURVE('',#4619,#4618,#3678,.T.);
#5766=EDGE_CURVE('',#4619,#4620,#955,.T.);
#5767=EDGE_CURVE('',#4620,#4621,#956,.T.);
#5768=EDGE_CURVE('',#4621,#4622,#957,.T.);
#5769=EDGE_CURVE('',#4623,#4622,#3679,.T.);
#5770=EDGE_CURVE('',#4623,#4624,#958,.T.);
#5771=EDGE_CURVE('',#4624,#4625,#959,.T.);
#5772=EDGE_CURVE('',#4625,#4626,#960,.T.);
#5773=EDGE_CURVE('',#4627,#4626,#3680,.T.);
#5774=EDGE_CURVE('',#4627,#4628,#961,.T.);
#5775=EDGE_CURVE('',#4628,#4629,#962,.T.);
#5776=EDGE_CURVE('',#4629,#4630,#963,.T.);
#5777=EDGE_CURVE('',#4631,#4630,#3681,.T.);
#5778=EDGE_CURVE('',#4631,#4632,#964,.T.);
#5779=EDGE_CURVE('',#4632,#4633,#965,.T.);
#5780=EDGE_CURVE('',#4633,#4634,#966,.T.);
#5781=EDGE_CURVE('',#4635,#4634,#3682,.T.);
#5782=EDGE_CURVE('',#4635,#4636,#967,.T.);
#5783=EDGE_CURVE('',#4636,#4637,#968,.T.);
#5784=EDGE_CURVE('',#4637,#4638,#969,.T.);
#5785=EDGE_CURVE('',#4639,#4638,#3683,.T.);
#5786=EDGE_CURVE('',#4639,#4640,#970,.T.);
#5787=EDGE_CURVE('',#4640,#4641,#971,.T.);
#5788=EDGE_CURVE('',#4641,#4642,#972,.T.);
#5789=EDGE_CURVE('',#4643,#4642,#3684,.T.);
#5790=EDGE_CURVE('',#4643,#4644,#973,.T.);
#5791=EDGE_CURVE('',#4644,#4645,#974,.T.);
#5792=EDGE_CURVE('',#4645,#4646,#975,.T.);
#5793=EDGE_CURVE('',#4647,#4646,#3685,.T.);
#5794=EDGE_CURVE('',#4647,#4648,#976,.T.);
#5795=EDGE_CURVE('',#4648,#4649,#977,.T.);
#5796=EDGE_CURVE('',#4649,#4650,#978,.T.);
#5797=EDGE_CURVE('',#4651,#4650,#3686,.T.);
#5798=EDGE_CURVE('',#4651,#4652,#979,.T.);
#5799=EDGE_CURVE('',#4652,#4653,#980,.T.);
#5800=EDGE_CURVE('',#4653,#4654,#981,.T.);
#5801=EDGE_CURVE('',#4655,#4654,#3687,.T.);
#5802=EDGE_CURVE('',#4655,#4656,#982,.T.);
#5803=EDGE_CURVE('',#4656,#4657,#983,.T.);
#5804=EDGE_CURVE('',#4657,#4658,#984,.T.);
#5805=EDGE_CURVE('',#4659,#4658,#3688,.T.);
#5806=EDGE_CURVE('',#4659,#4660,#985,.T.);
#5807=EDGE_CURVE('',#4660,#4661,#986,.T.);
#5808=EDGE_CURVE('',#4661,#4662,#987,.T.);
#5809=EDGE_CURVE('',#4663,#4662,#3689,.T.);
#5810=EDGE_CURVE('',#4663,#4664,#988,.T.);
#5811=EDGE_CURVE('',#4664,#4665,#989,.T.);
#5812=EDGE_CURVE('',#4665,#4666,#990,.T.);
#5813=EDGE_CURVE('',#4667,#4666,#3690,.T.);
#5814=EDGE_CURVE('',#4667,#4668,#991,.T.);
#5815=EDGE_CURVE('',#4668,#4669,#992,.T.);
#5816=EDGE_CURVE('',#4669,#4670,#2992,.T.);
#5817=EDGE_CURVE('',#4670,#4670,#3691,.T.);
#5818=EDGE_CURVE('',#4669,#4671,#993,.T.);
#5819=EDGE_CURVE('',#4671,#4672,#994,.T.);
#5820=EDGE_CURVE('',#4673,#4672,#3692,.T.);
#5821=EDGE_CURVE('',#4673,#4674,#995,.T.);
#5822=EDGE_CURVE('',#4674,#4675,#996,.T.);
#5823=EDGE_CURVE('',#4675,#4676,#997,.T.);
#5824=EDGE_CURVE('',#4677,#4676,#3693,.T.);
#5825=EDGE_CURVE('',#4677,#4678,#998,.T.);
#5826=EDGE_CURVE('',#4678,#4679,#999,.T.);
#5827=EDGE_CURVE('',#4679,#4680,#1000,.T.);
#5828=EDGE_CURVE('',#4681,#4680,#3694,.T.);
#5829=EDGE_CURVE('',#4681,#4682,#1001,.T.);
#5830=EDGE_CURVE('',#4682,#4683,#1002,.T.);
#5831=EDGE_CURVE('',#4683,#4684,#1003,.T.);
#5832=EDGE_CURVE('',#4685,#4684,#3695,.T.);
#5833=EDGE_CURVE('',#4685,#4686,#1004,.T.);
#5834=EDGE_CURVE('',#4686,#4687,#1005,.T.);
#5835=EDGE_CURVE('',#4687,#4688,#1006,.T.);
#5836=EDGE_CURVE('',#4689,#4688,#3696,.T.);
#5837=EDGE_CURVE('',#4689,#4690,#1007,.T.);
#5838=EDGE_CURVE('',#4690,#4691,#1008,.T.);
#5839=EDGE_CURVE('',#4691,#4692,#1009,.T.);
#5840=EDGE_CURVE('',#4693,#4692,#3697,.T.);
#5841=EDGE_CURVE('',#4693,#4694,#1010,.T.);
#5842=EDGE_CURVE('',#4694,#4695,#1011,.T.);
#5843=EDGE_CURVE('',#4695,#4696,#1012,.T.);
#5844=EDGE_CURVE('',#4697,#4696,#3698,.T.);
#5845=EDGE_CURVE('',#4697,#4698,#1013,.T.);
#5846=EDGE_CURVE('',#4698,#4699,#1014,.T.);
#5847=EDGE_CURVE('',#4699,#4700,#1015,.T.);
#5848=EDGE_CURVE('',#4701,#4700,#3699,.T.);
#5849=EDGE_CURVE('',#4701,#4702,#1016,.T.);
#5850=EDGE_CURVE('',#4702,#4703,#1017,.T.);
#5851=EDGE_CURVE('',#4703,#4704,#1018,.T.);
#5852=EDGE_CURVE('',#4705,#4704,#3700,.T.);
#5853=EDGE_CURVE('',#4705,#4706,#1019,.T.);
#5854=EDGE_CURVE('',#4706,#4707,#1020,.T.);
#5855=EDGE_CURVE('',#4707,#4708,#1021,.T.);
#5856=EDGE_CURVE('',#4709,#4708,#3701,.T.);
#5857=EDGE_CURVE('',#4709,#4710,#1022,.T.);
#5858=EDGE_CURVE('',#4710,#4711,#1023,.T.);
#5859=EDGE_CURVE('',#4711,#4712,#1024,.T.);
#5860=EDGE_CURVE('',#4713,#4712,#3702,.T.);
#5861=EDGE_CURVE('',#4713,#4714,#1025,.T.);
#5862=EDGE_CURVE('',#4714,#4715,#1026,.T.);
#5863=EDGE_CURVE('',#4715,#4716,#1027,.T.);
#5864=EDGE_CURVE('',#4717,#4716,#3703,.T.);
#5865=EDGE_CURVE('',#4717,#4718,#1028,.T.);
#5866=EDGE_CURVE('',#4718,#4719,#1029,.T.);
#5867=EDGE_CURVE('',#4719,#4720,#1030,.T.);
#5868=EDGE_CURVE('',#4721,#4720,#3704,.T.);
#5869=EDGE_CURVE('',#4721,#4722,#1031,.T.);
#5870=EDGE_CURVE('',#4722,#4723,#1032,.T.);
#5871=EDGE_CURVE('',#4723,#4724,#1033,.T.);
#5872=EDGE_CURVE('',#4725,#4724,#3705,.T.);
#5873=EDGE_CURVE('',#4725,#4726,#1034,.T.);
#5874=EDGE_CURVE('',#4726,#4727,#1035,.T.);
#5875=EDGE_CURVE('',#4727,#4728,#1036,.T.);
#5876=EDGE_CURVE('',#4729,#4728,#3706,.T.);
#5877=EDGE_CURVE('',#4729,#4730,#1037,.T.);
#5878=EDGE_CURVE('',#4730,#4731,#1038,.T.);
#5879=EDGE_CURVE('',#4731,#4732,#1039,.T.);
#5880=EDGE_CURVE('',#4733,#4732,#3707,.T.);
#5881=EDGE_CURVE('',#4733,#4734,#1040,.T.);
#5882=EDGE_CURVE('',#4734,#4735,#1041,.T.);
#5883=EDGE_CURVE('',#4735,#4736,#1042,.T.);
#5884=EDGE_CURVE('',#4737,#4736,#3708,.T.);
#5885=EDGE_CURVE('',#4737,#4738,#1043,.T.);
#5886=EDGE_CURVE('',#4738,#4739,#1044,.T.);
#5887=EDGE_CURVE('',#4739,#4740,#1045,.T.);
#5888=EDGE_CURVE('',#4741,#4740,#3709,.T.);
#5889=EDGE_CURVE('',#4741,#4742,#1046,.T.);
#5890=EDGE_CURVE('',#4742,#4743,#1047,.T.);
#5891=EDGE_CURVE('',#4743,#4744,#1048,.T.);
#5892=EDGE_CURVE('',#4745,#4744,#3710,.T.);
#5893=EDGE_CURVE('',#4745,#4746,#1049,.T.);
#5894=EDGE_CURVE('',#4746,#4747,#1050,.T.);
#5895=EDGE_CURVE('',#4747,#4748,#1051,.T.);
#5896=EDGE_CURVE('',#4749,#4748,#3711,.T.);
#5897=EDGE_CURVE('',#4749,#4750,#1052,.T.);
#5898=EDGE_CURVE('',#4750,#4751,#1053,.T.);
#5899=EDGE_CURVE('',#4751,#4752,#1054,.T.);
#5900=EDGE_CURVE('',#4753,#4752,#3712,.T.);
#5901=EDGE_CURVE('',#4753,#4754,#1055,.T.);
#5902=EDGE_CURVE('',#4754,#4755,#1056,.T.);
#5903=EDGE_CURVE('',#4755,#4756,#1057,.T.);
#5904=EDGE_CURVE('',#4757,#4756,#3713,.T.);
#5905=EDGE_CURVE('',#4757,#4580,#1058,.T.);
#5906=EDGE_CURVE('',#4619,#4394,#1059,.T.);
#5907=EDGE_CURVE('',#4395,#4618,#1060,.T.);
#5908=EDGE_CURVE('',#4389,#4622,#1061,.T.);
#5909=EDGE_CURVE('',#4623,#4388,#1062,.T.);
#5910=EDGE_CURVE('',#4615,#4382,#1063,.T.);
#5911=EDGE_CURVE('',#4383,#4614,#1064,.T.);
#5912=EDGE_CURVE('',#4611,#4376,#1065,.T.);
#5913=EDGE_CURVE('',#4377,#4610,#1066,.T.);
#5914=EDGE_CURVE('',#4607,#4370,#1067,.T.);
#5915=EDGE_CURVE('',#4371,#4606,#1068,.T.);
#5916=EDGE_CURVE('',#4603,#4364,#1069,.T.);
#5917=EDGE_CURVE('',#4365,#4602,#1070,.T.);
#5918=EDGE_CURVE('',#4599,#4358,#1071,.T.);
#5919=EDGE_CURVE('',#4359,#4598,#1072,.T.);
#5920=EDGE_CURVE('',#4595,#4352,#1073,.T.);
#5921=EDGE_CURVE('',#4353,#4594,#1074,.T.);
#5922=EDGE_CURVE('',#4591,#4346,#1075,.T.);
#5923=EDGE_CURVE('',#4347,#4590,#1076,.T.);
#5924=EDGE_CURVE('',#4587,#4340,#1077,.T.);
#5925=EDGE_CURVE('',#4341,#4586,#1078,.T.);
#5926=EDGE_CURVE('',#4583,#4334,#1079,.T.);
#5927=EDGE_CURVE('',#4335,#4582,#1080,.T.);
#5928=EDGE_CURVE('',#4757,#4328,#1081,.T.);
#5929=EDGE_CURVE('',#4329,#4756,#1082,.T.);
#5930=EDGE_CURVE('',#4753,#4322,#1083,.T.);
#5931=EDGE_CURVE('',#4323,#4752,#1084,.T.);
#5932=EDGE_CURVE('',#4749,#4316,#1085,.T.);
#5933=EDGE_CURVE('',#4317,#4748,#1086,.T.);
#5934=EDGE_CURVE('',#4745,#4310,#1087,.T.);
#5935=EDGE_CURVE('',#4311,#4744,#1088,.T.);
#5936=EDGE_CURVE('',#4741,#4304,#1089,.T.);
#5937=EDGE_CURVE('',#4305,#4740,#1090,.T.);
#5938=EDGE_CURVE('',#4737,#4298,#1091,.T.);
#5939=EDGE_CURVE('',#4299,#4736,#1092,.T.);
#5940=EDGE_CURVE('',#4733,#4292,#1093,.T.);
#5941=EDGE_CURVE('',#4293,#4732,#1094,.T.);
#5942=EDGE_CURVE('',#4729,#4286,#1095,.T.);
#5943=EDGE_CURVE('',#4287,#4728,#1096,.T.);
#5944=EDGE_CURVE('',#4725,#4280,#1097,.T.);
#5945=EDGE_CURVE('',#4281,#4724,#1098,.T.);
#5946=EDGE_CURVE('',#4721,#4274,#1099,.T.);
#5947=EDGE_CURVE('',#4275,#4720,#1100,.T.);
#5948=EDGE_CURVE('',#4717,#4268,#1101,.T.);
#5949=EDGE_CURVE('',#4269,#4716,#1102,.T.);
#5950=EDGE_CURVE('',#4713,#4262,#1103,.T.);
#5951=EDGE_CURVE('',#4263,#4712,#1104,.T.);
#5952=EDGE_CURVE('',#4709,#4256,#1105,.T.);
#5953=EDGE_CURVE('',#4257,#4708,#1106,.T.);
#5954=EDGE_CURVE('',#4705,#4250,#1107,.T.);
#5955=EDGE_CURVE('',#4251,#4704,#1108,.T.);
#5956=EDGE_CURVE('',#4701,#4244,#1109,.T.);
#5957=EDGE_CURVE('',#4245,#4700,#1110,.T.);
#5958=EDGE_CURVE('',#4697,#4238,#1111,.T.);
#5959=EDGE_CURVE('',#4239,#4696,#1112,.T.);
#5960=EDGE_CURVE('',#4693,#4232,#1113,.T.);
#5961=EDGE_CURVE('',#4233,#4692,#1114,.T.);
#5962=EDGE_CURVE('',#4689,#4226,#1115,.T.);
#5963=EDGE_CURVE('',#4227,#4688,#1116,.T.);
#5964=EDGE_CURVE('',#4685,#4220,#1117,.T.);
#5965=EDGE_CURVE('',#4221,#4684,#1118,.T.);
#5966=EDGE_CURVE('',#4681,#4214,#1119,.T.);
#5967=EDGE_CURVE('',#4215,#4680,#1120,.T.);
#5968=EDGE_CURVE('',#4677,#4208,#1121,.T.);
#5969=EDGE_CURVE('',#4209,#4676,#1122,.T.);
#5970=EDGE_CURVE('',#4673,#4202,#1123,.T.);
#5971=EDGE_CURVE('',#4203,#4672,#1124,.T.);
#5972=EDGE_CURVE('',#4667,#4196,#1125,.T.);
#5973=EDGE_CURVE('',#4197,#4666,#1126,.T.);
#5974=EDGE_CURVE('',#4663,#4190,#1127,.T.);
#5975=EDGE_CURVE('',#4191,#4662,#1128,.T.);
#5976=EDGE_CURVE('',#4659,#4184,#1129,.T.);
#5977=EDGE_CURVE('',#4185,#4658,#1130,.T.);
#5978=EDGE_CURVE('',#4655,#4178,#1131,.T.);
#5979=EDGE_CURVE('',#4179,#4654,#1132,.T.);
#5980=EDGE_CURVE('',#4651,#4172,#1133,.T.);
#5981=EDGE_CURVE('',#4173,#4650,#1134,.T.);
#5982=EDGE_CURVE('',#4647,#4166,#1135,.T.);
#5983=EDGE_CURVE('',#4167,#4646,#1136,.T.);
#5984=EDGE_CURVE('',#4643,#4160,#1137,.T.);
#5985=EDGE_CURVE('',#4161,#4642,#1138,.T.);
#5986=EDGE_CURVE('',#4639,#4154,#1139,.T.);
#5987=EDGE_CURVE('',#4155,#4638,#1140,.T.);
#5988=EDGE_CURVE('',#4635,#4148,#1141,.T.);
#5989=EDGE_CURVE('',#4149,#4634,#1142,.T.);
#5990=EDGE_CURVE('',#4631,#4142,#1143,.T.);
#5991=EDGE_CURVE('',#4143,#4630,#1144,.T.);
#5992=EDGE_CURVE('',#4627,#4136,#1145,.T.);
#5993=EDGE_CURVE('',#4137,#4626,#1146,.T.);
#5994=EDGE_CURVE('',#4391,#4445,#1147,.T.);
#5995=EDGE_CURVE('',#4444,#4386,#1148,.T.);
#5996=EDGE_CURVE('',#4448,#4392,#1149,.T.);
#5997=EDGE_CURVE('',#4397,#4449,#1150,.T.);
#5998=EDGE_CURVE('',#4452,#4380,#1151,.T.);
#5999=EDGE_CURVE('',#4385,#4453,#1152,.T.);
#6000=EDGE_CURVE('',#4456,#4374,#1153,.T.);
#6001=EDGE_CURVE('',#4379,#4457,#1154,.T.);
#6002=EDGE_CURVE('',#4460,#4368,#1155,.T.);
#6003=EDGE_CURVE('',#4373,#4461,#1156,.T.);
#6004=EDGE_CURVE('',#4464,#4362,#1157,.T.);
#6005=EDGE_CURVE('',#4367,#4465,#1158,.T.);
#6006=EDGE_CURVE('',#4472,#4350,#1159,.T.);
#6007=EDGE_CURVE('',#4355,#4473,#1160,.T.);
#6008=EDGE_CURVE('',#4468,#4356,#1161,.T.);
#6009=EDGE_CURVE('',#4361,#4469,#1162,.T.);
#6010=EDGE_CURVE('',#4476,#4344,#1163,.T.);
#6011=EDGE_CURVE('',#4349,#4477,#1164,.T.);
#6012=EDGE_CURVE('',#4480,#4338,#1165,.T.);
#6013=EDGE_CURVE('',#4343,#4481,#1166,.T.);
#6014=EDGE_CURVE('',#4484,#4332,#1167,.T.);
#6015=EDGE_CURVE('',#4337,#4485,#1168,.T.);
#6016=EDGE_CURVE('',#4490,#4326,#1169,.T.);
#6017=EDGE_CURVE('',#4331,#4491,#1170,.T.);
#6018=EDGE_CURVE('',#4494,#4320,#1171,.T.);
#6019=EDGE_CURVE('',#4325,#4495,#1172,.T.);
#6020=EDGE_CURVE('',#4498,#4314,#1173,.T.);
#6021=EDGE_CURVE('',#4319,#4499,#1174,.T.);
#6022=EDGE_CURVE('',#4502,#4308,#1175,.T.);
#6023=EDGE_CURVE('',#4313,#4503,#1176,.T.);
#6024=EDGE_CURVE('',#4506,#4302,#1177,.T.);
#6025=EDGE_CURVE('',#4307,#4507,#1178,.T.);
#6026=EDGE_CURVE('',#4510,#4296,#1179,.T.);
#6027=EDGE_CURVE('',#4301,#4511,#1180,.T.);
#6028=EDGE_CURVE('',#4514,#4290,#1181,.T.);
#6029=EDGE_CURVE('',#4295,#4515,#1182,.T.);
#6030=EDGE_CURVE('',#4518,#4284,#1183,.T.);
#6031=EDGE_CURVE('',#4289,#4519,#1184,.T.);
#6032=EDGE_CURVE('',#4522,#4278,#1185,.T.);
#6033=EDGE_CURVE('',#4283,#4523,#1186,.T.);
#6034=EDGE_CURVE('',#4526,#4272,#1187,.T.);
#6035=EDGE_CURVE('',#4277,#4527,#1188,.T.);
#6036=EDGE_CURVE('',#4530,#4266,#1189,.T.);
#6037=EDGE_CURVE('',#4271,#4531,#1190,.T.);
#6038=EDGE_CURVE('',#4534,#4260,#1191,.T.);
#6039=EDGE_CURVE('',#4265,#4535,#1192,.T.);
#6040=EDGE_CURVE('',#4538,#4254,#1193,.T.);
#6041=EDGE_CURVE('',#4259,#4539,#1194,.T.);
#6042=EDGE_CURVE('',#4542,#4248,#1195,.T.);
#6043=EDGE_CURVE('',#4253,#4543,#1196,.T.);
#6044=EDGE_CURVE('',#4546,#4242,#1197,.T.);
#6045=EDGE_CURVE('',#4247,#4547,#1198,.T.);
#6046=EDGE_CURVE('',#4550,#4236,#1199,.T.);
#6047=EDGE_CURVE('',#4241,#4551,#1200,.T.);
#6048=EDGE_CURVE('',#4554,#4230,#1201,.T.);
#6049=EDGE_CURVE('',#4235,#4555,#1202,.T.);
#6050=EDGE_CURVE('',#4562,#4218,#1203,.T.);
#6051=EDGE_CURVE('',#4223,#4563,#1204,.T.);
#6052=EDGE_CURVE('',#4558,#4224,#1205,.T.);
#6053=EDGE_CURVE('',#4229,#4559,#1206,.T.);
#6054=EDGE_CURVE('',#4566,#4212,#1207,.T.);
#6055=EDGE_CURVE('',#4217,#4567,#1208,.T.);
#6056=EDGE_CURVE('',#4570,#4206,#1209,.T.);
#6057=EDGE_CURVE('',#4211,#4571,#1210,.T.);
#6058=EDGE_CURVE('',#4574,#4200,#1211,.T.);
#6059=EDGE_CURVE('',#4205,#4575,#1212,.T.);
#6060=EDGE_CURVE('',#4400,#4194,#1213,.T.);
#6061=EDGE_CURVE('',#4199,#4401,#1214,.T.);
#6062=EDGE_CURVE('',#4404,#4188,#1215,.T.);
#6063=EDGE_CURVE('',#4193,#4405,#1216,.T.);
#6064=EDGE_CURVE('',#4408,#4182,#1217,.T.);
#6065=EDGE_CURVE('',#4187,#4409,#1218,.T.);
#6066=EDGE_CURVE('',#4412,#4176,#1219,.T.);
#6067=EDGE_CURVE('',#4181,#4413,#1220,.T.);
#6068=EDGE_CURVE('',#4416,#4170,#1221,.T.);
#6069=EDGE_CURVE('',#4175,#4417,#1222,.T.);
#6070=EDGE_CURVE('',#4420,#4164,#1223,.T.);
#6071=EDGE_CURVE('',#4169,#4421,#1224,.T.);
#6072=EDGE_CURVE('',#4424,#4158,#1225,.T.);
#6073=EDGE_CURVE('',#4163,#4425,#1226,.T.);
#6074=EDGE_CURVE('',#4428,#4152,#1227,.T.);
#6075=EDGE_CURVE('',#4157,#4429,#1228,.T.);
#6076=EDGE_CURVE('',#4432,#4146,#1229,.T.);
#6077=EDGE_CURVE('',#4151,#4433,#1230,.T.);
#6078=EDGE_CURVE('',#4436,#4140,#1231,.T.);
#6079=EDGE_CURVE('',#4145,#4437,#1232,.T.);
#6080=EDGE_CURVE('',#4440,#4134,#1233,.T.);
#6081=EDGE_CURVE('',#4139,#4441,#1234,.T.);
#6082=EDGE_CURVE('',#4758,#4576,#2993,.T.);
#6083=EDGE_CURVE('',#4758,#4759,#2994,.T.);
#6084=EDGE_CURVE('',#4759,#4577,#2995,.T.);
#6085=EDGE_CURVE('',#4760,#4579,#2996,.T.);
#6086=EDGE_CURVE('',#4761,#4578,#2997,.T.);
#6087=EDGE_CURVE('',#4760,#4761,#2998,.T.);
#6088=EDGE_CURVE('',#4758,#4760,#2999,.T.);
#6089=EDGE_CURVE('',#4759,#4761,#3000,.T.);
#6090=EDGE_CURVE('',#4762,#4442,#1235,.T.);
#6091=EDGE_CURVE('',#4763,#4762,#3714,.T.);
#6092=EDGE_CURVE('',#4764,#4763,#3715,.T.);
#6093=EDGE_CURVE('',#4764,#4443,#232,.T.);
#6094=EDGE_CURVE('',#4387,#4764,#3716,.T.);
#6095=EDGE_CURVE('',#4762,#4138,#3717,.T.);
#6096=EDGE_CURVE('',#4764,#4624,#1236,.T.);
#6097=EDGE_CURVE('',#4762,#4625,#233,.T.);
#6098=EDGE_CURVE('',#4765,#4144,#3718,.T.);
#6099=EDGE_CURVE('',#4765,#4438,#1237,.T.);
#6100=EDGE_CURVE('',#4766,#4439,#234,.T.);
#6101=EDGE_CURVE('',#4135,#4766,#3719,.T.);
#6102=EDGE_CURVE('',#4767,#4765,#3720,.T.);
#6103=EDGE_CURVE('',#4766,#4767,#3721,.T.);
#6104=EDGE_CURVE('',#4768,#4150,#3722,.T.);
#6105=EDGE_CURVE('',#4768,#4434,#1238,.T.);
#6106=EDGE_CURVE('',#4769,#4435,#235,.T.);
#6107=EDGE_CURVE('',#4141,#4769,#3723,.T.);
#6108=EDGE_CURVE('',#4770,#4768,#3724,.T.);
#6109=EDGE_CURVE('',#4769,#4770,#3725,.T.);
#6110=EDGE_CURVE('',#4771,#4156,#3726,.T.);
#6111=EDGE_CURVE('',#4771,#4430,#236,.T.);
#6112=EDGE_CURVE('',#4772,#4431,#237,.T.);
#6113=EDGE_CURVE('',#4147,#4772,#3727,.T.);
#6114=EDGE_CURVE('',#4773,#4771,#3728,.T.);
#6115=EDGE_CURVE('',#4772,#4773,#3729,.T.);
#6116=EDGE_CURVE('',#4774,#4162,#3730,.T.);
#6117=EDGE_CURVE('',#4774,#4426,#1239,.T.);
#6118=EDGE_CURVE('',#4775,#4427,#238,.T.);
#6119=EDGE_CURVE('',#4153,#4775,#3731,.T.);
#6120=EDGE_CURVE('',#4776,#4774,#3732,.T.);
#6121=EDGE_CURVE('',#4775,#4776,#3733,.T.);
#6122=EDGE_CURVE('',#4777,#4168,#3734,.T.);
#6123=EDGE_CURVE('',#4777,#4422,#1240,.T.);
#6124=EDGE_CURVE('',#4778,#4423,#239,.T.);
#6125=EDGE_CURVE('',#4159,#4778,#3735,.T.);
#6126=EDGE_CURVE('',#4779,#4777,#3736,.T.);
#6127=EDGE_CURVE('',#4778,#4779,#3737,.T.);
#6128=EDGE_CURVE('',#4780,#4174,#3738,.T.);
#6129=EDGE_CURVE('',#4780,#4418,#1241,.T.);
#6130=EDGE_CURVE('',#4781,#4419,#240,.T.);
#6131=EDGE_CURVE('',#4165,#4781,#3739,.T.);
#6132=EDGE_CURVE('',#4782,#4780,#3740,.T.);
#6133=EDGE_CURVE('',#4781,#4782,#3741,.T.);
#6134=EDGE_CURVE('',#4783,#4180,#3742,.T.);
#6135=EDGE_CURVE('',#4783,#4414,#1242,.T.);
#6136=EDGE_CURVE('',#4784,#4415,#241,.T.);
#6137=EDGE_CURVE('',#4171,#4784,#3743,.T.);
#6138=EDGE_CURVE('',#4785,#4783,#3744,.T.);
#6139=EDGE_CURVE('',#4784,#4785,#3745,.T.);
#6140=EDGE_CURVE('',#4786,#4186,#3746,.T.);
#6141=EDGE_CURVE('',#4786,#4410,#1243,.T.);
#6142=EDGE_CURVE('',#4787,#4411,#242,.T.);
#6143=EDGE_CURVE('',#4177,#4787,#3747,.T.);
#6144=EDGE_CURVE('',#4788,#4786,#3748,.T.);
#6145=EDGE_CURVE('',#4787,#4788,#3749,.T.);
#6146=EDGE_CURVE('',#4789,#4192,#3750,.T.);
#6147=EDGE_CURVE('',#4789,#4406,#1244,.T.);
#6148=EDGE_CURVE('',#4790,#4407,#243,.T.);
#6149=EDGE_CURVE('',#4183,#4790,#3751,.T.);
#6150=EDGE_CURVE('',#4791,#4789,#3752,.T.);
#6151=EDGE_CURVE('',#4790,#4791,#3753,.T.);
#6152=EDGE_CURVE('',#4792,#4198,#3754,.T.);
#6153=EDGE_CURVE('',#4792,#4402,#1245,.T.);
#6154=EDGE_CURVE('',#4793,#4403,#244,.T.);
#6155=EDGE_CURVE('',#4189,#4793,#3755,.T.);
#6156=EDGE_CURVE('',#4794,#4792,#3756,.T.);
#6157=EDGE_CURVE('',#4793,#4794,#3757,.T.);
#6158=EDGE_CURVE('',#4795,#4204,#3758,.T.);
#6159=EDGE_CURVE('',#4795,#4399,#1246,.T.);
#6160=EDGE_CURVE('',#4796,#4398,#245,.T.);
#6161=EDGE_CURVE('',#4195,#4796,#3759,.T.);
#6162=EDGE_CURVE('',#4797,#4795,#3760,.T.);
#6163=EDGE_CURVE('',#4796,#4797,#3761,.T.);
#6164=EDGE_CURVE('',#4798,#4210,#3762,.T.);
#6165=EDGE_CURVE('',#4798,#4572,#246,.T.);
#6166=EDGE_CURVE('',#4799,#4573,#247,.T.);
#6167=EDGE_CURVE('',#4201,#4799,#3763,.T.);
#6168=EDGE_CURVE('',#4800,#4798,#3764,.T.);
#6169=EDGE_CURVE('',#4799,#4800,#3765,.T.);
#6170=EDGE_CURVE('',#4801,#4216,#3766,.T.);
#6171=EDGE_CURVE('',#4801,#4568,#1247,.T.);
#6172=EDGE_CURVE('',#4802,#4569,#248,.T.);
#6173=EDGE_CURVE('',#4207,#4802,#3767,.T.);
#6174=EDGE_CURVE('',#4803,#4801,#3768,.T.);
#6175=EDGE_CURVE('',#4802,#4803,#3769,.T.);
#6176=EDGE_CURVE('',#4804,#4222,#3770,.T.);
#6177=EDGE_CURVE('',#4804,#4564,#1248,.T.);
#6178=EDGE_CURVE('',#4805,#4565,#249,.T.);
#6179=EDGE_CURVE('',#4213,#4805,#3771,.T.);
#6180=EDGE_CURVE('',#4806,#4804,#3772,.T.);
#6181=EDGE_CURVE('',#4805,#4806,#3773,.T.);
#6182=EDGE_CURVE('',#4807,#4561,#250,.T.);
#6183=EDGE_CURVE('',#4219,#4807,#3774,.T.);
#6184=EDGE_CURVE('',#4808,#4228,#3775,.T.);
#6185=EDGE_CURVE('',#4808,#4560,#251,.T.);
#6186=EDGE_CURVE('',#4809,#4808,#3776,.T.);
#6187=EDGE_CURVE('',#4807,#4809,#3777,.T.);
#6188=EDGE_CURVE('',#4810,#4234,#3778,.T.);
#6189=EDGE_CURVE('',#4810,#4556,#1249,.T.);
#6190=EDGE_CURVE('',#4811,#4557,#252,.T.);
#6191=EDGE_CURVE('',#4225,#4811,#3779,.T.);
#6192=EDGE_CURVE('',#4812,#4810,#3780,.T.);
#6193=EDGE_CURVE('',#4811,#4812,#3781,.T.);
#6194=EDGE_CURVE('',#4813,#4240,#3782,.T.);
#6195=EDGE_CURVE('',#4813,#4552,#1250,.T.);
#6196=EDGE_CURVE('',#4814,#4553,#253,.T.);
#6197=EDGE_CURVE('',#4231,#4814,#3783,.T.);
#6198=EDGE_CURVE('',#4815,#4813,#3784,.T.);
#6199=EDGE_CURVE('',#4814,#4815,#3785,.T.);
#6200=EDGE_CURVE('',#4816,#4246,#3786,.T.);
#6201=EDGE_CURVE('',#4816,#4548,#1251,.T.);
#6202=EDGE_CURVE('',#4817,#4549,#254,.T.);
#6203=EDGE_CURVE('',#4237,#4817,#3787,.T.);
#6204=EDGE_CURVE('',#4818,#4816,#3788,.T.);
#6205=EDGE_CURVE('',#4817,#4818,#3789,.T.);
#6206=EDGE_CURVE('',#4819,#4252,#3790,.T.);
#6207=EDGE_CURVE('',#4819,#4544,#1252,.T.);
#6208=EDGE_CURVE('',#4820,#4545,#255,.T.);
#6209=EDGE_CURVE('',#4243,#4820,#3791,.T.);
#6210=EDGE_CURVE('',#4821,#4819,#3792,.T.);
#6211=EDGE_CURVE('',#4820,#4821,#3793,.T.);
#6212=EDGE_CURVE('',#4822,#4258,#3794,.T.);
#6213=EDGE_CURVE('',#4822,#4540,#1253,.T.);
#6214=EDGE_CURVE('',#4823,#4541,#256,.T.);
#6215=EDGE_CURVE('',#4249,#4823,#3795,.T.);
#6216=EDGE_CURVE('',#4824,#4822,#3796,.T.);
#6217=EDGE_CURVE('',#4823,#4824,#3797,.T.);
#6218=EDGE_CURVE('',#4825,#4264,#3798,.T.);
#6219=EDGE_CURVE('',#4825,#4536,#1254,.T.);
#6220=EDGE_CURVE('',#4826,#4537,#257,.T.);
#6221=EDGE_CURVE('',#4255,#4826,#3799,.T.);
#6222=EDGE_CURVE('',#4827,#4825,#3800,.T.);
#6223=EDGE_CURVE('',#4826,#4827,#3801,.T.);
#6224=EDGE_CURVE('',#4828,#4270,#3802,.T.);
#6225=EDGE_CURVE('',#4828,#4532,#1255,.T.);
#6226=EDGE_CURVE('',#4829,#4533,#258,.T.);
#6227=EDGE_CURVE('',#4261,#4829,#3803,.T.);
#6228=EDGE_CURVE('',#4830,#4828,#3804,.T.);
#6229=EDGE_CURVE('',#4829,#4830,#3805,.T.);
#6230=EDGE_CURVE('',#4831,#4276,#3806,.T.);
#6231=EDGE_CURVE('',#4831,#4528,#1256,.T.);
#6232=EDGE_CURVE('',#4832,#4529,#259,.T.);
#6233=EDGE_CURVE('',#4267,#4832,#3807,.T.);
#6234=EDGE_CURVE('',#4833,#4831,#3808,.T.);
#6235=EDGE_CURVE('',#4832,#4833,#3809,.T.);
#6236=EDGE_CURVE('',#4834,#4282,#3810,.T.);
#6237=EDGE_CURVE('',#4834,#4524,#1257,.T.);
#6238=EDGE_CURVE('',#4835,#4525,#260,.T.);
#6239=EDGE_CURVE('',#4273,#4835,#3811,.T.);
#6240=EDGE_CURVE('',#4836,#4834,#3812,.T.);
#6241=EDGE_CURVE('',#4835,#4836,#3813,.T.);
#6242=EDGE_CURVE('',#4837,#4288,#3814,.T.);
#6243=EDGE_CURVE('',#4837,#4520,#261,.T.);
#6244=EDGE_CURVE('',#4838,#4521,#262,.T.);
#6245=EDGE_CURVE('',#4279,#4838,#3815,.T.);
#6246=EDGE_CURVE('',#4839,#4837,#3816,.T.);
#6247=EDGE_CURVE('',#4838,#4839,#3817,.T.);
#6248=EDGE_CURVE('',#4840,#4294,#3818,.T.);
#6249=EDGE_CURVE('',#4840,#4516,#263,.T.);
#6250=EDGE_CURVE('',#4841,#4517,#264,.T.);
#6251=EDGE_CURVE('',#4285,#4841,#3819,.T.);
#6252=EDGE_CURVE('',#4842,#4840,#3820,.T.);
#6253=EDGE_CURVE('',#4841,#4842,#3821,.T.);
#6254=EDGE_CURVE('',#4843,#4300,#3822,.T.);
#6255=EDGE_CURVE('',#4843,#4512,#1258,.T.);
#6256=EDGE_CURVE('',#4844,#4513,#265,.T.);
#6257=EDGE_CURVE('',#4291,#4844,#3823,.T.);
#6258=EDGE_CURVE('',#4845,#4843,#3824,.T.);
#6259=EDGE_CURVE('',#4844,#4845,#3825,.T.);
#6260=EDGE_CURVE('',#4846,#4306,#3826,.T.);
#6261=EDGE_CURVE('',#4846,#4508,#1259,.T.);
#6262=EDGE_CURVE('',#4847,#4509,#266,.T.);
#6263=EDGE_CURVE('',#4297,#4847,#3827,.T.);
#6264=EDGE_CURVE('',#4848,#4846,#3828,.T.);
#6265=EDGE_CURVE('',#4847,#4848,#3829,.T.);
#6266=EDGE_CURVE('',#4849,#4312,#3830,.T.);
#6267=EDGE_CURVE('',#4849,#4504,#1260,.T.);
#6268=EDGE_CURVE('',#4850,#4505,#267,.T.);
#6269=EDGE_CURVE('',#4303,#4850,#3831,.T.);
#6270=EDGE_CURVE('',#4851,#4849,#3832,.T.);
#6271=EDGE_CURVE('',#4850,#4851,#3833,.T.);
#6272=EDGE_CURVE('',#4852,#4318,#3834,.T.);
#6273=EDGE_CURVE('',#4852,#4500,#1261,.T.);
#6274=EDGE_CURVE('',#4853,#4501,#268,.T.);
#6275=EDGE_CURVE('',#4309,#4853,#3835,.T.);
#6276=EDGE_CURVE('',#4854,#4852,#3836,.T.);
#6277=EDGE_CURVE('',#4853,#4854,#3837,.T.);
#6278=EDGE_CURVE('',#4855,#4324,#3838,.T.);
#6279=EDGE_CURVE('',#4855,#4496,#1262,.T.);
#6280=EDGE_CURVE('',#4856,#4497,#269,.T.);
#6281=EDGE_CURVE('',#4315,#4856,#3839,.T.);
#6282=EDGE_CURVE('',#4857,#4855,#3840,.T.);
#6283=EDGE_CURVE('',#4856,#4857,#3841,.T.);
#6284=EDGE_CURVE('',#4858,#4330,#3842,.T.);
#6285=EDGE_CURVE('',#4858,#4492,#1263,.T.);
#6286=EDGE_CURVE('',#4859,#4493,#270,.T.);
#6287=EDGE_CURVE('',#4321,#4859,#3843,.T.);
#6288=EDGE_CURVE('',#4860,#4858,#3844,.T.);
#6289=EDGE_CURVE('',#4859,#4860,#3845,.T.);
#6290=EDGE_CURVE('',#4861,#4336,#3846,.T.);
#6291=EDGE_CURVE('',#4861,#4486,#271,.T.);
#6292=EDGE_CURVE('',#4862,#4489,#272,.T.);
#6293=EDGE_CURVE('',#4327,#4862,#3847,.T.);
#6294=EDGE_CURVE('',#4863,#4861,#3848,.T.);
#6295=EDGE_CURVE('',#4862,#4863,#3849,.T.);
#6296=EDGE_CURVE('',#4864,#4342,#3850,.T.);
#6297=EDGE_CURVE('',#4864,#4482,#273,.T.);
#6298=EDGE_CURVE('',#4865,#4483,#274,.T.);
#6299=EDGE_CURVE('',#4333,#4865,#3851,.T.);
#6300=EDGE_CURVE('',#4866,#4864,#3852,.T.);
#6301=EDGE_CURVE('',#4865,#4866,#3853,.T.);
#6302=EDGE_CURVE('',#4867,#4348,#3854,.T.);
#6303=EDGE_CURVE('',#4867,#4478,#1264,.T.);
#6304=EDGE_CURVE('',#4868,#4479,#275,.T.);
#6305=EDGE_CURVE('',#4339,#4868,#3855,.T.);
#6306=EDGE_CURVE('',#4869,#4867,#3856,.T.);
#6307=EDGE_CURVE('',#4868,#4869,#3857,.T.);
#6308=EDGE_CURVE('',#4870,#4354,#3858,.T.);
#6309=EDGE_CURVE('',#4870,#4474,#1265,.T.);
#6310=EDGE_CURVE('',#4871,#4475,#276,.T.);
#6311=EDGE_CURVE('',#4345,#4871,#3859,.T.);
#6312=EDGE_CURVE('',#4872,#4870,#3860,.T.);
#6313=EDGE_CURVE('',#4871,#4872,#3861,.T.);
#6314=EDGE_CURVE('',#4873,#4471,#277,.T.);
#6315=EDGE_CURVE('',#4351,#4873,#3862,.T.);
#6316=EDGE_CURVE('',#4874,#4360,#3863,.T.);
#6317=EDGE_CURVE('',#4874,#4470,#278,.T.);
#6318=EDGE_CURVE('',#4875,#4874,#3864,.T.);
#6319=EDGE_CURVE('',#4873,#4875,#3865,.T.);
#6320=EDGE_CURVE('',#4876,#4366,#3866,.T.);
#6321=EDGE_CURVE('',#4876,#4466,#1266,.T.);
#6322=EDGE_CURVE('',#4877,#4467,#279,.T.);
#6323=EDGE_CURVE('',#4357,#4877,#3867,.T.);
#6324=EDGE_CURVE('',#4878,#4876,#3868,.T.);
#6325=EDGE_CURVE('',#4877,#4878,#3869,.T.);
#6326=EDGE_CURVE('',#4879,#4372,#3870,.T.);
#6327=EDGE_CURVE('',#4879,#4462,#1267,.T.);
#6328=EDGE_CURVE('',#4880,#4463,#280,.T.);
#6329=EDGE_CURVE('',#4363,#4880,#3871,.T.);
#6330=EDGE_CURVE('',#4881,#4879,#3872,.T.);
#6331=EDGE_CURVE('',#4880,#4881,#3873,.T.);
#6332=EDGE_CURVE('',#4882,#4378,#3874,.T.);
#6333=EDGE_CURVE('',#4882,#4458,#1268,.T.);
#6334=EDGE_CURVE('',#4883,#4459,#281,.T.);
#6335=EDGE_CURVE('',#4369,#4883,#3875,.T.);
#6336=EDGE_CURVE('',#4884,#4882,#3876,.T.);
#6337=EDGE_CURVE('',#4883,#4884,#3877,.T.);
#6338=EDGE_CURVE('',#4885,#4384,#3878,.T.);
#6339=EDGE_CURVE('',#4885,#4454,#1269,.T.);
#6340=EDGE_CURVE('',#4886,#4455,#282,.T.);
#6341=EDGE_CURVE('',#4375,#4886,#3879,.T.);
#6342=EDGE_CURVE('',#4887,#4885,#3880,.T.);
#6343=EDGE_CURVE('',#4886,#4887,#3881,.T.);
#6344=EDGE_CURVE('',#4888,#4396,#3882,.T.);
#6345=EDGE_CURVE('',#4888,#4450,#1270,.T.);
#6346=EDGE_CURVE('',#4889,#4451,#283,.T.);
#6347=EDGE_CURVE('',#4381,#4889,#3883,.T.);
#6348=EDGE_CURVE('',#4890,#4888,#3884,.T.);
#6349=EDGE_CURVE('',#4889,#4890,#3885,.T.);
#6350=EDGE_CURVE('',#4891,#4390,#3886,.T.);
#6351=EDGE_CURVE('',#4891,#4446,#284,.T.);
#6352=EDGE_CURVE('',#4892,#4447,#285,.T.);
#6353=EDGE_CURVE('',#4393,#4892,#3887,.T.);
#6354=EDGE_CURVE('',#4893,#4891,#3888,.T.);
#6355=EDGE_CURVE('',#4892,#4893,#3889,.T.);
#6356=EDGE_CURVE('',#4766,#4628,#1271,.T.);
#6357=EDGE_CURVE('',#4765,#4629,#286,.T.);
#6358=EDGE_CURVE('',#4769,#4632,#1272,.T.);
#6359=EDGE_CURVE('',#4768,#4633,#287,.T.);
#6360=EDGE_CURVE('',#4772,#4636,#1273,.T.);
#6361=EDGE_CURVE('',#4771,#4637,#1274,.T.);
#6362=EDGE_CURVE('',#4775,#4640,#1275,.T.);
#6363=EDGE_CURVE('',#4774,#4641,#288,.T.);
#6364=EDGE_CURVE('',#4778,#4644,#1276,.T.);
#6365=EDGE_CURVE('',#4777,#4645,#289,.T.);
#6366=EDGE_CURVE('',#4781,#4648,#1277,.T.);
#6367=EDGE_CURVE('',#4780,#4649,#290,.T.);
#6368=EDGE_CURVE('',#4784,#4652,#1278,.T.);
#6369=EDGE_CURVE('',#4783,#4653,#291,.T.);
#6370=EDGE_CURVE('',#4787,#4656,#1279,.T.);
#6371=EDGE_CURVE('',#4786,#4657,#292,.T.);
#6372=EDGE_CURVE('',#4790,#4660,#1280,.T.);
#6373=EDGE_CURVE('',#4789,#4661,#293,.T.);
#6374=EDGE_CURVE('',#4793,#4664,#1281,.T.);
#6375=EDGE_CURVE('',#4792,#4665,#294,.T.);
#6376=EDGE_CURVE('',#4796,#4668,#1282,.T.);
#6377=EDGE_CURVE('',#4795,#4671,#295,.T.);
#6378=EDGE_CURVE('',#4799,#4674,#1283,.T.);
#6379=EDGE_CURVE('',#4798,#4675,#1284,.T.);
#6380=EDGE_CURVE('',#4802,#4678,#1285,.T.);
#6381=EDGE_CURVE('',#4801,#4679,#296,.T.);
#6382=EDGE_CURVE('',#4805,#4682,#1286,.T.);
#6383=EDGE_CURVE('',#4804,#4683,#297,.T.);
#6384=EDGE_CURVE('',#4808,#4687,#298,.T.);
#6385=EDGE_CURVE('',#4807,#4686,#1287,.T.);
#6386=EDGE_CURVE('',#4811,#4690,#1288,.T.);
#6387=EDGE_CURVE('',#4810,#4691,#299,.T.);
#6388=EDGE_CURVE('',#4814,#4694,#1289,.T.);
#6389=EDGE_CURVE('',#4813,#4695,#300,.T.);
#6390=EDGE_CURVE('',#4817,#4698,#1290,.T.);
#6391=EDGE_CURVE('',#4816,#4699,#301,.T.);
#6392=EDGE_CURVE('',#4820,#4702,#1291,.T.);
#6393=EDGE_CURVE('',#4819,#4703,#302,.T.);
#6394=EDGE_CURVE('',#4823,#4706,#1292,.T.);
#6395=EDGE_CURVE('',#4822,#4707,#303,.T.);
#6396=EDGE_CURVE('',#4826,#4710,#1293,.T.);
#6397=EDGE_CURVE('',#4825,#4711,#304,.T.);
#6398=EDGE_CURVE('',#4829,#4714,#1294,.T.);
#6399=EDGE_CURVE('',#4828,#4715,#305,.T.);
#6400=EDGE_CURVE('',#4832,#4718,#1295,.T.);
#6401=EDGE_CURVE('',#4831,#4719,#306,.T.);
#6402=EDGE_CURVE('',#4835,#4722,#1296,.T.);
#6403=EDGE_CURVE('',#4834,#4723,#307,.T.);
#6404=EDGE_CURVE('',#4838,#4726,#1297,.T.);
#6405=EDGE_CURVE('',#4837,#4727,#1298,.T.);
#6406=EDGE_CURVE('',#4841,#4730,#1299,.T.);
#6407=EDGE_CURVE('',#4840,#4731,#1300,.T.);
#6408=EDGE_CURVE('',#4844,#4734,#1301,.T.);
#6409=EDGE_CURVE('',#4843,#4735,#308,.T.);
#6410=EDGE_CURVE('',#4847,#4738,#1302,.T.);
#6411=EDGE_CURVE('',#4846,#4739,#309,.T.);
#6412=EDGE_CURVE('',#4850,#4742,#1303,.T.);
#6413=EDGE_CURVE('',#4849,#4743,#310,.T.);
#6414=EDGE_CURVE('',#4853,#4746,#1304,.T.);
#6415=EDGE_CURVE('',#4852,#4747,#311,.T.);
#6416=EDGE_CURVE('',#4856,#4750,#1305,.T.);
#6417=EDGE_CURVE('',#4855,#4751,#312,.T.);
#6418=EDGE_CURVE('',#4859,#4754,#1306,.T.);
#6419=EDGE_CURVE('',#4858,#4755,#313,.T.);
#6420=EDGE_CURVE('',#4862,#4580,#1307,.T.);
#6421=EDGE_CURVE('',#4861,#4581,#1308,.T.);
#6422=EDGE_CURVE('',#4865,#4584,#1309,.T.);
#6423=EDGE_CURVE('',#4864,#4585,#1310,.T.);
#6424=EDGE_CURVE('',#4868,#4588,#1311,.T.);
#6425=EDGE_CURVE('',#4867,#4589,#314,.T.);
#6426=EDGE_CURVE('',#4871,#4592,#1312,.T.);
#6427=EDGE_CURVE('',#4870,#4593,#315,.T.);
#6428=EDGE_CURVE('',#4874,#4597,#316,.T.);
#6429=EDGE_CURVE('',#4873,#4596,#1313,.T.);
#6430=EDGE_CURVE('',#4877,#4600,#1314,.T.);
#6431=EDGE_CURVE('',#4876,#4601,#317,.T.);
#6432=EDGE_CURVE('',#4880,#4604,#1315,.T.);
#6433=EDGE_CURVE('',#4879,#4605,#318,.T.);
#6434=EDGE_CURVE('',#4883,#4608,#1316,.T.);
#6435=EDGE_CURVE('',#4882,#4609,#319,.T.);
#6436=EDGE_CURVE('',#4886,#4612,#1317,.T.);
#6437=EDGE_CURVE('',#4885,#4613,#320,.T.);
#6438=EDGE_CURVE('',#4889,#4616,#1318,.T.);
#6439=EDGE_CURVE('',#4888,#4617,#321,.T.);
#6440=EDGE_CURVE('',#4892,#4620,#1319,.T.);
#6441=EDGE_CURVE('',#4891,#4621,#1320,.T.);
#7139=ORIENTED_EDGE('',*,*,#5280,.T.);
#7140=ORIENTED_EDGE('',*,*,#5281,.F.);
#7141=ORIENTED_EDGE('',*,*,#5282,.F.);
#7142=ORIENTED_EDGE('',*,*,#5283,.F.);
#7143=ORIENTED_EDGE('',*,*,#5284,.T.);
#7144=ORIENTED_EDGE('',*,*,#5285,.F.);
#7145=ORIENTED_EDGE('',*,*,#5286,.T.);
#7146=ORIENTED_EDGE('',*,*,#5287,.F.);
#7147=ORIENTED_EDGE('',*,*,#5288,.F.);
#7148=ORIENTED_EDGE('',*,*,#5289,.F.);
#7149=ORIENTED_EDGE('',*,*,#5290,.T.);
#7150=ORIENTED_EDGE('',*,*,#5291,.F.);
#7151=ORIENTED_EDGE('',*,*,#5292,.T.);
#7152=ORIENTED_EDGE('',*,*,#5293,.F.);
#7153=ORIENTED_EDGE('',*,*,#5294,.F.);
#7154=ORIENTED_EDGE('',*,*,#5295,.F.);
#7155=ORIENTED_EDGE('',*,*,#5296,.T.);
#7156=ORIENTED_EDGE('',*,*,#5297,.F.);
#7157=ORIENTED_EDGE('',*,*,#5298,.T.);
#7158=ORIENTED_EDGE('',*,*,#5299,.F.);
#7159=ORIENTED_EDGE('',*,*,#5300,.F.);
#7160=ORIENTED_EDGE('',*,*,#5301,.F.);
#7161=ORIENTED_EDGE('',*,*,#5302,.T.);
#7162=ORIENTED_EDGE('',*,*,#5303,.F.);
#7163=ORIENTED_EDGE('',*,*,#5304,.T.);
#7164=ORIENTED_EDGE('',*,*,#5305,.F.);
#7165=ORIENTED_EDGE('',*,*,#5306,.F.);
#7166=ORIENTED_EDGE('',*,*,#5307,.F.);
#7167=ORIENTED_EDGE('',*,*,#5308,.T.);
#7168=ORIENTED_EDGE('',*,*,#5309,.F.);
#7169=ORIENTED_EDGE('',*,*,#5310,.T.);
#7170=ORIENTED_EDGE('',*,*,#5311,.F.);
#7171=ORIENTED_EDGE('',*,*,#5312,.F.);
#7172=ORIENTED_EDGE('',*,*,#5313,.F.);
#7173=ORIENTED_EDGE('',*,*,#5314,.T.);
#7174=ORIENTED_EDGE('',*,*,#5315,.F.);
#7175=ORIENTED_EDGE('',*,*,#5316,.T.);
#7176=ORIENTED_EDGE('',*,*,#5317,.F.);
#7177=ORIENTED_EDGE('',*,*,#5318,.F.);
#7178=ORIENTED_EDGE('',*,*,#5319,.F.);
#7179=ORIENTED_EDGE('',*,*,#5320,.T.);
#7180=ORIENTED_EDGE('',*,*,#5321,.F.);
#7181=ORIENTED_EDGE('',*,*,#5322,.T.);
#7182=ORIENTED_EDGE('',*,*,#5323,.F.);
#7183=ORIENTED_EDGE('',*,*,#5324,.F.);
#7184=ORIENTED_EDGE('',*,*,#5325,.F.);
#7185=ORIENTED_EDGE('',*,*,#5326,.T.);
#7186=ORIENTED_EDGE('',*,*,#5327,.F.);
#7187=ORIENTED_EDGE('',*,*,#5328,.T.);
#7188=ORIENTED_EDGE('',*,*,#5329,.F.);
#7189=ORIENTED_EDGE('',*,*,#5330,.F.);
#7190=ORIENTED_EDGE('',*,*,#5331,.F.);
#7191=ORIENTED_EDGE('',*,*,#5332,.T.);
#7192=ORIENTED_EDGE('',*,*,#5333,.F.);
#7193=ORIENTED_EDGE('',*,*,#5334,.T.);
#7194=ORIENTED_EDGE('',*,*,#5335,.F.);
#7195=ORIENTED_EDGE('',*,*,#5336,.F.);
#7196=ORIENTED_EDGE('',*,*,#5337,.F.);
#7197=ORIENTED_EDGE('',*,*,#5338,.T.);
#7198=ORIENTED_EDGE('',*,*,#5339,.F.);
#7199=ORIENTED_EDGE('',*,*,#5340,.T.);
#7200=ORIENTED_EDGE('',*,*,#5341,.F.);
#7201=ORIENTED_EDGE('',*,*,#5342,.F.);
#7202=ORIENTED_EDGE('',*,*,#5343,.F.);
#7203=ORIENTED_EDGE('',*,*,#5344,.T.);
#7204=ORIENTED_EDGE('',*,*,#5345,.F.);
#7205=ORIENTED_EDGE('',*,*,#5346,.T.);
#7206=ORIENTED_EDGE('',*,*,#5347,.F.);
#7207=ORIENTED_EDGE('',*,*,#5348,.F.);
#7208=ORIENTED_EDGE('',*,*,#5349,.F.);
#7209=ORIENTED_EDGE('',*,*,#5350,.T.);
#7210=ORIENTED_EDGE('',*,*,#5351,.F.);
#7211=ORIENTED_EDGE('',*,*,#5352,.T.);
#7212=ORIENTED_EDGE('',*,*,#5353,.F.);
#7213=ORIENTED_EDGE('',*,*,#5354,.F.);
#7214=ORIENTED_EDGE('',*,*,#5355,.F.);
#7215=ORIENTED_EDGE('',*,*,#5356,.T.);
#7216=ORIENTED_EDGE('',*,*,#5357,.F.);
#7217=ORIENTED_EDGE('',*,*,#5358,.T.);
#7218=ORIENTED_EDGE('',*,*,#5359,.F.);
#7219=ORIENTED_EDGE('',*,*,#5360,.F.);
#7220=ORIENTED_EDGE('',*,*,#5361,.F.);
#7221=ORIENTED_EDGE('',*,*,#5362,.T.);
#7222=ORIENTED_EDGE('',*,*,#5363,.F.);
#7223=ORIENTED_EDGE('',*,*,#5364,.T.);
#7224=ORIENTED_EDGE('',*,*,#5365,.F.);
#7225=ORIENTED_EDGE('',*,*,#5366,.F.);
#7226=ORIENTED_EDGE('',*,*,#5367,.F.);
#7227=ORIENTED_EDGE('',*,*,#5368,.T.);
#7228=ORIENTED_EDGE('',*,*,#5369,.F.);
#7229=ORIENTED_EDGE('',*,*,#5370,.T.);
#7230=ORIENTED_EDGE('',*,*,#5371,.F.);
#7231=ORIENTED_EDGE('',*,*,#5372,.F.);
#7232=ORIENTED_EDGE('',*,*,#5373,.F.);
#7233=ORIENTED_EDGE('',*,*,#5374,.T.);
#7234=ORIENTED_EDGE('',*,*,#5375,.F.);
#7235=ORIENTED_EDGE('',*,*,#5376,.T.);
#7236=ORIENTED_EDGE('',*,*,#5377,.F.);
#7237=ORIENTED_EDGE('',*,*,#5378,.F.);
#7238=ORIENTED_EDGE('',*,*,#5379,.F.);
#7239=ORIENTED_EDGE('',*,*,#5380,.T.);
#7240=ORIENTED_EDGE('',*,*,#5381,.F.);
#7241=ORIENTED_EDGE('',*,*,#5382,.T.);
#7242=ORIENTED_EDGE('',*,*,#5383,.F.);
#7243=ORIENTED_EDGE('',*,*,#5384,.F.);
#7244=ORIENTED_EDGE('',*,*,#5385,.F.);
#7245=ORIENTED_EDGE('',*,*,#5386,.T.);
#7246=ORIENTED_EDGE('',*,*,#5387,.F.);
#7247=ORIENTED_EDGE('',*,*,#5388,.T.);
#7248=ORIENTED_EDGE('',*,*,#5389,.F.);
#7249=ORIENTED_EDGE('',*,*,#5390,.F.);
#7250=ORIENTED_EDGE('',*,*,#5391,.F.);
#7251=ORIENTED_EDGE('',*,*,#5392,.T.);
#7252=ORIENTED_EDGE('',*,*,#5393,.F.);
#7253=ORIENTED_EDGE('',*,*,#5394,.T.);
#7254=ORIENTED_EDGE('',*,*,#5395,.F.);
#7255=ORIENTED_EDGE('',*,*,#5396,.F.);
#7256=ORIENTED_EDGE('',*,*,#5397,.F.);
#7257=ORIENTED_EDGE('',*,*,#5398,.T.);
#7258=ORIENTED_EDGE('',*,*,#5399,.F.);
#7259=ORIENTED_EDGE('',*,*,#5400,.T.);
#7260=ORIENTED_EDGE('',*,*,#5401,.F.);
#7261=ORIENTED_EDGE('',*,*,#5402,.F.);
#7262=ORIENTED_EDGE('',*,*,#5403,.F.);
#7263=ORIENTED_EDGE('',*,*,#5404,.T.);
#7264=ORIENTED_EDGE('',*,*,#5405,.F.);
#7265=ORIENTED_EDGE('',*,*,#5406,.T.);
#7266=ORIENTED_EDGE('',*,*,#5407,.F.);
#7267=ORIENTED_EDGE('',*,*,#5408,.F.);
#7268=ORIENTED_EDGE('',*,*,#5409,.F.);
#7269=ORIENTED_EDGE('',*,*,#5410,.T.);
#7270=ORIENTED_EDGE('',*,*,#5411,.F.);
#7271=ORIENTED_EDGE('',*,*,#5412,.T.);
#7272=ORIENTED_EDGE('',*,*,#5413,.F.);
#7273=ORIENTED_EDGE('',*,*,#5414,.F.);
#7274=ORIENTED_EDGE('',*,*,#5415,.F.);
#7275=ORIENTED_EDGE('',*,*,#5416,.T.);
#7276=ORIENTED_EDGE('',*,*,#5417,.F.);
#7277=ORIENTED_EDGE('',*,*,#5418,.T.);
#7278=ORIENTED_EDGE('',*,*,#5419,.F.);
#7279=ORIENTED_EDGE('',*,*,#5420,.F.);
#7280=ORIENTED_EDGE('',*,*,#5421,.F.);
#7281=ORIENTED_EDGE('',*,*,#5422,.T.);
#7282=ORIENTED_EDGE('',*,*,#5423,.F.);
#7283=ORIENTED_EDGE('',*,*,#5424,.T.);
#7284=ORIENTED_EDGE('',*,*,#5425,.F.);
#7285=ORIENTED_EDGE('',*,*,#5426,.F.);
#7286=ORIENTED_EDGE('',*,*,#5427,.F.);
#7287=ORIENTED_EDGE('',*,*,#5428,.T.);
#7288=ORIENTED_EDGE('',*,*,#5429,.F.);
#7289=ORIENTED_EDGE('',*,*,#5430,.T.);
#7290=ORIENTED_EDGE('',*,*,#5431,.F.);
#7291=ORIENTED_EDGE('',*,*,#5432,.F.);
#7292=ORIENTED_EDGE('',*,*,#5433,.F.);
#7293=ORIENTED_EDGE('',*,*,#5434,.T.);
#7294=ORIENTED_EDGE('',*,*,#5435,.F.);
#7295=ORIENTED_EDGE('',*,*,#5436,.T.);
#7296=ORIENTED_EDGE('',*,*,#5437,.F.);
#7297=ORIENTED_EDGE('',*,*,#5438,.F.);
#7298=ORIENTED_EDGE('',*,*,#5439,.F.);
#7299=ORIENTED_EDGE('',*,*,#5440,.T.);
#7300=ORIENTED_EDGE('',*,*,#5441,.F.);
#7301=ORIENTED_EDGE('',*,*,#5442,.T.);
#7302=ORIENTED_EDGE('',*,*,#5443,.F.);
#7303=ORIENTED_EDGE('',*,*,#5444,.F.);
#7304=ORIENTED_EDGE('',*,*,#5445,.F.);
#7305=ORIENTED_EDGE('',*,*,#5446,.T.);
#7306=ORIENTED_EDGE('',*,*,#5447,.F.);
#7307=ORIENTED_EDGE('',*,*,#5448,.T.);
#7308=ORIENTED_EDGE('',*,*,#5449,.F.);
#7309=ORIENTED_EDGE('',*,*,#5450,.F.);
#7310=ORIENTED_EDGE('',*,*,#5451,.F.);
#7311=ORIENTED_EDGE('',*,*,#5452,.T.);
#7312=ORIENTED_EDGE('',*,*,#5453,.F.);
#7313=ORIENTED_EDGE('',*,*,#5454,.T.);
#7314=ORIENTED_EDGE('',*,*,#5455,.F.);
#7315=ORIENTED_EDGE('',*,*,#5456,.F.);
#7316=ORIENTED_EDGE('',*,*,#5457,.F.);
#7317=ORIENTED_EDGE('',*,*,#5458,.T.);
#7318=ORIENTED_EDGE('',*,*,#5459,.F.);
#7319=ORIENTED_EDGE('',*,*,#5460,.T.);
#7320=ORIENTED_EDGE('',*,*,#5461,.F.);
#7321=ORIENTED_EDGE('',*,*,#5462,.F.);
#7322=ORIENTED_EDGE('',*,*,#5463,.F.);
#7323=ORIENTED_EDGE('',*,*,#5464,.T.);
#7324=ORIENTED_EDGE('',*,*,#5465,.F.);
#7325=ORIENTED_EDGE('',*,*,#5466,.T.);
#7326=ORIENTED_EDGE('',*,*,#5467,.F.);
#7327=ORIENTED_EDGE('',*,*,#5468,.F.);
#7328=ORIENTED_EDGE('',*,*,#5469,.F.);
#7329=ORIENTED_EDGE('',*,*,#5470,.T.);
#7330=ORIENTED_EDGE('',*,*,#5471,.F.);
#7331=ORIENTED_EDGE('',*,*,#5472,.T.);
#7332=ORIENTED_EDGE('',*,*,#5473,.F.);
#7333=ORIENTED_EDGE('',*,*,#5474,.F.);
#7334=ORIENTED_EDGE('',*,*,#5475,.F.);
#7335=ORIENTED_EDGE('',*,*,#5476,.T.);
#7336=ORIENTED_EDGE('',*,*,#5477,.F.);
#7337=ORIENTED_EDGE('',*,*,#5478,.T.);
#7338=ORIENTED_EDGE('',*,*,#5479,.F.);
#7339=ORIENTED_EDGE('',*,*,#5480,.F.);
#7340=ORIENTED_EDGE('',*,*,#5481,.F.);
#7341=ORIENTED_EDGE('',*,*,#5482,.T.);
#7342=ORIENTED_EDGE('',*,*,#5483,.F.);
#7343=ORIENTED_EDGE('',*,*,#5484,.T.);
#7344=ORIENTED_EDGE('',*,*,#5485,.F.);
#7345=ORIENTED_EDGE('',*,*,#5486,.F.);
#7346=ORIENTED_EDGE('',*,*,#5487,.F.);
#7347=ORIENTED_EDGE('',*,*,#5488,.T.);
#7348=ORIENTED_EDGE('',*,*,#5489,.F.);
#7349=ORIENTED_EDGE('',*,*,#5490,.T.);
#7350=ORIENTED_EDGE('',*,*,#5491,.F.);
#7351=ORIENTED_EDGE('',*,*,#5492,.F.);
#7352=ORIENTED_EDGE('',*,*,#5493,.F.);
#7353=ORIENTED_EDGE('',*,*,#5494,.T.);
#7354=ORIENTED_EDGE('',*,*,#5495,.F.);
#7355=ORIENTED_EDGE('',*,*,#5496,.T.);
#7356=ORIENTED_EDGE('',*,*,#5497,.F.);
#7357=ORIENTED_EDGE('',*,*,#5498,.F.);
#7358=ORIENTED_EDGE('',*,*,#5499,.F.);
#7359=ORIENTED_EDGE('',*,*,#5500,.T.);
#7360=ORIENTED_EDGE('',*,*,#5501,.F.);
#7361=ORIENTED_EDGE('',*,*,#5502,.T.);
#7362=ORIENTED_EDGE('',*,*,#5503,.F.);
#7363=ORIENTED_EDGE('',*,*,#5504,.F.);
#7364=ORIENTED_EDGE('',*,*,#5505,.F.);
#7365=ORIENTED_EDGE('',*,*,#5506,.T.);
#7366=ORIENTED_EDGE('',*,*,#5507,.F.);
#7367=ORIENTED_EDGE('',*,*,#5508,.T.);
#7368=ORIENTED_EDGE('',*,*,#5509,.F.);
#7369=ORIENTED_EDGE('',*,*,#5510,.F.);
#7370=ORIENTED_EDGE('',*,*,#5511,.F.);
#7371=ORIENTED_EDGE('',*,*,#5512,.T.);
#7372=ORIENTED_EDGE('',*,*,#5513,.F.);
#7373=ORIENTED_EDGE('',*,*,#5514,.T.);
#7374=ORIENTED_EDGE('',*,*,#5515,.F.);
#7375=ORIENTED_EDGE('',*,*,#5516,.F.);
#7376=ORIENTED_EDGE('',*,*,#5517,.F.);
#7377=ORIENTED_EDGE('',*,*,#5518,.T.);
#7378=ORIENTED_EDGE('',*,*,#5519,.F.);
#7379=ORIENTED_EDGE('',*,*,#5520,.T.);
#7380=ORIENTED_EDGE('',*,*,#5521,.F.);
#7381=ORIENTED_EDGE('',*,*,#5522,.F.);
#7382=ORIENTED_EDGE('',*,*,#5523,.F.);
#7383=ORIENTED_EDGE('',*,*,#5524,.T.);
#7384=ORIENTED_EDGE('',*,*,#5525,.F.);
#7385=ORIENTED_EDGE('',*,*,#5526,.T.);
#7386=ORIENTED_EDGE('',*,*,#5527,.F.);
#7387=ORIENTED_EDGE('',*,*,#5528,.F.);
#7388=ORIENTED_EDGE('',*,*,#5529,.F.);
#7389=ORIENTED_EDGE('',*,*,#5530,.T.);
#7390=ORIENTED_EDGE('',*,*,#5531,.F.);
#7391=ORIENTED_EDGE('',*,*,#5532,.T.);
#7392=ORIENTED_EDGE('',*,*,#5533,.F.);
#7393=ORIENTED_EDGE('',*,*,#5534,.F.);
#7394=ORIENTED_EDGE('',*,*,#5535,.F.);
#7395=ORIENTED_EDGE('',*,*,#5536,.T.);
#7396=ORIENTED_EDGE('',*,*,#5537,.F.);
#7397=ORIENTED_EDGE('',*,*,#5538,.T.);
#7398=ORIENTED_EDGE('',*,*,#5539,.F.);
#7399=ORIENTED_EDGE('',*,*,#5540,.F.);
#7400=ORIENTED_EDGE('',*,*,#5541,.F.);
#7401=ORIENTED_EDGE('',*,*,#5542,.T.);
#7402=ORIENTED_EDGE('',*,*,#5543,.F.);
#7403=ORIENTED_EDGE('',*,*,#5544,.F.);
#7404=ORIENTED_EDGE('',*,*,#5545,.F.);
#7405=ORIENTED_EDGE('',*,*,#5546,.F.);
#7406=ORIENTED_EDGE('',*,*,#5547,.F.);
#7407=ORIENTED_EDGE('',*,*,#5548,.F.);
#7408=ORIENTED_EDGE('',*,*,#5549,.F.);
#7409=ORIENTED_EDGE('',*,*,#5550,.F.);
#7410=ORIENTED_EDGE('',*,*,#5551,.F.);
#7411=ORIENTED_EDGE('',*,*,#5552,.F.);
#7412=ORIENTED_EDGE('',*,*,#5553,.F.);
#7413=ORIENTED_EDGE('',*,*,#5554,.F.);
#7414=ORIENTED_EDGE('',*,*,#5555,.F.);
#7415=ORIENTED_EDGE('',*,*,#5556,.F.);
#7416=ORIENTED_EDGE('',*,*,#5557,.F.);
#7417=ORIENTED_EDGE('',*,*,#5558,.F.);
#7418=ORIENTED_EDGE('',*,*,#5559,.F.);
#7419=ORIENTED_EDGE('',*,*,#5560,.F.);
#7420=ORIENTED_EDGE('',*,*,#5561,.F.);
#7421=ORIENTED_EDGE('',*,*,#5562,.F.);
#7422=ORIENTED_EDGE('',*,*,#5563,.F.);
#7423=ORIENTED_EDGE('',*,*,#5564,.F.);
#7424=ORIENTED_EDGE('',*,*,#5565,.F.);
#7425=ORIENTED_EDGE('',*,*,#5566,.F.);
#7426=ORIENTED_EDGE('',*,*,#5567,.F.);
#7427=ORIENTED_EDGE('',*,*,#5568,.F.);
#7428=ORIENTED_EDGE('',*,*,#5569,.F.);
#7429=ORIENTED_EDGE('',*,*,#5570,.F.);
#7430=ORIENTED_EDGE('',*,*,#5571,.F.);
#7431=ORIENTED_EDGE('',*,*,#5572,.F.);
#7432=ORIENTED_EDGE('',*,*,#5573,.F.);
#7433=ORIENTED_EDGE('',*,*,#5574,.F.);
#7434=ORIENTED_EDGE('',*,*,#5575,.F.);
#7435=ORIENTED_EDGE('',*,*,#5576,.F.);
#7436=ORIENTED_EDGE('',*,*,#5577,.F.);
#7437=ORIENTED_EDGE('',*,*,#5578,.F.);
#7438=ORIENTED_EDGE('',*,*,#5579,.F.);
#7439=ORIENTED_EDGE('',*,*,#5580,.F.);
#7440=ORIENTED_EDGE('',*,*,#5581,.F.);
#7441=ORIENTED_EDGE('',*,*,#5582,.F.);
#7442=ORIENTED_EDGE('',*,*,#5583,.F.);
#7443=ORIENTED_EDGE('',*,*,#5584,.F.);
#7444=ORIENTED_EDGE('',*,*,#5585,.F.);
#7445=ORIENTED_EDGE('',*,*,#5586,.F.);
#7446=ORIENTED_EDGE('',*,*,#5587,.F.);
#7447=ORIENTED_EDGE('',*,*,#5588,.F.);
#7448=ORIENTED_EDGE('',*,*,#5589,.F.);
#7449=ORIENTED_EDGE('',*,*,#5590,.F.);
#7450=ORIENTED_EDGE('',*,*,#5591,.F.);
#7451=ORIENTED_EDGE('',*,*,#5592,.F.);
#7452=ORIENTED_EDGE('',*,*,#5593,.F.);
#7453=ORIENTED_EDGE('',*,*,#5594,.F.);
#7454=ORIENTED_EDGE('',*,*,#5595,.F.);
#7455=ORIENTED_EDGE('',*,*,#5596,.F.);
#7456=ORIENTED_EDGE('',*,*,#5597,.F.);
#7457=ORIENTED_EDGE('',*,*,#5598,.F.);
#7458=ORIENTED_EDGE('',*,*,#5599,.F.);
#7459=ORIENTED_EDGE('',*,*,#5600,.F.);
#7460=ORIENTED_EDGE('',*,*,#5601,.F.);
#7461=ORIENTED_EDGE('',*,*,#5602,.F.);
#7462=ORIENTED_EDGE('',*,*,#5603,.F.);
#7463=ORIENTED_EDGE('',*,*,#5604,.F.);
#7464=ORIENTED_EDGE('',*,*,#5605,.F.);
#7465=ORIENTED_EDGE('',*,*,#5606,.F.);
#7466=ORIENTED_EDGE('',*,*,#5607,.F.);
#7467=ORIENTED_EDGE('',*,*,#5608,.F.);
#7468=ORIENTED_EDGE('',*,*,#5609,.F.);
#7469=ORIENTED_EDGE('',*,*,#5610,.F.);
#7470=ORIENTED_EDGE('',*,*,#5611,.F.);
#7471=ORIENTED_EDGE('',*,*,#5612,.F.);
#7472=ORIENTED_EDGE('',*,*,#5613,.F.);
#7473=ORIENTED_EDGE('',*,*,#5614,.F.);
#7474=ORIENTED_EDGE('',*,*,#5615,.F.);
#7475=ORIENTED_EDGE('',*,*,#5616,.F.);
#7476=ORIENTED_EDGE('',*,*,#5617,.F.);
#7477=ORIENTED_EDGE('',*,*,#5618,.F.);
#7478=ORIENTED_EDGE('',*,*,#5619,.F.);
#7479=ORIENTED_EDGE('',*,*,#5620,.F.);
#7480=ORIENTED_EDGE('',*,*,#5621,.F.);
#7481=ORIENTED_EDGE('',*,*,#5622,.F.);
#7482=ORIENTED_EDGE('',*,*,#5623,.F.);
#7483=ORIENTED_EDGE('',*,*,#5624,.F.);
#7484=ORIENTED_EDGE('',*,*,#5625,.F.);
#7485=ORIENTED_EDGE('',*,*,#5626,.F.);
#7486=ORIENTED_EDGE('',*,*,#5627,.F.);
#7487=ORIENTED_EDGE('',*,*,#5628,.F.);
#7488=ORIENTED_EDGE('',*,*,#5629,.F.);
#7489=ORIENTED_EDGE('',*,*,#5630,.F.);
#7490=ORIENTED_EDGE('',*,*,#5631,.F.);
#7491=ORIENTED_EDGE('',*,*,#5632,.F.);
#7492=ORIENTED_EDGE('',*,*,#5633,.T.);
#7493=ORIENTED_EDGE('',*,*,#5634,.F.);
#7494=ORIENTED_EDGE('',*,*,#5633,.F.);
#7495=ORIENTED_EDGE('',*,*,#5635,.F.);
#7496=ORIENTED_EDGE('',*,*,#5636,.F.);
#7497=ORIENTED_EDGE('',*,*,#5637,.F.);
#7498=ORIENTED_EDGE('',*,*,#5638,.F.);
#7499=ORIENTED_EDGE('',*,*,#5639,.F.);
#7500=ORIENTED_EDGE('',*,*,#5640,.F.);
#7501=ORIENTED_EDGE('',*,*,#5641,.F.);
#7502=ORIENTED_EDGE('',*,*,#5642,.F.);
#7503=ORIENTED_EDGE('',*,*,#5643,.F.);
#7504=ORIENTED_EDGE('',*,*,#5644,.F.);
#7505=ORIENTED_EDGE('',*,*,#5645,.F.);
#7506=ORIENTED_EDGE('',*,*,#5646,.F.);
#7507=ORIENTED_EDGE('',*,*,#5647,.F.);
#7508=ORIENTED_EDGE('',*,*,#5648,.F.);
#7509=ORIENTED_EDGE('',*,*,#5649,.F.);
#7510=ORIENTED_EDGE('',*,*,#5650,.F.);
#7511=ORIENTED_EDGE('',*,*,#5651,.F.);
#7512=ORIENTED_EDGE('',*,*,#5652,.F.);
#7513=ORIENTED_EDGE('',*,*,#5653,.F.);
#7514=ORIENTED_EDGE('',*,*,#5654,.F.);
#7515=ORIENTED_EDGE('',*,*,#5655,.F.);
#7516=ORIENTED_EDGE('',*,*,#5656,.F.);
#7517=ORIENTED_EDGE('',*,*,#5657,.F.);
#7518=ORIENTED_EDGE('',*,*,#5658,.F.);
#7519=ORIENTED_EDGE('',*,*,#5659,.F.);
#7520=ORIENTED_EDGE('',*,*,#5660,.F.);
#7521=ORIENTED_EDGE('',*,*,#5661,.F.);
#7522=ORIENTED_EDGE('',*,*,#5662,.F.);
#7523=ORIENTED_EDGE('',*,*,#5663,.F.);
#7524=ORIENTED_EDGE('',*,*,#5664,.F.);
#7525=ORIENTED_EDGE('',*,*,#5665,.F.);
#7526=ORIENTED_EDGE('',*,*,#5666,.F.);
#7527=ORIENTED_EDGE('',*,*,#5667,.F.);
#7528=ORIENTED_EDGE('',*,*,#5668,.F.);
#7529=ORIENTED_EDGE('',*,*,#5669,.F.);
#7530=ORIENTED_EDGE('',*,*,#5670,.F.);
#7531=ORIENTED_EDGE('',*,*,#5671,.F.);
#7532=ORIENTED_EDGE('',*,*,#5672,.F.);
#7533=ORIENTED_EDGE('',*,*,#5673,.F.);
#7534=ORIENTED_EDGE('',*,*,#5674,.F.);
#7535=ORIENTED_EDGE('',*,*,#5675,.F.);
#7536=ORIENTED_EDGE('',*,*,#5676,.F.);
#7537=ORIENTED_EDGE('',*,*,#5677,.F.);
#7538=ORIENTED_EDGE('',*,*,#5678,.F.);
#7539=ORIENTED_EDGE('',*,*,#5679,.F.);
#7540=ORIENTED_EDGE('',*,*,#5680,.F.);
#7541=ORIENTED_EDGE('',*,*,#5681,.F.);
#7542=ORIENTED_EDGE('',*,*,#5682,.F.);
#7543=ORIENTED_EDGE('',*,*,#5683,.F.);
#7544=ORIENTED_EDGE('',*,*,#5684,.F.);
#7545=ORIENTED_EDGE('',*,*,#5685,.F.);
#7546=ORIENTED_EDGE('',*,*,#5686,.F.);
#7547=ORIENTED_EDGE('',*,*,#5687,.F.);
#7548=ORIENTED_EDGE('',*,*,#5688,.F.);
#7549=ORIENTED_EDGE('',*,*,#5689,.F.);
#7550=ORIENTED_EDGE('',*,*,#5690,.F.);
#7551=ORIENTED_EDGE('',*,*,#5691,.F.);
#7552=ORIENTED_EDGE('',*,*,#5692,.F.);
#7553=ORIENTED_EDGE('',*,*,#5693,.F.);
#7554=ORIENTED_EDGE('',*,*,#5694,.F.);
#7555=ORIENTED_EDGE('',*,*,#5695,.F.);
#7556=ORIENTED_EDGE('',*,*,#5696,.F.);
#7557=ORIENTED_EDGE('',*,*,#5697,.F.);
#7558=ORIENTED_EDGE('',*,*,#5698,.F.);
#7559=ORIENTED_EDGE('',*,*,#5699,.F.);
#7560=ORIENTED_EDGE('',*,*,#5700,.F.);
#7561=ORIENTED_EDGE('',*,*,#5701,.F.);
#7562=ORIENTED_EDGE('',*,*,#5702,.F.);
#7563=ORIENTED_EDGE('',*,*,#5703,.F.);
#7564=ORIENTED_EDGE('',*,*,#5704,.F.);
#7565=ORIENTED_EDGE('',*,*,#5705,.F.);
#7566=ORIENTED_EDGE('',*,*,#5706,.F.);
#7567=ORIENTED_EDGE('',*,*,#5707,.F.);
#7568=ORIENTED_EDGE('',*,*,#5708,.F.);
#7569=ORIENTED_EDGE('',*,*,#5709,.F.);
#7570=ORIENTED_EDGE('',*,*,#5710,.F.);
#7571=ORIENTED_EDGE('',*,*,#5711,.F.);
#7572=ORIENTED_EDGE('',*,*,#5712,.F.);
#7573=ORIENTED_EDGE('',*,*,#5713,.F.);
#7574=ORIENTED_EDGE('',*,*,#5714,.F.);
#7575=ORIENTED_EDGE('',*,*,#5715,.F.);
#7576=ORIENTED_EDGE('',*,*,#5716,.F.);
#7577=ORIENTED_EDGE('',*,*,#5717,.F.);
#7578=ORIENTED_EDGE('',*,*,#5718,.F.);
#7579=ORIENTED_EDGE('',*,*,#5719,.F.);
#7580=ORIENTED_EDGE('',*,*,#5720,.F.);
#7581=ORIENTED_EDGE('',*,*,#5721,.F.);
#7582=ORIENTED_EDGE('',*,*,#5722,.F.);
#7583=ORIENTED_EDGE('',*,*,#5723,.T.);
#7584=ORIENTED_EDGE('',*,*,#5724,.T.);
#7585=ORIENTED_EDGE('',*,*,#5725,.F.);
#7586=ORIENTED_EDGE('',*,*,#5726,.F.);
#7587=ORIENTED_EDGE('',*,*,#5727,.T.);
#7588=ORIENTED_EDGE('',*,*,#5728,.T.);
#7589=ORIENTED_EDGE('',*,*,#5729,.F.);
#7590=ORIENTED_EDGE('',*,*,#5730,.T.);
#7591=ORIENTED_EDGE('',*,*,#5731,.T.);
#7592=ORIENTED_EDGE('',*,*,#5732,.T.);
#7593=ORIENTED_EDGE('',*,*,#5733,.F.);
#7594=ORIENTED_EDGE('',*,*,#5734,.T.);
#7595=ORIENTED_EDGE('',*,*,#5735,.T.);
#7596=ORIENTED_EDGE('',*,*,#5736,.T.);
#7597=ORIENTED_EDGE('',*,*,#5737,.F.);
#7598=ORIENTED_EDGE('',*,*,#5738,.T.);
#7599=ORIENTED_EDGE('',*,*,#5739,.T.);
#7600=ORIENTED_EDGE('',*,*,#5740,.T.);
#7601=ORIENTED_EDGE('',*,*,#5741,.F.);
#7602=ORIENTED_EDGE('',*,*,#5742,.T.);
#7603=ORIENTED_EDGE('',*,*,#5743,.T.);
#7604=ORIENTED_EDGE('',*,*,#5744,.T.);
#7605=ORIENTED_EDGE('',*,*,#5745,.F.);
#7606=ORIENTED_EDGE('',*,*,#5746,.T.);
#7607=ORIENTED_EDGE('',*,*,#5747,.T.);
#7608=ORIENTED_EDGE('',*,*,#5748,.T.);
#7609=ORIENTED_EDGE('',*,*,#5749,.F.);
#7610=ORIENTED_EDGE('',*,*,#5750,.T.);
#7611=ORIENTED_EDGE('',*,*,#5751,.T.);
#7612=ORIENTED_EDGE('',*,*,#5752,.T.);
#7613=ORIENTED_EDGE('',*,*,#5753,.F.);
#7614=ORIENTED_EDGE('',*,*,#5754,.T.);
#7615=ORIENTED_EDGE('',*,*,#5755,.T.);
#7616=ORIENTED_EDGE('',*,*,#5756,.T.);
#7617=ORIENTED_EDGE('',*,*,#5757,.F.);
#7618=ORIENTED_EDGE('',*,*,#5758,.T.);
#7619=ORIENTED_EDGE('',*,*,#5759,.T.);
#7620=ORIENTED_EDGE('',*,*,#5760,.T.);
#7621=ORIENTED_EDGE('',*,*,#5761,.F.);
#7622=ORIENTED_EDGE('',*,*,#5762,.T.);
#7623=ORIENTED_EDGE('',*,*,#5763,.T.);
#7624=ORIENTED_EDGE('',*,*,#5764,.T.);
#7625=ORIENTED_EDGE('',*,*,#5765,.F.);
#7626=ORIENTED_EDGE('',*,*,#5766,.T.);
#7627=ORIENTED_EDGE('',*,*,#5767,.T.);
#7628=ORIENTED_EDGE('',*,*,#5768,.T.);
#7629=ORIENTED_EDGE('',*,*,#5769,.F.);
#7630=ORIENTED_EDGE('',*,*,#5770,.T.);
#7631=ORIENTED_EDGE('',*,*,#5771,.T.);
#7632=ORIENTED_EDGE('',*,*,#5772,.T.);
#7633=ORIENTED_EDGE('',*,*,#5773,.F.);
#7634=ORIENTED_EDGE('',*,*,#5774,.T.);
#7635=ORIENTED_EDGE('',*,*,#5775,.T.);
#7636=ORIENTED_EDGE('',*,*,#5776,.T.);
#7637=ORIENTED_EDGE('',*,*,#5777,.F.);
#7638=ORIENTED_EDGE('',*,*,#5778,.T.);
#7639=ORIENTED_EDGE('',*,*,#5779,.T.);
#7640=ORIENTED_EDGE('',*,*,#5780,.T.);
#7641=ORIENTED_EDGE('',*,*,#5781,.F.);
#7642=ORIENTED_EDGE('',*,*,#5782,.T.);
#7643=ORIENTED_EDGE('',*,*,#5783,.T.);
#7644=ORIENTED_EDGE('',*,*,#5784,.T.);
#7645=ORIENTED_EDGE('',*,*,#5785,.F.);
#7646=ORIENTED_EDGE('',*,*,#5786,.T.);
#7647=ORIENTED_EDGE('',*,*,#5787,.T.);
#7648=ORIENTED_EDGE('',*,*,#5788,.T.);
#7649=ORIENTED_EDGE('',*,*,#5789,.F.);
#7650=ORIENTED_EDGE('',*,*,#5790,.T.);
#7651=ORIENTED_EDGE('',*,*,#5791,.T.);
#7652=ORIENTED_EDGE('',*,*,#5792,.T.);
#7653=ORIENTED_EDGE('',*,*,#5793,.F.);
#7654=ORIENTED_EDGE('',*,*,#5794,.T.);
#7655=ORIENTED_EDGE('',*,*,#5795,.T.);
#7656=ORIENTED_EDGE('',*,*,#5796,.T.);
#7657=ORIENTED_EDGE('',*,*,#5797,.F.);
#7658=ORIENTED_EDGE('',*,*,#5798,.T.);
#7659=ORIENTED_EDGE('',*,*,#5799,.T.);
#7660=ORIENTED_EDGE('',*,*,#5800,.T.);
#7661=ORIENTED_EDGE('',*,*,#5801,.F.);
#7662=ORIENTED_EDGE('',*,*,#5802,.T.);
#7663=ORIENTED_EDGE('',*,*,#5803,.T.);
#7664=ORIENTED_EDGE('',*,*,#5804,.T.);
#7665=ORIENTED_EDGE('',*,*,#5805,.F.);
#7666=ORIENTED_EDGE('',*,*,#5806,.T.);
#7667=ORIENTED_EDGE('',*,*,#5807,.T.);
#7668=ORIENTED_EDGE('',*,*,#5808,.T.);
#7669=ORIENTED_EDGE('',*,*,#5809,.F.);
#7670=ORIENTED_EDGE('',*,*,#5810,.T.);
#7671=ORIENTED_EDGE('',*,*,#5811,.T.);
#7672=ORIENTED_EDGE('',*,*,#5812,.T.);
#7673=ORIENTED_EDGE('',*,*,#5813,.F.);
#7674=ORIENTED_EDGE('',*,*,#5814,.T.);
#7675=ORIENTED_EDGE('',*,*,#5815,.T.);
#7676=ORIENTED_EDGE('',*,*,#5816,.T.);
#7677=ORIENTED_EDGE('',*,*,#5817,.F.);
#7678=ORIENTED_EDGE('',*,*,#5816,.F.);
#7679=ORIENTED_EDGE('',*,*,#5818,.T.);
#7680=ORIENTED_EDGE('',*,*,#5819,.T.);
#7681=ORIENTED_EDGE('',*,*,#5820,.F.);
#7682=ORIENTED_EDGE('',*,*,#5821,.T.);
#7683=ORIENTED_EDGE('',*,*,#5822,.T.);
#7684=ORIENTED_EDGE('',*,*,#5823,.T.);
#7685=ORIENTED_EDGE('',*,*,#5824,.F.);
#7686=ORIENTED_EDGE('',*,*,#5825,.T.);
#7687=ORIENTED_EDGE('',*,*,#5826,.T.);
#7688=ORIENTED_EDGE('',*,*,#5827,.T.);
#7689=ORIENTED_EDGE('',*,*,#5828,.F.);
#7690=ORIENTED_EDGE('',*,*,#5829,.T.);
#7691=ORIENTED_EDGE('',*,*,#5830,.T.);
#7692=ORIENTED_EDGE('',*,*,#5831,.T.);
#7693=ORIENTED_EDGE('',*,*,#5832,.F.);
#7694=ORIENTED_EDGE('',*,*,#5833,.T.);
#7695=ORIENTED_EDGE('',*,*,#5834,.T.);
#7696=ORIENTED_EDGE('',*,*,#5835,.T.);
#7697=ORIENTED_EDGE('',*,*,#5836,.F.);
#7698=ORIENTED_EDGE('',*,*,#5837,.T.);
#7699=ORIENTED_EDGE('',*,*,#5838,.T.);
#7700=ORIENTED_EDGE('',*,*,#5839,.T.);
#7701=ORIENTED_EDGE('',*,*,#5840,.F.);
#7702=ORIENTED_EDGE('',*,*,#5841,.T.);
#7703=ORIENTED_EDGE('',*,*,#5842,.T.);
#7704=ORIENTED_EDGE('',*,*,#5843,.T.);
#7705=ORIENTED_EDGE('',*,*,#5844,.F.);
#7706=ORIENTED_EDGE('',*,*,#5845,.T.);
#7707=ORIENTED_EDGE('',*,*,#5846,.T.);
#7708=ORIENTED_EDGE('',*,*,#5847,.T.);
#7709=ORIENTED_EDGE('',*,*,#5848,.F.);
#7710=ORIENTED_EDGE('',*,*,#5849,.T.);
#7711=ORIENTED_EDGE('',*,*,#5850,.T.);
#7712=ORIENTED_EDGE('',*,*,#5851,.T.);
#7713=ORIENTED_EDGE('',*,*,#5852,.F.);
#7714=ORIENTED_EDGE('',*,*,#5853,.T.);
#7715=ORIENTED_EDGE('',*,*,#5854,.T.);
#7716=ORIENTED_EDGE('',*,*,#5855,.T.);
#7717=ORIENTED_EDGE('',*,*,#5856,.F.);
#7718=ORIENTED_EDGE('',*,*,#5857,.T.);
#7719=ORIENTED_EDGE('',*,*,#5858,.T.);
#7720=ORIENTED_EDGE('',*,*,#5859,.T.);
#7721=ORIENTED_EDGE('',*,*,#5860,.F.);
#7722=ORIENTED_EDGE('',*,*,#5861,.T.);
#7723=ORIENTED_EDGE('',*,*,#5862,.T.);
#7724=ORIENTED_EDGE('',*,*,#5863,.T.);
#7725=ORIENTED_EDGE('',*,*,#5864,.F.);
#7726=ORIENTED_EDGE('',*,*,#5865,.T.);
#7727=ORIENTED_EDGE('',*,*,#5866,.T.);
#7728=ORIENTED_EDGE('',*,*,#5867,.T.);
#7729=ORIENTED_EDGE('',*,*,#5868,.F.);
#7730=ORIENTED_EDGE('',*,*,#5869,.T.);
#7731=ORIENTED_EDGE('',*,*,#5870,.T.);
#7732=ORIENTED_EDGE('',*,*,#5871,.T.);
#7733=ORIENTED_EDGE('',*,*,#5872,.F.);
#7734=ORIENTED_EDGE('',*,*,#5873,.T.);
#7735=ORIENTED_EDGE('',*,*,#5874,.T.);
#7736=ORIENTED_EDGE('',*,*,#5875,.T.);
#7737=ORIENTED_EDGE('',*,*,#5876,.F.);
#7738=ORIENTED_EDGE('',*,*,#5877,.T.);
#7739=ORIENTED_EDGE('',*,*,#5878,.T.);
#7740=ORIENTED_EDGE('',*,*,#5879,.T.);
#7741=ORIENTED_EDGE('',*,*,#5880,.F.);
#7742=ORIENTED_EDGE('',*,*,#5881,.T.);
#7743=ORIENTED_EDGE('',*,*,#5882,.T.);
#7744=ORIENTED_EDGE('',*,*,#5883,.T.);
#7745=ORIENTED_EDGE('',*,*,#5884,.F.);
#7746=ORIENTED_EDGE('',*,*,#5885,.T.);
#7747=ORIENTED_EDGE('',*,*,#5886,.T.);
#7748=ORIENTED_EDGE('',*,*,#5887,.T.);
#7749=ORIENTED_EDGE('',*,*,#5888,.F.);
#7750=ORIENTED_EDGE('',*,*,#5889,.T.);
#7751=ORIENTED_EDGE('',*,*,#5890,.T.);
#7752=ORIENTED_EDGE('',*,*,#5891,.T.);
#7753=ORIENTED_EDGE('',*,*,#5892,.F.);
#7754=ORIENTED_EDGE('',*,*,#5893,.T.);
#7755=ORIENTED_EDGE('',*,*,#5894,.T.);
#7756=ORIENTED_EDGE('',*,*,#5895,.T.);
#7757=ORIENTED_EDGE('',*,*,#5896,.F.);
#7758=ORIENTED_EDGE('',*,*,#5897,.T.);
#7759=ORIENTED_EDGE('',*,*,#5898,.T.);
#7760=ORIENTED_EDGE('',*,*,#5899,.T.);
#7761=ORIENTED_EDGE('',*,*,#5900,.F.);
#7762=ORIENTED_EDGE('',*,*,#5901,.T.);
#7763=ORIENTED_EDGE('',*,*,#5902,.T.);
#7764=ORIENTED_EDGE('',*,*,#5903,.T.);
#7765=ORIENTED_EDGE('',*,*,#5904,.F.);
#7766=ORIENTED_EDGE('',*,*,#5905,.T.);
#7767=ORIENTED_EDGE('',*,*,#5906,.F.);
#7768=ORIENTED_EDGE('',*,*,#5765,.T.);
#7769=ORIENTED_EDGE('',*,*,#5907,.F.);
#7770=ORIENTED_EDGE('',*,*,#5540,.T.);
#7771=ORIENTED_EDGE('',*,*,#5908,.F.);
#7772=ORIENTED_EDGE('',*,*,#5534,.T.);
#7773=ORIENTED_EDGE('',*,*,#5909,.F.);
#7774=ORIENTED_EDGE('',*,*,#5769,.T.);
#7775=ORIENTED_EDGE('',*,*,#5910,.F.);
#7776=ORIENTED_EDGE('',*,*,#5761,.T.);
#7777=ORIENTED_EDGE('',*,*,#5911,.F.);
#7778=ORIENTED_EDGE('',*,*,#5528,.T.);
#7779=ORIENTED_EDGE('',*,*,#5912,.F.);
#7780=ORIENTED_EDGE('',*,*,#5757,.T.);
#7781=ORIENTED_EDGE('',*,*,#5913,.F.);
#7782=ORIENTED_EDGE('',*,*,#5522,.T.);
#7783=ORIENTED_EDGE('',*,*,#5914,.F.);
#7784=ORIENTED_EDGE('',*,*,#5753,.T.);
#7785=ORIENTED_EDGE('',*,*,#5915,.F.);
#7786=ORIENTED_EDGE('',*,*,#5516,.T.);
#7787=ORIENTED_EDGE('',*,*,#5916,.F.);
#7788=ORIENTED_EDGE('',*,*,#5749,.T.);
#7789=ORIENTED_EDGE('',*,*,#5917,.F.);
#7790=ORIENTED_EDGE('',*,*,#5510,.T.);
#7791=ORIENTED_EDGE('',*,*,#5918,.F.);
#7792=ORIENTED_EDGE('',*,*,#5745,.T.);
#7793=ORIENTED_EDGE('',*,*,#5919,.F.);
#7794=ORIENTED_EDGE('',*,*,#5504,.T.);
#7795=ORIENTED_EDGE('',*,*,#5920,.F.);
#7796=ORIENTED_EDGE('',*,*,#5741,.T.);
#7797=ORIENTED_EDGE('',*,*,#5921,.F.);
#7798=ORIENTED_EDGE('',*,*,#5498,.T.);
#7799=ORIENTED_EDGE('',*,*,#5922,.F.);
#7800=ORIENTED_EDGE('',*,*,#5737,.T.);
#7801=ORIENTED_EDGE('',*,*,#5923,.F.);
#7802=ORIENTED_EDGE('',*,*,#5492,.T.);
#7803=ORIENTED_EDGE('',*,*,#5924,.F.);
#7804=ORIENTED_EDGE('',*,*,#5733,.T.);
#7805=ORIENTED_EDGE('',*,*,#5925,.F.);
#7806=ORIENTED_EDGE('',*,*,#5486,.T.);
#7807=ORIENTED_EDGE('',*,*,#5926,.F.);
#7808=ORIENTED_EDGE('',*,*,#5729,.T.);
#7809=ORIENTED_EDGE('',*,*,#5927,.F.);
#7810=ORIENTED_EDGE('',*,*,#5480,.T.);
#7811=ORIENTED_EDGE('',*,*,#5928,.F.);
#7812=ORIENTED_EDGE('',*,*,#5904,.T.);
#7813=ORIENTED_EDGE('',*,*,#5929,.F.);
#7814=ORIENTED_EDGE('',*,*,#5474,.T.);
#7815=ORIENTED_EDGE('',*,*,#5930,.F.);
#7816=ORIENTED_EDGE('',*,*,#5900,.T.);
#7817=ORIENTED_EDGE('',*,*,#5931,.F.);
#7818=ORIENTED_EDGE('',*,*,#5468,.T.);
#7819=ORIENTED_EDGE('',*,*,#5932,.F.);
#7820=ORIENTED_EDGE('',*,*,#5896,.T.);
#7821=ORIENTED_EDGE('',*,*,#5933,.F.);
#7822=ORIENTED_EDGE('',*,*,#5462,.T.);
#7823=ORIENTED_EDGE('',*,*,#5934,.F.);
#7824=ORIENTED_EDGE('',*,*,#5892,.T.);
#7825=ORIENTED_EDGE('',*,*,#5935,.F.);
#7826=ORIENTED_EDGE('',*,*,#5456,.T.);
#7827=ORIENTED_EDGE('',*,*,#5936,.F.);
#7828=ORIENTED_EDGE('',*,*,#5888,.T.);
#7829=ORIENTED_EDGE('',*,*,#5937,.F.);
#7830=ORIENTED_EDGE('',*,*,#5450,.T.);
#7831=ORIENTED_EDGE('',*,*,#5938,.F.);
#7832=ORIENTED_EDGE('',*,*,#5884,.T.);
#7833=ORIENTED_EDGE('',*,*,#5939,.F.);
#7834=ORIENTED_EDGE('',*,*,#5444,.T.);
#7835=ORIENTED_EDGE('',*,*,#5940,.F.);
#7836=ORIENTED_EDGE('',*,*,#5880,.T.);
#7837=ORIENTED_EDGE('',*,*,#5941,.F.);
#7838=ORIENTED_EDGE('',*,*,#5438,.T.);
#7839=ORIENTED_EDGE('',*,*,#5942,.F.);
#7840=ORIENTED_EDGE('',*,*,#5876,.T.);
#7841=ORIENTED_EDGE('',*,*,#5943,.F.);
#7842=ORIENTED_EDGE('',*,*,#5432,.T.);
#7843=ORIENTED_EDGE('',*,*,#5944,.F.);
#7844=ORIENTED_EDGE('',*,*,#5872,.T.);
#7845=ORIENTED_EDGE('',*,*,#5945,.F.);
#7846=ORIENTED_EDGE('',*,*,#5426,.T.);
#7847=ORIENTED_EDGE('',*,*,#5946,.F.);
#7848=ORIENTED_EDGE('',*,*,#5868,.T.);
#7849=ORIENTED_EDGE('',*,*,#5947,.F.);
#7850=ORIENTED_EDGE('',*,*,#5420,.T.);
#7851=ORIENTED_EDGE('',*,*,#5948,.F.);
#7852=ORIENTED_EDGE('',*,*,#5864,.T.);
#7853=ORIENTED_EDGE('',*,*,#5949,.F.);
#7854=ORIENTED_EDGE('',*,*,#5414,.T.);
#7855=ORIENTED_EDGE('',*,*,#5950,.F.);
#7856=ORIENTED_EDGE('',*,*,#5860,.T.);
#7857=ORIENTED_EDGE('',*,*,#5951,.F.);
#7858=ORIENTED_EDGE('',*,*,#5408,.T.);
#7859=ORIENTED_EDGE('',*,*,#5952,.F.);
#7860=ORIENTED_EDGE('',*,*,#5856,.T.);
#7861=ORIENTED_EDGE('',*,*,#5953,.F.);
#7862=ORIENTED_EDGE('',*,*,#5402,.T.);
#7863=ORIENTED_EDGE('',*,*,#5954,.F.);
#7864=ORIENTED_EDGE('',*,*,#5852,.T.);
#7865=ORIENTED_EDGE('',*,*,#5955,.F.);
#7866=ORIENTED_EDGE('',*,*,#5396,.T.);
#7867=ORIENTED_EDGE('',*,*,#5956,.F.);
#7868=ORIENTED_EDGE('',*,*,#5848,.T.);
#7869=ORIENTED_EDGE('',*,*,#5957,.F.);
#7870=ORIENTED_EDGE('',*,*,#5390,.T.);
#7871=ORIENTED_EDGE('',*,*,#5958,.F.);
#7872=ORIENTED_EDGE('',*,*,#5844,.T.);
#7873=ORIENTED_EDGE('',*,*,#5959,.F.);
#7874=ORIENTED_EDGE('',*,*,#5384,.T.);
#7875=ORIENTED_EDGE('',*,*,#5960,.F.);
#7876=ORIENTED_EDGE('',*,*,#5840,.T.);
#7877=ORIENTED_EDGE('',*,*,#5961,.F.);
#7878=ORIENTED_EDGE('',*,*,#5378,.T.);
#7879=ORIENTED_EDGE('',*,*,#5962,.F.);
#7880=ORIENTED_EDGE('',*,*,#5836,.T.);
#7881=ORIENTED_EDGE('',*,*,#5963,.F.);
#7882=ORIENTED_EDGE('',*,*,#5372,.T.);
#7883=ORIENTED_EDGE('',*,*,#5964,.F.);
#7884=ORIENTED_EDGE('',*,*,#5832,.T.);
#7885=ORIENTED_EDGE('',*,*,#5965,.F.);
#7886=ORIENTED_EDGE('',*,*,#5366,.T.);
#7887=ORIENTED_EDGE('',*,*,#5966,.F.);
#7888=ORIENTED_EDGE('',*,*,#5828,.T.);
#7889=ORIENTED_EDGE('',*,*,#5967,.F.);
#7890=ORIENTED_EDGE('',*,*,#5360,.T.);
#7891=ORIENTED_EDGE('',*,*,#5968,.F.);
#7892=ORIENTED_EDGE('',*,*,#5824,.T.);
#7893=ORIENTED_EDGE('',*,*,#5969,.F.);
#7894=ORIENTED_EDGE('',*,*,#5354,.T.);
#7895=ORIENTED_EDGE('',*,*,#5970,.F.);
#7896=ORIENTED_EDGE('',*,*,#5820,.T.);
#7897=ORIENTED_EDGE('',*,*,#5971,.F.);
#7898=ORIENTED_EDGE('',*,*,#5348,.T.);
#7899=ORIENTED_EDGE('',*,*,#5972,.F.);
#7900=ORIENTED_EDGE('',*,*,#5813,.T.);
#7901=ORIENTED_EDGE('',*,*,#5973,.F.);
#7902=ORIENTED_EDGE('',*,*,#5342,.T.);
#7903=ORIENTED_EDGE('',*,*,#5974,.F.);
#7904=ORIENTED_EDGE('',*,*,#5809,.T.);
#7905=ORIENTED_EDGE('',*,*,#5975,.F.);
#7906=ORIENTED_EDGE('',*,*,#5336,.T.);
#7907=ORIENTED_EDGE('',*,*,#5976,.F.);
#7908=ORIENTED_EDGE('',*,*,#5805,.T.);
#7909=ORIENTED_EDGE('',*,*,#5977,.F.);
#7910=ORIENTED_EDGE('',*,*,#5330,.T.);
#7911=ORIENTED_EDGE('',*,*,#5978,.F.);
#7912=ORIENTED_EDGE('',*,*,#5801,.T.);
#7913=ORIENTED_EDGE('',*,*,#5979,.F.);
#7914=ORIENTED_EDGE('',*,*,#5324,.T.);
#7915=ORIENTED_EDGE('',*,*,#5980,.F.);
#7916=ORIENTED_EDGE('',*,*,#5797,.T.);
#7917=ORIENTED_EDGE('',*,*,#5981,.F.);
#7918=ORIENTED_EDGE('',*,*,#5318,.T.);
#7919=ORIENTED_EDGE('',*,*,#5982,.F.);
#7920=ORIENTED_EDGE('',*,*,#5793,.T.);
#7921=ORIENTED_EDGE('',*,*,#5983,.F.);
#7922=ORIENTED_EDGE('',*,*,#5312,.T.);
#7923=ORIENTED_EDGE('',*,*,#5984,.F.);
#7924=ORIENTED_EDGE('',*,*,#5789,.T.);
#7925=ORIENTED_EDGE('',*,*,#5985,.F.);
#7926=ORIENTED_EDGE('',*,*,#5306,.T.);
#7927=ORIENTED_EDGE('',*,*,#5986,.F.);
#7928=ORIENTED_EDGE('',*,*,#5785,.T.);
#7929=ORIENTED_EDGE('',*,*,#5987,.F.);
#7930=ORIENTED_EDGE('',*,*,#5300,.T.);
#7931=ORIENTED_EDGE('',*,*,#5988,.F.);
#7932=ORIENTED_EDGE('',*,*,#5781,.T.);
#7933=ORIENTED_EDGE('',*,*,#5989,.F.);
#7934=ORIENTED_EDGE('',*,*,#5294,.T.);
#7935=ORIENTED_EDGE('',*,*,#5990,.F.);
#7936=ORIENTED_EDGE('',*,*,#5777,.T.);
#7937=ORIENTED_EDGE('',*,*,#5991,.F.);
#7938=ORIENTED_EDGE('',*,*,#5288,.T.);
#7939=ORIENTED_EDGE('',*,*,#5992,.F.);
#7940=ORIENTED_EDGE('',*,*,#5773,.T.);
#7941=ORIENTED_EDGE('',*,*,#5993,.F.);
#7942=ORIENTED_EDGE('',*,*,#5282,.T.);
#7943=ORIENTED_EDGE('',*,*,#5537,.T.);
#7944=ORIENTED_EDGE('',*,*,#5994,.T.);
#7945=ORIENTED_EDGE('',*,*,#5590,.T.);
#7946=ORIENTED_EDGE('',*,*,#5995,.T.);
#7947=ORIENTED_EDGE('',*,*,#5594,.T.);
#7948=ORIENTED_EDGE('',*,*,#5996,.T.);
#7949=ORIENTED_EDGE('',*,*,#5543,.T.);
#7950=ORIENTED_EDGE('',*,*,#5997,.T.);
#7951=ORIENTED_EDGE('',*,*,#5598,.T.);
#7952=ORIENTED_EDGE('',*,*,#5998,.T.);
#7953=ORIENTED_EDGE('',*,*,#5531,.T.);
#7954=ORIENTED_EDGE('',*,*,#5999,.T.);
#7955=ORIENTED_EDGE('',*,*,#5602,.T.);
#7956=ORIENTED_EDGE('',*,*,#6000,.T.);
#7957=ORIENTED_EDGE('',*,*,#5525,.T.);
#7958=ORIENTED_EDGE('',*,*,#6001,.T.);
#7959=ORIENTED_EDGE('',*,*,#5606,.T.);
#7960=ORIENTED_EDGE('',*,*,#6002,.T.);
#7961=ORIENTED_EDGE('',*,*,#5519,.T.);
#7962=ORIENTED_EDGE('',*,*,#6003,.T.);
#7963=ORIENTED_EDGE('',*,*,#5610,.T.);
#7964=ORIENTED_EDGE('',*,*,#6004,.T.);
#7965=ORIENTED_EDGE('',*,*,#5513,.T.);
#7966=ORIENTED_EDGE('',*,*,#6005,.T.);
#7967=ORIENTED_EDGE('',*,*,#5618,.T.);
#7968=ORIENTED_EDGE('',*,*,#6006,.T.);
#7969=ORIENTED_EDGE('',*,*,#5501,.T.);
#7970=ORIENTED_EDGE('',*,*,#6007,.T.);
#7971=ORIENTED_EDGE('',*,*,#5614,.T.);
#7972=ORIENTED_EDGE('',*,*,#6008,.T.);
#7973=ORIENTED_EDGE('',*,*,#5507,.T.);
#7974=ORIENTED_EDGE('',*,*,#6009,.T.);
#7975=ORIENTED_EDGE('',*,*,#5622,.T.);
#7976=ORIENTED_EDGE('',*,*,#6010,.T.);
#7977=ORIENTED_EDGE('',*,*,#5495,.T.);
#7978=ORIENTED_EDGE('',*,*,#6011,.T.);
#7979=ORIENTED_EDGE('',*,*,#5626,.T.);
#7980=ORIENTED_EDGE('',*,*,#6012,.T.);
#7981=ORIENTED_EDGE('',*,*,#5489,.T.);
#7982=ORIENTED_EDGE('',*,*,#6013,.T.);
#7983=ORIENTED_EDGE('',*,*,#5630,.T.);
#7984=ORIENTED_EDGE('',*,*,#6014,.T.);
#7985=ORIENTED_EDGE('',*,*,#5483,.T.);
#7986=ORIENTED_EDGE('',*,*,#6015,.T.);
#7987=ORIENTED_EDGE('',*,*,#5637,.T.);
#7988=ORIENTED_EDGE('',*,*,#6016,.T.);
#7989=ORIENTED_EDGE('',*,*,#5477,.T.);
#7990=ORIENTED_EDGE('',*,*,#6017,.T.);
#7991=ORIENTED_EDGE('',*,*,#5641,.T.);
#7992=ORIENTED_EDGE('',*,*,#6018,.T.);
#7993=ORIENTED_EDGE('',*,*,#5471,.T.);
#7994=ORIENTED_EDGE('',*,*,#6019,.T.);
#7995=ORIENTED_EDGE('',*,*,#5645,.T.);
#7996=ORIENTED_EDGE('',*,*,#6020,.T.);
#7997=ORIENTED_EDGE('',*,*,#5465,.T.);
#7998=ORIENTED_EDGE('',*,*,#6021,.T.);
#7999=ORIENTED_EDGE('',*,*,#5649,.T.);
#8000=ORIENTED_EDGE('',*,*,#6022,.T.);
#8001=ORIENTED_EDGE('',*,*,#5459,.T.);
#8002=ORIENTED_EDGE('',*,*,#6023,.T.);
#8003=ORIENTED_EDGE('',*,*,#5653,.T.);
#8004=ORIENTED_EDGE('',*,*,#6024,.T.);
#8005=ORIENTED_EDGE('',*,*,#5453,.T.);
#8006=ORIENTED_EDGE('',*,*,#6025,.T.);
#8007=ORIENTED_EDGE('',*,*,#5657,.T.);
#8008=ORIENTED_EDGE('',*,*,#6026,.T.);
#8009=ORIENTED_EDGE('',*,*,#5447,.T.);
#8010=ORIENTED_EDGE('',*,*,#6027,.T.);
#8011=ORIENTED_EDGE('',*,*,#5661,.T.);
#8012=ORIENTED_EDGE('',*,*,#6028,.T.);
#8013=ORIENTED_EDGE('',*,*,#5441,.T.);
#8014=ORIENTED_EDGE('',*,*,#6029,.T.);
#8015=ORIENTED_EDGE('',*,*,#5665,.T.);
#8016=ORIENTED_EDGE('',*,*,#6030,.T.);
#8017=ORIENTED_EDGE('',*,*,#5435,.T.);
#8018=ORIENTED_EDGE('',*,*,#6031,.T.);
#8019=ORIENTED_EDGE('',*,*,#5669,.T.);
#8020=ORIENTED_EDGE('',*,*,#6032,.T.);
#8021=ORIENTED_EDGE('',*,*,#5429,.T.);
#8022=ORIENTED_EDGE('',*,*,#6033,.T.);
#8023=ORIENTED_EDGE('',*,*,#5673,.T.);
#8024=ORIENTED_EDGE('',*,*,#6034,.T.);
#8025=ORIENTED_EDGE('',*,*,#5423,.T.);
#8026=ORIENTED_EDGE('',*,*,#6035,.T.);
#8027=ORIENTED_EDGE('',*,*,#5677,.T.);
#8028=ORIENTED_EDGE('',*,*,#6036,.T.);
#8029=ORIENTED_EDGE('',*,*,#5417,.T.);
#8030=ORIENTED_EDGE('',*,*,#6037,.T.);
#8031=ORIENTED_EDGE('',*,*,#5681,.T.);
#8032=ORIENTED_EDGE('',*,*,#6038,.T.);
#8033=ORIENTED_EDGE('',*,*,#5411,.T.);
#8034=ORIENTED_EDGE('',*,*,#6039,.T.);
#8035=ORIENTED_EDGE('',*,*,#5685,.T.);
#8036=ORIENTED_EDGE('',*,*,#6040,.T.);
#8037=ORIENTED_EDGE('',*,*,#5405,.T.);
#8038=ORIENTED_EDGE('',*,*,#6041,.T.);
#8039=ORIENTED_EDGE('',*,*,#5689,.T.);
#8040=ORIENTED_EDGE('',*,*,#6042,.T.);
#8041=ORIENTED_EDGE('',*,*,#5399,.T.);
#8042=ORIENTED_EDGE('',*,*,#6043,.T.);
#8043=ORIENTED_EDGE('',*,*,#5693,.T.);
#8044=ORIENTED_EDGE('',*,*,#6044,.T.);
#8045=ORIENTED_EDGE('',*,*,#5393,.T.);
#8046=ORIENTED_EDGE('',*,*,#6045,.T.);
#8047=ORIENTED_EDGE('',*,*,#5697,.T.);
#8048=ORIENTED_EDGE('',*,*,#6046,.T.);
#8049=ORIENTED_EDGE('',*,*,#5387,.T.);
#8050=ORIENTED_EDGE('',*,*,#6047,.T.);
#8051=ORIENTED_EDGE('',*,*,#5701,.T.);
#8052=ORIENTED_EDGE('',*,*,#6048,.T.);
#8053=ORIENTED_EDGE('',*,*,#5381,.T.);
#8054=ORIENTED_EDGE('',*,*,#6049,.T.);
#8055=ORIENTED_EDGE('',*,*,#5709,.T.);
#8056=ORIENTED_EDGE('',*,*,#6050,.T.);
#8057=ORIENTED_EDGE('',*,*,#5369,.T.);
#8058=ORIENTED_EDGE('',*,*,#6051,.T.);
#8059=ORIENTED_EDGE('',*,*,#5705,.T.);
#8060=ORIENTED_EDGE('',*,*,#6052,.T.);
#8061=ORIENTED_EDGE('',*,*,#5375,.T.);
#8062=ORIENTED_EDGE('',*,*,#6053,.T.);
#8063=ORIENTED_EDGE('',*,*,#5713,.T.);
#8064=ORIENTED_EDGE('',*,*,#6054,.T.);
#8065=ORIENTED_EDGE('',*,*,#5363,.T.);
#8066=ORIENTED_EDGE('',*,*,#6055,.T.);
#8067=ORIENTED_EDGE('',*,*,#5717,.T.);
#8068=ORIENTED_EDGE('',*,*,#6056,.T.);
#8069=ORIENTED_EDGE('',*,*,#5357,.T.);
#8070=ORIENTED_EDGE('',*,*,#6057,.T.);
#8071=ORIENTED_EDGE('',*,*,#5721,.T.);
#8072=ORIENTED_EDGE('',*,*,#6058,.T.);
#8073=ORIENTED_EDGE('',*,*,#5351,.T.);
#8074=ORIENTED_EDGE('',*,*,#6059,.T.);
#8075=ORIENTED_EDGE('',*,*,#5546,.T.);
#8076=ORIENTED_EDGE('',*,*,#6060,.T.);
#8077=ORIENTED_EDGE('',*,*,#5345,.T.);
#8078=ORIENTED_EDGE('',*,*,#6061,.T.);
#8079=ORIENTED_EDGE('',*,*,#5550,.T.);
#8080=ORIENTED_EDGE('',*,*,#6062,.T.);
#8081=ORIENTED_EDGE('',*,*,#5339,.T.);
#8082=ORIENTED_EDGE('',*,*,#6063,.T.);
#8083=ORIENTED_EDGE('',*,*,#5554,.T.);
#8084=ORIENTED_EDGE('',*,*,#6064,.T.);
#8085=ORIENTED_EDGE('',*,*,#5333,.T.);
#8086=ORIENTED_EDGE('',*,*,#6065,.T.);
#8087=ORIENTED_EDGE('',*,*,#5558,.T.);
#8088=ORIENTED_EDGE('',*,*,#6066,.T.);
#8089=ORIENTED_EDGE('',*,*,#5327,.T.);
#8090=ORIENTED_EDGE('',*,*,#6067,.T.);
#8091=ORIENTED_EDGE('',*,*,#5562,.T.);
#8092=ORIENTED_EDGE('',*,*,#6068,.T.);
#8093=ORIENTED_EDGE('',*,*,#5321,.T.);
#8094=ORIENTED_EDGE('',*,*,#6069,.T.);
#8095=ORIENTED_EDGE('',*,*,#5566,.T.);
#8096=ORIENTED_EDGE('',*,*,#6070,.T.);
#8097=ORIENTED_EDGE('',*,*,#5315,.T.);
#8098=ORIENTED_EDGE('',*,*,#6071,.T.);
#8099=ORIENTED_EDGE('',*,*,#5570,.T.);
#8100=ORIENTED_EDGE('',*,*,#6072,.T.);
#8101=ORIENTED_EDGE('',*,*,#5309,.T.);
#8102=ORIENTED_EDGE('',*,*,#6073,.T.);
#8103=ORIENTED_EDGE('',*,*,#5574,.T.);
#8104=ORIENTED_EDGE('',*,*,#6074,.T.);
#8105=ORIENTED_EDGE('',*,*,#5303,.T.);
#8106=ORIENTED_EDGE('',*,*,#6075,.T.);
#8107=ORIENTED_EDGE('',*,*,#5578,.T.);
#8108=ORIENTED_EDGE('',*,*,#6076,.T.);
#8109=ORIENTED_EDGE('',*,*,#5297,.T.);
#8110=ORIENTED_EDGE('',*,*,#6077,.T.);
#8111=ORIENTED_EDGE('',*,*,#5582,.T.);
#8112=ORIENTED_EDGE('',*,*,#6078,.T.);
#8113=ORIENTED_EDGE('',*,*,#5291,.T.);
#8114=ORIENTED_EDGE('',*,*,#6079,.T.);
#8115=ORIENTED_EDGE('',*,*,#5586,.T.);
#8116=ORIENTED_EDGE('',*,*,#6080,.T.);
#8117=ORIENTED_EDGE('',*,*,#5285,.T.);
#8118=ORIENTED_EDGE('',*,*,#6081,.T.);
#8119=ORIENTED_EDGE('',*,*,#5634,.T.);
#8120=ORIENTED_EDGE('',*,*,#5723,.F.);
#8121=ORIENTED_EDGE('',*,*,#6082,.F.);
#8122=ORIENTED_EDGE('',*,*,#6083,.T.);
#8123=ORIENTED_EDGE('',*,*,#6084,.T.);
#8124=ORIENTED_EDGE('',*,*,#5817,.T.);
#8125=ORIENTED_EDGE('',*,*,#6085,.T.);
#8126=ORIENTED_EDGE('',*,*,#5725,.T.);
#8127=ORIENTED_EDGE('',*,*,#6086,.F.);
#8128=ORIENTED_EDGE('',*,*,#6087,.F.);
#8129=ORIENTED_EDGE('',*,*,#6085,.F.);
#8130=ORIENTED_EDGE('',*,*,#6088,.F.);
#8131=ORIENTED_EDGE('',*,*,#6082,.T.);
#8132=ORIENTED_EDGE('',*,*,#5726,.T.);
#8133=ORIENTED_EDGE('',*,*,#6086,.T.);
#8134=ORIENTED_EDGE('',*,*,#5724,.F.);
#8135=ORIENTED_EDGE('',*,*,#6084,.F.);
#8136=ORIENTED_EDGE('',*,*,#6089,.T.);
#8137=ORIENTED_EDGE('',*,*,#6087,.T.);
#8138=ORIENTED_EDGE('',*,*,#6089,.F.);
#8139=ORIENTED_EDGE('',*,*,#6083,.F.);
#8140=ORIENTED_EDGE('',*,*,#6088,.T.);
#8141=ORIENTED_EDGE('',*,*,#5588,.T.);
#8142=ORIENTED_EDGE('',*,*,#6090,.F.);
#8143=ORIENTED_EDGE('',*,*,#6091,.F.);
#8144=ORIENTED_EDGE('',*,*,#6092,.F.);
#8145=ORIENTED_EDGE('',*,*,#6093,.T.);
#8146=ORIENTED_EDGE('',*,*,#5589,.T.);
#8147=ORIENTED_EDGE('',*,*,#6093,.F.);
#8148=ORIENTED_EDGE('',*,*,#6094,.F.);
#8149=ORIENTED_EDGE('',*,*,#5532,.F.);
#8150=ORIENTED_EDGE('',*,*,#5995,.F.);
#8151=ORIENTED_EDGE('',*,*,#5587,.T.);
#8152=ORIENTED_EDGE('',*,*,#6081,.F.);
#8153=ORIENTED_EDGE('',*,*,#5284,.F.);
#8154=ORIENTED_EDGE('',*,*,#6095,.F.);
#8155=ORIENTED_EDGE('',*,*,#6090,.T.);
#8156=ORIENTED_EDGE('',*,*,#6096,.F.);
#8157=ORIENTED_EDGE('',*,*,#6092,.T.);
#8158=ORIENTED_EDGE('',*,*,#6091,.T.);
#8159=ORIENTED_EDGE('',*,*,#6097,.T.);
#8160=ORIENTED_EDGE('',*,*,#5771,.F.);
#8161=ORIENTED_EDGE('',*,*,#5909,.T.);
#8162=ORIENTED_EDGE('',*,*,#5533,.T.);
#8163=ORIENTED_EDGE('',*,*,#6094,.T.);
#8164=ORIENTED_EDGE('',*,*,#6096,.T.);
#8165=ORIENTED_EDGE('',*,*,#5770,.F.);
#8166=ORIENTED_EDGE('',*,*,#6097,.F.);
#8167=ORIENTED_EDGE('',*,*,#6095,.T.);
#8168=ORIENTED_EDGE('',*,*,#5283,.T.);
#8169=ORIENTED_EDGE('',*,*,#5993,.T.);
#8170=ORIENTED_EDGE('',*,*,#5772,.F.);
#8171=ORIENTED_EDGE('',*,*,#6098,.F.);
#8172=ORIENTED_EDGE('',*,*,#6099,.T.);
#8173=ORIENTED_EDGE('',*,*,#5583,.T.);
#8174=ORIENTED_EDGE('',*,*,#6079,.F.);
#8175=ORIENTED_EDGE('',*,*,#5290,.F.);
#8176=ORIENTED_EDGE('',*,*,#6080,.F.);
#8177=ORIENTED_EDGE('',*,*,#5585,.T.);
#8178=ORIENTED_EDGE('',*,*,#6100,.F.);
#8179=ORIENTED_EDGE('',*,*,#6101,.F.);
#8180=ORIENTED_EDGE('',*,*,#5280,.F.);
#8181=ORIENTED_EDGE('',*,*,#5584,.T.);
#8182=ORIENTED_EDGE('',*,*,#6099,.F.);
#8183=ORIENTED_EDGE('',*,*,#6102,.F.);
#8184=ORIENTED_EDGE('',*,*,#6103,.F.);
#8185=ORIENTED_EDGE('',*,*,#6100,.T.);
#8186=ORIENTED_EDGE('',*,*,#6104,.F.);
#8187=ORIENTED_EDGE('',*,*,#6105,.T.);
#8188=ORIENTED_EDGE('',*,*,#5579,.T.);
#8189=ORIENTED_EDGE('',*,*,#6077,.F.);
#8190=ORIENTED_EDGE('',*,*,#5296,.F.);
#8191=ORIENTED_EDGE('',*,*,#6078,.F.);
#8192=ORIENTED_EDGE('',*,*,#5581,.T.);
#8193=ORIENTED_EDGE('',*,*,#6106,.F.);
#8194=ORIENTED_EDGE('',*,*,#6107,.F.);
#8195=ORIENTED_EDGE('',*,*,#5286,.F.);
#8196=ORIENTED_EDGE('',*,*,#5580,.T.);
#8197=ORIENTED_EDGE('',*,*,#6105,.F.);
#8198=ORIENTED_EDGE('',*,*,#6108,.F.);
#8199=ORIENTED_EDGE('',*,*,#6109,.F.);
#8200=ORIENTED_EDGE('',*,*,#6106,.T.);
#8201=ORIENTED_EDGE('',*,*,#6110,.F.);
#8202=ORIENTED_EDGE('',*,*,#6111,.T.);
#8203=ORIENTED_EDGE('',*,*,#5575,.T.);
#8204=ORIENTED_EDGE('',*,*,#6075,.F.);
#8205=ORIENTED_EDGE('',*,*,#5302,.F.);
#8206=ORIENTED_EDGE('',*,*,#6076,.F.);
#8207=ORIENTED_EDGE('',*,*,#5577,.T.);
#8208=ORIENTED_EDGE('',*,*,#6112,.F.);
#8209=ORIENTED_EDGE('',*,*,#6113,.F.);
#8210=ORIENTED_EDGE('',*,*,#5292,.F.);
#8211=ORIENTED_EDGE('',*,*,#5576,.T.);
#8212=ORIENTED_EDGE('',*,*,#6111,.F.);
#8213=ORIENTED_EDGE('',*,*,#6114,.F.);
#8214=ORIENTED_EDGE('',*,*,#6115,.F.);
#8215=ORIENTED_EDGE('',*,*,#6112,.T.);
#8216=ORIENTED_EDGE('',*,*,#6116,.F.);
#8217=ORIENTED_EDGE('',*,*,#6117,.T.);
#8218=ORIENTED_EDGE('',*,*,#5571,.T.);
#8219=ORIENTED_EDGE('',*,*,#6073,.F.);
#8220=ORIENTED_EDGE('',*,*,#5308,.F.);
#8221=ORIENTED_EDGE('',*,*,#6074,.F.);
#8222=ORIENTED_EDGE('',*,*,#5573,.T.);
#8223=ORIENTED_EDGE('',*,*,#6118,.F.);
#8224=ORIENTED_EDGE('',*,*,#6119,.F.);
#8225=ORIENTED_EDGE('',*,*,#5298,.F.);
#8226=ORIENTED_EDGE('',*,*,#5572,.T.);
#8227=ORIENTED_EDGE('',*,*,#6117,.F.);
#8228=ORIENTED_EDGE('',*,*,#6120,.F.);
#8229=ORIENTED_EDGE('',*,*,#6121,.F.);
#8230=ORIENTED_EDGE('',*,*,#6118,.T.);
#8231=ORIENTED_EDGE('',*,*,#6122,.F.);
#8232=ORIENTED_EDGE('',*,*,#6123,.T.);
#8233=ORIENTED_EDGE('',*,*,#5567,.T.);
#8234=ORIENTED_EDGE('',*,*,#6071,.F.);
#8235=ORIENTED_EDGE('',*,*,#5314,.F.);
#8236=ORIENTED_EDGE('',*,*,#6072,.F.);
#8237=ORIENTED_EDGE('',*,*,#5569,.T.);
#8238=ORIENTED_EDGE('',*,*,#6124,.F.);
#8239=ORIENTED_EDGE('',*,*,#6125,.F.);
#8240=ORIENTED_EDGE('',*,*,#5304,.F.);
#8241=ORIENTED_EDGE('',*,*,#5568,.T.);
#8242=ORIENTED_EDGE('',*,*,#6123,.F.);
#8243=ORIENTED_EDGE('',*,*,#6126,.F.);
#8244=ORIENTED_EDGE('',*,*,#6127,.F.);
#8245=ORIENTED_EDGE('',*,*,#6124,.T.);
#8246=ORIENTED_EDGE('',*,*,#6128,.F.);
#8247=ORIENTED_EDGE('',*,*,#6129,.T.);
#8248=ORIENTED_EDGE('',*,*,#5563,.T.);
#8249=ORIENTED_EDGE('',*,*,#6069,.F.);
#8250=ORIENTED_EDGE('',*,*,#5320,.F.);
#8251=ORIENTED_EDGE('',*,*,#6070,.F.);
#8252=ORIENTED_EDGE('',*,*,#5565,.T.);
#8253=ORIENTED_EDGE('',*,*,#6130,.F.);
#8254=ORIENTED_EDGE('',*,*,#6131,.F.);
#8255=ORIENTED_EDGE('',*,*,#5310,.F.);
#8256=ORIENTED_EDGE('',*,*,#5564,.T.);
#8257=ORIENTED_EDGE('',*,*,#6129,.F.);
#8258=ORIENTED_EDGE('',*,*,#6132,.F.);
#8259=ORIENTED_EDGE('',*,*,#6133,.F.);
#8260=ORIENTED_EDGE('',*,*,#6130,.T.);
#8261=ORIENTED_EDGE('',*,*,#6134,.F.);
#8262=ORIENTED_EDGE('',*,*,#6135,.T.);
#8263=ORIENTED_EDGE('',*,*,#5559,.T.);
#8264=ORIENTED_EDGE('',*,*,#6067,.F.);
#8265=ORIENTED_EDGE('',*,*,#5326,.F.);
#8266=ORIENTED_EDGE('',*,*,#6068,.F.);
#8267=ORIENTED_EDGE('',*,*,#5561,.T.);
#8268=ORIENTED_EDGE('',*,*,#6136,.F.);
#8269=ORIENTED_EDGE('',*,*,#6137,.F.);
#8270=ORIENTED_EDGE('',*,*,#5316,.F.);
#8271=ORIENTED_EDGE('',*,*,#5560,.T.);
#8272=ORIENTED_EDGE('',*,*,#6135,.F.);
#8273=ORIENTED_EDGE('',*,*,#6138,.F.);
#8274=ORIENTED_EDGE('',*,*,#6139,.F.);
#8275=ORIENTED_EDGE('',*,*,#6136,.T.);
#8276=ORIENTED_EDGE('',*,*,#6140,.F.);
#8277=ORIENTED_EDGE('',*,*,#6141,.T.);
#8278=ORIENTED_EDGE('',*,*,#5555,.T.);
#8279=ORIENTED_EDGE('',*,*,#6065,.F.);
#8280=ORIENTED_EDGE('',*,*,#5332,.F.);
#8281=ORIENTED_EDGE('',*,*,#6066,.F.);
#8282=ORIENTED_EDGE('',*,*,#5557,.T.);
#8283=ORIENTED_EDGE('',*,*,#6142,.F.);
#8284=ORIENTED_EDGE('',*,*,#6143,.F.);
#8285=ORIENTED_EDGE('',*,*,#5322,.F.);
#8286=ORIENTED_EDGE('',*,*,#5556,.T.);
#8287=ORIENTED_EDGE('',*,*,#6141,.F.);
#8288=ORIENTED_EDGE('',*,*,#6144,.F.);
#8289=ORIENTED_EDGE('',*,*,#6145,.F.);
#8290=ORIENTED_EDGE('',*,*,#6142,.T.);
#8291=ORIENTED_EDGE('',*,*,#6146,.F.);
#8292=ORIENTED_EDGE('',*,*,#6147,.T.);
#8293=ORIENTED_EDGE('',*,*,#5551,.T.);
#8294=ORIENTED_EDGE('',*,*,#6063,.F.);
#8295=ORIENTED_EDGE('',*,*,#5338,.F.);
#8296=ORIENTED_EDGE('',*,*,#6064,.F.);
#8297=ORIENTED_EDGE('',*,*,#5553,.T.);
#8298=ORIENTED_EDGE('',*,*,#6148,.F.);
#8299=ORIENTED_EDGE('',*,*,#6149,.F.);
#8300=ORIENTED_EDGE('',*,*,#5328,.F.);
#8301=ORIENTED_EDGE('',*,*,#5552,.T.);
#8302=ORIENTED_EDGE('',*,*,#6147,.F.);
#8303=ORIENTED_EDGE('',*,*,#6150,.F.);
#8304=ORIENTED_EDGE('',*,*,#6151,.F.);
#8305=ORIENTED_EDGE('',*,*,#6148,.T.);
#8306=ORIENTED_EDGE('',*,*,#6152,.F.);
#8307=ORIENTED_EDGE('',*,*,#6153,.T.);
#8308=ORIENTED_EDGE('',*,*,#5547,.T.);
#8309=ORIENTED_EDGE('',*,*,#6061,.F.);
#8310=ORIENTED_EDGE('',*,*,#5344,.F.);
#8311=ORIENTED_EDGE('',*,*,#6062,.F.);
#8312=ORIENTED_EDGE('',*,*,#5549,.T.);
#8313=ORIENTED_EDGE('',*,*,#6154,.F.);
#8314=ORIENTED_EDGE('',*,*,#6155,.F.);
#8315=ORIENTED_EDGE('',*,*,#5334,.F.);
#8316=ORIENTED_EDGE('',*,*,#5548,.T.);
#8317=ORIENTED_EDGE('',*,*,#6153,.F.);
#8318=ORIENTED_EDGE('',*,*,#6156,.F.);
#8319=ORIENTED_EDGE('',*,*,#6157,.F.);
#8320=ORIENTED_EDGE('',*,*,#6154,.T.);
#8321=ORIENTED_EDGE('',*,*,#6158,.F.);
#8322=ORIENTED_EDGE('',*,*,#6159,.T.);
#8323=ORIENTED_EDGE('',*,*,#5722,.T.);
#8324=ORIENTED_EDGE('',*,*,#6059,.F.);
#8325=ORIENTED_EDGE('',*,*,#5350,.F.);
#8326=ORIENTED_EDGE('',*,*,#6060,.F.);
#8327=ORIENTED_EDGE('',*,*,#5545,.T.);
#8328=ORIENTED_EDGE('',*,*,#6160,.F.);
#8329=ORIENTED_EDGE('',*,*,#6161,.F.);
#8330=ORIENTED_EDGE('',*,*,#5340,.F.);
#8331=ORIENTED_EDGE('',*,*,#5544,.T.);
#8332=ORIENTED_EDGE('',*,*,#6159,.F.);
#8333=ORIENTED_EDGE('',*,*,#6162,.F.);
#8334=ORIENTED_EDGE('',*,*,#6163,.F.);
#8335=ORIENTED_EDGE('',*,*,#6160,.T.);
#8336=ORIENTED_EDGE('',*,*,#6164,.F.);
#8337=ORIENTED_EDGE('',*,*,#6165,.T.);
#8338=ORIENTED_EDGE('',*,*,#5718,.T.);
#8339=ORIENTED_EDGE('',*,*,#6057,.F.);
#8340=ORIENTED_EDGE('',*,*,#5356,.F.);
#8341=ORIENTED_EDGE('',*,*,#6058,.F.);
#8342=ORIENTED_EDGE('',*,*,#5720,.T.);
#8343=ORIENTED_EDGE('',*,*,#6166,.F.);
#8344=ORIENTED_EDGE('',*,*,#6167,.F.);
#8345=ORIENTED_EDGE('',*,*,#5346,.F.);
#8346=ORIENTED_EDGE('',*,*,#5719,.T.);
#8347=ORIENTED_EDGE('',*,*,#6165,.F.);
#8348=ORIENTED_EDGE('',*,*,#6168,.F.);
#8349=ORIENTED_EDGE('',*,*,#6169,.F.);
#8350=ORIENTED_EDGE('',*,*,#6166,.T.);
#8351=ORIENTED_EDGE('',*,*,#6170,.F.);
#8352=ORIENTED_EDGE('',*,*,#6171,.T.);
#8353=ORIENTED_EDGE('',*,*,#5714,.T.);
#8354=ORIENTED_EDGE('',*,*,#6055,.F.);
#8355=ORIENTED_EDGE('',*,*,#5362,.F.);
#8356=ORIENTED_EDGE('',*,*,#6056,.F.);
#8357=ORIENTED_EDGE('',*,*,#5716,.T.);
#8358=ORIENTED_EDGE('',*,*,#6172,.F.);
#8359=ORIENTED_EDGE('',*,*,#6173,.F.);
#8360=ORIENTED_EDGE('',*,*,#5352,.F.);
#8361=ORIENTED_EDGE('',*,*,#5715,.T.);
#8362=ORIENTED_EDGE('',*,*,#6171,.F.);
#8363=ORIENTED_EDGE('',*,*,#6174,.F.);
#8364=ORIENTED_EDGE('',*,*,#6175,.F.);
#8365=ORIENTED_EDGE('',*,*,#6172,.T.);
#8366=ORIENTED_EDGE('',*,*,#6176,.F.);
#8367=ORIENTED_EDGE('',*,*,#6177,.T.);
#8368=ORIENTED_EDGE('',*,*,#5710,.T.);
#8369=ORIENTED_EDGE('',*,*,#6051,.F.);
#8370=ORIENTED_EDGE('',*,*,#5368,.F.);
#8371=ORIENTED_EDGE('',*,*,#6054,.F.);
#8372=ORIENTED_EDGE('',*,*,#5712,.T.);
#8373=ORIENTED_EDGE('',*,*,#6178,.F.);
#8374=ORIENTED_EDGE('',*,*,#6179,.F.);
#8375=ORIENTED_EDGE('',*,*,#5358,.F.);
#8376=ORIENTED_EDGE('',*,*,#5711,.T.);
#8377=ORIENTED_EDGE('',*,*,#6177,.F.);
#8378=ORIENTED_EDGE('',*,*,#6180,.F.);
#8379=ORIENTED_EDGE('',*,*,#6181,.F.);
#8380=ORIENTED_EDGE('',*,*,#6178,.T.);
#8381=ORIENTED_EDGE('',*,*,#6050,.F.);
#8382=ORIENTED_EDGE('',*,*,#5708,.T.);
#8383=ORIENTED_EDGE('',*,*,#6182,.F.);
#8384=ORIENTED_EDGE('',*,*,#6183,.F.);
#8385=ORIENTED_EDGE('',*,*,#5364,.F.);
#8386=ORIENTED_EDGE('',*,*,#6184,.F.);
#8387=ORIENTED_EDGE('',*,*,#6185,.T.);
#8388=ORIENTED_EDGE('',*,*,#5706,.T.);
#8389=ORIENTED_EDGE('',*,*,#6053,.F.);
#8390=ORIENTED_EDGE('',*,*,#5374,.F.);
#8391=ORIENTED_EDGE('',*,*,#5707,.T.);
#8392=ORIENTED_EDGE('',*,*,#6185,.F.);
#8393=ORIENTED_EDGE('',*,*,#6186,.F.);
#8394=ORIENTED_EDGE('',*,*,#6187,.F.);
#8395=ORIENTED_EDGE('',*,*,#6182,.T.);
#8396=ORIENTED_EDGE('',*,*,#6188,.F.);
#8397=ORIENTED_EDGE('',*,*,#6189,.T.);
#8398=ORIENTED_EDGE('',*,*,#5702,.T.);
#8399=ORIENTED_EDGE('',*,*,#6049,.F.);
#8400=ORIENTED_EDGE('',*,*,#5380,.F.);
#8401=ORIENTED_EDGE('',*,*,#6052,.F.);
#8402=ORIENTED_EDGE('',*,*,#5704,.T.);
#8403=ORIENTED_EDGE('',*,*,#6190,.F.);
#8404=ORIENTED_EDGE('',*,*,#6191,.F.);
#8405=ORIENTED_EDGE('',*,*,#5370,.F.);
#8406=ORIENTED_EDGE('',*,*,#5703,.T.);
#8407=ORIENTED_EDGE('',*,*,#6189,.F.);
#8408=ORIENTED_EDGE('',*,*,#6192,.F.);
#8409=ORIENTED_EDGE('',*,*,#6193,.F.);
#8410=ORIENTED_EDGE('',*,*,#6190,.T.);
#8411=ORIENTED_EDGE('',*,*,#6194,.F.);
#8412=ORIENTED_EDGE('',*,*,#6195,.T.);
#8413=ORIENTED_EDGE('',*,*,#5698,.T.);
#8414=ORIENTED_EDGE('',*,*,#6047,.F.);
#8415=ORIENTED_EDGE('',*,*,#5386,.F.);
#8416=ORIENTED_EDGE('',*,*,#6048,.F.);
#8417=ORIENTED_EDGE('',*,*,#5700,.T.);
#8418=ORIENTED_EDGE('',*,*,#6196,.F.);
#8419=ORIENTED_EDGE('',*,*,#6197,.F.);
#8420=ORIENTED_EDGE('',*,*,#5376,.F.);
#8421=ORIENTED_EDGE('',*,*,#5699,.T.);
#8422=ORIENTED_EDGE('',*,*,#6195,.F.);
#8423=ORIENTED_EDGE('',*,*,#6198,.F.);
#8424=ORIENTED_EDGE('',*,*,#6199,.F.);
#8425=ORIENTED_EDGE('',*,*,#6196,.T.);
#8426=ORIENTED_EDGE('',*,*,#6200,.F.);
#8427=ORIENTED_EDGE('',*,*,#6201,.T.);
#8428=ORIENTED_EDGE('',*,*,#5694,.T.);
#8429=ORIENTED_EDGE('',*,*,#6045,.F.);
#8430=ORIENTED_EDGE('',*,*,#5392,.F.);
#8431=ORIENTED_EDGE('',*,*,#6046,.F.);
#8432=ORIENTED_EDGE('',*,*,#5696,.T.);
#8433=ORIENTED_EDGE('',*,*,#6202,.F.);
#8434=ORIENTED_EDGE('',*,*,#6203,.F.);
#8435=ORIENTED_EDGE('',*,*,#5382,.F.);
#8436=ORIENTED_EDGE('',*,*,#5695,.T.);
#8437=ORIENTED_EDGE('',*,*,#6201,.F.);
#8438=ORIENTED_EDGE('',*,*,#6204,.F.);
#8439=ORIENTED_EDGE('',*,*,#6205,.F.);
#8440=ORIENTED_EDGE('',*,*,#6202,.T.);
#8441=ORIENTED_EDGE('',*,*,#6206,.F.);
#8442=ORIENTED_EDGE('',*,*,#6207,.T.);
#8443=ORIENTED_EDGE('',*,*,#5690,.T.);
#8444=ORIENTED_EDGE('',*,*,#6043,.F.);
#8445=ORIENTED_EDGE('',*,*,#5398,.F.);
#8446=ORIENTED_EDGE('',*,*,#6044,.F.);
#8447=ORIENTED_EDGE('',*,*,#5692,.T.);
#8448=ORIENTED_EDGE('',*,*,#6208,.F.);
#8449=ORIENTED_EDGE('',*,*,#6209,.F.);
#8450=ORIENTED_EDGE('',*,*,#5388,.F.);
#8451=ORIENTED_EDGE('',*,*,#5691,.T.);
#8452=ORIENTED_EDGE('',*,*,#6207,.F.);
#8453=ORIENTED_EDGE('',*,*,#6210,.F.);
#8454=ORIENTED_EDGE('',*,*,#6211,.F.);
#8455=ORIENTED_EDGE('',*,*,#6208,.T.);
#8456=ORIENTED_EDGE('',*,*,#6212,.F.);
#8457=ORIENTED_EDGE('',*,*,#6213,.T.);
#8458=ORIENTED_EDGE('',*,*,#5686,.T.);
#8459=ORIENTED_EDGE('',*,*,#6041,.F.);
#8460=ORIENTED_EDGE('',*,*,#5404,.F.);
#8461=ORIENTED_EDGE('',*,*,#6042,.F.);
#8462=ORIENTED_EDGE('',*,*,#5688,.T.);
#8463=ORIENTED_EDGE('',*,*,#6214,.F.);
#8464=ORIENTED_EDGE('',*,*,#6215,.F.);
#8465=ORIENTED_EDGE('',*,*,#5394,.F.);
#8466=ORIENTED_EDGE('',*,*,#5687,.T.);
#8467=ORIENTED_EDGE('',*,*,#6213,.F.);
#8468=ORIENTED_EDGE('',*,*,#6216,.F.);
#8469=ORIENTED_EDGE('',*,*,#6217,.F.);
#8470=ORIENTED_EDGE('',*,*,#6214,.T.);
#8471=ORIENTED_EDGE('',*,*,#6218,.F.);
#8472=ORIENTED_EDGE('',*,*,#6219,.T.);
#8473=ORIENTED_EDGE('',*,*,#5682,.T.);
#8474=ORIENTED_EDGE('',*,*,#6039,.F.);
#8475=ORIENTED_EDGE('',*,*,#5410,.F.);
#8476=ORIENTED_EDGE('',*,*,#6040,.F.);
#8477=ORIENTED_EDGE('',*,*,#5684,.T.);
#8478=ORIENTED_EDGE('',*,*,#6220,.F.);
#8479=ORIENTED_EDGE('',*,*,#6221,.F.);
#8480=ORIENTED_EDGE('',*,*,#5400,.F.);
#8481=ORIENTED_EDGE('',*,*,#5683,.T.);
#8482=ORIENTED_EDGE('',*,*,#6219,.F.);
#8483=ORIENTED_EDGE('',*,*,#6222,.F.);
#8484=ORIENTED_EDGE('',*,*,#6223,.F.);
#8485=ORIENTED_EDGE('',*,*,#6220,.T.);
#8486=ORIENTED_EDGE('',*,*,#6224,.F.);
#8487=ORIENTED_EDGE('',*,*,#6225,.T.);
#8488=ORIENTED_EDGE('',*,*,#5678,.T.);
#8489=ORIENTED_EDGE('',*,*,#6037,.F.);
#8490=ORIENTED_EDGE('',*,*,#5416,.F.);
#8491=ORIENTED_EDGE('',*,*,#6038,.F.);
#8492=ORIENTED_EDGE('',*,*,#5680,.T.);
#8493=ORIENTED_EDGE('',*,*,#6226,.F.);
#8494=ORIENTED_EDGE('',*,*,#6227,.F.);
#8495=ORIENTED_EDGE('',*,*,#5406,.F.);
#8496=ORIENTED_EDGE('',*,*,#5679,.T.);
#8497=ORIENTED_EDGE('',*,*,#6225,.F.);
#8498=ORIENTED_EDGE('',*,*,#6228,.F.);
#8499=ORIENTED_EDGE('',*,*,#6229,.F.);
#8500=ORIENTED_EDGE('',*,*,#6226,.T.);
#8501=ORIENTED_EDGE('',*,*,#6230,.F.);
#8502=ORIENTED_EDGE('',*,*,#6231,.T.);
#8503=ORIENTED_EDGE('',*,*,#5674,.T.);
#8504=ORIENTED_EDGE('',*,*,#6035,.F.);
#8505=ORIENTED_EDGE('',*,*,#5422,.F.);
#8506=ORIENTED_EDGE('',*,*,#6036,.F.);
#8507=ORIENTED_EDGE('',*,*,#5676,.T.);
#8508=ORIENTED_EDGE('',*,*,#6232,.F.);
#8509=ORIENTED_EDGE('',*,*,#6233,.F.);
#8510=ORIENTED_EDGE('',*,*,#5412,.F.);
#8511=ORIENTED_EDGE('',*,*,#5675,.T.);
#8512=ORIENTED_EDGE('',*,*,#6231,.F.);
#8513=ORIENTED_EDGE('',*,*,#6234,.F.);
#8514=ORIENTED_EDGE('',*,*,#6235,.F.);
#8515=ORIENTED_EDGE('',*,*,#6232,.T.);
#8516=ORIENTED_EDGE('',*,*,#6236,.F.);
#8517=ORIENTED_EDGE('',*,*,#6237,.T.);
#8518=ORIENTED_EDGE('',*,*,#5670,.T.);
#8519=ORIENTED_EDGE('',*,*,#6033,.F.);
#8520=ORIENTED_EDGE('',*,*,#5428,.F.);
#8521=ORIENTED_EDGE('',*,*,#6034,.F.);
#8522=ORIENTED_EDGE('',*,*,#5672,.T.);
#8523=ORIENTED_EDGE('',*,*,#6238,.F.);
#8524=ORIENTED_EDGE('',*,*,#6239,.F.);
#8525=ORIENTED_EDGE('',*,*,#5418,.F.);
#8526=ORIENTED_EDGE('',*,*,#5671,.T.);
#8527=ORIENTED_EDGE('',*,*,#6237,.F.);
#8528=ORIENTED_EDGE('',*,*,#6240,.F.);
#8529=ORIENTED_EDGE('',*,*,#6241,.F.);
#8530=ORIENTED_EDGE('',*,*,#6238,.T.);
#8531=ORIENTED_EDGE('',*,*,#6242,.F.);
#8532=ORIENTED_EDGE('',*,*,#6243,.T.);
#8533=ORIENTED_EDGE('',*,*,#5666,.T.);
#8534=ORIENTED_EDGE('',*,*,#6031,.F.);
#8535=ORIENTED_EDGE('',*,*,#5434,.F.);
#8536=ORIENTED_EDGE('',*,*,#6032,.F.);
#8537=ORIENTED_EDGE('',*,*,#5668,.T.);
#8538=ORIENTED_EDGE('',*,*,#6244,.F.);
#8539=ORIENTED_EDGE('',*,*,#6245,.F.);
#8540=ORIENTED_EDGE('',*,*,#5424,.F.);
#8541=ORIENTED_EDGE('',*,*,#5667,.T.);
#8542=ORIENTED_EDGE('',*,*,#6243,.F.);
#8543=ORIENTED_EDGE('',*,*,#6246,.F.);
#8544=ORIENTED_EDGE('',*,*,#6247,.F.);
#8545=ORIENTED_EDGE('',*,*,#6244,.T.);
#8546=ORIENTED_EDGE('',*,*,#6248,.F.);
#8547=ORIENTED_EDGE('',*,*,#6249,.T.);
#8548=ORIENTED_EDGE('',*,*,#5662,.T.);
#8549=ORIENTED_EDGE('',*,*,#6029,.F.);
#8550=ORIENTED_EDGE('',*,*,#5440,.F.);
#8551=ORIENTED_EDGE('',*,*,#6030,.F.);
#8552=ORIENTED_EDGE('',*,*,#5664,.T.);
#8553=ORIENTED_EDGE('',*,*,#6250,.F.);
#8554=ORIENTED_EDGE('',*,*,#6251,.F.);
#8555=ORIENTED_EDGE('',*,*,#5430,.F.);
#8556=ORIENTED_EDGE('',*,*,#5663,.T.);
#8557=ORIENTED_EDGE('',*,*,#6249,.F.);
#8558=ORIENTED_EDGE('',*,*,#6252,.F.);
#8559=ORIENTED_EDGE('',*,*,#6253,.F.);
#8560=ORIENTED_EDGE('',*,*,#6250,.T.);
#8561=ORIENTED_EDGE('',*,*,#6254,.F.);
#8562=ORIENTED_EDGE('',*,*,#6255,.T.);
#8563=ORIENTED_EDGE('',*,*,#5658,.T.);
#8564=ORIENTED_EDGE('',*,*,#6027,.F.);
#8565=ORIENTED_EDGE('',*,*,#5446,.F.);
#8566=ORIENTED_EDGE('',*,*,#6028,.F.);
#8567=ORIENTED_EDGE('',*,*,#5660,.T.);
#8568=ORIENTED_EDGE('',*,*,#6256,.F.);
#8569=ORIENTED_EDGE('',*,*,#6257,.F.);
#8570=ORIENTED_EDGE('',*,*,#5436,.F.);
#8571=ORIENTED_EDGE('',*,*,#5659,.T.);
#8572=ORIENTED_EDGE('',*,*,#6255,.F.);
#8573=ORIENTED_EDGE('',*,*,#6258,.F.);
#8574=ORIENTED_EDGE('',*,*,#6259,.F.);
#8575=ORIENTED_EDGE('',*,*,#6256,.T.);
#8576=ORIENTED_EDGE('',*,*,#6260,.F.);
#8577=ORIENTED_EDGE('',*,*,#6261,.T.);
#8578=ORIENTED_EDGE('',*,*,#5654,.T.);
#8579=ORIENTED_EDGE('',*,*,#6025,.F.);
#8580=ORIENTED_EDGE('',*,*,#5452,.F.);
#8581=ORIENTED_EDGE('',*,*,#6026,.F.);
#8582=ORIENTED_EDGE('',*,*,#5656,.T.);
#8583=ORIENTED_EDGE('',*,*,#6262,.F.);
#8584=ORIENTED_EDGE('',*,*,#6263,.F.);
#8585=ORIENTED_EDGE('',*,*,#5442,.F.);
#8586=ORIENTED_EDGE('',*,*,#5655,.T.);
#8587=ORIENTED_EDGE('',*,*,#6261,.F.);
#8588=ORIENTED_EDGE('',*,*,#6264,.F.);
#8589=ORIENTED_EDGE('',*,*,#6265,.F.);
#8590=ORIENTED_EDGE('',*,*,#6262,.T.);
#8591=ORIENTED_EDGE('',*,*,#6266,.F.);
#8592=ORIENTED_EDGE('',*,*,#6267,.T.);
#8593=ORIENTED_EDGE('',*,*,#5650,.T.);
#8594=ORIENTED_EDGE('',*,*,#6023,.F.);
#8595=ORIENTED_EDGE('',*,*,#5458,.F.);
#8596=ORIENTED_EDGE('',*,*,#6024,.F.);
#8597=ORIENTED_EDGE('',*,*,#5652,.T.);
#8598=ORIENTED_EDGE('',*,*,#6268,.F.);
#8599=ORIENTED_EDGE('',*,*,#6269,.F.);
#8600=ORIENTED_EDGE('',*,*,#5448,.F.);
#8601=ORIENTED_EDGE('',*,*,#5651,.T.);
#8602=ORIENTED_EDGE('',*,*,#6267,.F.);
#8603=ORIENTED_EDGE('',*,*,#6270,.F.);
#8604=ORIENTED_EDGE('',*,*,#6271,.F.);
#8605=ORIENTED_EDGE('',*,*,#6268,.T.);
#8606=ORIENTED_EDGE('',*,*,#6272,.F.);
#8607=ORIENTED_EDGE('',*,*,#6273,.T.);
#8608=ORIENTED_EDGE('',*,*,#5646,.T.);
#8609=ORIENTED_EDGE('',*,*,#6021,.F.);
#8610=ORIENTED_EDGE('',*,*,#5464,.F.);
#8611=ORIENTED_EDGE('',*,*,#6022,.F.);
#8612=ORIENTED_EDGE('',*,*,#5648,.T.);
#8613=ORIENTED_EDGE('',*,*,#6274,.F.);
#8614=ORIENTED_EDGE('',*,*,#6275,.F.);
#8615=ORIENTED_EDGE('',*,*,#5454,.F.);
#8616=ORIENTED_EDGE('',*,*,#5647,.T.);
#8617=ORIENTED_EDGE('',*,*,#6273,.F.);
#8618=ORIENTED_EDGE('',*,*,#6276,.F.);
#8619=ORIENTED_EDGE('',*,*,#6277,.F.);
#8620=ORIENTED_EDGE('',*,*,#6274,.T.);
#8621=ORIENTED_EDGE('',*,*,#6278,.F.);
#8622=ORIENTED_EDGE('',*,*,#6279,.T.);
#8623=ORIENTED_EDGE('',*,*,#5642,.T.);
#8624=ORIENTED_EDGE('',*,*,#6019,.F.);
#8625=ORIENTED_EDGE('',*,*,#5470,.F.);
#8626=ORIENTED_EDGE('',*,*,#6020,.F.);
#8627=ORIENTED_EDGE('',*,*,#5644,.T.);
#8628=ORIENTED_EDGE('',*,*,#6280,.F.);
#8629=ORIENTED_EDGE('',*,*,#6281,.F.);
#8630=ORIENTED_EDGE('',*,*,#5460,.F.);
#8631=ORIENTED_EDGE('',*,*,#5643,.T.);
#8632=ORIENTED_EDGE('',*,*,#6279,.F.);
#8633=ORIENTED_EDGE('',*,*,#6282,.F.);
#8634=ORIENTED_EDGE('',*,*,#6283,.F.);
#8635=ORIENTED_EDGE('',*,*,#6280,.T.);
#8636=ORIENTED_EDGE('',*,*,#6284,.F.);
#8637=ORIENTED_EDGE('',*,*,#6285,.T.);
#8638=ORIENTED_EDGE('',*,*,#5638,.T.);
#8639=ORIENTED_EDGE('',*,*,#6017,.F.);
#8640=ORIENTED_EDGE('',*,*,#5476,.F.);
#8641=ORIENTED_EDGE('',*,*,#6018,.F.);
#8642=ORIENTED_EDGE('',*,*,#5640,.T.);
#8643=ORIENTED_EDGE('',*,*,#6286,.F.);
#8644=ORIENTED_EDGE('',*,*,#6287,.F.);
#8645=ORIENTED_EDGE('',*,*,#5466,.F.);
#8646=ORIENTED_EDGE('',*,*,#5639,.T.);
#8647=ORIENTED_EDGE('',*,*,#6285,.F.);
#8648=ORIENTED_EDGE('',*,*,#6288,.F.);
#8649=ORIENTED_EDGE('',*,*,#6289,.F.);
#8650=ORIENTED_EDGE('',*,*,#6286,.T.);
#8651=ORIENTED_EDGE('',*,*,#6290,.F.);
#8652=ORIENTED_EDGE('',*,*,#6291,.T.);
#8653=ORIENTED_EDGE('',*,*,#5631,.T.);
#8654=ORIENTED_EDGE('',*,*,#6015,.F.);
#8655=ORIENTED_EDGE('',*,*,#5482,.F.);
#8656=ORIENTED_EDGE('',*,*,#6016,.F.);
#8657=ORIENTED_EDGE('',*,*,#5636,.T.);
#8658=ORIENTED_EDGE('',*,*,#6292,.F.);
#8659=ORIENTED_EDGE('',*,*,#6293,.F.);
#8660=ORIENTED_EDGE('',*,*,#5472,.F.);
#8661=ORIENTED_EDGE('',*,*,#5635,.T.);
#8662=ORIENTED_EDGE('',*,*,#5632,.T.);
#8663=ORIENTED_EDGE('',*,*,#6291,.F.);
#8664=ORIENTED_EDGE('',*,*,#6294,.F.);
#8665=ORIENTED_EDGE('',*,*,#6295,.F.);
#8666=ORIENTED_EDGE('',*,*,#6292,.T.);
#8667=ORIENTED_EDGE('',*,*,#6296,.F.);
#8668=ORIENTED_EDGE('',*,*,#6297,.T.);
#8669=ORIENTED_EDGE('',*,*,#5627,.T.);
#8670=ORIENTED_EDGE('',*,*,#6013,.F.);
#8671=ORIENTED_EDGE('',*,*,#5488,.F.);
#8672=ORIENTED_EDGE('',*,*,#6014,.F.);
#8673=ORIENTED_EDGE('',*,*,#5629,.T.);
#8674=ORIENTED_EDGE('',*,*,#6298,.F.);
#8675=ORIENTED_EDGE('',*,*,#6299,.F.);
#8676=ORIENTED_EDGE('',*,*,#5478,.F.);
#8677=ORIENTED_EDGE('',*,*,#5628,.T.);
#8678=ORIENTED_EDGE('',*,*,#6297,.F.);
#8679=ORIENTED_EDGE('',*,*,#6300,.F.);
#8680=ORIENTED_EDGE('',*,*,#6301,.F.);
#8681=ORIENTED_EDGE('',*,*,#6298,.T.);
#8682=ORIENTED_EDGE('',*,*,#6302,.F.);
#8683=ORIENTED_EDGE('',*,*,#6303,.T.);
#8684=ORIENTED_EDGE('',*,*,#5623,.T.);
#8685=ORIENTED_EDGE('',*,*,#6011,.F.);
#8686=ORIENTED_EDGE('',*,*,#5494,.F.);
#8687=ORIENTED_EDGE('',*,*,#6012,.F.);
#8688=ORIENTED_EDGE('',*,*,#5625,.T.);
#8689=ORIENTED_EDGE('',*,*,#6304,.F.);
#8690=ORIENTED_EDGE('',*,*,#6305,.F.);
#8691=ORIENTED_EDGE('',*,*,#5484,.F.);
#8692=ORIENTED_EDGE('',*,*,#5624,.T.);
#8693=ORIENTED_EDGE('',*,*,#6303,.F.);
#8694=ORIENTED_EDGE('',*,*,#6306,.F.);
#8695=ORIENTED_EDGE('',*,*,#6307,.F.);
#8696=ORIENTED_EDGE('',*,*,#6304,.T.);
#8697=ORIENTED_EDGE('',*,*,#6308,.F.);
#8698=ORIENTED_EDGE('',*,*,#6309,.T.);
#8699=ORIENTED_EDGE('',*,*,#5619,.T.);
#8700=ORIENTED_EDGE('',*,*,#6007,.F.);
#8701=ORIENTED_EDGE('',*,*,#5500,.F.);
#8702=ORIENTED_EDGE('',*,*,#6010,.F.);
#8703=ORIENTED_EDGE('',*,*,#5621,.T.);
#8704=ORIENTED_EDGE('',*,*,#6310,.F.);
#8705=ORIENTED_EDGE('',*,*,#6311,.F.);
#8706=ORIENTED_EDGE('',*,*,#5490,.F.);
#8707=ORIENTED_EDGE('',*,*,#5620,.T.);
#8708=ORIENTED_EDGE('',*,*,#6309,.F.);
#8709=ORIENTED_EDGE('',*,*,#6312,.F.);
#8710=ORIENTED_EDGE('',*,*,#6313,.F.);
#8711=ORIENTED_EDGE('',*,*,#6310,.T.);
#8712=ORIENTED_EDGE('',*,*,#6006,.F.);
#8713=ORIENTED_EDGE('',*,*,#5617,.T.);
#8714=ORIENTED_EDGE('',*,*,#6314,.F.);
#8715=ORIENTED_EDGE('',*,*,#6315,.F.);
#8716=ORIENTED_EDGE('',*,*,#5496,.F.);
#8717=ORIENTED_EDGE('',*,*,#6316,.F.);
#8718=ORIENTED_EDGE('',*,*,#6317,.T.);
#8719=ORIENTED_EDGE('',*,*,#5615,.T.);
#8720=ORIENTED_EDGE('',*,*,#6009,.F.);
#8721=ORIENTED_EDGE('',*,*,#5506,.F.);
#8722=ORIENTED_EDGE('',*,*,#5616,.T.);
#8723=ORIENTED_EDGE('',*,*,#6317,.F.);
#8724=ORIENTED_EDGE('',*,*,#6318,.F.);
#8725=ORIENTED_EDGE('',*,*,#6319,.F.);
#8726=ORIENTED_EDGE('',*,*,#6314,.T.);
#8727=ORIENTED_EDGE('',*,*,#6320,.F.);
#8728=ORIENTED_EDGE('',*,*,#6321,.T.);
#8729=ORIENTED_EDGE('',*,*,#5611,.T.);
#8730=ORIENTED_EDGE('',*,*,#6005,.F.);
#8731=ORIENTED_EDGE('',*,*,#5512,.F.);
#8732=ORIENTED_EDGE('',*,*,#6008,.F.);
#8733=ORIENTED_EDGE('',*,*,#5613,.T.);
#8734=ORIENTED_EDGE('',*,*,#6322,.F.);
#8735=ORIENTED_EDGE('',*,*,#6323,.F.);
#8736=ORIENTED_EDGE('',*,*,#5502,.F.);
#8737=ORIENTED_EDGE('',*,*,#5612,.T.);
#8738=ORIENTED_EDGE('',*,*,#6321,.F.);
#8739=ORIENTED_EDGE('',*,*,#6324,.F.);
#8740=ORIENTED_EDGE('',*,*,#6325,.F.);
#8741=ORIENTED_EDGE('',*,*,#6322,.T.);
#8742=ORIENTED_EDGE('',*,*,#6326,.F.);
#8743=ORIENTED_EDGE('',*,*,#6327,.T.);
#8744=ORIENTED_EDGE('',*,*,#5607,.T.);
#8745=ORIENTED_EDGE('',*,*,#6003,.F.);
#8746=ORIENTED_EDGE('',*,*,#5518,.F.);
#8747=ORIENTED_EDGE('',*,*,#6004,.F.);
#8748=ORIENTED_EDGE('',*,*,#5609,.T.);
#8749=ORIENTED_EDGE('',*,*,#6328,.F.);
#8750=ORIENTED_EDGE('',*,*,#6329,.F.);
#8751=ORIENTED_EDGE('',*,*,#5508,.F.);
#8752=ORIENTED_EDGE('',*,*,#5608,.T.);
#8753=ORIENTED_EDGE('',*,*,#6327,.F.);
#8754=ORIENTED_EDGE('',*,*,#6330,.F.);
#8755=ORIENTED_EDGE('',*,*,#6331,.F.);
#8756=ORIENTED_EDGE('',*,*,#6328,.T.);
#8757=ORIENTED_EDGE('',*,*,#6332,.F.);
#8758=ORIENTED_EDGE('',*,*,#6333,.T.);
#8759=ORIENTED_EDGE('',*,*,#5603,.T.);
#8760=ORIENTED_EDGE('',*,*,#6001,.F.);
#8761=ORIENTED_EDGE('',*,*,#5524,.F.);
#8762=ORIENTED_EDGE('',*,*,#6002,.F.);
#8763=ORIENTED_EDGE('',*,*,#5605,.T.);
#8764=ORIENTED_EDGE('',*,*,#6334,.F.);
#8765=ORIENTED_EDGE('',*,*,#6335,.F.);
#8766=ORIENTED_EDGE('',*,*,#5514,.F.);
#8767=ORIENTED_EDGE('',*,*,#5604,.T.);
#8768=ORIENTED_EDGE('',*,*,#6333,.F.);
#8769=ORIENTED_EDGE('',*,*,#6336,.F.);
#8770=ORIENTED_EDGE('',*,*,#6337,.F.);
#8771=ORIENTED_EDGE('',*,*,#6334,.T.);
#8772=ORIENTED_EDGE('',*,*,#6338,.F.);
#8773=ORIENTED_EDGE('',*,*,#6339,.T.);
#8774=ORIENTED_EDGE('',*,*,#5599,.T.);
#8775=ORIENTED_EDGE('',*,*,#5999,.F.);
#8776=ORIENTED_EDGE('',*,*,#5530,.F.);
#8777=ORIENTED_EDGE('',*,*,#6000,.F.);
#8778=ORIENTED_EDGE('',*,*,#5601,.T.);
#8779=ORIENTED_EDGE('',*,*,#6340,.F.);
#8780=ORIENTED_EDGE('',*,*,#6341,.F.);
#8781=ORIENTED_EDGE('',*,*,#5520,.F.);
#8782=ORIENTED_EDGE('',*,*,#5600,.T.);
#8783=ORIENTED_EDGE('',*,*,#6339,.F.);
#8784=ORIENTED_EDGE('',*,*,#6342,.F.);
#8785=ORIENTED_EDGE('',*,*,#6343,.F.);
#8786=ORIENTED_EDGE('',*,*,#6340,.T.);
#8787=ORIENTED_EDGE('',*,*,#6344,.F.);
#8788=ORIENTED_EDGE('',*,*,#6345,.T.);
#8789=ORIENTED_EDGE('',*,*,#5595,.T.);
#8790=ORIENTED_EDGE('',*,*,#5997,.F.);
#8791=ORIENTED_EDGE('',*,*,#5542,.F.);
#8792=ORIENTED_EDGE('',*,*,#5998,.F.);
#8793=ORIENTED_EDGE('',*,*,#5597,.T.);
#8794=ORIENTED_EDGE('',*,*,#6346,.F.);
#8795=ORIENTED_EDGE('',*,*,#6347,.F.);
#8796=ORIENTED_EDGE('',*,*,#5526,.F.);
#8797=ORIENTED_EDGE('',*,*,#5596,.T.);
#8798=ORIENTED_EDGE('',*,*,#6345,.F.);
#8799=ORIENTED_EDGE('',*,*,#6348,.F.);
#8800=ORIENTED_EDGE('',*,*,#6349,.F.);
#8801=ORIENTED_EDGE('',*,*,#6346,.T.);
#8802=ORIENTED_EDGE('',*,*,#6350,.F.);
#8803=ORIENTED_EDGE('',*,*,#6351,.T.);
#8804=ORIENTED_EDGE('',*,*,#5591,.T.);
#8805=ORIENTED_EDGE('',*,*,#5994,.F.);
#8806=ORIENTED_EDGE('',*,*,#5536,.F.);
#8807=ORIENTED_EDGE('',*,*,#5996,.F.);
#8808=ORIENTED_EDGE('',*,*,#5593,.T.);
#8809=ORIENTED_EDGE('',*,*,#6352,.F.);
#8810=ORIENTED_EDGE('',*,*,#6353,.F.);
#8811=ORIENTED_EDGE('',*,*,#5538,.F.);
#8812=ORIENTED_EDGE('',*,*,#5592,.T.);
#8813=ORIENTED_EDGE('',*,*,#6351,.F.);
#8814=ORIENTED_EDGE('',*,*,#6354,.F.);
#8815=ORIENTED_EDGE('',*,*,#6355,.F.);
#8816=ORIENTED_EDGE('',*,*,#6352,.T.);
#8817=ORIENTED_EDGE('',*,*,#6356,.F.);
#8818=ORIENTED_EDGE('',*,*,#6103,.T.);
#8819=ORIENTED_EDGE('',*,*,#6102,.T.);
#8820=ORIENTED_EDGE('',*,*,#6357,.T.);
#8821=ORIENTED_EDGE('',*,*,#5775,.F.);
#8822=ORIENTED_EDGE('',*,*,#5992,.T.);
#8823=ORIENTED_EDGE('',*,*,#5281,.T.);
#8824=ORIENTED_EDGE('',*,*,#6101,.T.);
#8825=ORIENTED_EDGE('',*,*,#6356,.T.);
#8826=ORIENTED_EDGE('',*,*,#5774,.F.);
#8827=ORIENTED_EDGE('',*,*,#6357,.F.);
#8828=ORIENTED_EDGE('',*,*,#6098,.T.);
#8829=ORIENTED_EDGE('',*,*,#5289,.T.);
#8830=ORIENTED_EDGE('',*,*,#5991,.T.);
#8831=ORIENTED_EDGE('',*,*,#5776,.F.);
#8832=ORIENTED_EDGE('',*,*,#6358,.F.);
#8833=ORIENTED_EDGE('',*,*,#6109,.T.);
#8834=ORIENTED_EDGE('',*,*,#6108,.T.);
#8835=ORIENTED_EDGE('',*,*,#6359,.T.);
#8836=ORIENTED_EDGE('',*,*,#5779,.F.);
#8837=ORIENTED_EDGE('',*,*,#5990,.T.);
#8838=ORIENTED_EDGE('',*,*,#5287,.T.);
#8839=ORIENTED_EDGE('',*,*,#6107,.T.);
#8840=ORIENTED_EDGE('',*,*,#6358,.T.);
#8841=ORIENTED_EDGE('',*,*,#5778,.F.);
#8842=ORIENTED_EDGE('',*,*,#6359,.F.);
#8843=ORIENTED_EDGE('',*,*,#6104,.T.);
#8844=ORIENTED_EDGE('',*,*,#5295,.T.);
#8845=ORIENTED_EDGE('',*,*,#5989,.T.);
#8846=ORIENTED_EDGE('',*,*,#5780,.F.);
#8847=ORIENTED_EDGE('',*,*,#6360,.F.);
#8848=ORIENTED_EDGE('',*,*,#6115,.T.);
#8849=ORIENTED_EDGE('',*,*,#6114,.T.);
#8850=ORIENTED_EDGE('',*,*,#6361,.T.);
#8851=ORIENTED_EDGE('',*,*,#5783,.F.);
#8852=ORIENTED_EDGE('',*,*,#5988,.T.);
#8853=ORIENTED_EDGE('',*,*,#5293,.T.);
#8854=ORIENTED_EDGE('',*,*,#6113,.T.);
#8855=ORIENTED_EDGE('',*,*,#6360,.T.);
#8856=ORIENTED_EDGE('',*,*,#5782,.F.);
#8857=ORIENTED_EDGE('',*,*,#6361,.F.);
#8858=ORIENTED_EDGE('',*,*,#6110,.T.);
#8859=ORIENTED_EDGE('',*,*,#5301,.T.);
#8860=ORIENTED_EDGE('',*,*,#5987,.T.);
#8861=ORIENTED_EDGE('',*,*,#5784,.F.);
#8862=ORIENTED_EDGE('',*,*,#6362,.F.);
#8863=ORIENTED_EDGE('',*,*,#6121,.T.);
#8864=ORIENTED_EDGE('',*,*,#6120,.T.);
#8865=ORIENTED_EDGE('',*,*,#6363,.T.);
#8866=ORIENTED_EDGE('',*,*,#5787,.F.);
#8867=ORIENTED_EDGE('',*,*,#5986,.T.);
#8868=ORIENTED_EDGE('',*,*,#5299,.T.);
#8869=ORIENTED_EDGE('',*,*,#6119,.T.);
#8870=ORIENTED_EDGE('',*,*,#6362,.T.);
#8871=ORIENTED_EDGE('',*,*,#5786,.F.);
#8872=ORIENTED_EDGE('',*,*,#6363,.F.);
#8873=ORIENTED_EDGE('',*,*,#6116,.T.);
#8874=ORIENTED_EDGE('',*,*,#5307,.T.);
#8875=ORIENTED_EDGE('',*,*,#5985,.T.);
#8876=ORIENTED_EDGE('',*,*,#5788,.F.);
#8877=ORIENTED_EDGE('',*,*,#6364,.F.);
#8878=ORIENTED_EDGE('',*,*,#6127,.T.);
#8879=ORIENTED_EDGE('',*,*,#6126,.T.);
#8880=ORIENTED_EDGE('',*,*,#6365,.T.);
#8881=ORIENTED_EDGE('',*,*,#5791,.F.);
#8882=ORIENTED_EDGE('',*,*,#5984,.T.);
#8883=ORIENTED_EDGE('',*,*,#5305,.T.);
#8884=ORIENTED_EDGE('',*,*,#6125,.T.);
#8885=ORIENTED_EDGE('',*,*,#6364,.T.);
#8886=ORIENTED_EDGE('',*,*,#5790,.F.);
#8887=ORIENTED_EDGE('',*,*,#6365,.F.);
#8888=ORIENTED_EDGE('',*,*,#6122,.T.);
#8889=ORIENTED_EDGE('',*,*,#5313,.T.);
#8890=ORIENTED_EDGE('',*,*,#5983,.T.);
#8891=ORIENTED_EDGE('',*,*,#5792,.F.);
#8892=ORIENTED_EDGE('',*,*,#6366,.F.);
#8893=ORIENTED_EDGE('',*,*,#6133,.T.);
#8894=ORIENTED_EDGE('',*,*,#6132,.T.);
#8895=ORIENTED_EDGE('',*,*,#6367,.T.);
#8896=ORIENTED_EDGE('',*,*,#5795,.F.);
#8897=ORIENTED_EDGE('',*,*,#5982,.T.);
#8898=ORIENTED_EDGE('',*,*,#5311,.T.);
#8899=ORIENTED_EDGE('',*,*,#6131,.T.);
#8900=ORIENTED_EDGE('',*,*,#6366,.T.);
#8901=ORIENTED_EDGE('',*,*,#5794,.F.);
#8902=ORIENTED_EDGE('',*,*,#6367,.F.);
#8903=ORIENTED_EDGE('',*,*,#6128,.T.);
#8904=ORIENTED_EDGE('',*,*,#5319,.T.);
#8905=ORIENTED_EDGE('',*,*,#5981,.T.);
#8906=ORIENTED_EDGE('',*,*,#5796,.F.);
#8907=ORIENTED_EDGE('',*,*,#6368,.F.);
#8908=ORIENTED_EDGE('',*,*,#6139,.T.);
#8909=ORIENTED_EDGE('',*,*,#6138,.T.);
#8910=ORIENTED_EDGE('',*,*,#6369,.T.);
#8911=ORIENTED_EDGE('',*,*,#5799,.F.);
#8912=ORIENTED_EDGE('',*,*,#5980,.T.);
#8913=ORIENTED_EDGE('',*,*,#5317,.T.);
#8914=ORIENTED_EDGE('',*,*,#6137,.T.);
#8915=ORIENTED_EDGE('',*,*,#6368,.T.);
#8916=ORIENTED_EDGE('',*,*,#5798,.F.);
#8917=ORIENTED_EDGE('',*,*,#6369,.F.);
#8918=ORIENTED_EDGE('',*,*,#6134,.T.);
#8919=ORIENTED_EDGE('',*,*,#5325,.T.);
#8920=ORIENTED_EDGE('',*,*,#5979,.T.);
#8921=ORIENTED_EDGE('',*,*,#5800,.F.);
#8922=ORIENTED_EDGE('',*,*,#6370,.F.);
#8923=ORIENTED_EDGE('',*,*,#6145,.T.);
#8924=ORIENTED_EDGE('',*,*,#6144,.T.);
#8925=ORIENTED_EDGE('',*,*,#6371,.T.);
#8926=ORIENTED_EDGE('',*,*,#5803,.F.);
#8927=ORIENTED_EDGE('',*,*,#5978,.T.);
#8928=ORIENTED_EDGE('',*,*,#5323,.T.);
#8929=ORIENTED_EDGE('',*,*,#6143,.T.);
#8930=ORIENTED_EDGE('',*,*,#6370,.T.);
#8931=ORIENTED_EDGE('',*,*,#5802,.F.);
#8932=ORIENTED_EDGE('',*,*,#6371,.F.);
#8933=ORIENTED_EDGE('',*,*,#6140,.T.);
#8934=ORIENTED_EDGE('',*,*,#5331,.T.);
#8935=ORIENTED_EDGE('',*,*,#5977,.T.);
#8936=ORIENTED_EDGE('',*,*,#5804,.F.);
#8937=ORIENTED_EDGE('',*,*,#6372,.F.);
#8938=ORIENTED_EDGE('',*,*,#6151,.T.);
#8939=ORIENTED_EDGE('',*,*,#6150,.T.);
#8940=ORIENTED_EDGE('',*,*,#6373,.T.);
#8941=ORIENTED_EDGE('',*,*,#5807,.F.);
#8942=ORIENTED_EDGE('',*,*,#5976,.T.);
#8943=ORIENTED_EDGE('',*,*,#5329,.T.);
#8944=ORIENTED_EDGE('',*,*,#6149,.T.);
#8945=ORIENTED_EDGE('',*,*,#6372,.T.);
#8946=ORIENTED_EDGE('',*,*,#5806,.F.);
#8947=ORIENTED_EDGE('',*,*,#6373,.F.);
#8948=ORIENTED_EDGE('',*,*,#6146,.T.);
#8949=ORIENTED_EDGE('',*,*,#5337,.T.);
#8950=ORIENTED_EDGE('',*,*,#5975,.T.);
#8951=ORIENTED_EDGE('',*,*,#5808,.F.);
#8952=ORIENTED_EDGE('',*,*,#6374,.F.);
#8953=ORIENTED_EDGE('',*,*,#6157,.T.);
#8954=ORIENTED_EDGE('',*,*,#6156,.T.);
#8955=ORIENTED_EDGE('',*,*,#6375,.T.);
#8956=ORIENTED_EDGE('',*,*,#5811,.F.);
#8957=ORIENTED_EDGE('',*,*,#5974,.T.);
#8958=ORIENTED_EDGE('',*,*,#5335,.T.);
#8959=ORIENTED_EDGE('',*,*,#6155,.T.);
#8960=ORIENTED_EDGE('',*,*,#6374,.T.);
#8961=ORIENTED_EDGE('',*,*,#5810,.F.);
#8962=ORIENTED_EDGE('',*,*,#6375,.F.);
#8963=ORIENTED_EDGE('',*,*,#6152,.T.);
#8964=ORIENTED_EDGE('',*,*,#5343,.T.);
#8965=ORIENTED_EDGE('',*,*,#5973,.T.);
#8966=ORIENTED_EDGE('',*,*,#5812,.F.);
#8967=ORIENTED_EDGE('',*,*,#6376,.F.);
#8968=ORIENTED_EDGE('',*,*,#6163,.T.);
#8969=ORIENTED_EDGE('',*,*,#6162,.T.);
#8970=ORIENTED_EDGE('',*,*,#6377,.T.);
#8971=ORIENTED_EDGE('',*,*,#5818,.F.);
#8972=ORIENTED_EDGE('',*,*,#5815,.F.);
#8973=ORIENTED_EDGE('',*,*,#5972,.T.);
#8974=ORIENTED_EDGE('',*,*,#5341,.T.);
#8975=ORIENTED_EDGE('',*,*,#6161,.T.);
#8976=ORIENTED_EDGE('',*,*,#6376,.T.);
#8977=ORIENTED_EDGE('',*,*,#5814,.F.);
#8978=ORIENTED_EDGE('',*,*,#6377,.F.);
#8979=ORIENTED_EDGE('',*,*,#6158,.T.);
#8980=ORIENTED_EDGE('',*,*,#5349,.T.);
#8981=ORIENTED_EDGE('',*,*,#5971,.T.);
#8982=ORIENTED_EDGE('',*,*,#5819,.F.);
#8983=ORIENTED_EDGE('',*,*,#6378,.F.);
#8984=ORIENTED_EDGE('',*,*,#6169,.T.);
#8985=ORIENTED_EDGE('',*,*,#6168,.T.);
#8986=ORIENTED_EDGE('',*,*,#6379,.T.);
#8987=ORIENTED_EDGE('',*,*,#5822,.F.);
#8988=ORIENTED_EDGE('',*,*,#5970,.T.);
#8989=ORIENTED_EDGE('',*,*,#5347,.T.);
#8990=ORIENTED_EDGE('',*,*,#6167,.T.);
#8991=ORIENTED_EDGE('',*,*,#6378,.T.);
#8992=ORIENTED_EDGE('',*,*,#5821,.F.);
#8993=ORIENTED_EDGE('',*,*,#6379,.F.);
#8994=ORIENTED_EDGE('',*,*,#6164,.T.);
#8995=ORIENTED_EDGE('',*,*,#5355,.T.);
#8996=ORIENTED_EDGE('',*,*,#5969,.T.);
#8997=ORIENTED_EDGE('',*,*,#5823,.F.);
#8998=ORIENTED_EDGE('',*,*,#6380,.F.);
#8999=ORIENTED_EDGE('',*,*,#6175,.T.);
#9000=ORIENTED_EDGE('',*,*,#6174,.T.);
#9001=ORIENTED_EDGE('',*,*,#6381,.T.);
#9002=ORIENTED_EDGE('',*,*,#5826,.F.);
#9003=ORIENTED_EDGE('',*,*,#5968,.T.);
#9004=ORIENTED_EDGE('',*,*,#5353,.T.);
#9005=ORIENTED_EDGE('',*,*,#6173,.T.);
#9006=ORIENTED_EDGE('',*,*,#6380,.T.);
#9007=ORIENTED_EDGE('',*,*,#5825,.F.);
#9008=ORIENTED_EDGE('',*,*,#6381,.F.);
#9009=ORIENTED_EDGE('',*,*,#6170,.T.);
#9010=ORIENTED_EDGE('',*,*,#5361,.T.);
#9011=ORIENTED_EDGE('',*,*,#5967,.T.);
#9012=ORIENTED_EDGE('',*,*,#5827,.F.);
#9013=ORIENTED_EDGE('',*,*,#6382,.F.);
#9014=ORIENTED_EDGE('',*,*,#6181,.T.);
#9015=ORIENTED_EDGE('',*,*,#6180,.T.);
#9016=ORIENTED_EDGE('',*,*,#6383,.T.);
#9017=ORIENTED_EDGE('',*,*,#5830,.F.);
#9018=ORIENTED_EDGE('',*,*,#5966,.T.);
#9019=ORIENTED_EDGE('',*,*,#5359,.T.);
#9020=ORIENTED_EDGE('',*,*,#6179,.T.);
#9021=ORIENTED_EDGE('',*,*,#6382,.T.);
#9022=ORIENTED_EDGE('',*,*,#5829,.F.);
#9023=ORIENTED_EDGE('',*,*,#6383,.F.);
#9024=ORIENTED_EDGE('',*,*,#6176,.T.);
#9025=ORIENTED_EDGE('',*,*,#5367,.T.);
#9026=ORIENTED_EDGE('',*,*,#5965,.T.);
#9027=ORIENTED_EDGE('',*,*,#5831,.F.);
#9028=ORIENTED_EDGE('',*,*,#6384,.F.);
#9029=ORIENTED_EDGE('',*,*,#6184,.T.);
#9030=ORIENTED_EDGE('',*,*,#5373,.T.);
#9031=ORIENTED_EDGE('',*,*,#5963,.T.);
#9032=ORIENTED_EDGE('',*,*,#5835,.F.);
#9033=ORIENTED_EDGE('',*,*,#5964,.T.);
#9034=ORIENTED_EDGE('',*,*,#5365,.T.);
#9035=ORIENTED_EDGE('',*,*,#6183,.T.);
#9036=ORIENTED_EDGE('',*,*,#6385,.T.);
#9037=ORIENTED_EDGE('',*,*,#5833,.F.);
#9038=ORIENTED_EDGE('',*,*,#6385,.F.);
#9039=ORIENTED_EDGE('',*,*,#6187,.T.);
#9040=ORIENTED_EDGE('',*,*,#6186,.T.);
#9041=ORIENTED_EDGE('',*,*,#6384,.T.);
#9042=ORIENTED_EDGE('',*,*,#5834,.F.);
#9043=ORIENTED_EDGE('',*,*,#6386,.F.);
#9044=ORIENTED_EDGE('',*,*,#6193,.T.);
#9045=ORIENTED_EDGE('',*,*,#6192,.T.);
#9046=ORIENTED_EDGE('',*,*,#6387,.T.);
#9047=ORIENTED_EDGE('',*,*,#5838,.F.);
#9048=ORIENTED_EDGE('',*,*,#5962,.T.);
#9049=ORIENTED_EDGE('',*,*,#5371,.T.);
#9050=ORIENTED_EDGE('',*,*,#6191,.T.);
#9051=ORIENTED_EDGE('',*,*,#6386,.T.);
#9052=ORIENTED_EDGE('',*,*,#5837,.F.);
#9053=ORIENTED_EDGE('',*,*,#6387,.F.);
#9054=ORIENTED_EDGE('',*,*,#6188,.T.);
#9055=ORIENTED_EDGE('',*,*,#5379,.T.);
#9056=ORIENTED_EDGE('',*,*,#5961,.T.);
#9057=ORIENTED_EDGE('',*,*,#5839,.F.);
#9058=ORIENTED_EDGE('',*,*,#6388,.F.);
#9059=ORIENTED_EDGE('',*,*,#6199,.T.);
#9060=ORIENTED_EDGE('',*,*,#6198,.T.);
#9061=ORIENTED_EDGE('',*,*,#6389,.T.);
#9062=ORIENTED_EDGE('',*,*,#5842,.F.);
#9063=ORIENTED_EDGE('',*,*,#5960,.T.);
#9064=ORIENTED_EDGE('',*,*,#5377,.T.);
#9065=ORIENTED_EDGE('',*,*,#6197,.T.);
#9066=ORIENTED_EDGE('',*,*,#6388,.T.);
#9067=ORIENTED_EDGE('',*,*,#5841,.F.);
#9068=ORIENTED_EDGE('',*,*,#6389,.F.);
#9069=ORIENTED_EDGE('',*,*,#6194,.T.);
#9070=ORIENTED_EDGE('',*,*,#5385,.T.);
#9071=ORIENTED_EDGE('',*,*,#5959,.T.);
#9072=ORIENTED_EDGE('',*,*,#5843,.F.);
#9073=ORIENTED_EDGE('',*,*,#6390,.F.);
#9074=ORIENTED_EDGE('',*,*,#6205,.T.);
#9075=ORIENTED_EDGE('',*,*,#6204,.T.);
#9076=ORIENTED_EDGE('',*,*,#6391,.T.);
#9077=ORIENTED_EDGE('',*,*,#5846,.F.);
#9078=ORIENTED_EDGE('',*,*,#5958,.T.);
#9079=ORIENTED_EDGE('',*,*,#5383,.T.);
#9080=ORIENTED_EDGE('',*,*,#6203,.T.);
#9081=ORIENTED_EDGE('',*,*,#6390,.T.);
#9082=ORIENTED_EDGE('',*,*,#5845,.F.);
#9083=ORIENTED_EDGE('',*,*,#6391,.F.);
#9084=ORIENTED_EDGE('',*,*,#6200,.T.);
#9085=ORIENTED_EDGE('',*,*,#5391,.T.);
#9086=ORIENTED_EDGE('',*,*,#5957,.T.);
#9087=ORIENTED_EDGE('',*,*,#5847,.F.);
#9088=ORIENTED_EDGE('',*,*,#6392,.F.);
#9089=ORIENTED_EDGE('',*,*,#6211,.T.);
#9090=ORIENTED_EDGE('',*,*,#6210,.T.);
#9091=ORIENTED_EDGE('',*,*,#6393,.T.);
#9092=ORIENTED_EDGE('',*,*,#5850,.F.);
#9093=ORIENTED_EDGE('',*,*,#5956,.T.);
#9094=ORIENTED_EDGE('',*,*,#5389,.T.);
#9095=ORIENTED_EDGE('',*,*,#6209,.T.);
#9096=ORIENTED_EDGE('',*,*,#6392,.T.);
#9097=ORIENTED_EDGE('',*,*,#5849,.F.);
#9098=ORIENTED_EDGE('',*,*,#6393,.F.);
#9099=ORIENTED_EDGE('',*,*,#6206,.T.);
#9100=ORIENTED_EDGE('',*,*,#5397,.T.);
#9101=ORIENTED_EDGE('',*,*,#5955,.T.);
#9102=ORIENTED_EDGE('',*,*,#5851,.F.);
#9103=ORIENTED_EDGE('',*,*,#6394,.F.);
#9104=ORIENTED_EDGE('',*,*,#6217,.T.);
#9105=ORIENTED_EDGE('',*,*,#6216,.T.);
#9106=ORIENTED_EDGE('',*,*,#6395,.T.);
#9107=ORIENTED_EDGE('',*,*,#5854,.F.);
#9108=ORIENTED_EDGE('',*,*,#5954,.T.);
#9109=ORIENTED_EDGE('',*,*,#5395,.T.);
#9110=ORIENTED_EDGE('',*,*,#6215,.T.);
#9111=ORIENTED_EDGE('',*,*,#6394,.T.);
#9112=ORIENTED_EDGE('',*,*,#5853,.F.);
#9113=ORIENTED_EDGE('',*,*,#6395,.F.);
#9114=ORIENTED_EDGE('',*,*,#6212,.T.);
#9115=ORIENTED_EDGE('',*,*,#5403,.T.);
#9116=ORIENTED_EDGE('',*,*,#5953,.T.);
#9117=ORIENTED_EDGE('',*,*,#5855,.F.);
#9118=ORIENTED_EDGE('',*,*,#6396,.F.);
#9119=ORIENTED_EDGE('',*,*,#6223,.T.);
#9120=ORIENTED_EDGE('',*,*,#6222,.T.);
#9121=ORIENTED_EDGE('',*,*,#6397,.T.);
#9122=ORIENTED_EDGE('',*,*,#5858,.F.);
#9123=ORIENTED_EDGE('',*,*,#5952,.T.);
#9124=ORIENTED_EDGE('',*,*,#5401,.T.);
#9125=ORIENTED_EDGE('',*,*,#6221,.T.);
#9126=ORIENTED_EDGE('',*,*,#6396,.T.);
#9127=ORIENTED_EDGE('',*,*,#5857,.F.);
#9128=ORIENTED_EDGE('',*,*,#6397,.F.);
#9129=ORIENTED_EDGE('',*,*,#6218,.T.);
#9130=ORIENTED_EDGE('',*,*,#5409,.T.);
#9131=ORIENTED_EDGE('',*,*,#5951,.T.);
#9132=ORIENTED_EDGE('',*,*,#5859,.F.);
#9133=ORIENTED_EDGE('',*,*,#6398,.F.);
#9134=ORIENTED_EDGE('',*,*,#6229,.T.);
#9135=ORIENTED_EDGE('',*,*,#6228,.T.);
#9136=ORIENTED_EDGE('',*,*,#6399,.T.);
#9137=ORIENTED_EDGE('',*,*,#5862,.F.);
#9138=ORIENTED_EDGE('',*,*,#5950,.T.);
#9139=ORIENTED_EDGE('',*,*,#5407,.T.);
#9140=ORIENTED_EDGE('',*,*,#6227,.T.);
#9141=ORIENTED_EDGE('',*,*,#6398,.T.);
#9142=ORIENTED_EDGE('',*,*,#5861,.F.);
#9143=ORIENTED_EDGE('',*,*,#6399,.F.);
#9144=ORIENTED_EDGE('',*,*,#6224,.T.);
#9145=ORIENTED_EDGE('',*,*,#5415,.T.);
#9146=ORIENTED_EDGE('',*,*,#5949,.T.);
#9147=ORIENTED_EDGE('',*,*,#5863,.F.);
#9148=ORIENTED_EDGE('',*,*,#6400,.F.);
#9149=ORIENTED_EDGE('',*,*,#6235,.T.);
#9150=ORIENTED_EDGE('',*,*,#6234,.T.);
#9151=ORIENTED_EDGE('',*,*,#6401,.T.);
#9152=ORIENTED_EDGE('',*,*,#5866,.F.);
#9153=ORIENTED_EDGE('',*,*,#5948,.T.);
#9154=ORIENTED_EDGE('',*,*,#5413,.T.);
#9155=ORIENTED_EDGE('',*,*,#6233,.T.);
#9156=ORIENTED_EDGE('',*,*,#6400,.T.);
#9157=ORIENTED_EDGE('',*,*,#5865,.F.);
#9158=ORIENTED_EDGE('',*,*,#6401,.F.);
#9159=ORIENTED_EDGE('',*,*,#6230,.T.);
#9160=ORIENTED_EDGE('',*,*,#5421,.T.);
#9161=ORIENTED_EDGE('',*,*,#5947,.T.);
#9162=ORIENTED_EDGE('',*,*,#5867,.F.);
#9163=ORIENTED_EDGE('',*,*,#6402,.F.);
#9164=ORIENTED_EDGE('',*,*,#6241,.T.);
#9165=ORIENTED_EDGE('',*,*,#6240,.T.);
#9166=ORIENTED_EDGE('',*,*,#6403,.T.);
#9167=ORIENTED_EDGE('',*,*,#5870,.F.);
#9168=ORIENTED_EDGE('',*,*,#5946,.T.);
#9169=ORIENTED_EDGE('',*,*,#5419,.T.);
#9170=ORIENTED_EDGE('',*,*,#6239,.T.);
#9171=ORIENTED_EDGE('',*,*,#6402,.T.);
#9172=ORIENTED_EDGE('',*,*,#5869,.F.);
#9173=ORIENTED_EDGE('',*,*,#6403,.F.);
#9174=ORIENTED_EDGE('',*,*,#6236,.T.);
#9175=ORIENTED_EDGE('',*,*,#5427,.T.);
#9176=ORIENTED_EDGE('',*,*,#5945,.T.);
#9177=ORIENTED_EDGE('',*,*,#5871,.F.);
#9178=ORIENTED_EDGE('',*,*,#6404,.F.);
#9179=ORIENTED_EDGE('',*,*,#6247,.T.);
#9180=ORIENTED_EDGE('',*,*,#6246,.T.);
#9181=ORIENTED_EDGE('',*,*,#6405,.T.);
#9182=ORIENTED_EDGE('',*,*,#5874,.F.);
#9183=ORIENTED_EDGE('',*,*,#5944,.T.);
#9184=ORIENTED_EDGE('',*,*,#5425,.T.);
#9185=ORIENTED_EDGE('',*,*,#6245,.T.);
#9186=ORIENTED_EDGE('',*,*,#6404,.T.);
#9187=ORIENTED_EDGE('',*,*,#5873,.F.);
#9188=ORIENTED_EDGE('',*,*,#6405,.F.);
#9189=ORIENTED_EDGE('',*,*,#6242,.T.);
#9190=ORIENTED_EDGE('',*,*,#5433,.T.);
#9191=ORIENTED_EDGE('',*,*,#5943,.T.);
#9192=ORIENTED_EDGE('',*,*,#5875,.F.);
#9193=ORIENTED_EDGE('',*,*,#6406,.F.);
#9194=ORIENTED_EDGE('',*,*,#6253,.T.);
#9195=ORIENTED_EDGE('',*,*,#6252,.T.);
#9196=ORIENTED_EDGE('',*,*,#6407,.T.);
#9197=ORIENTED_EDGE('',*,*,#5878,.F.);
#9198=ORIENTED_EDGE('',*,*,#5942,.T.);
#9199=ORIENTED_EDGE('',*,*,#5431,.T.);
#9200=ORIENTED_EDGE('',*,*,#6251,.T.);
#9201=ORIENTED_EDGE('',*,*,#6406,.T.);
#9202=ORIENTED_EDGE('',*,*,#5877,.F.);
#9203=ORIENTED_EDGE('',*,*,#6407,.F.);
#9204=ORIENTED_EDGE('',*,*,#6248,.T.);
#9205=ORIENTED_EDGE('',*,*,#5439,.T.);
#9206=ORIENTED_EDGE('',*,*,#5941,.T.);
#9207=ORIENTED_EDGE('',*,*,#5879,.F.);
#9208=ORIENTED_EDGE('',*,*,#6408,.F.);
#9209=ORIENTED_EDGE('',*,*,#6259,.T.);
#9210=ORIENTED_EDGE('',*,*,#6258,.T.);
#9211=ORIENTED_EDGE('',*,*,#6409,.T.);
#9212=ORIENTED_EDGE('',*,*,#5882,.F.);
#9213=ORIENTED_EDGE('',*,*,#5940,.T.);
#9214=ORIENTED_EDGE('',*,*,#5437,.T.);
#9215=ORIENTED_EDGE('',*,*,#6257,.T.);
#9216=ORIENTED_EDGE('',*,*,#6408,.T.);
#9217=ORIENTED_EDGE('',*,*,#5881,.F.);
#9218=ORIENTED_EDGE('',*,*,#6409,.F.);
#9219=ORIENTED_EDGE('',*,*,#6254,.T.);
#9220=ORIENTED_EDGE('',*,*,#5445,.T.);
#9221=ORIENTED_EDGE('',*,*,#5939,.T.);
#9222=ORIENTED_EDGE('',*,*,#5883,.F.);
#9223=ORIENTED_EDGE('',*,*,#6410,.F.);
#9224=ORIENTED_EDGE('',*,*,#6265,.T.);
#9225=ORIENTED_EDGE('',*,*,#6264,.T.);
#9226=ORIENTED_EDGE('',*,*,#6411,.T.);
#9227=ORIENTED_EDGE('',*,*,#5886,.F.);
#9228=ORIENTED_EDGE('',*,*,#5938,.T.);
#9229=ORIENTED_EDGE('',*,*,#5443,.T.);
#9230=ORIENTED_EDGE('',*,*,#6263,.T.);
#9231=ORIENTED_EDGE('',*,*,#6410,.T.);
#9232=ORIENTED_EDGE('',*,*,#5885,.F.);
#9233=ORIENTED_EDGE('',*,*,#6411,.F.);
#9234=ORIENTED_EDGE('',*,*,#6260,.T.);
#9235=ORIENTED_EDGE('',*,*,#5451,.T.);
#9236=ORIENTED_EDGE('',*,*,#5937,.T.);
#9237=ORIENTED_EDGE('',*,*,#5887,.F.);
#9238=ORIENTED_EDGE('',*,*,#6412,.F.);
#9239=ORIENTED_EDGE('',*,*,#6271,.T.);
#9240=ORIENTED_EDGE('',*,*,#6270,.T.);
#9241=ORIENTED_EDGE('',*,*,#6413,.T.);
#9242=ORIENTED_EDGE('',*,*,#5890,.F.);
#9243=ORIENTED_EDGE('',*,*,#5936,.T.);
#9244=ORIENTED_EDGE('',*,*,#5449,.T.);
#9245=ORIENTED_EDGE('',*,*,#6269,.T.);
#9246=ORIENTED_EDGE('',*,*,#6412,.T.);
#9247=ORIENTED_EDGE('',*,*,#5889,.F.);
#9248=ORIENTED_EDGE('',*,*,#6413,.F.);
#9249=ORIENTED_EDGE('',*,*,#6266,.T.);
#9250=ORIENTED_EDGE('',*,*,#5457,.T.);
#9251=ORIENTED_EDGE('',*,*,#5935,.T.);
#9252=ORIENTED_EDGE('',*,*,#5891,.F.);
#9253=ORIENTED_EDGE('',*,*,#6414,.F.);
#9254=ORIENTED_EDGE('',*,*,#6277,.T.);
#9255=ORIENTED_EDGE('',*,*,#6276,.T.);
#9256=ORIENTED_EDGE('',*,*,#6415,.T.);
#9257=ORIENTED_EDGE('',*,*,#5894,.F.);
#9258=ORIENTED_EDGE('',*,*,#5934,.T.);
#9259=ORIENTED_EDGE('',*,*,#5455,.T.);
#9260=ORIENTED_EDGE('',*,*,#6275,.T.);
#9261=ORIENTED_EDGE('',*,*,#6414,.T.);
#9262=ORIENTED_EDGE('',*,*,#5893,.F.);
#9263=ORIENTED_EDGE('',*,*,#6415,.F.);
#9264=ORIENTED_EDGE('',*,*,#6272,.T.);
#9265=ORIENTED_EDGE('',*,*,#5463,.T.);
#9266=ORIENTED_EDGE('',*,*,#5933,.T.);
#9267=ORIENTED_EDGE('',*,*,#5895,.F.);
#9268=ORIENTED_EDGE('',*,*,#6416,.F.);
#9269=ORIENTED_EDGE('',*,*,#6283,.T.);
#9270=ORIENTED_EDGE('',*,*,#6282,.T.);
#9271=ORIENTED_EDGE('',*,*,#6417,.T.);
#9272=ORIENTED_EDGE('',*,*,#5898,.F.);
#9273=ORIENTED_EDGE('',*,*,#5932,.T.);
#9274=ORIENTED_EDGE('',*,*,#5461,.T.);
#9275=ORIENTED_EDGE('',*,*,#6281,.T.);
#9276=ORIENTED_EDGE('',*,*,#6416,.T.);
#9277=ORIENTED_EDGE('',*,*,#5897,.F.);
#9278=ORIENTED_EDGE('',*,*,#6417,.F.);
#9279=ORIENTED_EDGE('',*,*,#6278,.T.);
#9280=ORIENTED_EDGE('',*,*,#5469,.T.);
#9281=ORIENTED_EDGE('',*,*,#5931,.T.);
#9282=ORIENTED_EDGE('',*,*,#5899,.F.);
#9283=ORIENTED_EDGE('',*,*,#6418,.F.);
#9284=ORIENTED_EDGE('',*,*,#6289,.T.);
#9285=ORIENTED_EDGE('',*,*,#6288,.T.);
#9286=ORIENTED_EDGE('',*,*,#6419,.T.);
#9287=ORIENTED_EDGE('',*,*,#5902,.F.);
#9288=ORIENTED_EDGE('',*,*,#5930,.T.);
#9289=ORIENTED_EDGE('',*,*,#5467,.T.);
#9290=ORIENTED_EDGE('',*,*,#6287,.T.);
#9291=ORIENTED_EDGE('',*,*,#6418,.T.);
#9292=ORIENTED_EDGE('',*,*,#5901,.F.);
#9293=ORIENTED_EDGE('',*,*,#6419,.F.);
#9294=ORIENTED_EDGE('',*,*,#6284,.T.);
#9295=ORIENTED_EDGE('',*,*,#5475,.T.);
#9296=ORIENTED_EDGE('',*,*,#5929,.T.);
#9297=ORIENTED_EDGE('',*,*,#5903,.F.);
#9298=ORIENTED_EDGE('',*,*,#6420,.F.);
#9299=ORIENTED_EDGE('',*,*,#6295,.T.);
#9300=ORIENTED_EDGE('',*,*,#6294,.T.);
#9301=ORIENTED_EDGE('',*,*,#6421,.T.);
#9302=ORIENTED_EDGE('',*,*,#5727,.F.);
#9303=ORIENTED_EDGE('',*,*,#5928,.T.);
#9304=ORIENTED_EDGE('',*,*,#5473,.T.);
#9305=ORIENTED_EDGE('',*,*,#6293,.T.);
#9306=ORIENTED_EDGE('',*,*,#6420,.T.);
#9307=ORIENTED_EDGE('',*,*,#5905,.F.);
#9308=ORIENTED_EDGE('',*,*,#6421,.F.);
#9309=ORIENTED_EDGE('',*,*,#6290,.T.);
#9310=ORIENTED_EDGE('',*,*,#5481,.T.);
#9311=ORIENTED_EDGE('',*,*,#5927,.T.);
#9312=ORIENTED_EDGE('',*,*,#5728,.F.);
#9313=ORIENTED_EDGE('',*,*,#6422,.F.);
#9314=ORIENTED_EDGE('',*,*,#6301,.T.);
#9315=ORIENTED_EDGE('',*,*,#6300,.T.);
#9316=ORIENTED_EDGE('',*,*,#6423,.T.);
#9317=ORIENTED_EDGE('',*,*,#5731,.F.);
#9318=ORIENTED_EDGE('',*,*,#5926,.T.);
#9319=ORIENTED_EDGE('',*,*,#5479,.T.);
#9320=ORIENTED_EDGE('',*,*,#6299,.T.);
#9321=ORIENTED_EDGE('',*,*,#6422,.T.);
#9322=ORIENTED_EDGE('',*,*,#5730,.F.);
#9323=ORIENTED_EDGE('',*,*,#6423,.F.);
#9324=ORIENTED_EDGE('',*,*,#6296,.T.);
#9325=ORIENTED_EDGE('',*,*,#5487,.T.);
#9326=ORIENTED_EDGE('',*,*,#5925,.T.);
#9327=ORIENTED_EDGE('',*,*,#5732,.F.);
#9328=ORIENTED_EDGE('',*,*,#6424,.F.);
#9329=ORIENTED_EDGE('',*,*,#6307,.T.);
#9330=ORIENTED_EDGE('',*,*,#6306,.T.);
#9331=ORIENTED_EDGE('',*,*,#6425,.T.);
#9332=ORIENTED_EDGE('',*,*,#5735,.F.);
#9333=ORIENTED_EDGE('',*,*,#5924,.T.);
#9334=ORIENTED_EDGE('',*,*,#5485,.T.);
#9335=ORIENTED_EDGE('',*,*,#6305,.T.);
#9336=ORIENTED_EDGE('',*,*,#6424,.T.);
#9337=ORIENTED_EDGE('',*,*,#5734,.F.);
#9338=ORIENTED_EDGE('',*,*,#6425,.F.);
#9339=ORIENTED_EDGE('',*,*,#6302,.T.);
#9340=ORIENTED_EDGE('',*,*,#5493,.T.);
#9341=ORIENTED_EDGE('',*,*,#5923,.T.);
#9342=ORIENTED_EDGE('',*,*,#5736,.F.);
#9343=ORIENTED_EDGE('',*,*,#6426,.F.);
#9344=ORIENTED_EDGE('',*,*,#6313,.T.);
#9345=ORIENTED_EDGE('',*,*,#6312,.T.);
#9346=ORIENTED_EDGE('',*,*,#6427,.T.);
#9347=ORIENTED_EDGE('',*,*,#5739,.F.);
#9348=ORIENTED_EDGE('',*,*,#5922,.T.);
#9349=ORIENTED_EDGE('',*,*,#5491,.T.);
#9350=ORIENTED_EDGE('',*,*,#6311,.T.);
#9351=ORIENTED_EDGE('',*,*,#6426,.T.);
#9352=ORIENTED_EDGE('',*,*,#5738,.F.);
#9353=ORIENTED_EDGE('',*,*,#6427,.F.);
#9354=ORIENTED_EDGE('',*,*,#6308,.T.);
#9355=ORIENTED_EDGE('',*,*,#5499,.T.);
#9356=ORIENTED_EDGE('',*,*,#5921,.T.);
#9357=ORIENTED_EDGE('',*,*,#5740,.F.);
#9358=ORIENTED_EDGE('',*,*,#6428,.F.);
#9359=ORIENTED_EDGE('',*,*,#6316,.T.);
#9360=ORIENTED_EDGE('',*,*,#5505,.T.);
#9361=ORIENTED_EDGE('',*,*,#5919,.T.);
#9362=ORIENTED_EDGE('',*,*,#5744,.F.);
#9363=ORIENTED_EDGE('',*,*,#5920,.T.);
#9364=ORIENTED_EDGE('',*,*,#5497,.T.);
#9365=ORIENTED_EDGE('',*,*,#6315,.T.);
#9366=ORIENTED_EDGE('',*,*,#6429,.T.);
#9367=ORIENTED_EDGE('',*,*,#5742,.F.);
#9368=ORIENTED_EDGE('',*,*,#6429,.F.);
#9369=ORIENTED_EDGE('',*,*,#6319,.T.);
#9370=ORIENTED_EDGE('',*,*,#6318,.T.);
#9371=ORIENTED_EDGE('',*,*,#6428,.T.);
#9372=ORIENTED_EDGE('',*,*,#5743,.F.);
#9373=ORIENTED_EDGE('',*,*,#6430,.F.);
#9374=ORIENTED_EDGE('',*,*,#6325,.T.);
#9375=ORIENTED_EDGE('',*,*,#6324,.T.);
#9376=ORIENTED_EDGE('',*,*,#6431,.T.);
#9377=ORIENTED_EDGE('',*,*,#5747,.F.);
#9378=ORIENTED_EDGE('',*,*,#5918,.T.);
#9379=ORIENTED_EDGE('',*,*,#5503,.T.);
#9380=ORIENTED_EDGE('',*,*,#6323,.T.);
#9381=ORIENTED_EDGE('',*,*,#6430,.T.);
#9382=ORIENTED_EDGE('',*,*,#5746,.F.);
#9383=ORIENTED_EDGE('',*,*,#6431,.F.);
#9384=ORIENTED_EDGE('',*,*,#6320,.T.);
#9385=ORIENTED_EDGE('',*,*,#5511,.T.);
#9386=ORIENTED_EDGE('',*,*,#5917,.T.);
#9387=ORIENTED_EDGE('',*,*,#5748,.F.);
#9388=ORIENTED_EDGE('',*,*,#6432,.F.);
#9389=ORIENTED_EDGE('',*,*,#6331,.T.);
#9390=ORIENTED_EDGE('',*,*,#6330,.T.);
#9391=ORIENTED_EDGE('',*,*,#6433,.T.);
#9392=ORIENTED_EDGE('',*,*,#5751,.F.);
#9393=ORIENTED_EDGE('',*,*,#5916,.T.);
#9394=ORIENTED_EDGE('',*,*,#5509,.T.);
#9395=ORIENTED_EDGE('',*,*,#6329,.T.);
#9396=ORIENTED_EDGE('',*,*,#6432,.T.);
#9397=ORIENTED_EDGE('',*,*,#5750,.F.);
#9398=ORIENTED_EDGE('',*,*,#6433,.F.);
#9399=ORIENTED_EDGE('',*,*,#6326,.T.);
#9400=ORIENTED_EDGE('',*,*,#5517,.T.);
#9401=ORIENTED_EDGE('',*,*,#5915,.T.);
#9402=ORIENTED_EDGE('',*,*,#5752,.F.);
#9403=ORIENTED_EDGE('',*,*,#6434,.F.);
#9404=ORIENTED_EDGE('',*,*,#6337,.T.);
#9405=ORIENTED_EDGE('',*,*,#6336,.T.);
#9406=ORIENTED_EDGE('',*,*,#6435,.T.);
#9407=ORIENTED_EDGE('',*,*,#5755,.F.);
#9408=ORIENTED_EDGE('',*,*,#5914,.T.);
#9409=ORIENTED_EDGE('',*,*,#5515,.T.);
#9410=ORIENTED_EDGE('',*,*,#6335,.T.);
#9411=ORIENTED_EDGE('',*,*,#6434,.T.);
#9412=ORIENTED_EDGE('',*,*,#5754,.F.);
#9413=ORIENTED_EDGE('',*,*,#6435,.F.);
#9414=ORIENTED_EDGE('',*,*,#6332,.T.);
#9415=ORIENTED_EDGE('',*,*,#5523,.T.);
#9416=ORIENTED_EDGE('',*,*,#5913,.T.);
#9417=ORIENTED_EDGE('',*,*,#5756,.F.);
#9418=ORIENTED_EDGE('',*,*,#6436,.F.);
#9419=ORIENTED_EDGE('',*,*,#6343,.T.);
#9420=ORIENTED_EDGE('',*,*,#6342,.T.);
#9421=ORIENTED_EDGE('',*,*,#6437,.T.);
#9422=ORIENTED_EDGE('',*,*,#5759,.F.);
#9423=ORIENTED_EDGE('',*,*,#5912,.T.);
#9424=ORIENTED_EDGE('',*,*,#5521,.T.);
#9425=ORIENTED_EDGE('',*,*,#6341,.T.);
#9426=ORIENTED_EDGE('',*,*,#6436,.T.);
#9427=ORIENTED_EDGE('',*,*,#5758,.F.);
#9428=ORIENTED_EDGE('',*,*,#6437,.F.);
#9429=ORIENTED_EDGE('',*,*,#6338,.T.);
#9430=ORIENTED_EDGE('',*,*,#5529,.T.);
#9431=ORIENTED_EDGE('',*,*,#5911,.T.);
#9432=ORIENTED_EDGE('',*,*,#5760,.F.);
#9433=ORIENTED_EDGE('',*,*,#6438,.F.);
#9434=ORIENTED_EDGE('',*,*,#6349,.T.);
#9435=ORIENTED_EDGE('',*,*,#6348,.T.);
#9436=ORIENTED_EDGE('',*,*,#6439,.T.);
#9437=ORIENTED_EDGE('',*,*,#5763,.F.);
#9438=ORIENTED_EDGE('',*,*,#5910,.T.);
#9439=ORIENTED_EDGE('',*,*,#5527,.T.);
#9440=ORIENTED_EDGE('',*,*,#6347,.T.);
#9441=ORIENTED_EDGE('',*,*,#6438,.T.);
#9442=ORIENTED_EDGE('',*,*,#5762,.F.);
#9443=ORIENTED_EDGE('',*,*,#6439,.F.);
#9444=ORIENTED_EDGE('',*,*,#6344,.T.);
#9445=ORIENTED_EDGE('',*,*,#5541,.T.);
#9446=ORIENTED_EDGE('',*,*,#5907,.T.);
#9447=ORIENTED_EDGE('',*,*,#5764,.F.);
#9448=ORIENTED_EDGE('',*,*,#6440,.F.);
#9449=ORIENTED_EDGE('',*,*,#6355,.T.);
#9450=ORIENTED_EDGE('',*,*,#6354,.T.);
#9451=ORIENTED_EDGE('',*,*,#6441,.T.);
#9452=ORIENTED_EDGE('',*,*,#5767,.F.);
#9453=ORIENTED_EDGE('',*,*,#5906,.T.);
#9454=ORIENTED_EDGE('',*,*,#5539,.T.);
#9455=ORIENTED_EDGE('',*,*,#6353,.T.);
#9456=ORIENTED_EDGE('',*,*,#6440,.T.);
#9457=ORIENTED_EDGE('',*,*,#5766,.F.);
#9458=ORIENTED_EDGE('',*,*,#6441,.F.);
#9459=ORIENTED_EDGE('',*,*,#6350,.T.);
#9460=ORIENTED_EDGE('',*,*,#5535,.T.);
#9461=ORIENTED_EDGE('',*,*,#5908,.T.);
#9462=ORIENTED_EDGE('',*,*,#5768,.F.);
#10065=CYLINDRICAL_SURFACE('',#11289,15.);
#10066=CYLINDRICAL_SURFACE('',#11338,43.5);
#10067=CYLINDRICAL_SURFACE('',#11339,43.5);
#10068=CYLINDRICAL_SURFACE('',#11340,43.5);
#10069=CYLINDRICAL_SURFACE('',#11341,43.5);
#10070=CYLINDRICAL_SURFACE('',#11342,43.5);
#10071=CYLINDRICAL_SURFACE('',#11343,43.5);
#10072=CYLINDRICAL_SURFACE('',#11344,43.5);
#10073=CYLINDRICAL_SURFACE('',#11345,43.5);
#10074=CYLINDRICAL_SURFACE('',#11346,43.5);
#10075=CYLINDRICAL_SURFACE('',#11347,43.5);
#10076=CYLINDRICAL_SURFACE('',#11348,43.5);
#10077=CYLINDRICAL_SURFACE('',#11349,43.5);
#10078=CYLINDRICAL_SURFACE('',#11350,43.5);
#10079=CYLINDRICAL_SURFACE('',#11351,43.5);
#10080=CYLINDRICAL_SURFACE('',#11352,43.5);
#10081=CYLINDRICAL_SURFACE('',#11353,43.5);
#10082=CYLINDRICAL_SURFACE('',#11354,43.5);
#10083=CYLINDRICAL_SURFACE('',#11355,43.5);
#10084=CYLINDRICAL_SURFACE('',#11356,43.5);
#10085=CYLINDRICAL_SURFACE('',#11357,43.5);
#10086=CYLINDRICAL_SURFACE('',#11358,43.5);
#10087=CYLINDRICAL_SURFACE('',#11359,43.5);
#10088=CYLINDRICAL_SURFACE('',#11360,43.5);
#10089=CYLINDRICAL_SURFACE('',#11361,43.5);
#10090=CYLINDRICAL_SURFACE('',#11362,43.5);
#10091=CYLINDRICAL_SURFACE('',#11363,43.5);
#10092=CYLINDRICAL_SURFACE('',#11364,43.5);
#10093=CYLINDRICAL_SURFACE('',#11365,43.5);
#10094=CYLINDRICAL_SURFACE('',#11366,43.5);
#10095=CYLINDRICAL_SURFACE('',#11367,43.5);
#10096=CYLINDRICAL_SURFACE('',#11368,43.5);
#10097=CYLINDRICAL_SURFACE('',#11369,43.5);
#10098=CYLINDRICAL_SURFACE('',#11370,43.5);
#10099=CYLINDRICAL_SURFACE('',#11371,43.5);
#10100=CYLINDRICAL_SURFACE('',#11372,43.5);
#10101=CYLINDRICAL_SURFACE('',#11373,43.5);
#10102=CYLINDRICAL_SURFACE('',#11374,43.5);
#10103=CYLINDRICAL_SURFACE('',#11375,43.5);
#10104=CYLINDRICAL_SURFACE('',#11376,43.5);
#10105=CYLINDRICAL_SURFACE('',#11377,43.5);
#10106=CYLINDRICAL_SURFACE('',#11378,43.5);
#10107=CYLINDRICAL_SURFACE('',#11379,43.5);
#10108=CYLINDRICAL_SURFACE('',#11380,43.5);
#10109=CYLINDRICAL_SURFACE('',#11381,43.5);
#10110=CYLINDRICAL_SURFACE('',#11382,43.5);
#10111=CYLINDRICAL_SURFACE('',#11383,43.5);
#10112=CYLINDRICAL_SURFACE('',#11384,43.5);
#10113=CYLINDRICAL_SURFACE('',#11385,43.5);
#10114=CYLINDRICAL_SURFACE('',#11386,43.5);
#10115=CYLINDRICAL_SURFACE('',#11387,43.5);
#10116=CYLINDRICAL_SURFACE('',#11388,43.5);
#10117=CYLINDRICAL_SURFACE('',#11389,43.5);
#10118=CYLINDRICAL_SURFACE('',#11390,43.5);
#10119=CYLINDRICAL_SURFACE('',#11391,43.5);
#10120=CYLINDRICAL_SURFACE('',#11392,43.5);
#10121=CYLINDRICAL_SURFACE('',#11393,43.5);
#10122=CYLINDRICAL_SURFACE('',#11394,43.5);
#10123=CYLINDRICAL_SURFACE('',#11395,43.5);
#10124=CYLINDRICAL_SURFACE('',#11396,43.5);
#10125=CYLINDRICAL_SURFACE('',#11397,43.5);
#10126=CYLINDRICAL_SURFACE('',#11398,43.5);
#10127=CYLINDRICAL_SURFACE('',#11399,43.5);
#10128=CYLINDRICAL_SURFACE('',#11400,43.5);
#10129=CYLINDRICAL_SURFACE('',#11401,43.5);
#10130=CYLINDRICAL_SURFACE('',#11402,43.5);
#10131=CYLINDRICAL_SURFACE('',#11403,43.5);
#10132=CYLINDRICAL_SURFACE('',#11404,43.5);
#10133=CYLINDRICAL_SURFACE('',#11405,43.5);
#10134=CYLINDRICAL_SURFACE('',#11406,43.5);
#10135=CYLINDRICAL_SURFACE('',#11407,43.5);
#10136=CYLINDRICAL_SURFACE('',#11408,43.5);
#10137=CYLINDRICAL_SURFACE('',#11409,43.5);
#10138=CYLINDRICAL_SURFACE('',#11410,43.5);
#10139=CYLINDRICAL_SURFACE('',#11411,43.5);
#10140=CYLINDRICAL_SURFACE('',#11412,43.5);
#10141=CYLINDRICAL_SURFACE('',#11413,43.5);
#10142=CYLINDRICAL_SURFACE('',#11414,43.5);
#10143=CYLINDRICAL_SURFACE('',#11415,43.5);
#10144=CYLINDRICAL_SURFACE('',#11416,43.5);
#10145=CYLINDRICAL_SURFACE('',#11417,43.5);
#10146=CYLINDRICAL_SURFACE('',#11418,43.5);
#10147=CYLINDRICAL_SURFACE('',#11419,43.5);
#10148=CYLINDRICAL_SURFACE('',#11420,43.5);
#10149=CYLINDRICAL_SURFACE('',#11421,43.5);
#10150=CYLINDRICAL_SURFACE('',#11422,43.5);
#10151=CYLINDRICAL_SURFACE('',#11423,43.5);
#10152=CYLINDRICAL_SURFACE('',#11424,43.5);
#10153=CYLINDRICAL_SURFACE('',#11425,43.5);
#10293=ADVANCED_FACE('',(#1648),#183,.F.);
#10294=ADVANCED_FACE('',(#1649),#184,.F.);
#10295=ADVANCED_FACE('',(#1650),#185,.F.);
#10296=ADVANCED_FACE('',(#1651),#186,.F.);
#10297=ADVANCED_FACE('',(#1652),#187,.F.);
#10298=ADVANCED_FACE('',(#1653),#188,.F.);
#10299=ADVANCED_FACE('',(#1654),#189,.F.);
#10300=ADVANCED_FACE('',(#1655),#190,.F.);
#10301=ADVANCED_FACE('',(#1656),#191,.F.);
#10302=ADVANCED_FACE('',(#1657),#192,.F.);
#10303=ADVANCED_FACE('',(#1658),#193,.F.);
#10304=ADVANCED_FACE('',(#1659),#194,.F.);
#10305=ADVANCED_FACE('',(#1660),#195,.F.);
#10306=ADVANCED_FACE('',(#1661),#196,.F.);
#10307=ADVANCED_FACE('',(#1662),#197,.F.);
#10308=ADVANCED_FACE('',(#1663),#198,.F.);
#10309=ADVANCED_FACE('',(#1664),#199,.F.);
#10310=ADVANCED_FACE('',(#1665),#200,.F.);
#10311=ADVANCED_FACE('',(#1666),#201,.F.);
#10312=ADVANCED_FACE('',(#1667),#202,.F.);
#10313=ADVANCED_FACE('',(#1668),#203,.F.);
#10314=ADVANCED_FACE('',(#1669),#204,.F.);
#10315=ADVANCED_FACE('',(#1670),#205,.F.);
#10316=ADVANCED_FACE('',(#1671),#206,.F.);
#10317=ADVANCED_FACE('',(#1672),#207,.F.);
#10318=ADVANCED_FACE('',(#1673),#208,.F.);
#10319=ADVANCED_FACE('',(#1674),#209,.F.);
#10320=ADVANCED_FACE('',(#1675),#210,.F.);
#10321=ADVANCED_FACE('',(#1676),#211,.F.);
#10322=ADVANCED_FACE('',(#1677),#212,.F.);
#10323=ADVANCED_FACE('',(#1678),#213,.F.);
#10324=ADVANCED_FACE('',(#1679),#214,.F.);
#10325=ADVANCED_FACE('',(#1680),#215,.F.);
#10326=ADVANCED_FACE('',(#1681),#216,.F.);
#10327=ADVANCED_FACE('',(#1682),#217,.F.);
#10328=ADVANCED_FACE('',(#1683),#218,.F.);
#10329=ADVANCED_FACE('',(#1684),#219,.F.);
#10330=ADVANCED_FACE('',(#1685),#220,.F.);
#10331=ADVANCED_FACE('',(#1686),#221,.F.);
#10332=ADVANCED_FACE('',(#1687),#222,.F.);
#10333=ADVANCED_FACE('',(#1688),#223,.F.);
#10334=ADVANCED_FACE('',(#1689),#224,.F.);
#10335=ADVANCED_FACE('',(#1690),#225,.F.);
#10336=ADVANCED_FACE('',(#1691),#226,.F.);
#10337=ADVANCED_FACE('',(#1692),#594,.T.);
#10338=ADVANCED_FACE('',(#1693),#10065,.F.);
#10339=ADVANCED_FACE('',(#1694),#595,.T.);
#10340=ADVANCED_FACE('',(#1695),#10066,.T.);
#10341=ADVANCED_FACE('',(#1696),#10067,.T.);
#10342=ADVANCED_FACE('',(#1697),#10068,.T.);
#10343=ADVANCED_FACE('',(#1698),#10069,.T.);
#10344=ADVANCED_FACE('',(#1699),#10070,.T.);
#10345=ADVANCED_FACE('',(#1700),#10071,.T.);
#10346=ADVANCED_FACE('',(#1701),#10072,.T.);
#10347=ADVANCED_FACE('',(#1702),#10073,.T.);
#10348=ADVANCED_FACE('',(#1703),#10074,.T.);
#10349=ADVANCED_FACE('',(#1704),#10075,.T.);
#10350=ADVANCED_FACE('',(#1705),#10076,.T.);
#10351=ADVANCED_FACE('',(#1706),#10077,.T.);
#10352=ADVANCED_FACE('',(#1707),#10078,.T.);
#10353=ADVANCED_FACE('',(#1708),#10079,.T.);
#10354=ADVANCED_FACE('',(#1709),#10080,.T.);
#10355=ADVANCED_FACE('',(#1710),#10081,.T.);
#10356=ADVANCED_FACE('',(#1711),#10082,.T.);
#10357=ADVANCED_FACE('',(#1712),#10083,.T.);
#10358=ADVANCED_FACE('',(#1713),#10084,.T.);
#10359=ADVANCED_FACE('',(#1714),#10085,.T.);
#10360=ADVANCED_FACE('',(#1715),#10086,.T.);
#10361=ADVANCED_FACE('',(#1716),#10087,.T.);
#10362=ADVANCED_FACE('',(#1717),#10088,.T.);
#10363=ADVANCED_FACE('',(#1718),#10089,.T.);
#10364=ADVANCED_FACE('',(#1719),#10090,.T.);
#10365=ADVANCED_FACE('',(#1720),#10091,.T.);
#10366=ADVANCED_FACE('',(#1721),#10092,.T.);
#10367=ADVANCED_FACE('',(#1722),#10093,.T.);
#10368=ADVANCED_FACE('',(#1723),#10094,.T.);
#10369=ADVANCED_FACE('',(#1724),#10095,.T.);
#10370=ADVANCED_FACE('',(#1725),#10096,.T.);
#10371=ADVANCED_FACE('',(#1726),#10097,.T.);
#10372=ADVANCED_FACE('',(#1727),#10098,.T.);
#10373=ADVANCED_FACE('',(#1728),#10099,.T.);
#10374=ADVANCED_FACE('',(#1729),#10100,.T.);
#10375=ADVANCED_FACE('',(#1730),#10101,.T.);
#10376=ADVANCED_FACE('',(#1731),#10102,.T.);
#10377=ADVANCED_FACE('',(#1732),#10103,.T.);
#10378=ADVANCED_FACE('',(#1733),#10104,.T.);
#10379=ADVANCED_FACE('',(#1734),#10105,.T.);
#10380=ADVANCED_FACE('',(#1735),#10106,.T.);
#10381=ADVANCED_FACE('',(#1736),#10107,.T.);
#10382=ADVANCED_FACE('',(#1737),#10108,.T.);
#10383=ADVANCED_FACE('',(#1738),#10109,.T.);
#10384=ADVANCED_FACE('',(#1739),#10110,.T.);
#10385=ADVANCED_FACE('',(#1740),#10111,.T.);
#10386=ADVANCED_FACE('',(#1741),#10112,.T.);
#10387=ADVANCED_FACE('',(#1742),#10113,.T.);
#10388=ADVANCED_FACE('',(#1743),#10114,.T.);
#10389=ADVANCED_FACE('',(#1744),#10115,.T.);
#10390=ADVANCED_FACE('',(#1745),#10116,.T.);
#10391=ADVANCED_FACE('',(#1746),#10117,.T.);
#10392=ADVANCED_FACE('',(#1747),#10118,.T.);
#10393=ADVANCED_FACE('',(#1748),#10119,.T.);
#10394=ADVANCED_FACE('',(#1749),#10120,.T.);
#10395=ADVANCED_FACE('',(#1750),#10121,.T.);
#10396=ADVANCED_FACE('',(#1751),#10122,.T.);
#10397=ADVANCED_FACE('',(#1752),#10123,.T.);
#10398=ADVANCED_FACE('',(#1753),#10124,.T.);
#10399=ADVANCED_FACE('',(#1754),#10125,.T.);
#10400=ADVANCED_FACE('',(#1755),#10126,.T.);
#10401=ADVANCED_FACE('',(#1756),#10127,.T.);
#10402=ADVANCED_FACE('',(#1757),#10128,.T.);
#10403=ADVANCED_FACE('',(#1758),#10129,.T.);
#10404=ADVANCED_FACE('',(#1759),#10130,.T.);
#10405=ADVANCED_FACE('',(#1760),#10131,.T.);
#10406=ADVANCED_FACE('',(#1761),#10132,.T.);
#10407=ADVANCED_FACE('',(#1762),#10133,.T.);
#10408=ADVANCED_FACE('',(#1763),#10134,.T.);
#10409=ADVANCED_FACE('',(#1764),#10135,.T.);
#10410=ADVANCED_FACE('',(#1765),#10136,.T.);
#10411=ADVANCED_FACE('',(#1766),#10137,.T.);
#10412=ADVANCED_FACE('',(#1767),#10138,.T.);
#10413=ADVANCED_FACE('',(#1768),#10139,.T.);
#10414=ADVANCED_FACE('',(#1769),#10140,.T.);
#10415=ADVANCED_FACE('',(#1770),#10141,.T.);
#10416=ADVANCED_FACE('',(#1771),#10142,.T.);
#10417=ADVANCED_FACE('',(#1772),#10143,.T.);
#10418=ADVANCED_FACE('',(#1773),#10144,.T.);
#10419=ADVANCED_FACE('',(#1774),#10145,.T.);
#10420=ADVANCED_FACE('',(#1775),#10146,.T.);
#10421=ADVANCED_FACE('',(#1776),#10147,.T.);
#10422=ADVANCED_FACE('',(#1777),#10148,.T.);
#10423=ADVANCED_FACE('',(#1778),#10149,.T.);
#10424=ADVANCED_FACE('',(#1779),#10150,.T.);
#10425=ADVANCED_FACE('',(#1780),#10151,.T.);
#10426=ADVANCED_FACE('',(#1781),#10152,.T.);
#10427=ADVANCED_FACE('',(#1782),#10153,.T.);
#10428=ADVANCED_FACE('',(#1783,#1405),#1504,.T.);
#10429=ADVANCED_FACE('',(#1784,#1406),#1505,.F.);
#10430=ADVANCED_FACE('',(#1785),#1506,.T.);
#10431=ADVANCED_FACE('',(#1786),#1507,.F.);
#10432=ADVANCED_FACE('',(#1787),#1508,.F.);
#10433=ADVANCED_FACE('',(#1788),#328,.F.);
#10434=ADVANCED_FACE('',(#1789),#329,.F.);
#10435=ADVANCED_FACE('',(#1790),#330,.F.);
#10436=ADVANCED_FACE('',(#1791),#331,.T.);
#10437=ADVANCED_FACE('',(#1792),#332,.T.);
#10438=ADVANCED_FACE('',(#1793),#333,.T.);
#10439=ADVANCED_FACE('',(#1794),#334,.F.);
#10440=ADVANCED_FACE('',(#1795),#335,.F.);
#10441=ADVANCED_FACE('',(#1796),#336,.F.);
#10442=ADVANCED_FACE('',(#1797),#337,.F.);
#10443=ADVANCED_FACE('',(#1798),#338,.F.);
#10444=ADVANCED_FACE('',(#1799),#339,.F.);
#10445=ADVANCED_FACE('',(#1800),#340,.F.);
#10446=ADVANCED_FACE('',(#1801),#341,.F.);
#10447=ADVANCED_FACE('',(#1802),#342,.F.);
#10448=ADVANCED_FACE('',(#1803),#343,.F.);
#10449=ADVANCED_FACE('',(#1804),#344,.F.);
#10450=ADVANCED_FACE('',(#1805),#345,.F.);
#10451=ADVANCED_FACE('',(#1806),#346,.F.);
#10452=ADVANCED_FACE('',(#1807),#347,.F.);
#10453=ADVANCED_FACE('',(#1808),#348,.F.);
#10454=ADVANCED_FACE('',(#1809),#349,.F.);
#10455=ADVANCED_FACE('',(#1810),#350,.F.);
#10456=ADVANCED_FACE('',(#1811),#351,.F.);
#10457=ADVANCED_FACE('',(#1812),#352,.F.);
#10458=ADVANCED_FACE('',(#1813),#353,.F.);
#10459=ADVANCED_FACE('',(#1814),#354,.F.);
#10460=ADVANCED_FACE('',(#1815),#355,.F.);
#10461=ADVANCED_FACE('',(#1816),#356,.F.);
#10462=ADVANCED_FACE('',(#1817),#357,.F.);
#10463=ADVANCED_FACE('',(#1818),#358,.F.);
#10464=ADVANCED_FACE('',(#1819),#359,.F.);
#10465=ADVANCED_FACE('',(#1820),#360,.F.);
#10466=ADVANCED_FACE('',(#1821),#361,.F.);
#10467=ADVANCED_FACE('',(#1822),#362,.F.);
#10468=ADVANCED_FACE('',(#1823),#363,.F.);
#10469=ADVANCED_FACE('',(#1824),#364,.F.);
#10470=ADVANCED_FACE('',(#1825),#365,.F.);
#10471=ADVANCED_FACE('',(#1826),#366,.F.);
#10472=ADVANCED_FACE('',(#1827),#367,.F.);
#10473=ADVANCED_FACE('',(#1828),#368,.F.);
#10474=ADVANCED_FACE('',(#1829),#369,.F.);
#10475=ADVANCED_FACE('',(#1830),#370,.F.);
#10476=ADVANCED_FACE('',(#1831),#371,.F.);
#10477=ADVANCED_FACE('',(#1832),#372,.F.);
#10478=ADVANCED_FACE('',(#1833),#373,.F.);
#10479=ADVANCED_FACE('',(#1834),#374,.F.);
#10480=ADVANCED_FACE('',(#1835),#375,.F.);
#10481=ADVANCED_FACE('',(#1836),#376,.F.);
#10482=ADVANCED_FACE('',(#1837),#377,.F.);
#10483=ADVANCED_FACE('',(#1838),#378,.F.);
#10484=ADVANCED_FACE('',(#1839),#379,.F.);
#10485=ADVANCED_FACE('',(#1840),#380,.F.);
#10486=ADVANCED_FACE('',(#1841),#381,.F.);
#10487=ADVANCED_FACE('',(#1842),#382,.F.);
#10488=ADVANCED_FACE('',(#1843),#383,.F.);
#10489=ADVANCED_FACE('',(#1844),#384,.F.);
#10490=ADVANCED_FACE('',(#1845),#385,.F.);
#10491=ADVANCED_FACE('',(#1846),#386,.F.);
#10492=ADVANCED_FACE('',(#1847),#387,.F.);
#10493=ADVANCED_FACE('',(#1848),#388,.F.);
#10494=ADVANCED_FACE('',(#1849),#389,.F.);
#10495=ADVANCED_FACE('',(#1850),#390,.F.);
#10496=ADVANCED_FACE('',(#1851),#391,.F.);
#10497=ADVANCED_FACE('',(#1852),#392,.F.);
#10498=ADVANCED_FACE('',(#1853),#393,.F.);
#10499=ADVANCED_FACE('',(#1854),#394,.F.);
#10500=ADVANCED_FACE('',(#1855),#395,.F.);
#10501=ADVANCED_FACE('',(#1856),#396,.F.);
#10502=ADVANCED_FACE('',(#1857),#397,.F.);
#10503=ADVANCED_FACE('',(#1858),#398,.F.);
#10504=ADVANCED_FACE('',(#1859),#399,.F.);
#10505=ADVANCED_FACE('',(#1860),#400,.F.);
#10506=ADVANCED_FACE('',(#1861),#401,.F.);
#10507=ADVANCED_FACE('',(#1862),#402,.F.);
#10508=ADVANCED_FACE('',(#1863),#403,.F.);
#10509=ADVANCED_FACE('',(#1864),#404,.F.);
#10510=ADVANCED_FACE('',(#1865),#405,.F.);
#10511=ADVANCED_FACE('',(#1866),#406,.F.);
#10512=ADVANCED_FACE('',(#1867),#407,.F.);
#10513=ADVANCED_FACE('',(#1868),#408,.F.);
#10514=ADVANCED_FACE('',(#1869),#409,.F.);
#10515=ADVANCED_FACE('',(#1870),#410,.F.);
#10516=ADVANCED_FACE('',(#1871),#411,.F.);
#10517=ADVANCED_FACE('',(#1872),#412,.F.);
#10518=ADVANCED_FACE('',(#1873),#413,.F.);
#10519=ADVANCED_FACE('',(#1874),#414,.F.);
#10520=ADVANCED_FACE('',(#1875),#415,.F.);
#10521=ADVANCED_FACE('',(#1876),#416,.F.);
#10522=ADVANCED_FACE('',(#1877),#417,.F.);
#10523=ADVANCED_FACE('',(#1878),#418,.F.);
#10524=ADVANCED_FACE('',(#1879),#419,.F.);
#10525=ADVANCED_FACE('',(#1880),#420,.F.);
#10526=ADVANCED_FACE('',(#1881),#421,.F.);
#10527=ADVANCED_FACE('',(#1882),#422,.F.);
#10528=ADVANCED_FACE('',(#1883),#423,.F.);
#10529=ADVANCED_FACE('',(#1884),#424,.F.);
#10530=ADVANCED_FACE('',(#1885),#425,.F.);
#10531=ADVANCED_FACE('',(#1886),#426,.F.);
#10532=ADVANCED_FACE('',(#1887),#427,.F.);
#10533=ADVANCED_FACE('',(#1888),#428,.F.);
#10534=ADVANCED_FACE('',(#1889),#429,.F.);
#10535=ADVANCED_FACE('',(#1890),#430,.F.);
#10536=ADVANCED_FACE('',(#1891),#431,.F.);
#10537=ADVANCED_FACE('',(#1892),#432,.F.);
#10538=ADVANCED_FACE('',(#1893),#433,.F.);
#10539=ADVANCED_FACE('',(#1894),#434,.F.);
#10540=ADVANCED_FACE('',(#1895),#435,.F.);
#10541=ADVANCED_FACE('',(#1896),#436,.F.);
#10542=ADVANCED_FACE('',(#1897),#437,.F.);
#10543=ADVANCED_FACE('',(#1898),#438,.F.);
#10544=ADVANCED_FACE('',(#1899),#439,.F.);
#10545=ADVANCED_FACE('',(#1900),#440,.F.);
#10546=ADVANCED_FACE('',(#1901),#441,.F.);
#10547=ADVANCED_FACE('',(#1902),#442,.F.);
#10548=ADVANCED_FACE('',(#1903),#443,.F.);
#10549=ADVANCED_FACE('',(#1904),#444,.F.);
#10550=ADVANCED_FACE('',(#1905),#445,.F.);
#10551=ADVANCED_FACE('',(#1906),#446,.F.);
#10552=ADVANCED_FACE('',(#1907),#447,.F.);
#10553=ADVANCED_FACE('',(#1908),#448,.F.);
#10554=ADVANCED_FACE('',(#1909),#449,.F.);
#10555=ADVANCED_FACE('',(#1910),#450,.F.);
#10556=ADVANCED_FACE('',(#1911),#451,.F.);
#10557=ADVANCED_FACE('',(#1912),#452,.F.);
#10558=ADVANCED_FACE('',(#1913),#453,.F.);
#10559=ADVANCED_FACE('',(#1914),#454,.F.);
#10560=ADVANCED_FACE('',(#1915),#455,.F.);
#10561=ADVANCED_FACE('',(#1916),#456,.F.);
#10562=ADVANCED_FACE('',(#1917),#457,.F.);
#10563=ADVANCED_FACE('',(#1918),#458,.F.);
#10564=ADVANCED_FACE('',(#1919),#459,.F.);
#10565=ADVANCED_FACE('',(#1920),#460,.F.);
#10566=ADVANCED_FACE('',(#1921),#461,.F.);
#10567=ADVANCED_FACE('',(#1922),#462,.F.);
#10568=ADVANCED_FACE('',(#1923),#463,.T.);
#10569=ADVANCED_FACE('',(#1924),#464,.T.);
#10570=ADVANCED_FACE('',(#1925),#465,.T.);
#10571=ADVANCED_FACE('',(#1926),#466,.T.);
#10572=ADVANCED_FACE('',(#1927),#467,.T.);
#10573=ADVANCED_FACE('',(#1928),#468,.T.);
#10574=ADVANCED_FACE('',(#1929),#469,.T.);
#10575=ADVANCED_FACE('',(#1930),#470,.T.);
#10576=ADVANCED_FACE('',(#1931),#471,.T.);
#10577=ADVANCED_FACE('',(#1932),#472,.T.);
#10578=ADVANCED_FACE('',(#1933),#473,.T.);
#10579=ADVANCED_FACE('',(#1934),#474,.T.);
#10580=ADVANCED_FACE('',(#1935),#475,.T.);
#10581=ADVANCED_FACE('',(#1936),#476,.T.);
#10582=ADVANCED_FACE('',(#1937),#477,.T.);
#10583=ADVANCED_FACE('',(#1938),#478,.T.);
#10584=ADVANCED_FACE('',(#1939),#479,.T.);
#10585=ADVANCED_FACE('',(#1940),#480,.T.);
#10586=ADVANCED_FACE('',(#1941),#481,.T.);
#10587=ADVANCED_FACE('',(#1942),#482,.T.);
#10588=ADVANCED_FACE('',(#1943),#483,.T.);
#10589=ADVANCED_FACE('',(#1944),#484,.T.);
#10590=ADVANCED_FACE('',(#1945),#485,.T.);
#10591=ADVANCED_FACE('',(#1946),#486,.T.);
#10592=ADVANCED_FACE('',(#1947),#487,.T.);
#10593=ADVANCED_FACE('',(#1948),#488,.T.);
#10594=ADVANCED_FACE('',(#1949),#489,.T.);
#10595=ADVANCED_FACE('',(#1950),#490,.T.);
#10596=ADVANCED_FACE('',(#1951),#491,.T.);
#10597=ADVANCED_FACE('',(#1952),#492,.T.);
#10598=ADVANCED_FACE('',(#1953),#493,.T.);
#10599=ADVANCED_FACE('',(#1954),#494,.T.);
#10600=ADVANCED_FACE('',(#1955),#495,.T.);
#10601=ADVANCED_FACE('',(#1956),#496,.T.);
#10602=ADVANCED_FACE('',(#1957),#497,.T.);
#10603=ADVANCED_FACE('',(#1958),#498,.T.);
#10604=ADVANCED_FACE('',(#1959),#499,.T.);
#10605=ADVANCED_FACE('',(#1960),#500,.T.);
#10606=ADVANCED_FACE('',(#1961),#501,.T.);
#10607=ADVANCED_FACE('',(#1962),#502,.T.);
#10608=ADVANCED_FACE('',(#1963),#503,.T.);
#10609=ADVANCED_FACE('',(#1964),#504,.T.);
#10610=ADVANCED_FACE('',(#1965),#505,.T.);
#10611=ADVANCED_FACE('',(#1966),#506,.T.);
#10612=ADVANCED_FACE('',(#1967),#507,.T.);
#10613=ADVANCED_FACE('',(#1968),#508,.T.);
#10614=ADVANCED_FACE('',(#1969),#509,.T.);
#10615=ADVANCED_FACE('',(#1970),#510,.T.);
#10616=ADVANCED_FACE('',(#1971),#511,.T.);
#10617=ADVANCED_FACE('',(#1972),#512,.T.);
#10618=ADVANCED_FACE('',(#1973),#513,.T.);
#10619=ADVANCED_FACE('',(#1974),#514,.T.);
#10620=ADVANCED_FACE('',(#1975),#515,.T.);
#10621=ADVANCED_FACE('',(#1976),#516,.T.);
#10622=ADVANCED_FACE('',(#1977),#517,.T.);
#10623=ADVANCED_FACE('',(#1978),#518,.T.);
#10624=ADVANCED_FACE('',(#1979),#519,.T.);
#10625=ADVANCED_FACE('',(#1980),#520,.T.);
#10626=ADVANCED_FACE('',(#1981),#521,.T.);
#10627=ADVANCED_FACE('',(#1982),#522,.T.);
#10628=ADVANCED_FACE('',(#1983),#523,.T.);
#10629=ADVANCED_FACE('',(#1984),#524,.T.);
#10630=ADVANCED_FACE('',(#1985),#525,.T.);
#10631=ADVANCED_FACE('',(#1986),#526,.T.);
#10632=ADVANCED_FACE('',(#1987),#527,.T.);
#10633=ADVANCED_FACE('',(#1988),#528,.T.);
#10634=ADVANCED_FACE('',(#1989),#529,.T.);
#10635=ADVANCED_FACE('',(#1990),#530,.T.);
#10636=ADVANCED_FACE('',(#1991),#531,.T.);
#10637=ADVANCED_FACE('',(#1992),#532,.T.);
#10638=ADVANCED_FACE('',(#1993),#533,.T.);
#10639=ADVANCED_FACE('',(#1994),#534,.T.);
#10640=ADVANCED_FACE('',(#1995),#535,.T.);
#10641=ADVANCED_FACE('',(#1996),#536,.T.);
#10642=ADVANCED_FACE('',(#1997),#537,.T.);
#10643=ADVANCED_FACE('',(#1998),#538,.T.);
#10644=ADVANCED_FACE('',(#1999),#539,.T.);
#10645=ADVANCED_FACE('',(#2000),#540,.T.);
#10646=ADVANCED_FACE('',(#2001),#541,.T.);
#10647=ADVANCED_FACE('',(#2002),#542,.T.);
#10648=ADVANCED_FACE('',(#2003),#543,.T.);
#10649=ADVANCED_FACE('',(#2004),#544,.T.);
#10650=ADVANCED_FACE('',(#2005),#545,.T.);
#10651=ADVANCED_FACE('',(#2006),#546,.T.);
#10652=ADVANCED_FACE('',(#2007),#547,.T.);
#10653=ADVANCED_FACE('',(#2008),#548,.T.);
#10654=ADVANCED_FACE('',(#2009),#549,.T.);
#10655=ADVANCED_FACE('',(#2010),#550,.T.);
#10656=ADVANCED_FACE('',(#2011),#551,.T.);
#10657=ADVANCED_FACE('',(#2012),#552,.T.);
#10658=ADVANCED_FACE('',(#2013),#553,.T.);
#10659=ADVANCED_FACE('',(#2014),#554,.T.);
#10660=ADVANCED_FACE('',(#2015),#555,.T.);
#10661=ADVANCED_FACE('',(#2016),#556,.T.);
#10662=ADVANCED_FACE('',(#2017),#557,.T.);
#10663=ADVANCED_FACE('',(#2018),#558,.T.);
#10664=ADVANCED_FACE('',(#2019),#559,.T.);
#10665=ADVANCED_FACE('',(#2020),#560,.T.);
#10666=ADVANCED_FACE('',(#2021),#561,.T.);
#10667=ADVANCED_FACE('',(#2022),#562,.T.);
#10668=ADVANCED_FACE('',(#2023),#563,.T.);
#10669=ADVANCED_FACE('',(#2024),#564,.T.);
#10670=ADVANCED_FACE('',(#2025),#565,.T.);
#10671=ADVANCED_FACE('',(#2026),#566,.T.);
#10672=ADVANCED_FACE('',(#2027),#567,.T.);
#10673=ADVANCED_FACE('',(#2028),#568,.T.);
#10674=ADVANCED_FACE('',(#2029),#569,.T.);
#10675=ADVANCED_FACE('',(#2030),#570,.T.);
#10676=ADVANCED_FACE('',(#2031),#571,.T.);
#10677=ADVANCED_FACE('',(#2032),#572,.T.);
#10678=ADVANCED_FACE('',(#2033),#573,.T.);
#10679=ADVANCED_FACE('',(#2034),#574,.T.);
#10680=ADVANCED_FACE('',(#2035),#575,.T.);
#10681=ADVANCED_FACE('',(#2036),#576,.T.);
#10682=ADVANCED_FACE('',(#2037),#577,.T.);
#10683=ADVANCED_FACE('',(#2038),#578,.T.);
#10684=ADVANCED_FACE('',(#2039),#579,.T.);
#10685=ADVANCED_FACE('',(#2040),#580,.T.);
#10686=ADVANCED_FACE('',(#2041),#581,.T.);
#10687=ADVANCED_FACE('',(#2042),#582,.T.);
#10688=ADVANCED_FACE('',(#2043),#583,.T.);
#10689=ADVANCED_FACE('',(#2044),#584,.T.);
#10690=ADVANCED_FACE('',(#2045),#585,.T.);
#10691=ADVANCED_FACE('',(#2046),#586,.T.);
#10692=ADVANCED_FACE('',(#2047),#587,.T.);
#10693=ADVANCED_FACE('',(#2048),#588,.T.);
#10694=ADVANCED_FACE('',(#2049),#589,.T.);
#10695=ADVANCED_FACE('',(#2050),#590,.T.);
#10696=ADVANCED_FACE('',(#2051),#591,.T.);
#10822=CLOSED_SHELL('',(#10293,#10294,#10295,#10296,#10297,#10298,#10299,
#10300,#10301,#10302,#10303,#10304,#10305,#10306,#10307,#10308,#10309,#10310,
#10311,#10312,#10313,#10314,#10315,#10316,#10317,#10318,#10319,#10320,#10321,
#10322,#10323,#10324,#10325,#10326,#10327,#10328,#10329,#10330,#10331,#10332,
#10333,#10334,#10335,#10336,#10337,#10338,#10339,#10340,#10341,#10342,#10343,
#10344,#10345,#10346,#10347,#10348,#10349,#10350,#10351,#10352,#10353,#10354,
#10355,#10356,#10357,#10358,#10359,#10360,#10361,#10362,#10363,#10364,#10365,
#10366,#10367,#10368,#10369,#10370,#10371,#10372,#10373,#10374,#10375,#10376,
#10377,#10378,#10379,#10380,#10381,#10382,#10383,#10384,#10385,#10386,#10387,
#10388,#10389,#10390,#10391,#10392,#10393,#10394,#10395,#10396,#10397,#10398,
#10399,#10400,#10401,#10402,#10403,#10404,#10405,#10406,#10407,#10408,#10409,
#10410,#10411,#10412,#10413,#10414,#10415,#10416,#10417,#10418,#10419,#10420,
#10421,#10422,#10423,#10424,#10425,#10426,#10427,#10428,#10429,#10430,#10431,
#10432,#10433,#10434,#10435,#10436,#10437,#10438,#10439,#10440,#10441,#10442,
#10443,#10444,#10445,#10446,#10447,#10448,#10449,#10450,#10451,#10452,#10453,
#10454,#10455,#10456,#10457,#10458,#10459,#10460,#10461,#10462,#10463,#10464,
#10465,#10466,#10467,#10468,#10469,#10470,#10471,#10472,#10473,#10474,#10475,
#10476,#10477,#10478,#10479,#10480,#10481,#10482,#10483,#10484,#10485,#10486,
#10487,#10488,#10489,#10490,#10491,#10492,#10493,#10494,#10495,#10496,#10497,
#10498,#10499,#10500,#10501,#10502,#10503,#10504,#10505,#10506,#10507,#10508,
#10509,#10510,#10511,#10512,#10513,#10514,#10515,#10516,#10517,#10518,#10519,
#10520,#10521,#10522,#10523,#10524,#10525,#10526,#10527,#10528,#10529,#10530,
#10531,#10532,#10533,#10534,#10535,#10536,#10537,#10538,#10539,#10540,#10541,
#10542,#10543,#10544,#10545,#10546,#10547,#10548,#10549,#10550,#10551,#10552,
#10553,#10554,#10555,#10556,#10557,#10558,#10559,#10560,#10561,#10562,#10563,
#10564,#10565,#10566,#10567,#10568,#10569,#10570,#10571,#10572,#10573,#10574,
#10575,#10576,#10577,#10578,#10579,#10580,#10581,#10582,#10583,#10584,#10585,
#10586,#10587,#10588,#10589,#10590,#10591,#10592,#10593,#10594,#10595,#10596,
#10597,#10598,#10599,#10600,#10601,#10602,#10603,#10604,#10605,#10606,#10607,
#10608,#10609,#10610,#10611,#10612,#10613,#10614,#10615,#10616,#10617,#10618,
#10619,#10620,#10621,#10622,#10623,#10624,#10625,#10626,#10627,#10628,#10629,
#10630,#10631,#10632,#10633,#10634,#10635,#10636,#10637,#10638,#10639,#10640,
#10641,#10642,#10643,#10644,#10645,#10646,#10647,#10648,#10649,#10650,#10651,
#10652,#10653,#10654,#10655,#10656,#10657,#10658,#10659,#10660,#10661,#10662,
#10663,#10664,#10665,#10666,#10667,#10668,#10669,#10670,#10671,#10672,#10673,
#10674,#10675,#10676,#10677,#10678,#10679,#10680,#10681,#10682,#10683,#10684,
#10685,#10686,#10687,#10688,#10689,#10690,#10691,#10692,#10693,#10694,#10695,
#10696));
#11110=AXIS2_PLACEMENT_3D('',#17301,#12300,#12301);
#11111=AXIS2_PLACEMENT_3D('',#17302,#12302,#12303);
#11112=AXIS2_PLACEMENT_3D('',#17319,#12304,#12305);
#11113=AXIS2_PLACEMENT_3D('',#17342,#12306,#12307);
#11114=AXIS2_PLACEMENT_3D('',#17343,#12308,#12309);
#11115=AXIS2_PLACEMENT_3D('',#17360,#12310,#12311);
#11116=AXIS2_PLACEMENT_3D('',#17383,#12312,#12313);
#11117=AXIS2_PLACEMENT_3D('',#17384,#12314,#12315);
#11118=AXIS2_PLACEMENT_3D('',#17407,#12316,#12317);
#11119=AXIS2_PLACEMENT_3D('',#17430,#12318,#12319);
#11120=AXIS2_PLACEMENT_3D('',#17431,#12320,#12321);
#11121=AXIS2_PLACEMENT_3D('',#17448,#12322,#12323);
#11122=AXIS2_PLACEMENT_3D('',#17465,#12324,#12325);
#11123=AXIS2_PLACEMENT_3D('',#17466,#12326,#12327);
#11124=AXIS2_PLACEMENT_3D('',#17483,#12328,#12329);
#11125=AXIS2_PLACEMENT_3D('',#17506,#12330,#12331);
#11126=AXIS2_PLACEMENT_3D('',#17507,#12332,#12333);
#11127=AXIS2_PLACEMENT_3D('',#17524,#12334,#12335);
#11128=AXIS2_PLACEMENT_3D('',#17547,#12336,#12337);
#11129=AXIS2_PLACEMENT_3D('',#17548,#12338,#12339);
#11130=AXIS2_PLACEMENT_3D('',#17565,#12340,#12341);
#11131=AXIS2_PLACEMENT_3D('',#17588,#12342,#12343);
#11132=AXIS2_PLACEMENT_3D('',#17589,#12344,#12345);
#11133=AXIS2_PLACEMENT_3D('',#17606,#12346,#12347);
#11134=AXIS2_PLACEMENT_3D('',#17629,#12348,#12349);
#11135=AXIS2_PLACEMENT_3D('',#17630,#12350,#12351);
#11136=AXIS2_PLACEMENT_3D('',#17647,#12352,#12353);
#11137=AXIS2_PLACEMENT_3D('',#17670,#12354,#12355);
#11138=AXIS2_PLACEMENT_3D('',#17671,#12356,#12357);
#11139=AXIS2_PLACEMENT_3D('',#17688,#12358,#12359);
#11140=AXIS2_PLACEMENT_3D('',#17711,#12360,#12361);
#11141=AXIS2_PLACEMENT_3D('',#17712,#12362,#12363);
#11142=AXIS2_PLACEMENT_3D('',#17729,#12364,#12365);
#11143=AXIS2_PLACEMENT_3D('',#17752,#12366,#12367);
#11144=AXIS2_PLACEMENT_3D('',#17753,#12368,#12369);
#11145=AXIS2_PLACEMENT_3D('',#17776,#12370,#12371);
#11146=AXIS2_PLACEMENT_3D('',#17799,#12372,#12373);
#11147=AXIS2_PLACEMENT_3D('',#17800,#12374,#12375);
#11148=AXIS2_PLACEMENT_3D('',#17817,#12376,#12377);
#11149=AXIS2_PLACEMENT_3D('',#17834,#12378,#12379);
#11150=AXIS2_PLACEMENT_3D('',#17835,#12380,#12381);
#11151=AXIS2_PLACEMENT_3D('',#17852,#12382,#12383);
#11152=AXIS2_PLACEMENT_3D('',#17875,#12384,#12385);
#11153=AXIS2_PLACEMENT_3D('',#17876,#12386,#12387);
#11154=AXIS2_PLACEMENT_3D('',#17893,#12388,#12389);
#11155=AXIS2_PLACEMENT_3D('',#17916,#12390,#12391);
#11156=AXIS2_PLACEMENT_3D('',#17917,#12392,#12393);
#11157=AXIS2_PLACEMENT_3D('',#17934,#12394,#12395);
#11158=AXIS2_PLACEMENT_3D('',#17957,#12396,#12397);
#11159=AXIS2_PLACEMENT_3D('',#17958,#12398,#12399);
#11160=AXIS2_PLACEMENT_3D('',#17975,#12400,#12401);
#11161=AXIS2_PLACEMENT_3D('',#17998,#12402,#12403);
#11162=AXIS2_PLACEMENT_3D('',#17999,#12404,#12405);
#11163=AXIS2_PLACEMENT_3D('',#18016,#12406,#12407);
#11164=AXIS2_PLACEMENT_3D('',#18039,#12408,#12409);
#11165=AXIS2_PLACEMENT_3D('',#18040,#12410,#12411);
#11166=AXIS2_PLACEMENT_3D('',#18057,#12412,#12413);
#11167=AXIS2_PLACEMENT_3D('',#18080,#12414,#12415);
#11168=AXIS2_PLACEMENT_3D('',#18081,#12416,#12417);
#11169=AXIS2_PLACEMENT_3D('',#18098,#12418,#12419);
#11170=AXIS2_PLACEMENT_3D('',#18121,#12420,#12421);
#11171=AXIS2_PLACEMENT_3D('',#18122,#12422,#12423);
#11172=AXIS2_PLACEMENT_3D('',#18139,#12424,#12425);
#11173=AXIS2_PLACEMENT_3D('',#18162,#12426,#12427);
#11174=AXIS2_PLACEMENT_3D('',#18163,#12428,#12429);
#11175=AXIS2_PLACEMENT_3D('',#18180,#12430,#12431);
#11176=AXIS2_PLACEMENT_3D('',#18203,#12432,#12433);
#11177=AXIS2_PLACEMENT_3D('',#18204,#12434,#12435);
#11178=AXIS2_PLACEMENT_3D('',#18221,#12436,#12437);
#11179=AXIS2_PLACEMENT_3D('',#18244,#12438,#12439);
#11180=AXIS2_PLACEMENT_3D('',#18245,#12440,#12441);
#11181=AXIS2_PLACEMENT_3D('',#18262,#12442,#12443);
#11182=AXIS2_PLACEMENT_3D('',#18285,#12444,#12445);
#11183=AXIS2_PLACEMENT_3D('',#18286,#12446,#12447);
#11184=AXIS2_PLACEMENT_3D('',#18309,#12448,#12449);
#11185=AXIS2_PLACEMENT_3D('',#18332,#12450,#12451);
#11186=AXIS2_PLACEMENT_3D('',#18333,#12452,#12453);
#11187=AXIS2_PLACEMENT_3D('',#18356,#12454,#12455);
#11188=AXIS2_PLACEMENT_3D('',#18373,#12456,#12457);
#11189=AXIS2_PLACEMENT_3D('',#18374,#12458,#12459);
#11190=AXIS2_PLACEMENT_3D('',#18391,#12460,#12461);
#11191=AXIS2_PLACEMENT_3D('',#18408,#12462,#12463);
#11192=AXIS2_PLACEMENT_3D('',#18409,#12464,#12465);
#11193=AXIS2_PLACEMENT_3D('',#18426,#12466,#12467);
#11194=AXIS2_PLACEMENT_3D('',#18449,#12468,#12469);
#11195=AXIS2_PLACEMENT_3D('',#18450,#12470,#12471);
#11196=AXIS2_PLACEMENT_3D('',#18467,#12472,#12473);
#11197=AXIS2_PLACEMENT_3D('',#18490,#12474,#12475);
#11198=AXIS2_PLACEMENT_3D('',#18491,#12476,#12477);
#11199=AXIS2_PLACEMENT_3D('',#18508,#12478,#12479);
#11200=AXIS2_PLACEMENT_3D('',#18531,#12480,#12481);
#11201=AXIS2_PLACEMENT_3D('',#18532,#12482,#12483);
#11202=AXIS2_PLACEMENT_3D('',#18549,#12484,#12485);
#11203=AXIS2_PLACEMENT_3D('',#18572,#12486,#12487);
#11204=AXIS2_PLACEMENT_3D('',#18573,#12488,#12489);
#11205=AXIS2_PLACEMENT_3D('',#18590,#12490,#12491);
#11206=AXIS2_PLACEMENT_3D('',#18613,#12492,#12493);
#11207=AXIS2_PLACEMENT_3D('',#18614,#12494,#12495);
#11208=AXIS2_PLACEMENT_3D('',#18637,#12496,#12497);
#11209=AXIS2_PLACEMENT_3D('',#18660,#12498,#12499);
#11210=AXIS2_PLACEMENT_3D('',#18661,#12500,#12501);
#11211=AXIS2_PLACEMENT_3D('',#18684,#12502,#12503);
#11212=AXIS2_PLACEMENT_3D('',#18701,#12504,#12505);
#11213=AXIS2_PLACEMENT_3D('',#18702,#12506,#12507);
#11214=AXIS2_PLACEMENT_3D('',#18719,#12508,#12509);
#11215=AXIS2_PLACEMENT_3D('',#18736,#12510,#12511);
#11216=AXIS2_PLACEMENT_3D('',#18737,#12512,#12513);
#11217=AXIS2_PLACEMENT_3D('',#18754,#12514,#12515);
#11218=AXIS2_PLACEMENT_3D('',#18777,#12516,#12517);
#11219=AXIS2_PLACEMENT_3D('',#18778,#12518,#12519);
#11220=AXIS2_PLACEMENT_3D('',#18795,#12520,#12521);
#11221=AXIS2_PLACEMENT_3D('',#18818,#12522,#12523);
#11222=AXIS2_PLACEMENT_3D('',#18819,#12524,#12525);
#11223=AXIS2_PLACEMENT_3D('',#18836,#12526,#12527);
#11224=AXIS2_PLACEMENT_3D('',#18859,#12528,#12529);
#11225=AXIS2_PLACEMENT_3D('',#18860,#12530,#12531);
#11226=AXIS2_PLACEMENT_3D('',#18877,#12532,#12533);
#11227=AXIS2_PLACEMENT_3D('',#18900,#12534,#12535);
#11228=AXIS2_PLACEMENT_3D('',#18901,#12536,#12537);
#11229=AXIS2_PLACEMENT_3D('',#18918,#12538,#12539);
#11230=AXIS2_PLACEMENT_3D('',#18941,#12540,#12541);
#11231=AXIS2_PLACEMENT_3D('',#18942,#12542,#12543);
#11232=AXIS2_PLACEMENT_3D('',#18959,#12544,#12545);
#11233=AXIS2_PLACEMENT_3D('',#18982,#12546,#12547);
#11234=AXIS2_PLACEMENT_3D('',#18983,#12548,#12549);
#11235=AXIS2_PLACEMENT_3D('',#19000,#12550,#12551);
#11236=AXIS2_PLACEMENT_3D('',#19023,#12552,#12553);
#11237=AXIS2_PLACEMENT_3D('',#19024,#12554,#12555);
#11238=AXIS2_PLACEMENT_3D('',#19041,#12556,#12557);
#11239=AXIS2_PLACEMENT_3D('',#19058,#12558,#12559);
#11240=AXIS2_PLACEMENT_3D('',#19059,#12560,#12561);
#11241=AXIS2_PLACEMENT_3D('',#19082,#12562,#12563);
#11242=AXIS2_PLACEMENT_3D('',#19105,#12564,#12565);
#11243=AXIS2_PLACEMENT_3D('',#19106,#12566,#12567);
#11244=AXIS2_PLACEMENT_3D('',#19130,#12568,#12569);
#11245=AXIS2_PLACEMENT_3D('',#19159,#12570,#12571);
#11246=AXIS2_PLACEMENT_3D('',#19188,#12572,#12573);
#11247=AXIS2_PLACEMENT_3D('',#19217,#12574,#12575);
#11248=AXIS2_PLACEMENT_3D('',#19246,#12576,#12577);
#11249=AXIS2_PLACEMENT_3D('',#19275,#12578,#12579);
#11250=AXIS2_PLACEMENT_3D('',#19304,#12580,#12581);
#11251=AXIS2_PLACEMENT_3D('',#19333,#12582,#12583);
#11252=AXIS2_PLACEMENT_3D('',#19362,#12584,#12585);
#11253=AXIS2_PLACEMENT_3D('',#19391,#12586,#12587);
#11254=AXIS2_PLACEMENT_3D('',#19420,#12588,#12589);
#11255=AXIS2_PLACEMENT_3D('',#19449,#12590,#12591);
#11256=AXIS2_PLACEMENT_3D('',#19478,#12592,#12593);
#11257=AXIS2_PLACEMENT_3D('',#19507,#12594,#12595);
#11258=AXIS2_PLACEMENT_3D('',#19536,#12596,#12597);
#11259=AXIS2_PLACEMENT_3D('',#19565,#12598,#12599);
#11260=AXIS2_PLACEMENT_3D('',#19594,#12600,#12601);
#11261=AXIS2_PLACEMENT_3D('',#19623,#12602,#12603);
#11262=AXIS2_PLACEMENT_3D('',#19652,#12604,#12605);
#11263=AXIS2_PLACEMENT_3D('',#19681,#12606,#12607);
#11264=AXIS2_PLACEMENT_3D('',#19710,#12608,#12609);
#11265=AXIS2_PLACEMENT_3D('',#19739,#12610,#12611);
#11266=AXIS2_PLACEMENT_3D('',#19757,#12613,#12614);
#11267=AXIS2_PLACEMENT_3D('',#19778,#12615,#12616);
#11268=AXIS2_PLACEMENT_3D('',#19807,#12617,#12618);
#11269=AXIS2_PLACEMENT_3D('',#19836,#12619,#12620);
#11270=AXIS2_PLACEMENT_3D('',#19865,#12621,#12622);
#11271=AXIS2_PLACEMENT_3D('',#19894,#12623,#12624);
#11272=AXIS2_PLACEMENT_3D('',#19923,#12625,#12626);
#11273=AXIS2_PLACEMENT_3D('',#19952,#12627,#12628);
#11274=AXIS2_PLACEMENT_3D('',#19981,#12629,#12630);
#11275=AXIS2_PLACEMENT_3D('',#20010,#12631,#12632);
#11276=AXIS2_PLACEMENT_3D('',#20039,#12633,#12634);
#11277=AXIS2_PLACEMENT_3D('',#20068,#12635,#12636);
#11278=AXIS2_PLACEMENT_3D('',#20097,#12637,#12638);
#11279=AXIS2_PLACEMENT_3D('',#20126,#12639,#12640);
#11280=AXIS2_PLACEMENT_3D('',#20155,#12641,#12642);
#11281=AXIS2_PLACEMENT_3D('',#20184,#12643,#12644);
#11282=AXIS2_PLACEMENT_3D('',#20213,#12645,#12646);
#11283=AXIS2_PLACEMENT_3D('',#20242,#12647,#12648);
#11284=AXIS2_PLACEMENT_3D('',#20271,#12649,#12650);
#11285=AXIS2_PLACEMENT_3D('',#20300,#12651,#12652);
#11286=AXIS2_PLACEMENT_3D('',#20329,#12653,#12654);
#11287=AXIS2_PLACEMENT_3D('',#20358,#12655,#12656);
#11288=AXIS2_PLACEMENT_3D('',#20387,#12657,#12658);
#11289=AXIS2_PLACEMENT_3D('',#20395,#12659,#12660);
#11290=AXIS2_PLACEMENT_3D('',#20398,#12661,#12662);
#11291=AXIS2_PLACEMENT_3D('',#20402,#12664,#12665);
#11292=AXIS2_PLACEMENT_3D('',#20404,#12667,#12668);
#11293=AXIS2_PLACEMENT_3D('',#20428,#12669,#12670);
#11294=AXIS2_PLACEMENT_3D('',#20457,#12671,#12672);
#11295=AXIS2_PLACEMENT_3D('',#20486,#12673,#12674);
#11296=AXIS2_PLACEMENT_3D('',#20515,#12675,#12676);
#11297=AXIS2_PLACEMENT_3D('',#20544,#12677,#12678);
#11298=AXIS2_PLACEMENT_3D('',#20573,#12679,#12680);
#11299=AXIS2_PLACEMENT_3D('',#20602,#12681,#12682);
#11300=AXIS2_PLACEMENT_3D('',#20631,#12683,#12684);
#11301=AXIS2_PLACEMENT_3D('',#20660,#12685,#12686);
#11302=AXIS2_PLACEMENT_3D('',#20689,#12687,#12688);
#11303=AXIS2_PLACEMENT_3D('',#20718,#12689,#12690);
#11304=AXIS2_PLACEMENT_3D('',#20747,#12691,#12692);
#11305=AXIS2_PLACEMENT_3D('',#20776,#12693,#12694);
#11306=AXIS2_PLACEMENT_3D('',#20805,#12695,#12696);
#11307=AXIS2_PLACEMENT_3D('',#20834,#12697,#12698);
#11308=AXIS2_PLACEMENT_3D('',#20863,#12699,#12700);
#11309=AXIS2_PLACEMENT_3D('',#20892,#12701,#12702);
#11310=AXIS2_PLACEMENT_3D('',#20921,#12703,#12704);
#11311=AXIS2_PLACEMENT_3D('',#20950,#12705,#12706);
#11312=AXIS2_PLACEMENT_3D('',#20979,#12707,#12708);
#11313=AXIS2_PLACEMENT_3D('',#21008,#12709,#12710);
#11314=AXIS2_PLACEMENT_3D('',#21037,#12711,#12712);
#11315=AXIS2_PLACEMENT_3D('',#21059,#12714,#12715);
#11316=AXIS2_PLACEMENT_3D('',#21076,#12716,#12717);
#11317=AXIS2_PLACEMENT_3D('',#21105,#12718,#12719);
#11318=AXIS2_PLACEMENT_3D('',#21134,#12720,#12721);
#11319=AXIS2_PLACEMENT_3D('',#21163,#12722,#12723);
#11320=AXIS2_PLACEMENT_3D('',#21192,#12724,#12725);
#11321=AXIS2_PLACEMENT_3D('',#21221,#12726,#12727);
#11322=AXIS2_PLACEMENT_3D('',#21250,#12728,#12729);
#11323=AXIS2_PLACEMENT_3D('',#21279,#12730,#12731);
#11324=AXIS2_PLACEMENT_3D('',#21308,#12732,#12733);
#11325=AXIS2_PLACEMENT_3D('',#21337,#12734,#12735);
#11326=AXIS2_PLACEMENT_3D('',#21366,#12736,#12737);
#11327=AXIS2_PLACEMENT_3D('',#21395,#12738,#12739);
#11328=AXIS2_PLACEMENT_3D('',#21424,#12740,#12741);
#11329=AXIS2_PLACEMENT_3D('',#21453,#12742,#12743);
#11330=AXIS2_PLACEMENT_3D('',#21482,#12744,#12745);
#11331=AXIS2_PLACEMENT_3D('',#21511,#12746,#12747);
#11332=AXIS2_PLACEMENT_3D('',#21540,#12748,#12749);
#11333=AXIS2_PLACEMENT_3D('',#21569,#12750,#12751);
#11334=AXIS2_PLACEMENT_3D('',#21598,#12752,#12753);
#11335=AXIS2_PLACEMENT_3D('',#21627,#12754,#12755);
#11336=AXIS2_PLACEMENT_3D('',#21656,#12756,#12757);
#11337=AXIS2_PLACEMENT_3D('',#21685,#12758,#12759);
#11338=AXIS2_PLACEMENT_3D('',#21693,#12760,#12761);
#11339=AXIS2_PLACEMENT_3D('',#21706,#12762,#12763);
#11340=AXIS2_PLACEMENT_3D('',#21719,#12764,#12765);
#11341=AXIS2_PLACEMENT_3D('',#21732,#12766,#12767);
#11342=AXIS2_PLACEMENT_3D('',#21745,#12768,#12769);
#11343=AXIS2_PLACEMENT_3D('',#21758,#12770,#12771);
#11344=AXIS2_PLACEMENT_3D('',#21771,#12772,#12773);
#11345=AXIS2_PLACEMENT_3D('',#21784,#12774,#12775);
#11346=AXIS2_PLACEMENT_3D('',#21797,#12776,#12777);
#11347=AXIS2_PLACEMENT_3D('',#21810,#12778,#12779);
#11348=AXIS2_PLACEMENT_3D('',#21823,#12780,#12781);
#11349=AXIS2_PLACEMENT_3D('',#21836,#12782,#12783);
#11350=AXIS2_PLACEMENT_3D('',#21849,#12784,#12785);
#11351=AXIS2_PLACEMENT_3D('',#21862,#12786,#12787);
#11352=AXIS2_PLACEMENT_3D('',#21875,#12788,#12789);
#11353=AXIS2_PLACEMENT_3D('',#21888,#12790,#12791);
#11354=AXIS2_PLACEMENT_3D('',#21901,#12792,#12793);
#11355=AXIS2_PLACEMENT_3D('',#21914,#12794,#12795);
#11356=AXIS2_PLACEMENT_3D('',#21927,#12796,#12797);
#11357=AXIS2_PLACEMENT_3D('',#21940,#12798,#12799);
#11358=AXIS2_PLACEMENT_3D('',#21953,#12800,#12801);
#11359=AXIS2_PLACEMENT_3D('',#21966,#12802,#12803);
#11360=AXIS2_PLACEMENT_3D('',#21979,#12804,#12805);
#11361=AXIS2_PLACEMENT_3D('',#21992,#12806,#12807);
#11362=AXIS2_PLACEMENT_3D('',#22005,#12808,#12809);
#11363=AXIS2_PLACEMENT_3D('',#22018,#12810,#12811);
#11364=AXIS2_PLACEMENT_3D('',#22031,#12812,#12813);
#11365=AXIS2_PLACEMENT_3D('',#22044,#12814,#12815);
#11366=AXIS2_PLACEMENT_3D('',#22057,#12816,#12817);
#11367=AXIS2_PLACEMENT_3D('',#22070,#12818,#12819);
#11368=AXIS2_PLACEMENT_3D('',#22083,#12820,#12821);
#11369=AXIS2_PLACEMENT_3D('',#22096,#12822,#12823);
#11370=AXIS2_PLACEMENT_3D('',#22109,#12824,#12825);
#11371=AXIS2_PLACEMENT_3D('',#22122,#12826,#12827);
#11372=AXIS2_PLACEMENT_3D('',#22135,#12828,#12829);
#11373=AXIS2_PLACEMENT_3D('',#22148,#12830,#12831);
#11374=AXIS2_PLACEMENT_3D('',#22161,#12832,#12833);
#11375=AXIS2_PLACEMENT_3D('',#22174,#12834,#12835);
#11376=AXIS2_PLACEMENT_3D('',#22187,#12836,#12837);
#11377=AXIS2_PLACEMENT_3D('',#22200,#12838,#12839);
#11378=AXIS2_PLACEMENT_3D('',#22213,#12840,#12841);
#11379=AXIS2_PLACEMENT_3D('',#22226,#12842,#12843);
#11380=AXIS2_PLACEMENT_3D('',#22239,#12844,#12845);
#11381=AXIS2_PLACEMENT_3D('',#22252,#12846,#12847);
#11382=AXIS2_PLACEMENT_3D('',#22265,#12848,#12849);
#11383=AXIS2_PLACEMENT_3D('',#22278,#12850,#12851);
#11384=AXIS2_PLACEMENT_3D('',#22291,#12852,#12853);
#11385=AXIS2_PLACEMENT_3D('',#22304,#12854,#12855);
#11386=AXIS2_PLACEMENT_3D('',#22317,#12856,#12857);
#11387=AXIS2_PLACEMENT_3D('',#22330,#12858,#12859);
#11388=AXIS2_PLACEMENT_3D('',#22343,#12860,#12861);
#11389=AXIS2_PLACEMENT_3D('',#22356,#12862,#12863);
#11390=AXIS2_PLACEMENT_3D('',#22369,#12864,#12865);
#11391=AXIS2_PLACEMENT_3D('',#22382,#12866,#12867);
#11392=AXIS2_PLACEMENT_3D('',#22395,#12868,#12869);
#11393=AXIS2_PLACEMENT_3D('',#22408,#12870,#12871);
#11394=AXIS2_PLACEMENT_3D('',#22421,#12872,#12873);
#11395=AXIS2_PLACEMENT_3D('',#22434,#12874,#12875);
#11396=AXIS2_PLACEMENT_3D('',#22447,#12876,#12877);
#11397=AXIS2_PLACEMENT_3D('',#22460,#12878,#12879);
#11398=AXIS2_PLACEMENT_3D('',#22473,#12880,#12881);
#11399=AXIS2_PLACEMENT_3D('',#22486,#12882,#12883);
#11400=AXIS2_PLACEMENT_3D('',#22499,#12884,#12885);
#11401=AXIS2_PLACEMENT_3D('',#22512,#12886,#12887);
#11402=AXIS2_PLACEMENT_3D('',#22525,#12888,#12889);
#11403=AXIS2_PLACEMENT_3D('',#22538,#12890,#12891);
#11404=AXIS2_PLACEMENT_3D('',#22551,#12892,#12893);
#11405=AXIS2_PLACEMENT_3D('',#22564,#12894,#12895);
#11406=AXIS2_PLACEMENT_3D('',#22577,#12896,#12897);
#11407=AXIS2_PLACEMENT_3D('',#22590,#12898,#12899);
#11408=AXIS2_PLACEMENT_3D('',#22603,#12900,#12901);
#11409=AXIS2_PLACEMENT_3D('',#22616,#12902,#12903);
#11410=AXIS2_PLACEMENT_3D('',#22629,#12904,#12905);
#11411=AXIS2_PLACEMENT_3D('',#22642,#12906,#12907);
#11412=AXIS2_PLACEMENT_3D('',#22655,#12908,#12909);
#11413=AXIS2_PLACEMENT_3D('',#22668,#12910,#12911);
#11414=AXIS2_PLACEMENT_3D('',#22681,#12912,#12913);
#11415=AXIS2_PLACEMENT_3D('',#22694,#12914,#12915);
#11416=AXIS2_PLACEMENT_3D('',#22707,#12916,#12917);
#11417=AXIS2_PLACEMENT_3D('',#22720,#12918,#12919);
#11418=AXIS2_PLACEMENT_3D('',#22733,#12920,#12921);
#11419=AXIS2_PLACEMENT_3D('',#22746,#12922,#12923);
#11420=AXIS2_PLACEMENT_3D('',#22759,#12924,#12925);
#11421=AXIS2_PLACEMENT_3D('',#22772,#12926,#12927);
#11422=AXIS2_PLACEMENT_3D('',#22785,#12928,#12929);
#11423=AXIS2_PLACEMENT_3D('',#22798,#12930,#12931);
#11424=AXIS2_PLACEMENT_3D('',#22811,#12932,#12933);
#11425=AXIS2_PLACEMENT_3D('',#22824,#12934,#12935);
#11426=AXIS2_PLACEMENT_3D('',#22837,#12936,#12937);
#11427=AXIS2_PLACEMENT_3D('',#22843,#12941,#12942);
#11428=AXIS2_PLACEMENT_3D('',#22849,#12946,#12947);
#11429=AXIS2_PLACEMENT_3D('',#22851,#12949,#12950);
#11430=AXIS2_PLACEMENT_3D('',#22853,#12952,#12953);
#11431=AXIS2_PLACEMENT_3D('',#22944,#12954,#12955);
#11432=AXIS2_PLACEMENT_3D('',#22946,#12956,#12957);
#11433=AXIS2_PLACEMENT_3D('',#22988,#12958,#12959);
#11434=AXIS2_PLACEMENT_3D('',#23025,#12960,#12961);
#11435=AXIS2_PLACEMENT_3D('',#23223,#12962,#12963);
#11436=AXIS2_PLACEMENT_3D('',#23318,#12964,#12965);
#11437=AXIS2_PLACEMENT_3D('',#23356,#12966,#12967);
#11438=AXIS2_PLACEMENT_3D('',#23357,#12968,#12969);
#11439=AXIS2_PLACEMENT_3D('',#23395,#12970,#12971);
#11440=AXIS2_PLACEMENT_3D('',#23490,#12972,#12973);
#11441=AXIS2_PLACEMENT_3D('',#23528,#12974,#12975);
#11442=AXIS2_PLACEMENT_3D('',#23529,#12976,#12977);
#11443=AXIS2_PLACEMENT_3D('',#23567,#12978,#12979);
#11444=AXIS2_PLACEMENT_3D('',#23615,#12980,#12981);
#11445=AXIS2_PLACEMENT_3D('',#23653,#12982,#12983);
#11446=AXIS2_PLACEMENT_3D('',#23654,#12984,#12985);
#11447=AXIS2_PLACEMENT_3D('',#23692,#12986,#12987);
#11448=AXIS2_PLACEMENT_3D('',#23787,#12988,#12989);
#11449=AXIS2_PLACEMENT_3D('',#23825,#12990,#12991);
#11450=AXIS2_PLACEMENT_3D('',#23826,#12992,#12993);
#11451=AXIS2_PLACEMENT_3D('',#23864,#12994,#12995);
#11452=AXIS2_PLACEMENT_3D('',#23959,#12996,#12997);
#11453=AXIS2_PLACEMENT_3D('',#23997,#12998,#12999);
#11454=AXIS2_PLACEMENT_3D('',#23998,#13000,#13001);
#11455=AXIS2_PLACEMENT_3D('',#24036,#13002,#13003);
#11456=AXIS2_PLACEMENT_3D('',#24131,#13004,#13005);
#11457=AXIS2_PLACEMENT_3D('',#24169,#13006,#13007);
#11458=AXIS2_PLACEMENT_3D('',#24170,#13008,#13009);
#11459=AXIS2_PLACEMENT_3D('',#24208,#13010,#13011);
#11460=AXIS2_PLACEMENT_3D('',#24303,#13012,#13013);
#11461=AXIS2_PLACEMENT_3D('',#24341,#13014,#13015);
#11462=AXIS2_PLACEMENT_3D('',#24342,#13016,#13017);
#11463=AXIS2_PLACEMENT_3D('',#24380,#13018,#13019);
#11464=AXIS2_PLACEMENT_3D('',#24475,#13020,#13021);
#11465=AXIS2_PLACEMENT_3D('',#24513,#13022,#13023);
#11466=AXIS2_PLACEMENT_3D('',#24514,#13024,#13025);
#11467=AXIS2_PLACEMENT_3D('',#24552,#13026,#13027);
#11468=AXIS2_PLACEMENT_3D('',#24647,#13028,#13029);
#11469=AXIS2_PLACEMENT_3D('',#24685,#13030,#13031);
#11470=AXIS2_PLACEMENT_3D('',#24686,#13032,#13033);
#11471=AXIS2_PLACEMENT_3D('',#24724,#13034,#13035);
#11472=AXIS2_PLACEMENT_3D('',#24819,#13036,#13037);
#11473=AXIS2_PLACEMENT_3D('',#24857,#13038,#13039);
#11474=AXIS2_PLACEMENT_3D('',#24858,#13040,#13041);
#11475=AXIS2_PLACEMENT_3D('',#24896,#13042,#13043);
#11476=AXIS2_PLACEMENT_3D('',#24991,#13044,#13045);
#11477=AXIS2_PLACEMENT_3D('',#25029,#13046,#13047);
#11478=AXIS2_PLACEMENT_3D('',#25030,#13048,#13049);
#11479=AXIS2_PLACEMENT_3D('',#25068,#13050,#13051);
#11480=AXIS2_PLACEMENT_3D('',#25116,#13052,#13053);
#11481=AXIS2_PLACEMENT_3D('',#25154,#13054,#13055);
#11482=AXIS2_PLACEMENT_3D('',#25155,#13056,#13057);
#11483=AXIS2_PLACEMENT_3D('',#25193,#13058,#13059);
#11484=AXIS2_PLACEMENT_3D('',#25288,#13060,#13061);
#11485=AXIS2_PLACEMENT_3D('',#25326,#13062,#13063);
#11486=AXIS2_PLACEMENT_3D('',#25327,#13064,#13065);
#11487=AXIS2_PLACEMENT_3D('',#25365,#13066,#13067);
#11488=AXIS2_PLACEMENT_3D('',#25460,#13068,#13069);
#11489=AXIS2_PLACEMENT_3D('',#25498,#13070,#13071);
#11490=AXIS2_PLACEMENT_3D('',#25499,#13072,#13073);
#11491=AXIS2_PLACEMENT_3D('',#25542,#13074,#13075);
#11492=AXIS2_PLACEMENT_3D('',#25580,#13076,#13077);
#11493=AXIS2_PLACEMENT_3D('',#25623,#13078,#13079);
#11494=AXIS2_PLACEMENT_3D('',#25624,#13080,#13081);
#11495=AXIS2_PLACEMENT_3D('',#25662,#13082,#13083);
#11496=AXIS2_PLACEMENT_3D('',#25757,#13084,#13085);
#11497=AXIS2_PLACEMENT_3D('',#25795,#13086,#13087);
#11498=AXIS2_PLACEMENT_3D('',#25796,#13088,#13089);
#11499=AXIS2_PLACEMENT_3D('',#25834,#13090,#13091);
#11500=AXIS2_PLACEMENT_3D('',#25929,#13092,#13093);
#11501=AXIS2_PLACEMENT_3D('',#25967,#13094,#13095);
#11502=AXIS2_PLACEMENT_3D('',#25968,#13096,#13097);
#11503=AXIS2_PLACEMENT_3D('',#26006,#13098,#13099);
#11504=AXIS2_PLACEMENT_3D('',#26101,#13100,#13101);
#11505=AXIS2_PLACEMENT_3D('',#26139,#13102,#13103);
#11506=AXIS2_PLACEMENT_3D('',#26140,#13104,#13105);
#11507=AXIS2_PLACEMENT_3D('',#26178,#13106,#13107);
#11508=AXIS2_PLACEMENT_3D('',#26273,#13108,#13109);
#11509=AXIS2_PLACEMENT_3D('',#26311,#13110,#13111);
#11510=AXIS2_PLACEMENT_3D('',#26312,#13112,#13113);
#11511=AXIS2_PLACEMENT_3D('',#26350,#13114,#13115);
#11512=AXIS2_PLACEMENT_3D('',#26445,#13116,#13117);
#11513=AXIS2_PLACEMENT_3D('',#26483,#13118,#13119);
#11514=AXIS2_PLACEMENT_3D('',#26484,#13120,#13121);
#11515=AXIS2_PLACEMENT_3D('',#26522,#13122,#13123);
#11516=AXIS2_PLACEMENT_3D('',#26617,#13124,#13125);
#11517=AXIS2_PLACEMENT_3D('',#26655,#13126,#13127);
#11518=AXIS2_PLACEMENT_3D('',#26656,#13128,#13129);
#11519=AXIS2_PLACEMENT_3D('',#26694,#13130,#13131);
#11520=AXIS2_PLACEMENT_3D('',#26789,#13132,#13133);
#11521=AXIS2_PLACEMENT_3D('',#26827,#13134,#13135);
#11522=AXIS2_PLACEMENT_3D('',#26828,#13136,#13137);
#11523=AXIS2_PLACEMENT_3D('',#26866,#13138,#13139);
#11524=AXIS2_PLACEMENT_3D('',#26961,#13140,#13141);
#11525=AXIS2_PLACEMENT_3D('',#26999,#13142,#13143);
#11526=AXIS2_PLACEMENT_3D('',#27000,#13144,#13145);
#11527=AXIS2_PLACEMENT_3D('',#27038,#13146,#13147);
#11528=AXIS2_PLACEMENT_3D('',#27133,#13148,#13149);
#11529=AXIS2_PLACEMENT_3D('',#27171,#13150,#13151);
#11530=AXIS2_PLACEMENT_3D('',#27172,#13152,#13153);
#11531=AXIS2_PLACEMENT_3D('',#27210,#13154,#13155);
#11532=AXIS2_PLACEMENT_3D('',#27258,#13156,#13157);
#11533=AXIS2_PLACEMENT_3D('',#27296,#13158,#13159);
#11534=AXIS2_PLACEMENT_3D('',#27297,#13160,#13161);
#11535=AXIS2_PLACEMENT_3D('',#27335,#13162,#13163);
#11536=AXIS2_PLACEMENT_3D('',#27383,#13164,#13165);
#11537=AXIS2_PLACEMENT_3D('',#27421,#13166,#13167);
#11538=AXIS2_PLACEMENT_3D('',#27422,#13168,#13169);
#11539=AXIS2_PLACEMENT_3D('',#27460,#13170,#13171);
#11540=AXIS2_PLACEMENT_3D('',#27555,#13172,#13173);
#11541=AXIS2_PLACEMENT_3D('',#27593,#13174,#13175);
#11542=AXIS2_PLACEMENT_3D('',#27594,#13176,#13177);
#11543=AXIS2_PLACEMENT_3D('',#27632,#13178,#13179);
#11544=AXIS2_PLACEMENT_3D('',#27727,#13180,#13181);
#11545=AXIS2_PLACEMENT_3D('',#27765,#13182,#13183);
#11546=AXIS2_PLACEMENT_3D('',#27766,#13184,#13185);
#11547=AXIS2_PLACEMENT_3D('',#27804,#13186,#13187);
#11548=AXIS2_PLACEMENT_3D('',#27899,#13188,#13189);
#11549=AXIS2_PLACEMENT_3D('',#27937,#13190,#13191);
#11550=AXIS2_PLACEMENT_3D('',#27938,#13192,#13193);
#11551=AXIS2_PLACEMENT_3D('',#27976,#13194,#13195);
#11552=AXIS2_PLACEMENT_3D('',#28071,#13196,#13197);
#11553=AXIS2_PLACEMENT_3D('',#28109,#13198,#13199);
#11554=AXIS2_PLACEMENT_3D('',#28110,#13200,#13201);
#11555=AXIS2_PLACEMENT_3D('',#28148,#13202,#13203);
#11556=AXIS2_PLACEMENT_3D('',#28243,#13204,#13205);
#11557=AXIS2_PLACEMENT_3D('',#28281,#13206,#13207);
#11558=AXIS2_PLACEMENT_3D('',#28282,#13208,#13209);
#11559=AXIS2_PLACEMENT_3D('',#28320,#13210,#13211);
#11560=AXIS2_PLACEMENT_3D('',#28415,#13212,#13213);
#11561=AXIS2_PLACEMENT_3D('',#28453,#13214,#13215);
#11562=AXIS2_PLACEMENT_3D('',#28454,#13216,#13217);
#11563=AXIS2_PLACEMENT_3D('',#28492,#13218,#13219);
#11564=AXIS2_PLACEMENT_3D('',#28540,#13220,#13221);
#11565=AXIS2_PLACEMENT_3D('',#28578,#13222,#13223);
#11566=AXIS2_PLACEMENT_3D('',#28579,#13224,#13225);
#11567=AXIS2_PLACEMENT_3D('',#28617,#13226,#13227);
#11568=AXIS2_PLACEMENT_3D('',#28665,#13228,#13229);
#11569=AXIS2_PLACEMENT_3D('',#28703,#13230,#13231);
#11570=AXIS2_PLACEMENT_3D('',#28704,#13232,#13233);
#11571=AXIS2_PLACEMENT_3D('',#28742,#13234,#13235);
#11572=AXIS2_PLACEMENT_3D('',#28837,#13236,#13237);
#11573=AXIS2_PLACEMENT_3D('',#28875,#13238,#13239);
#11574=AXIS2_PLACEMENT_3D('',#28876,#13240,#13241);
#11575=AXIS2_PLACEMENT_3D('',#28914,#13242,#13243);
#11576=AXIS2_PLACEMENT_3D('',#29009,#13244,#13245);
#11577=AXIS2_PLACEMENT_3D('',#29047,#13246,#13247);
#11578=AXIS2_PLACEMENT_3D('',#29048,#13248,#13249);
#11579=AXIS2_PLACEMENT_3D('',#29091,#13250,#13251);
#11580=AXIS2_PLACEMENT_3D('',#29129,#13252,#13253);
#11581=AXIS2_PLACEMENT_3D('',#29172,#13254,#13255);
#11582=AXIS2_PLACEMENT_3D('',#29173,#13256,#13257);
#11583=AXIS2_PLACEMENT_3D('',#29211,#13258,#13259);
#11584=AXIS2_PLACEMENT_3D('',#29306,#13260,#13261);
#11585=AXIS2_PLACEMENT_3D('',#29344,#13262,#13263);
#11586=AXIS2_PLACEMENT_3D('',#29345,#13264,#13265);
#11587=AXIS2_PLACEMENT_3D('',#29383,#13266,#13267);
#11588=AXIS2_PLACEMENT_3D('',#29478,#13268,#13269);
#11589=AXIS2_PLACEMENT_3D('',#29516,#13270,#13271);
#11590=AXIS2_PLACEMENT_3D('',#29517,#13272,#13273);
#11591=AXIS2_PLACEMENT_3D('',#29555,#13274,#13275);
#11592=AXIS2_PLACEMENT_3D('',#29650,#13276,#13277);
#11593=AXIS2_PLACEMENT_3D('',#29688,#13278,#13279);
#11594=AXIS2_PLACEMENT_3D('',#29689,#13280,#13281);
#11595=AXIS2_PLACEMENT_3D('',#29727,#13282,#13283);
#11596=AXIS2_PLACEMENT_3D('',#29822,#13284,#13285);
#11597=AXIS2_PLACEMENT_3D('',#29860,#13286,#13287);
#11598=AXIS2_PLACEMENT_3D('',#29861,#13288,#13289);
#11599=AXIS2_PLACEMENT_3D('',#29899,#13290,#13291);
#11600=AXIS2_PLACEMENT_3D('',#29994,#13292,#13293);
#11601=AXIS2_PLACEMENT_3D('',#30032,#13294,#13295);
#11602=AXIS2_PLACEMENT_3D('',#30033,#13296,#13297);
#11603=AXIS2_PLACEMENT_3D('',#30071,#13298,#13299);
#11604=AXIS2_PLACEMENT_3D('',#30119,#13300,#13301);
#11605=AXIS2_PLACEMENT_3D('',#30157,#13302,#13303);
#11606=AXIS2_PLACEMENT_3D('',#30158,#13304,#13305);
#12300=DIRECTION('axis',(0.,0.,1.));
#12301=DIRECTION('refdir',(1.,0.,0.));
#12302=DIRECTION('center_axis',(7.09974814698911E-30,-7.88860905221012E-30,
1.));
#12303=DIRECTION('ref_axis',(1.,-2.12941982799268E-29,-7.09343725974734E-30));
#12304=DIRECTION('center_axis',(-7.09974814698911E-30,7.88860905221012E-30,
-1.));
#12305=DIRECTION('ref_axis',(1.,-2.12959150172473E-29,-7.09974814698911E-30));
#12306=DIRECTION('center_axis',(7.09974814698911E-30,-7.88860905221012E-30,
1.));
#12307=DIRECTION('ref_axis',(-1.,2.12959150172473E-29,7.09974814698911E-30));
#12308=DIRECTION('center_axis',(7.09974814698911E-30,-7.88860905221012E-30,
1.));
#12309=DIRECTION('ref_axis',(1.,-2.12941982799268E-29,-7.09343725974734E-30));
#12310=DIRECTION('center_axis',(-7.09974814698911E-30,7.88860905221012E-30,
-1.));
#12311=DIRECTION('ref_axis',(1.,-2.12959150172473E-29,-7.09974814698911E-30));
#12312=DIRECTION('center_axis',(7.09974814698911E-30,-7.88860905221012E-30,
1.));
#12313=DIRECTION('ref_axis',(-1.,2.12959150172473E-29,7.09974814698911E-30));
#12314=DIRECTION('center_axis',(7.09974814698911E-30,-7.88860905221012E-30,
1.));
#12315=DIRECTION('ref_axis',(1.,-2.12941982799268E-29,-7.09343725974734E-30));
#12316=DIRECTION('center_axis',(-7.09974814698911E-30,7.88860905221012E-30,
-1.));
#12317=DIRECTION('ref_axis',(1.,-2.12959150172473E-29,-7.09974814698911E-30));
#12318=DIRECTION('center_axis',(7.09974814698911E-30,-7.88860905221012E-30,
1.));
#12319=DIRECTION('ref_axis',(-1.,2.12959150172473E-29,7.09974814698911E-30));
#12320=DIRECTION('center_axis',(7.09974814698911E-30,-7.88860905221012E-30,
1.));
#12321=DIRECTION('ref_axis',(1.,-2.12941982799268E-29,-7.09343725974734E-30));
#12322=DIRECTION('center_axis',(-7.09974814698911E-30,7.88860905221012E-30,
-1.));
#12323=DIRECTION('ref_axis',(1.,1.95399252334027E-14,-7.09974814698895E-30));
#12324=DIRECTION('center_axis',(7.09974814698911E-30,-7.88860905221012E-30,
1.));
#12325=DIRECTION('ref_axis',(-1.,-5.32907051820073E-15,7.09974814698906E-30));
#12326=DIRECTION('center_axis',(7.09974814698911E-30,-7.88860905221012E-30,
1.));
#12327=DIRECTION('ref_axis',(1.,-2.12941982799268E-29,-7.09343725974734E-30));
#12328=DIRECTION('center_axis',(-7.09974814698911E-30,7.88860905221012E-30,
-1.));
#12329=DIRECTION('ref_axis',(1.,2.1316282072803E-14,-7.09974814698894E-30));
#12330=DIRECTION('center_axis',(7.09974814698911E-30,-7.88860905221012E-30,
1.));
#12331=DIRECTION('ref_axis',(-1.,2.6645352591004E-15,7.09974814698913E-30));
#12332=DIRECTION('center_axis',(7.09974814698911E-30,-7.88860905221012E-30,
1.));
#12333=DIRECTION('ref_axis',(1.,-2.12941982799268E-29,-7.09343725974734E-30));
#12334=DIRECTION('center_axis',(-7.09974814698911E-30,7.88860905221012E-30,
-1.));
#12335=DIRECTION('ref_axis',(1.,-2.1316282072803E-14,-7.09974814698928E-30));
#12336=DIRECTION('center_axis',(7.09974814698911E-30,-7.88860905221012E-30,
1.));
#12337=DIRECTION('ref_axis',(-1.,1.77635683940027E-15,7.09974814698912E-30));
#12338=DIRECTION('center_axis',(7.09974814698911E-30,-7.88860905221012E-30,
1.));
#12339=DIRECTION('ref_axis',(1.,-2.12941982799268E-29,-7.09343725974734E-30));
#12340=DIRECTION('center_axis',(-7.09974814698911E-30,7.88860905221012E-30,
-1.));
#12341=DIRECTION('ref_axis',(1.,-2.12959150172473E-29,-7.09974814698911E-30));
#12342=DIRECTION('center_axis',(7.09974814698911E-30,-7.88860905221012E-30,
1.));
#12343=DIRECTION('ref_axis',(-1.,-2.66453525910035E-15,7.09974814698909E-30));
#12344=DIRECTION('center_axis',(7.09974814698911E-30,-7.88860905221012E-30,
1.));
#12345=DIRECTION('ref_axis',(1.,-2.12941982799268E-29,-7.09343725974734E-30));
#12346=DIRECTION('center_axis',(-7.09974814698911E-30,7.88860905221012E-30,
-1.));
#12347=DIRECTION('ref_axis',(1.,-2.12959150172473E-29,-7.09974814698911E-30));
#12348=DIRECTION('center_axis',(7.09974814698911E-30,-7.88860905221012E-30,
1.));
#12349=DIRECTION('ref_axis',(-1.,8.88178419700147E-16,7.09974814698911E-30));
#12350=DIRECTION('center_axis',(7.09974814698911E-30,-7.88860905221012E-30,
1.));
#12351=DIRECTION('ref_axis',(1.,-2.12941982799268E-29,-7.09343725974734E-30));
#12352=DIRECTION('center_axis',(-7.09974814698911E-30,7.88860905221012E-30,
-1.));
#12353=DIRECTION('ref_axis',(1.,-2.12959150172473E-29,-7.09974814698911E-30));
#12354=DIRECTION('center_axis',(7.09974814698911E-30,-7.88860905221012E-30,
1.));
#12355=DIRECTION('ref_axis',(-1.,2.12959150172473E-29,7.09974814698911E-30));
#12356=DIRECTION('center_axis',(7.09974814698911E-30,-7.88860905221012E-30,
1.));
#12357=DIRECTION('ref_axis',(1.,-2.12941982799268E-29,-7.09343725974734E-30));
#12358=DIRECTION('center_axis',(-7.09974814698911E-30,7.88860905221012E-30,
-1.));
#12359=DIRECTION('ref_axis',(1.,-2.12959150172473E-29,-7.09974814698911E-30));
#12360=DIRECTION('center_axis',(7.09974814698911E-30,-7.88860905221012E-30,
1.));
#12361=DIRECTION('ref_axis',(-1.,8.88178419700147E-16,7.09974814698911E-30));
#12362=DIRECTION('center_axis',(7.09974814698911E-30,-7.88860905221012E-30,
1.));
#12363=DIRECTION('ref_axis',(1.,-2.12941982799268E-29,-7.09343725974734E-30));
#12364=DIRECTION('center_axis',(-7.09974814698911E-30,7.88860905221012E-30,
-1.));
#12365=DIRECTION('ref_axis',(1.,-2.12959150172473E-29,-7.09974814698911E-30));
#12366=DIRECTION('center_axis',(7.09974814698911E-30,-7.88860905221012E-30,
1.));
#12367=DIRECTION('ref_axis',(-1.,2.12959150172473E-29,7.09974814698911E-30));
#12368=DIRECTION('center_axis',(7.09974814698911E-30,-7.88860905221012E-30,
1.));
#12369=DIRECTION('ref_axis',(1.,-2.12941982799268E-29,-7.09343725974734E-30));
#12370=DIRECTION('center_axis',(-7.09974814698911E-30,7.88860905221012E-30,
-1.));
#12371=DIRECTION('ref_axis',(1.,-2.12959150172473E-29,-7.09974814698911E-30));
#12372=DIRECTION('center_axis',(7.09974814698911E-30,-7.88860905221012E-30,
1.));
#12373=DIRECTION('ref_axis',(-1.,-8.5265128291212E-14,7.09974814698844E-30));
#12374=DIRECTION('center_axis',(7.09974814698911E-30,-7.88860905221012E-30,
1.));
#12375=DIRECTION('ref_axis',(1.,-2.12941982799268E-29,-7.09343725974734E-30));
#12376=DIRECTION('center_axis',(-7.09974814698911E-30,7.88860905221012E-30,
-1.));
#12377=DIRECTION('ref_axis',(1.,-2.12959150172473E-29,-7.09974814698911E-30));
#12378=DIRECTION('center_axis',(7.09974814698911E-30,-7.88860905221012E-30,
1.));
#12379=DIRECTION('ref_axis',(-1.,-1.77635683940025E-14,7.09974814698897E-30));
#12380=DIRECTION('center_axis',(7.09974814698911E-30,-7.88860905221012E-30,
1.));
#12381=DIRECTION('ref_axis',(1.,-2.12941982799268E-29,-7.09343725974734E-30));
#12382=DIRECTION('center_axis',(-7.09974814698911E-30,7.88860905221012E-30,
-1.));
#12383=DIRECTION('ref_axis',(1.,-2.12959150172473E-29,-7.09974814698911E-30));
#12384=DIRECTION('center_axis',(7.09974814698911E-30,-7.88860905221012E-30,
1.));
#12385=DIRECTION('ref_axis',(-1.,-4.17443857259059E-14,7.09974814698878E-30));
#12386=DIRECTION('center_axis',(7.09974814698911E-30,-7.88860905221012E-30,
1.));
#12387=DIRECTION('ref_axis',(1.,-2.12941982799268E-29,-7.09343725974734E-30));
#12388=DIRECTION('center_axis',(-7.09974814698911E-30,7.88860905221012E-30,
-1.));
#12389=DIRECTION('ref_axis',(1.,-2.12959150172473E-29,-7.09974814698911E-30));
#12390=DIRECTION('center_axis',(7.09974814698911E-30,-7.88860905221012E-30,
1.));
#12391=DIRECTION('ref_axis',(-1.,1.01252339845814E-13,7.0997481469899E-30));
#12392=DIRECTION('center_axis',(7.09974814698911E-30,-7.88860905221012E-30,
1.));
#12393=DIRECTION('ref_axis',(1.,-2.12941982799268E-29,-7.09343725974734E-30));
#12394=DIRECTION('center_axis',(-7.09974814698911E-30,7.88860905221012E-30,
-1.));
#12395=DIRECTION('ref_axis',(1.,-2.12959150172473E-29,-7.09974814698911E-30));
#12396=DIRECTION('center_axis',(7.09974814698911E-30,-7.88860905221012E-30,
1.));
#12397=DIRECTION('ref_axis',(-1.,-1.33226762955019E-14,7.099748146989E-30));
#12398=DIRECTION('center_axis',(7.09974814698911E-30,-7.88860905221012E-30,
1.));
#12399=DIRECTION('ref_axis',(1.,-2.12941982799268E-29,-7.09343725974734E-30));
#12400=DIRECTION('center_axis',(-7.09974814698911E-30,7.88860905221012E-30,
-1.));
#12401=DIRECTION('ref_axis',(1.,-2.12959150172473E-29,-7.09974814698911E-30));
#12402=DIRECTION('center_axis',(7.09974814698911E-30,-7.88860905221012E-30,
1.));
#12403=DIRECTION('ref_axis',(-1.,2.57571741713037E-14,7.09974814698931E-30));
#12404=DIRECTION('center_axis',(7.09974814698911E-30,-7.88860905221012E-30,
1.));
#12405=DIRECTION('ref_axis',(1.,-2.12941982799268E-29,-7.09343725974734E-30));
#12406=DIRECTION('center_axis',(-7.09974814698911E-30,7.88860905221012E-30,
-1.));
#12407=DIRECTION('ref_axis',(1.,-2.12959150172473E-29,-7.09974814698911E-30));
#12408=DIRECTION('center_axis',(7.09974814698911E-30,-7.88860905221012E-30,
1.));
#12409=DIRECTION('ref_axis',(-1.,3.73034936274053E-14,7.0997481469894E-30));
#12410=DIRECTION('center_axis',(7.09974814698911E-30,-7.88860905221012E-30,
1.));
#12411=DIRECTION('ref_axis',(1.,-2.12941982799268E-29,-7.09343725974734E-30));
#12412=DIRECTION('center_axis',(-7.09974814698911E-30,7.88860905221012E-30,
-1.));
#12413=DIRECTION('ref_axis',(1.,-2.12959150172473E-29,-7.09974814698911E-30));
#12414=DIRECTION('center_axis',(7.09974814698911E-30,-7.88860905221012E-30,
1.));
#12415=DIRECTION('ref_axis',(-1.,-2.48689957516035E-14,7.09974814698891E-30));
#12416=DIRECTION('center_axis',(7.09974814698911E-30,-7.88860905221012E-30,
1.));
#12417=DIRECTION('ref_axis',(1.,-2.12941982799268E-29,-7.09343725974734E-30));
#12418=DIRECTION('center_axis',(-7.09974814698911E-30,7.88860905221012E-30,
-1.));
#12419=DIRECTION('ref_axis',(1.,-2.12959150172473E-29,-7.09974814698911E-30));
#12420=DIRECTION('center_axis',(7.09974814698911E-30,-7.88860905221012E-30,
1.));
#12421=DIRECTION('ref_axis',(-1.,2.12959150172473E-29,7.09974814698911E-30));
#12422=DIRECTION('center_axis',(7.09974814698911E-30,-7.88860905221012E-30,
1.));
#12423=DIRECTION('ref_axis',(1.,-2.12941982799268E-29,-7.09343725974734E-30));
#12424=DIRECTION('center_axis',(-7.09974814698911E-30,7.88860905221012E-30,
-1.));
#12425=DIRECTION('ref_axis',(1.,6.3948846218409E-14,-7.0997481469886E-30));
#12426=DIRECTION('center_axis',(7.09974814698911E-30,-7.88860905221012E-30,
1.));
#12427=DIRECTION('ref_axis',(-1.,4.61852778244065E-14,7.09974814698947E-30));
#12428=DIRECTION('center_axis',(7.09974814698911E-30,-7.88860905221012E-30,
1.));
#12429=DIRECTION('ref_axis',(1.,-2.12941982799268E-29,-7.09343725974734E-30));
#12430=DIRECTION('center_axis',(-7.09974814698911E-30,7.88860905221012E-30,
-1.));
#12431=DIRECTION('ref_axis',(1.,2.1316282072803E-14,-7.09974814698894E-30));
#12432=DIRECTION('center_axis',(7.09974814698911E-30,-7.88860905221012E-30,
1.));
#12433=DIRECTION('ref_axis',(-1.,2.22044604925032E-14,7.09974814698928E-30));
#12434=DIRECTION('center_axis',(7.09974814698911E-30,-7.88860905221012E-30,
1.));
#12435=DIRECTION('ref_axis',(1.,-2.12941982799268E-29,-7.09343725974734E-30));
#12436=DIRECTION('center_axis',(-7.09974814698911E-30,7.88860905221012E-30,
-1.));
#12437=DIRECTION('ref_axis',(1.,2.22044604925031E-14,-7.09974814698893E-30));
#12438=DIRECTION('center_axis',(7.09974814698911E-30,-7.88860905221012E-30,
1.));
#12439=DIRECTION('ref_axis',(-1.,2.12959150172473E-29,7.09974814698911E-30));
#12440=DIRECTION('center_axis',(7.09974814698911E-30,-7.88860905221012E-30,
1.));
#12441=DIRECTION('ref_axis',(1.,-2.12941982799268E-29,-7.09343725974734E-30));
#12442=DIRECTION('center_axis',(-7.09974814698911E-30,7.88860905221012E-30,
-1.));
#12443=DIRECTION('ref_axis',(1.,-4.52970994047064E-14,-7.09974814698946E-30));
#12444=DIRECTION('center_axis',(7.09974814698911E-30,-7.88860905221012E-30,
1.));
#12445=DIRECTION('ref_axis',(-1.,2.12959150172473E-29,7.09974814698911E-30));
#12446=DIRECTION('center_axis',(7.09974814698911E-30,-7.88860905221012E-30,
1.));
#12447=DIRECTION('ref_axis',(1.,-2.12941982799268E-29,-7.09343725974734E-30));
#12448=DIRECTION('center_axis',(-7.09974814698911E-30,7.88860905221012E-30,
-1.));
#12449=DIRECTION('ref_axis',(1.,4.70734562441066E-14,-7.09974814698873E-30));
#12450=DIRECTION('center_axis',(7.09974814698911E-30,-7.88860905221012E-30,
1.));
#12451=DIRECTION('ref_axis',(-1.,4.08562073062058E-14,7.09974814698943E-30));
#12452=DIRECTION('center_axis',(7.09974814698911E-30,-7.88860905221012E-30,
1.));
#12453=DIRECTION('ref_axis',(1.,-2.12941982799268E-29,-7.09343725974734E-30));
#12454=DIRECTION('center_axis',(-7.09974814698911E-30,7.88860905221012E-30,
-1.));
#12455=DIRECTION('ref_axis',(1.,-4.88498130835069E-14,-7.09974814698949E-30));
#12456=DIRECTION('center_axis',(7.09974814698911E-30,-7.88860905221012E-30,
1.));
#12457=DIRECTION('ref_axis',(-1.,-3.90798504668055E-14,7.0997481469888E-30));
#12458=DIRECTION('center_axis',(7.09974814698911E-30,-7.88860905221012E-30,
1.));
#12459=DIRECTION('ref_axis',(1.,-2.12941982799268E-29,-7.09343725974734E-30));
#12460=DIRECTION('center_axis',(-7.09974814698911E-30,7.88860905221012E-30,
-1.));
#12461=DIRECTION('ref_axis',(1.,-2.12959150172473E-29,-7.09974814698911E-30));
#12462=DIRECTION('center_axis',(7.09974814698911E-30,-7.88860905221012E-30,
1.));
#12463=DIRECTION('ref_axis',(-1.,-7.63833440942108E-14,7.0997481469885E-30));
#12464=DIRECTION('center_axis',(7.09974814698911E-30,-7.88860905221012E-30,
1.));
#12465=DIRECTION('ref_axis',(1.,-2.12941982799268E-29,-7.09343725974734E-30));
#12466=DIRECTION('center_axis',(-7.09974814698911E-30,7.88860905221012E-30,
-1.));
#12467=DIRECTION('ref_axis',(1.,5.15143483426073E-14,-7.0997481469887E-30));
#12468=DIRECTION('center_axis',(7.09974814698911E-30,-7.88860905221012E-30,
1.));
#12469=DIRECTION('ref_axis',(-1.,2.12959150172473E-29,7.09974814698911E-30));
#12470=DIRECTION('center_axis',(7.09974814698911E-30,-7.88860905221012E-30,
1.));
#12471=DIRECTION('ref_axis',(1.,-2.12941982799268E-29,-7.09343725974734E-30));
#12472=DIRECTION('center_axis',(-7.09974814698911E-30,7.88860905221012E-30,
-1.));
#12473=DIRECTION('ref_axis',(1.,-7.90478793533112E-14,-7.09974814698973E-30));
#12474=DIRECTION('center_axis',(7.09974814698911E-30,-7.88860905221012E-30,
1.));
#12475=DIRECTION('ref_axis',(-1.,2.12959150172473E-29,7.09974814698911E-30));
#12476=DIRECTION('center_axis',(7.09974814698911E-30,-7.88860905221012E-30,
1.));
#12477=DIRECTION('ref_axis',(1.,-2.12941982799268E-29,-7.09343725974734E-30));
#12478=DIRECTION('center_axis',(-7.09974814698911E-30,7.88860905221012E-30,
-1.));
#12479=DIRECTION('ref_axis',(1.,4.70734562441066E-14,-7.09974814698873E-30));
#12480=DIRECTION('center_axis',(7.09974814698911E-30,-7.88860905221012E-30,
1.));
#12481=DIRECTION('ref_axis',(-1.,2.12959150172473E-29,7.09974814698911E-30));
#12482=DIRECTION('center_axis',(7.09974814698911E-30,-7.88860905221012E-30,
1.));
#12483=DIRECTION('ref_axis',(1.,-2.12941982799268E-29,-7.09343725974734E-30));
#12484=DIRECTION('center_axis',(-7.09974814698911E-30,7.88860905221012E-30,
-1.));
#12485=DIRECTION('ref_axis',(1.,-2.75335310107039E-14,-7.09974814698932E-30));
#12486=DIRECTION('center_axis',(7.09974814698911E-30,-7.88860905221012E-30,
1.));
#12487=DIRECTION('ref_axis',(-1.,3.28626015289047E-14,7.09974814698937E-30));
#12488=DIRECTION('center_axis',(7.09974814698911E-30,-7.88860905221012E-30,
1.));
#12489=DIRECTION('ref_axis',(1.,-2.12941982799268E-29,-7.09343725974734E-30));
#12490=DIRECTION('center_axis',(-7.09974814698911E-30,7.88860905221012E-30,
-1.));
#12491=DIRECTION('ref_axis',(1.,-1.4210854715202E-14,-7.09974814698922E-30));
#12492=DIRECTION('center_axis',(7.09974814698911E-30,-7.88860905221012E-30,
1.));
#12493=DIRECTION('ref_axis',(-1.,2.12959150172473E-29,7.09974814698911E-30));
#12494=DIRECTION('center_axis',(7.09974814698911E-30,-7.88860905221012E-30,
1.));
#12495=DIRECTION('ref_axis',(1.,-2.12941982799268E-29,-7.09343725974734E-30));
#12496=DIRECTION('center_axis',(-7.09974814698911E-30,7.88860905221012E-30,
-1.));
#12497=DIRECTION('ref_axis',(1.,-1.59872115546023E-14,-7.09974814698923E-30));
#12498=DIRECTION('center_axis',(7.09974814698911E-30,-7.88860905221012E-30,
1.));
#12499=DIRECTION('ref_axis',(-1.,2.12959150172473E-29,7.09974814698911E-30));
#12500=DIRECTION('center_axis',(7.09974814698911E-30,-7.88860905221012E-30,
1.));
#12501=DIRECTION('ref_axis',(1.,-2.12941982799268E-29,-7.09343725974734E-30));
#12502=DIRECTION('center_axis',(-7.09974814698911E-30,7.88860905221012E-30,
-1.));
#12503=DIRECTION('ref_axis',(1.,-2.12959150172473E-29,-7.09974814698911E-30));
#12504=DIRECTION('center_axis',(7.09974814698911E-30,-7.88860905221012E-30,
1.));
#12505=DIRECTION('ref_axis',(-1.,-2.8421709430404E-14,7.09974814698888E-30));
#12506=DIRECTION('center_axis',(7.09974814698911E-30,-7.88860905221012E-30,
1.));
#12507=DIRECTION('ref_axis',(1.,-2.12941982799268E-29,-7.09343725974734E-30));
#12508=DIRECTION('center_axis',(-7.09974814698911E-30,7.88860905221012E-30,
-1.));
#12509=DIRECTION('ref_axis',(1.,8.88178419700104E-16,-7.0997481469891E-30));
#12510=DIRECTION('center_axis',(7.09974814698911E-30,-7.88860905221012E-30,
1.));
#12511=DIRECTION('ref_axis',(-1.,2.75335310107039E-14,7.09974814698932E-30));
#12512=DIRECTION('center_axis',(7.09974814698911E-30,-7.88860905221012E-30,
1.));
#12513=DIRECTION('ref_axis',(1.,-2.12941982799268E-29,-7.09343725974734E-30));
#12514=DIRECTION('center_axis',(-7.09974814698911E-30,7.88860905221012E-30,
-1.));
#12515=DIRECTION('ref_axis',(1.,8.88178419700104E-16,-7.0997481469891E-30));
#12516=DIRECTION('center_axis',(7.09974814698911E-30,-7.88860905221012E-30,
1.));
#12517=DIRECTION('ref_axis',(-1.,2.12959150172473E-29,7.09974814698911E-30));
#12518=DIRECTION('center_axis',(7.09974814698911E-30,-7.88860905221012E-30,
1.));
#12519=DIRECTION('ref_axis',(1.,-2.12941982799268E-29,-7.09343725974734E-30));
#12520=DIRECTION('center_axis',(-7.09974814698911E-30,7.88860905221012E-30,
-1.));
#12521=DIRECTION('ref_axis',(1.,-8.88178419700147E-16,-7.09974814698911E-30));
#12522=DIRECTION('center_axis',(7.09974814698911E-30,-7.88860905221012E-30,
1.));
#12523=DIRECTION('ref_axis',(-1.,2.12959150172473E-29,7.09974814698911E-30));
#12524=DIRECTION('center_axis',(7.09974814698911E-30,-7.88860905221012E-30,
1.));
#12525=DIRECTION('ref_axis',(1.,-2.12941982799268E-29,-7.09343725974734E-30));
#12526=DIRECTION('center_axis',(-7.09974814698911E-30,7.88860905221012E-30,
-1.));
#12527=DIRECTION('ref_axis',(1.,-2.12959150172473E-29,-7.09974814698911E-30));
#12528=DIRECTION('center_axis',(7.09974814698911E-30,-7.88860905221012E-30,
1.));
#12529=DIRECTION('ref_axis',(-1.,2.12959150172473E-29,7.09974814698911E-30));
#12530=DIRECTION('center_axis',(7.09974814698911E-30,-7.88860905221012E-30,
1.));
#12531=DIRECTION('ref_axis',(1.,-2.12941982799268E-29,-7.09343725974734E-30));
#12532=DIRECTION('center_axis',(-7.09974814698911E-30,7.88860905221012E-30,
-1.));
#12533=DIRECTION('ref_axis',(1.,1.77635683940023E-15,-7.09974814698909E-30));
#12534=DIRECTION('center_axis',(7.09974814698911E-30,-7.88860905221012E-30,
1.));
#12535=DIRECTION('ref_axis',(-1.,2.12959150172473E-29,7.09974814698911E-30));
#12536=DIRECTION('center_axis',(7.09974814698911E-30,-7.88860905221012E-30,
1.));
#12537=DIRECTION('ref_axis',(1.,-2.12941982799268E-29,-7.09343725974734E-30));
#12538=DIRECTION('center_axis',(-7.09974814698911E-30,7.88860905221012E-30,
-1.));
#12539=DIRECTION('ref_axis',(1.,-2.12959150172473E-29,-7.09974814698911E-30));
#12540=DIRECTION('center_axis',(7.09974814698911E-30,-7.88860905221012E-30,
1.));
#12541=DIRECTION('ref_axis',(-1.,-2.04281036531029E-14,7.09974814698895E-30));
#12542=DIRECTION('center_axis',(7.09974814698911E-30,-7.88860905221012E-30,
1.));
#12543=DIRECTION('ref_axis',(1.,-2.12941982799268E-29,-7.09343725974734E-30));
#12544=DIRECTION('center_axis',(-7.09974814698911E-30,7.88860905221012E-30,
-1.));
#12545=DIRECTION('ref_axis',(1.,-2.12959150172473E-29,-7.09974814698911E-30));
#12546=DIRECTION('center_axis',(7.09974814698911E-30,-7.88860905221012E-30,
1.));
#12547=DIRECTION('ref_axis',(-1.,2.12959150172473E-29,7.09974814698911E-30));
#12548=DIRECTION('center_axis',(7.09974814698911E-30,-7.88860905221012E-30,
1.));
#12549=DIRECTION('ref_axis',(1.,-2.12941982799268E-29,-7.09343725974734E-30));
#12550=DIRECTION('center_axis',(-7.09974814698911E-30,7.88860905221012E-30,
-1.));
#12551=DIRECTION('ref_axis',(1.,-2.12959150172473E-29,-7.09974814698911E-30));
#12552=DIRECTION('center_axis',(7.09974814698911E-30,-7.88860905221012E-30,
1.));
#12553=DIRECTION('ref_axis',(-1.,8.88178419700128E-15,7.09974814698918E-30));
#12554=DIRECTION('center_axis',(7.09974814698911E-30,-7.88860905221012E-30,
1.));
#12555=DIRECTION('ref_axis',(1.,-2.12941982799268E-29,-7.09343725974734E-30));
#12556=DIRECTION('center_axis',(-7.09974814698911E-30,7.88860905221012E-30,
-1.));
#12557=DIRECTION('ref_axis',(1.,-2.12959150172473E-29,-7.09974814698911E-30));
#12558=DIRECTION('center_axis',(7.09974814698911E-30,-7.88860905221012E-30,
1.));
#12559=DIRECTION('ref_axis',(-1.,2.12959150172473E-29,7.09974814698911E-30));
#12560=DIRECTION('center_axis',(7.09974814698911E-30,-7.88860905221012E-30,
1.));
#12561=DIRECTION('ref_axis',(1.,-2.12941982799268E-29,-7.09343725974734E-30));
#12562=DIRECTION('center_axis',(-7.09974814698911E-30,7.88860905221012E-30,
-1.));
#12563=DIRECTION('ref_axis',(1.,-2.12959150172473E-29,-7.09974814698911E-30));
#12564=DIRECTION('center_axis',(7.09974814698911E-30,-7.88860905221012E-30,
1.));
#12565=DIRECTION('ref_axis',(-1.,2.12959150172473E-29,7.09974814698911E-30));
#12566=DIRECTION('center_axis',(-7.09974814698911E-30,7.88860905221012E-30,
-1.));
#12567=DIRECTION('ref_axis',(-1.,2.1291967674334E-29,7.09974814698911E-30));
#12568=DIRECTION('center_axis',(-7.09974814698911E-30,7.88860905221012E-30,
-1.));
#12569=DIRECTION('ref_axis',(1.,-2.12941982799268E-29,-7.09974814698911E-30));
#12570=DIRECTION('center_axis',(-7.09974814698911E-30,7.88860905221012E-30,
-1.));
#12571=DIRECTION('ref_axis',(1.,-2.12941982799268E-29,-7.09974814698911E-30));
#12572=DIRECTION('center_axis',(-7.09974814698911E-30,7.88860905221012E-30,
-1.));
#12573=DIRECTION('ref_axis',(1.,-2.12941982799268E-29,-7.09974814698911E-30));
#12574=DIRECTION('center_axis',(-7.09974814698911E-30,7.88860905221012E-30,
-1.));
#12575=DIRECTION('ref_axis',(1.,-2.12941982799268E-29,-7.09974814698911E-30));
#12576=DIRECTION('center_axis',(-7.09974814698911E-30,7.88860905221012E-30,
-1.));
#12577=DIRECTION('ref_axis',(1.,-1.4210854715202E-14,-7.09974814698922E-30));
#12578=DIRECTION('center_axis',(-7.09974814698911E-30,7.88860905221012E-30,
-1.));
#12579=DIRECTION('ref_axis',(1.,1.4210854715202E-14,-7.09974814698899E-30));
#12580=DIRECTION('center_axis',(-7.09974814698911E-30,7.88860905221012E-30,
-1.));
#12581=DIRECTION('ref_axis',(1.,-2.12941982799268E-29,-7.09974814698911E-30));
#12582=DIRECTION('center_axis',(-7.09974814698911E-30,7.88860905221012E-30,
-1.));
#12583=DIRECTION('ref_axis',(1.,-1.24344978758018E-14,-7.0997481469892E-30));
#12584=DIRECTION('center_axis',(-7.09974814698911E-30,7.88860905221012E-30,
-1.));
#12585=DIRECTION('ref_axis',(1.,-2.12941982799268E-29,-7.09974814698911E-30));
#12586=DIRECTION('center_axis',(-7.09974814698911E-30,7.88860905221012E-30,
-1.));
#12587=DIRECTION('ref_axis',(1.,-2.12941982799268E-29,-7.09974814698911E-30));
#12588=DIRECTION('center_axis',(-7.09974814698911E-30,7.88860905221012E-30,
-1.));
#12589=DIRECTION('ref_axis',(1.,-2.12941982799268E-29,-7.09974814698911E-30));
#12590=DIRECTION('center_axis',(-7.09974814698911E-30,7.88860905221012E-30,
-1.));
#12591=DIRECTION('ref_axis',(1.,-2.12941982799268E-29,-7.09974814698911E-30));
#12592=DIRECTION('center_axis',(-7.09974814698911E-30,7.88860905221012E-30,
-1.));
#12593=DIRECTION('ref_axis',(1.,-2.12941982799268E-29,-7.09974814698911E-30));
#12594=DIRECTION('center_axis',(-7.09974814698911E-30,7.88860905221012E-30,
-1.));
#12595=DIRECTION('ref_axis',(1.,-2.12941982799268E-29,-7.09974814698911E-30));
#12596=DIRECTION('center_axis',(-7.09974814698911E-30,7.88860905221012E-30,
-1.));
#12597=DIRECTION('ref_axis',(1.,-2.12941982799268E-29,-7.09974814698911E-30));
#12598=DIRECTION('center_axis',(-7.09974814698911E-30,7.88860905221012E-30,
-1.));
#12599=DIRECTION('ref_axis',(1.,-2.6645352591004E-15,-7.09974814698913E-30));
#12600=DIRECTION('center_axis',(-7.09974814698911E-30,7.88860905221012E-30,
-1.));
#12601=DIRECTION('ref_axis',(1.,-2.12941982799268E-29,-7.09974814698911E-30));
#12602=DIRECTION('center_axis',(-7.09974814698911E-30,7.88860905221012E-30,
-1.));
#12603=DIRECTION('ref_axis',(1.,-2.12941982799268E-29,-7.09974814698911E-30));
#12604=DIRECTION('center_axis',(-7.09974814698911E-30,7.88860905221012E-30,
-1.));
#12605=DIRECTION('ref_axis',(1.,-8.88178419700147E-16,-7.09974814698911E-30));
#12606=DIRECTION('center_axis',(-7.09974814698911E-30,7.88860905221012E-30,
-1.));
#12607=DIRECTION('ref_axis',(1.,-2.12941982799268E-29,-7.09974814698911E-30));
#12608=DIRECTION('center_axis',(-7.09974814698911E-30,7.88860905221012E-30,
-1.));
#12609=DIRECTION('ref_axis',(1.,-2.12941982799268E-29,-7.09974814698911E-30));
#12610=DIRECTION('center_axis',(-7.09974814698911E-30,7.88860905221012E-30,
-1.));
#12611=DIRECTION('ref_axis',(1.,-2.12941982799268E-29,-7.09974814698911E-30));
#12612=DIRECTION('',(-0.707106781186543,8.65956056235582E-17,0.707106781186552));
#12613=DIRECTION('center_axis',(7.09974814698911E-30,-7.88860905221012E-30,
1.));
#12614=DIRECTION('ref_axis',(1.,-2.1291967674334E-29,-7.09974814698911E-30));
#12615=DIRECTION('center_axis',(-7.09974814698911E-30,7.88860905221012E-30,
-1.));
#12616=DIRECTION('ref_axis',(1.,-4.44089209850065E-15,-7.09974814698914E-30));
#12617=DIRECTION('center_axis',(-7.09974814698911E-30,7.88860905221012E-30,
-1.));
#12618=DIRECTION('ref_axis',(1.,1.59872115546022E-14,-7.09974814698898E-30));
#12619=DIRECTION('center_axis',(-7.09974814698911E-30,7.88860905221012E-30,
-1.));
#12620=DIRECTION('ref_axis',(1.,-5.15143483426073E-14,-7.09974814698951E-30));
#12621=DIRECTION('center_axis',(-7.09974814698911E-30,7.88860905221012E-30,
-1.));
#12622=DIRECTION('ref_axis',(1.,-8.88178419700147E-16,-7.09974814698911E-30));
#12623=DIRECTION('center_axis',(-7.09974814698911E-30,7.88860905221012E-30,
-1.));
#12624=DIRECTION('ref_axis',(1.,5.6843418860808E-14,-7.09974814698866E-30));
#12625=DIRECTION('center_axis',(-7.09974814698911E-30,7.88860905221012E-30,
-1.));
#12626=DIRECTION('ref_axis',(1.,3.19744231092045E-14,-7.09974814698885E-30));
#12627=DIRECTION('center_axis',(-7.09974814698911E-30,7.88860905221012E-30,
-1.));
#12628=DIRECTION('ref_axis',(1.,-2.12941982799268E-29,-7.09974814698911E-30));
#12629=DIRECTION('center_axis',(-7.09974814698911E-30,7.88860905221012E-30,
-1.));
#12630=DIRECTION('ref_axis',(1.,4.61852778244065E-14,-7.09974814698874E-30));
#12631=DIRECTION('center_axis',(-7.09974814698911E-30,7.88860905221012E-30,
-1.));
#12632=DIRECTION('ref_axis',(1.,4.44089209850063E-14,-7.09974814698876E-30));
#12633=DIRECTION('center_axis',(-7.09974814698911E-30,7.88860905221012E-30,
-1.));
#12634=DIRECTION('ref_axis',(1.,4.2632564145606E-14,-7.09974814698877E-30));
#12635=DIRECTION('center_axis',(-7.09974814698911E-30,7.88860905221012E-30,
-1.));
#12636=DIRECTION('ref_axis',(1.,2.75335310107039E-14,-7.09974814698889E-30));
#12637=DIRECTION('center_axis',(-7.09974814698911E-30,7.88860905221012E-30,
-1.));
#12638=DIRECTION('ref_axis',(1.,-5.50670620214078E-14,-7.09974814698954E-30));
#12639=DIRECTION('center_axis',(-7.09974814698911E-30,7.88860905221012E-30,
-1.));
#12640=DIRECTION('ref_axis',(1.,2.57571741713036E-14,-7.0997481469889E-30));
#12641=DIRECTION('center_axis',(-7.09974814698911E-30,7.88860905221012E-30,
-1.));
#12642=DIRECTION('ref_axis',(1.,1.24344978758017E-14,-7.09974814698901E-30));
#12643=DIRECTION('center_axis',(-7.09974814698911E-30,7.88860905221012E-30,
-1.));
#12644=DIRECTION('ref_axis',(1.,-2.48689957516035E-14,-7.0997481469893E-30));
#12645=DIRECTION('center_axis',(-7.09974814698911E-30,7.88860905221012E-30,
-1.));
#12646=DIRECTION('ref_axis',(1.,-2.48689957516035E-14,-7.0997481469893E-30));
#12647=DIRECTION('center_axis',(-7.09974814698911E-30,7.88860905221012E-30,
-1.));
#12648=DIRECTION('ref_axis',(1.,-2.12941982799268E-29,-7.09974814698911E-30));
#12649=DIRECTION('center_axis',(-7.09974814698911E-30,7.88860905221012E-30,
-1.));
#12650=DIRECTION('ref_axis',(1.,-2.12941982799268E-29,-7.09974814698911E-30));
#12651=DIRECTION('center_axis',(-7.09974814698911E-30,7.88860905221012E-30,
-1.));
#12652=DIRECTION('ref_axis',(1.,-2.12941982799268E-29,-7.09974814698911E-30));
#12653=DIRECTION('center_axis',(-7.09974814698911E-30,7.88860905221012E-30,
-1.));
#12654=DIRECTION('ref_axis',(1.,-2.12941982799268E-29,-7.09974814698911E-30));
#12655=DIRECTION('center_axis',(-7.09974814698911E-30,7.88860905221012E-30,
-1.));
#12656=DIRECTION('ref_axis',(1.,-2.12941982799268E-29,-7.09974814698911E-30));
#12657=DIRECTION('center_axis',(-7.09974814698911E-30,7.88860905221012E-30,
-1.));
#12658=DIRECTION('ref_axis',(1.,-2.12941982799268E-29,-7.09974814698911E-30));
#12659=DIRECTION('center_axis',(-7.09974814698911E-30,7.88860905221012E-30,
-1.));
#12660=DIRECTION('ref_axis',(1.83697019872082E-16,-1.,-7.88860905221012E-30));
#12661=DIRECTION('center_axis',(7.09974814698911E-30,-7.88860905221012E-30,
1.));
#12662=DIRECTION('ref_axis',(1.,-2.12879456519602E-29,-7.09974814698911E-30));
#12663=DIRECTION('',(-7.09974814698911E-30,7.88860905221012E-30,-1.));
#12664=DIRECTION('center_axis',(7.09974814698911E-30,-7.88860905221012E-30,
1.));
#12665=DIRECTION('ref_axis',(1.,-2.12879456519602E-29,-7.09974814698911E-30));
#12666=DIRECTION('',(-7.09974814698911E-30,7.88860905221012E-30,-1.));
#12667=DIRECTION('center_axis',(7.09974814698911E-30,-7.88860905221012E-30,
1.));
#12668=DIRECTION('ref_axis',(1.,-2.12959150172473E-29,-7.0997481469891E-30));
#12669=DIRECTION('center_axis',(7.09974814698911E-30,-7.88860905221012E-30,
1.));
#12670=DIRECTION('ref_axis',(1.,-2.12959150172473E-29,-7.0997481469891E-30));
#12671=DIRECTION('center_axis',(7.09974814698911E-30,-7.88860905221012E-30,
1.));
#12672=DIRECTION('ref_axis',(1.,-2.12959150172473E-29,-7.0997481469891E-30));
#12673=DIRECTION('center_axis',(7.09974814698911E-30,-7.88860905221012E-30,
1.));
#12674=DIRECTION('ref_axis',(1.,-2.12959150172473E-29,-7.0997481469891E-30));
#12675=DIRECTION('center_axis',(7.09974814698911E-30,-7.88860905221012E-30,
1.));
#12676=DIRECTION('ref_axis',(1.,-2.12959150172473E-29,-7.0997481469891E-30));
#12677=DIRECTION('center_axis',(7.09974814698911E-30,-7.88860905221012E-30,
1.));
#12678=DIRECTION('ref_axis',(1.,-2.12959150172473E-29,-7.0997481469891E-30));
#12679=DIRECTION('center_axis',(7.09974814698911E-30,-7.88860905221012E-30,
1.));
#12680=DIRECTION('ref_axis',(1.,-2.12959150172473E-29,-7.0997481469891E-30));
#12681=DIRECTION('center_axis',(7.09974814698911E-30,-7.88860905221012E-30,
1.));
#12682=DIRECTION('ref_axis',(1.,-2.12959150172473E-29,-7.0997481469891E-30));
#12683=DIRECTION('center_axis',(7.09974814698911E-30,-7.88860905221012E-30,
1.));
#12684=DIRECTION('ref_axis',(1.,-2.12959150172473E-29,-7.0997481469891E-30));
#12685=DIRECTION('center_axis',(7.09974814698911E-30,-7.88860905221012E-30,
1.));
#12686=DIRECTION('ref_axis',(1.,-2.12959150172473E-29,-7.0997481469891E-30));
#12687=DIRECTION('center_axis',(7.09974814698911E-30,-7.88860905221012E-30,
1.));
#12688=DIRECTION('ref_axis',(1.,-2.12959150172473E-29,-7.0997481469891E-30));
#12689=DIRECTION('center_axis',(7.09974814698911E-30,-7.88860905221012E-30,
1.));
#12690=DIRECTION('ref_axis',(1.,-2.12959150172473E-29,-7.0997481469891E-30));
#12691=DIRECTION('center_axis',(7.09974814698911E-30,-7.88860905221012E-30,
1.));
#12692=DIRECTION('ref_axis',(1.,-2.12959150172473E-29,-7.0997481469891E-30));
#12693=DIRECTION('center_axis',(7.09974814698911E-30,-7.88860905221012E-30,
1.));
#12694=DIRECTION('ref_axis',(1.,-2.12959150172473E-29,-7.0997481469891E-30));
#12695=DIRECTION('center_axis',(7.09974814698911E-30,-7.88860905221012E-30,
1.));
#12696=DIRECTION('ref_axis',(1.,-2.12959150172473E-29,-7.0997481469891E-30));
#12697=DIRECTION('center_axis',(7.09974814698911E-30,-7.88860905221012E-30,
1.));
#12698=DIRECTION('ref_axis',(1.,-2.12959150172473E-29,-7.0997481469891E-30));
#12699=DIRECTION('center_axis',(7.09974814698911E-30,-7.88860905221012E-30,
1.));
#12700=DIRECTION('ref_axis',(1.,-2.12959150172473E-29,-7.0997481469891E-30));
#12701=DIRECTION('center_axis',(7.09974814698911E-30,-7.88860905221012E-30,
1.));
#12702=DIRECTION('ref_axis',(1.,-2.12959150172473E-29,-7.0997481469891E-30));
#12703=DIRECTION('center_axis',(7.09974814698911E-30,-7.88860905221012E-30,
1.));
#12704=DIRECTION('ref_axis',(1.,-2.12959150172473E-29,-7.0997481469891E-30));
#12705=DIRECTION('center_axis',(7.09974814698911E-30,-7.88860905221012E-30,
1.));
#12706=DIRECTION('ref_axis',(1.,-2.12959150172473E-29,-7.0997481469891E-30));
#12707=DIRECTION('center_axis',(7.09974814698911E-30,-7.88860905221012E-30,
1.));
#12708=DIRECTION('ref_axis',(1.,-2.12959150172473E-29,-7.0997481469891E-30));
#12709=DIRECTION('center_axis',(7.09974814698911E-30,-7.88860905221012E-30,
1.));
#12710=DIRECTION('ref_axis',(1.,-2.12959150172473E-29,-7.0997481469891E-30));
#12711=DIRECTION('center_axis',(7.09974814698911E-30,-7.88860905221012E-30,
1.));
#12712=DIRECTION('ref_axis',(1.,-2.12959150172473E-29,-7.0997481469891E-30));
#12713=DIRECTION('',(0.707106781186549,8.659560562354E-17,-0.707106781186546));
#12714=DIRECTION('center_axis',(-7.09974814698911E-30,7.88860905221012E-30,
-1.));
#12715=DIRECTION('ref_axis',(1.,-2.12919676743341E-29,-7.09974814698911E-30));
#12716=DIRECTION('center_axis',(7.09974814698911E-30,-7.88860905221012E-30,
1.));
#12717=DIRECTION('ref_axis',(1.,-2.12959150172473E-29,-7.0997481469891E-30));
#12718=DIRECTION('center_axis',(7.09974814698911E-30,-7.88860905221012E-30,
1.));
#12719=DIRECTION('ref_axis',(1.,-2.12959150172473E-29,-7.0997481469891E-30));
#12720=DIRECTION('center_axis',(7.09974814698911E-30,-7.88860905221012E-30,
1.));
#12721=DIRECTION('ref_axis',(1.,-2.12959150172473E-29,-7.0997481469891E-30));
#12722=DIRECTION('center_axis',(7.09974814698911E-30,-7.88860905221012E-30,
1.));
#12723=DIRECTION('ref_axis',(1.,-2.12959150172473E-29,-7.0997481469891E-30));
#12724=DIRECTION('center_axis',(7.09974814698911E-30,-7.88860905221012E-30,
1.));
#12725=DIRECTION('ref_axis',(1.,-2.12959150172473E-29,-7.0997481469891E-30));
#12726=DIRECTION('center_axis',(7.09974814698911E-30,-7.88860905221012E-30,
1.));
#12727=DIRECTION('ref_axis',(1.,-2.12959150172473E-29,-7.0997481469891E-30));
#12728=DIRECTION('center_axis',(7.09974814698911E-30,-7.88860905221012E-30,
1.));
#12729=DIRECTION('ref_axis',(1.,-2.12959150172473E-29,-7.0997481469891E-30));
#12730=DIRECTION('center_axis',(7.09974814698911E-30,-7.88860905221012E-30,
1.));
#12731=DIRECTION('ref_axis',(1.,-2.12959150172473E-29,-7.0997481469891E-30));
#12732=DIRECTION('center_axis',(7.09974814698911E-30,-7.88860905221012E-30,
1.));
#12733=DIRECTION('ref_axis',(1.,-2.12959150172473E-29,-7.0997481469891E-30));
#12734=DIRECTION('center_axis',(7.09974814698911E-30,-7.88860905221012E-30,
1.));
#12735=DIRECTION('ref_axis',(1.,-2.12959150172473E-29,-7.0997481469891E-30));
#12736=DIRECTION('center_axis',(7.09974814698911E-30,-7.88860905221012E-30,
1.));
#12737=DIRECTION('ref_axis',(1.,-2.12959150172473E-29,-7.0997481469891E-30));
#12738=DIRECTION('center_axis',(7.09974814698911E-30,-7.88860905221012E-30,
1.));
#12739=DIRECTION('ref_axis',(1.,-2.12959150172473E-29,-7.0997481469891E-30));
#12740=DIRECTION('center_axis',(7.09974814698911E-30,-7.88860905221012E-30,
1.));
#12741=DIRECTION('ref_axis',(1.,-2.12959150172473E-29,-7.0997481469891E-30));
#12742=DIRECTION('center_axis',(7.09974814698911E-30,-7.88860905221012E-30,
1.));
#12743=DIRECTION('ref_axis',(1.,-2.12959150172473E-29,-7.0997481469891E-30));
#12744=DIRECTION('center_axis',(7.09974814698911E-30,-7.88860905221012E-30,
1.));
#12745=DIRECTION('ref_axis',(1.,-2.12959150172473E-29,-7.0997481469891E-30));
#12746=DIRECTION('center_axis',(7.09974814698911E-30,-7.88860905221012E-30,
1.));
#12747=DIRECTION('ref_axis',(1.,-2.12959150172473E-29,-7.0997481469891E-30));
#12748=DIRECTION('center_axis',(7.09974814698911E-30,-7.88860905221012E-30,
1.));
#12749=DIRECTION('ref_axis',(1.,-2.12959150172473E-29,-7.0997481469891E-30));
#12750=DIRECTION('center_axis',(7.09974814698911E-30,-7.88860905221012E-30,
1.));
#12751=DIRECTION('ref_axis',(1.,-2.12959150172473E-29,-7.0997481469891E-30));
#12752=DIRECTION('center_axis',(7.09974814698911E-30,-7.88860905221012E-30,
1.));
#12753=DIRECTION('ref_axis',(1.,-2.12959150172473E-29,-7.0997481469891E-30));
#12754=DIRECTION('center_axis',(7.09974814698911E-30,-7.88860905221012E-30,
1.));
#12755=DIRECTION('ref_axis',(1.,-2.12959150172473E-29,-7.0997481469891E-30));
#12756=DIRECTION('center_axis',(7.09974814698911E-30,-7.88860905221012E-30,
1.));
#12757=DIRECTION('ref_axis',(1.,-2.12959150172473E-29,-7.0997481469891E-30));
#12758=DIRECTION('center_axis',(7.09974814698911E-30,-7.88860905221012E-30,
1.));
#12759=DIRECTION('ref_axis',(1.,-2.12959150172473E-29,-7.0997481469891E-30));
#12760=DIRECTION('center_axis',(-7.09974814698911E-30,7.88860905221012E-30,
-1.));
#12761=DIRECTION('ref_axis',(-1.,2.12959150172473E-29,7.09974814698911E-30));
#12762=DIRECTION('center_axis',(-7.09974814698911E-30,7.88860905221012E-30,
-1.));
#12763=DIRECTION('ref_axis',(-1.,2.12959150172473E-29,7.09974814698911E-30));
#12764=DIRECTION('center_axis',(-7.09974814698911E-30,7.88860905221012E-30,
-1.));
#12765=DIRECTION('ref_axis',(-1.,2.12959150172473E-29,7.09974814698911E-30));
#12766=DIRECTION('center_axis',(-7.09974814698911E-30,7.88860905221012E-30,
-1.));
#12767=DIRECTION('ref_axis',(-1.,2.12959150172473E-29,7.09974814698911E-30));
#12768=DIRECTION('center_axis',(-7.09974814698911E-30,7.88860905221012E-30,
-1.));
#12769=DIRECTION('ref_axis',(-1.,2.12959150172473E-29,7.09974814698911E-30));
#12770=DIRECTION('center_axis',(-7.09974814698911E-30,7.88860905221012E-30,
-1.));
#12771=DIRECTION('ref_axis',(-1.,2.12959150172473E-29,7.09974814698911E-30));
#12772=DIRECTION('center_axis',(-7.09974814698911E-30,7.88860905221012E-30,
-1.));
#12773=DIRECTION('ref_axis',(-1.,2.12959150172473E-29,7.09974814698911E-30));
#12774=DIRECTION('center_axis',(-7.09974814698911E-30,7.88860905221012E-30,
-1.));
#12775=DIRECTION('ref_axis',(-1.,2.12959150172473E-29,7.09974814698911E-30));
#12776=DIRECTION('center_axis',(-7.09974814698911E-30,7.88860905221012E-30,
-1.));
#12777=DIRECTION('ref_axis',(-1.,2.12959150172473E-29,7.09974814698911E-30));
#12778=DIRECTION('center_axis',(-7.09974814698911E-30,7.88860905221012E-30,
-1.));
#12779=DIRECTION('ref_axis',(-1.,2.12959150172473E-29,7.09974814698911E-30));
#12780=DIRECTION('center_axis',(-7.09974814698911E-30,7.88860905221012E-30,
-1.));
#12781=DIRECTION('ref_axis',(-1.,2.12959150172473E-29,7.09974814698911E-30));
#12782=DIRECTION('center_axis',(-7.09974814698911E-30,7.88860905221012E-30,
-1.));
#12783=DIRECTION('ref_axis',(-1.,2.12959150172473E-29,7.09974814698911E-30));
#12784=DIRECTION('center_axis',(-7.09974814698911E-30,7.88860905221012E-30,
-1.));
#12785=DIRECTION('ref_axis',(-1.,2.12959150172473E-29,7.09974814698911E-30));
#12786=DIRECTION('center_axis',(-7.09974814698911E-30,7.88860905221012E-30,
-1.));
#12787=DIRECTION('ref_axis',(-1.,2.12959150172473E-29,7.09974814698911E-30));
#12788=DIRECTION('center_axis',(-7.09974814698911E-30,7.88860905221012E-30,
-1.));
#12789=DIRECTION('ref_axis',(-1.,2.12959150172473E-29,7.09974814698911E-30));
#12790=DIRECTION('center_axis',(-7.09974814698911E-30,7.88860905221012E-30,
-1.));
#12791=DIRECTION('ref_axis',(-1.,2.12959150172473E-29,7.09974814698911E-30));
#12792=DIRECTION('center_axis',(-7.09974814698911E-30,7.88860905221012E-30,
-1.));
#12793=DIRECTION('ref_axis',(-1.,2.12959150172473E-29,7.09974814698911E-30));
#12794=DIRECTION('center_axis',(-7.09974814698911E-30,7.88860905221012E-30,
-1.));
#12795=DIRECTION('ref_axis',(-1.,2.12959150172473E-29,7.09974814698911E-30));
#12796=DIRECTION('center_axis',(-7.09974814698911E-30,7.88860905221012E-30,
-1.));
#12797=DIRECTION('ref_axis',(-1.,2.12959150172473E-29,7.09974814698911E-30));
#12798=DIRECTION('center_axis',(-7.09974814698911E-30,7.88860905221012E-30,
-1.));
#12799=DIRECTION('ref_axis',(-1.,2.12959150172473E-29,7.09974814698911E-30));
#12800=DIRECTION('center_axis',(-7.09974814698911E-30,7.88860905221012E-30,
-1.));
#12801=DIRECTION('ref_axis',(-1.,2.12959150172473E-29,7.09974814698911E-30));
#12802=DIRECTION('center_axis',(-7.09974814698911E-30,7.88860905221012E-30,
-1.));
#12803=DIRECTION('ref_axis',(-1.,2.12959150172473E-29,7.09974814698911E-30));
#12804=DIRECTION('center_axis',(-7.09974814698911E-30,7.88860905221012E-30,
-1.));
#12805=DIRECTION('ref_axis',(-1.,2.12959150172473E-29,7.09974814698911E-30));
#12806=DIRECTION('center_axis',(-7.09974814698911E-30,7.88860905221012E-30,
-1.));
#12807=DIRECTION('ref_axis',(-1.,2.12959150172473E-29,7.09974814698911E-30));
#12808=DIRECTION('center_axis',(-7.09974814698911E-30,7.88860905221012E-30,
-1.));
#12809=DIRECTION('ref_axis',(-1.,2.12959150172473E-29,7.09974814698911E-30));
#12810=DIRECTION('center_axis',(-7.09974814698911E-30,7.88860905221012E-30,
-1.));
#12811=DIRECTION('ref_axis',(-1.,2.12959150172473E-29,7.09974814698911E-30));
#12812=DIRECTION('center_axis',(-7.09974814698911E-30,7.88860905221012E-30,
-1.));
#12813=DIRECTION('ref_axis',(-1.,2.12959150172473E-29,7.09974814698911E-30));
#12814=DIRECTION('center_axis',(-7.09974814698911E-30,7.88860905221012E-30,
-1.));
#12815=DIRECTION('ref_axis',(-1.,2.12959150172473E-29,7.09974814698911E-30));
#12816=DIRECTION('center_axis',(-7.09974814698911E-30,7.88860905221012E-30,
-1.));
#12817=DIRECTION('ref_axis',(-1.,2.12959150172473E-29,7.09974814698911E-30));
#12818=DIRECTION('center_axis',(-7.09974814698911E-30,7.88860905221012E-30,
-1.));
#12819=DIRECTION('ref_axis',(-1.,2.12959150172473E-29,7.09974814698911E-30));
#12820=DIRECTION('center_axis',(-7.09974814698911E-30,7.88860905221012E-30,
-1.));
#12821=DIRECTION('ref_axis',(-1.,2.12959150172473E-29,7.09974814698911E-30));
#12822=DIRECTION('center_axis',(-7.09974814698911E-30,7.88860905221012E-30,
-1.));
#12823=DIRECTION('ref_axis',(-1.,2.12959150172473E-29,7.09974814698911E-30));
#12824=DIRECTION('center_axis',(-7.09974814698911E-30,7.88860905221012E-30,
-1.));
#12825=DIRECTION('ref_axis',(-1.,2.12959150172473E-29,7.09974814698911E-30));
#12826=DIRECTION('center_axis',(-7.09974814698911E-30,7.88860905221012E-30,
-1.));
#12827=DIRECTION('ref_axis',(-1.,2.12959150172473E-29,7.09974814698911E-30));
#12828=DIRECTION('center_axis',(-7.09974814698911E-30,7.88860905221012E-30,
-1.));
#12829=DIRECTION('ref_axis',(-1.,2.12959150172473E-29,7.09974814698911E-30));
#12830=DIRECTION('center_axis',(-7.09974814698911E-30,7.88860905221012E-30,
-1.));
#12831=DIRECTION('ref_axis',(-1.,2.12959150172473E-29,7.09974814698911E-30));
#12832=DIRECTION('center_axis',(-7.09974814698911E-30,7.88860905221012E-30,
-1.));
#12833=DIRECTION('ref_axis',(-1.,2.12959150172473E-29,7.09974814698911E-30));
#12834=DIRECTION('center_axis',(-7.09974814698911E-30,7.88860905221012E-30,
-1.));
#12835=DIRECTION('ref_axis',(-1.,2.12959150172473E-29,7.09974814698911E-30));
#12836=DIRECTION('center_axis',(-7.09974814698911E-30,7.88860905221012E-30,
-1.));
#12837=DIRECTION('ref_axis',(-1.,2.12959150172473E-29,7.09974814698911E-30));
#12838=DIRECTION('center_axis',(-7.09974814698911E-30,7.88860905221012E-30,
-1.));
#12839=DIRECTION('ref_axis',(-1.,2.12959150172473E-29,7.09974814698911E-30));
#12840=DIRECTION('center_axis',(-7.09974814698911E-30,7.88860905221012E-30,
-1.));
#12841=DIRECTION('ref_axis',(-1.,2.12959150172473E-29,7.09974814698911E-30));
#12842=DIRECTION('center_axis',(-7.09974814698911E-30,7.88860905221012E-30,
-1.));
#12843=DIRECTION('ref_axis',(-1.,2.12959150172473E-29,7.09974814698911E-30));
#12844=DIRECTION('center_axis',(-7.09974814698911E-30,7.88860905221012E-30,
-1.));
#12845=DIRECTION('ref_axis',(-1.,2.12959150172473E-29,7.09974814698911E-30));
#12846=DIRECTION('center_axis',(-7.09974814698911E-30,7.88860905221012E-30,
-1.));
#12847=DIRECTION('ref_axis',(-1.,2.12959150172473E-29,7.09974814698911E-30));
#12848=DIRECTION('center_axis',(-7.09974814698911E-30,7.88860905221012E-30,
-1.));
#12849=DIRECTION('ref_axis',(-1.,2.12959150172473E-29,7.09974814698911E-30));
#12850=DIRECTION('center_axis',(-7.09974814698911E-30,7.88860905221012E-30,
-1.));
#12851=DIRECTION('ref_axis',(-1.,2.12959150172473E-29,7.09974814698911E-30));
#12852=DIRECTION('center_axis',(-7.09974814698911E-30,7.88860905221012E-30,
-1.));
#12853=DIRECTION('ref_axis',(-1.,2.12959150172473E-29,7.09974814698911E-30));
#12854=DIRECTION('center_axis',(-7.09974814698911E-30,7.88860905221012E-30,
-1.));
#12855=DIRECTION('ref_axis',(-1.,2.12959150172473E-29,7.09974814698911E-30));
#12856=DIRECTION('center_axis',(-7.09974814698911E-30,7.88860905221012E-30,
-1.));
#12857=DIRECTION('ref_axis',(-1.,2.12959150172473E-29,7.09974814698911E-30));
#12858=DIRECTION('center_axis',(-7.09974814698911E-30,7.88860905221012E-30,
-1.));
#12859=DIRECTION('ref_axis',(-1.,2.12959150172473E-29,7.09974814698911E-30));
#12860=DIRECTION('center_axis',(-7.09974814698911E-30,7.88860905221012E-30,
-1.));
#12861=DIRECTION('ref_axis',(-1.,2.12959150172473E-29,7.09974814698911E-30));
#12862=DIRECTION('center_axis',(-7.09974814698911E-30,7.88860905221012E-30,
-1.));
#12863=DIRECTION('ref_axis',(-1.,2.12959150172473E-29,7.09974814698911E-30));
#12864=DIRECTION('center_axis',(-7.09974814698911E-30,7.88860905221012E-30,
-1.));
#12865=DIRECTION('ref_axis',(-1.,2.12959150172473E-29,7.09974814698911E-30));
#12866=DIRECTION('center_axis',(-7.09974814698911E-30,7.88860905221012E-30,
-1.));
#12867=DIRECTION('ref_axis',(-1.,2.12959150172473E-29,7.09974814698911E-30));
#12868=DIRECTION('center_axis',(-7.09974814698911E-30,7.88860905221012E-30,
-1.));
#12869=DIRECTION('ref_axis',(-1.,2.12959150172473E-29,7.09974814698911E-30));
#12870=DIRECTION('center_axis',(-7.09974814698911E-30,7.88860905221012E-30,
-1.));
#12871=DIRECTION('ref_axis',(-1.,2.12959150172473E-29,7.09974814698911E-30));
#12872=DIRECTION('center_axis',(-7.09974814698911E-30,7.88860905221012E-30,
-1.));
#12873=DIRECTION('ref_axis',(-1.,2.12959150172473E-29,7.09974814698911E-30));
#12874=DIRECTION('center_axis',(-7.09974814698911E-30,7.88860905221012E-30,
-1.));
#12875=DIRECTION('ref_axis',(-1.,2.12959150172473E-29,7.09974814698911E-30));
#12876=DIRECTION('center_axis',(-7.09974814698911E-30,7.88860905221012E-30,
-1.));
#12877=DIRECTION('ref_axis',(-1.,2.12959150172473E-29,7.09974814698911E-30));
#12878=DIRECTION('center_axis',(-7.09974814698911E-30,7.88860905221012E-30,
-1.));
#12879=DIRECTION('ref_axis',(-1.,2.12959150172473E-29,7.09974814698911E-30));
#12880=DIRECTION('center_axis',(-7.09974814698911E-30,7.88860905221012E-30,
-1.));
#12881=DIRECTION('ref_axis',(-1.,2.12959150172473E-29,7.09974814698911E-30));
#12882=DIRECTION('center_axis',(-7.09974814698911E-30,7.88860905221012E-30,
-1.));
#12883=DIRECTION('ref_axis',(-1.,2.12959150172473E-29,7.09974814698911E-30));
#12884=DIRECTION('center_axis',(-7.09974814698911E-30,7.88860905221012E-30,
-1.));
#12885=DIRECTION('ref_axis',(-1.,2.12959150172473E-29,7.09974814698911E-30));
#12886=DIRECTION('center_axis',(-7.09974814698911E-30,7.88860905221012E-30,
-1.));
#12887=DIRECTION('ref_axis',(-1.,2.12959150172473E-29,7.09974814698911E-30));
#12888=DIRECTION('center_axis',(-7.09974814698911E-30,7.88860905221012E-30,
-1.));
#12889=DIRECTION('ref_axis',(-1.,2.12959150172473E-29,7.09974814698911E-30));
#12890=DIRECTION('center_axis',(-7.09974814698911E-30,7.88860905221012E-30,
-1.));
#12891=DIRECTION('ref_axis',(-1.,2.12959150172473E-29,7.09974814698911E-30));
#12892=DIRECTION('center_axis',(-7.09974814698911E-30,7.88860905221012E-30,
-1.));
#12893=DIRECTION('ref_axis',(-1.,2.12959150172473E-29,7.09974814698911E-30));
#12894=DIRECTION('center_axis',(-7.09974814698911E-30,7.88860905221012E-30,
-1.));
#12895=DIRECTION('ref_axis',(-1.,2.12959150172473E-29,7.09974814698911E-30));
#12896=DIRECTION('center_axis',(-7.09974814698911E-30,7.88860905221012E-30,
-1.));
#12897=DIRECTION('ref_axis',(-1.,2.12959150172473E-29,7.09974814698911E-30));
#12898=DIRECTION('center_axis',(-7.09974814698911E-30,7.88860905221012E-30,
-1.));
#12899=DIRECTION('ref_axis',(-1.,2.12959150172473E-29,7.09974814698911E-30));
#12900=DIRECTION('center_axis',(-7.09974814698911E-30,7.88860905221012E-30,
-1.));
#12901=DIRECTION('ref_axis',(-1.,2.12959150172473E-29,7.09974814698911E-30));
#12902=DIRECTION('center_axis',(-7.09974814698911E-30,7.88860905221012E-30,
-1.));
#12903=DIRECTION('ref_axis',(-1.,2.12959150172473E-29,7.09974814698911E-30));
#12904=DIRECTION('center_axis',(-7.09974814698911E-30,7.88860905221012E-30,
-1.));
#12905=DIRECTION('ref_axis',(-1.,2.12959150172473E-29,7.09974814698911E-30));
#12906=DIRECTION('center_axis',(-7.09974814698911E-30,7.88860905221012E-30,
-1.));
#12907=DIRECTION('ref_axis',(-1.,2.12959150172473E-29,7.09974814698911E-30));
#12908=DIRECTION('center_axis',(-7.09974814698911E-30,7.88860905221012E-30,
-1.));
#12909=DIRECTION('ref_axis',(-1.,2.12959150172473E-29,7.09974814698911E-30));
#12910=DIRECTION('center_axis',(-7.09974814698911E-30,7.88860905221012E-30,
-1.));
#12911=DIRECTION('ref_axis',(-1.,2.12959150172473E-29,7.09974814698911E-30));
#12912=DIRECTION('center_axis',(-7.09974814698911E-30,7.88860905221012E-30,
-1.));
#12913=DIRECTION('ref_axis',(-1.,2.12959150172473E-29,7.09974814698911E-30));
#12914=DIRECTION('center_axis',(-7.09974814698911E-30,7.88860905221012E-30,
-1.));
#12915=DIRECTION('ref_axis',(-1.,2.12959150172473E-29,7.09974814698911E-30));
#12916=DIRECTION('center_axis',(-7.09974814698911E-30,7.88860905221012E-30,
-1.));
#12917=DIRECTION('ref_axis',(-1.,2.12959150172473E-29,7.09974814698911E-30));
#12918=DIRECTION('center_axis',(-7.09974814698911E-30,7.88860905221012E-30,
-1.));
#12919=DIRECTION('ref_axis',(-1.,2.12959150172473E-29,7.09974814698911E-30));
#12920=DIRECTION('center_axis',(-7.09974814698911E-30,7.88860905221012E-30,
-1.));
#12921=DIRECTION('ref_axis',(-1.,2.12959150172473E-29,7.09974814698911E-30));
#12922=DIRECTION('center_axis',(-7.09974814698911E-30,7.88860905221012E-30,
-1.));
#12923=DIRECTION('ref_axis',(-1.,2.12959150172473E-29,7.09974814698911E-30));
#12924=DIRECTION('center_axis',(-7.09974814698911E-30,7.88860905221012E-30,
-1.));
#12925=DIRECTION('ref_axis',(-1.,2.12959150172473E-29,7.09974814698911E-30));
#12926=DIRECTION('center_axis',(-7.09974814698911E-30,7.88860905221012E-30,
-1.));
#12927=DIRECTION('ref_axis',(-1.,2.12959150172473E-29,7.09974814698911E-30));
#12928=DIRECTION('center_axis',(-7.09974814698911E-30,7.88860905221012E-30,
-1.));
#12929=DIRECTION('ref_axis',(-1.,2.12959150172473E-29,7.09974814698911E-30));
#12930=DIRECTION('center_axis',(-7.09974814698911E-30,7.88860905221012E-30,
-1.));
#12931=DIRECTION('ref_axis',(-1.,2.12959150172473E-29,7.09974814698911E-30));
#12932=DIRECTION('center_axis',(-7.09974814698911E-30,7.88860905221012E-30,
-1.));
#12933=DIRECTION('ref_axis',(-1.,2.12959150172473E-29,7.09974814698911E-30));
#12934=DIRECTION('center_axis',(-7.09974814698911E-30,7.88860905221012E-30,
-1.));
#12935=DIRECTION('ref_axis',(-1.,2.12959150172473E-29,7.09974814698911E-30));
#12936=DIRECTION('center_axis',(-6.70531769437859E-30,-7.88860905221012E-30,
1.));
#12937=DIRECTION('ref_axis',(1.,-2.12941982799268E-29,6.70531769437859E-30));
#12938=DIRECTION('',(2.12941982799268E-29,-1.,6.31088724176809E-30));
#12939=DIRECTION('',(1.,-2.12941982799268E-29,6.70531769437859E-30));
#12940=DIRECTION('',(2.12941982799268E-29,-1.,6.31088724176809E-30));
#12941=DIRECTION('center_axis',(-6.70531769437859E-30,-7.88860905221012E-30,
1.));
#12942=DIRECTION('ref_axis',(1.,-2.12941982799268E-29,6.70531769437859E-30));
#12943=DIRECTION('',(2.12941982799268E-29,-1.,6.31088724176809E-30));
#12944=DIRECTION('',(2.12941982799268E-29,-1.,6.31088724176809E-30));
#12945=DIRECTION('',(1.,-2.12941982799268E-29,6.70531769437859E-30));
#12946=DIRECTION('center_axis',(1.,-2.12941982799268E-29,-7.09974814698911E-30));
#12947=DIRECTION('ref_axis',(-7.09974814698911E-30,7.88860905221012E-30,
-1.));
#12948=DIRECTION('',(-7.09974814698911E-30,7.88860905221012E-30,-1.));
#12949=DIRECTION('center_axis',(1.,-2.12941982799268E-29,-7.09974814698911E-30));
#12950=DIRECTION('ref_axis',(-7.09974814698911E-30,7.88860905221012E-30,
-1.));
#12951=DIRECTION('',(-7.09974814698911E-30,7.88860905221012E-30,-1.));
#12952=DIRECTION('center_axis',(-2.12941982799268E-29,1.,7.88860905221012E-30));
#12953=DIRECTION('ref_axis',(7.09974814698911E-30,-7.88860905221012E-30,
1.));
#12954=DIRECTION('center_axis',(7.09974814698911E-30,-7.88860905221012E-30,
1.));
#12955=DIRECTION('ref_axis',(-1.,-1.10026367343295E-58,7.0997481469891E-30));
#12956=DIRECTION('center_axis',(7.09974814698911E-30,-7.88860905221012E-30,
1.));
#12957=DIRECTION('ref_axis',(-1.,-1.10026367343295E-58,7.0997481469891E-30));
#12958=DIRECTION('center_axis',(-7.09974814698911E-30,7.88860905221012E-30,
-1.));
#12959=DIRECTION('ref_axis',(1.,1.0890276736257E-58,-7.09974814698911E-30));
#12960=DIRECTION('center_axis',(-7.09974814698911E-30,7.88860905221012E-30,
-1.));
#12961=DIRECTION('ref_axis',(-1.,-1.0890276736257E-58,7.09974814698911E-30));
#12962=DIRECTION('center_axis',(-7.09974814698911E-30,7.88860905221012E-30,
-1.));
#12963=DIRECTION('ref_axis',(-0.989821441880933,0.142314838273285,8.1501490693107E-30));
#12964=DIRECTION('center_axis',(-7.09974814698911E-30,7.88860905221012E-30,
-1.));
#12965=DIRECTION('ref_axis',(0.989821441880933,-0.142314838273285,-8.1501490693107E-30));
#12966=DIRECTION('center_axis',(7.09974814698911E-30,-7.88860905221012E-30,
1.));
#12967=DIRECTION('ref_axis',(-0.989821441880933,0.142314838273285,8.15014906931069E-30));
#12968=DIRECTION('center_axis',(7.09974814698911E-30,-7.88860905221012E-30,
1.));
#12969=DIRECTION('ref_axis',(-0.989821441880933,0.142314838273285,8.15014906931069E-30));
#12970=DIRECTION('center_axis',(-7.09974814698911E-30,7.88860905221012E-30,
-1.));
#12971=DIRECTION('ref_axis',(-0.959492973614497,0.28173255684143,9.0346364596702E-30));
#12972=DIRECTION('center_axis',(-7.09974814698911E-30,7.88860905221012E-30,
-1.));
#12973=DIRECTION('ref_axis',(0.959492973614497,-0.281732556841431,-9.03463645967021E-30));
#12974=DIRECTION('center_axis',(7.09974814698911E-30,-7.88860905221012E-30,
1.));
#12975=DIRECTION('ref_axis',(-0.959492973614497,0.28173255684143,9.0346364596702E-30));
#12976=DIRECTION('center_axis',(7.09974814698911E-30,-7.88860905221012E-30,
1.));
#12977=DIRECTION('ref_axis',(-0.959492973614497,0.28173255684143,9.0346364596702E-30));
#12978=DIRECTION('center_axis',(-7.09974814698911E-30,7.88860905221012E-30,
-1.));
#12979=DIRECTION('ref_axis',(-0.909631995354518,0.415415013001887,9.73520470545092E-30));
#12980=DIRECTION('center_axis',(-7.09974814698911E-30,7.88860905221012E-30,
-1.));
#12981=DIRECTION('ref_axis',(0.909631995354518,-0.415415013001887,-9.73520470545091E-30));
#12982=DIRECTION('center_axis',(7.09974814698911E-30,-7.88860905221012E-30,
1.));
#12983=DIRECTION('ref_axis',(-0.909631995354518,0.415415013001887,9.73520470545091E-30));
#12984=DIRECTION('center_axis',(7.09974814698911E-30,-7.88860905221012E-30,
1.));
#12985=DIRECTION('ref_axis',(-0.909631995354518,0.415415013001887,9.73520470545091E-30));
#12986=DIRECTION('center_axis',(-7.09974814698911E-30,7.88860905221012E-30,
-1.));
#12987=DIRECTION('ref_axis',(-0.841253532831181,0.540640817455599,1.02375922574407E-29));
#12988=DIRECTION('center_axis',(-7.09974814698911E-30,7.88860905221012E-30,
-1.));
#12989=DIRECTION('ref_axis',(0.84125353283118,-0.540640817455599,-1.02375922574407E-29));
#12990=DIRECTION('center_axis',(7.09974814698911E-30,-7.88860905221012E-30,
1.));
#12991=DIRECTION('ref_axis',(-0.84125353283118,0.5406408174556,1.02375922574407E-29));
#12992=DIRECTION('center_axis',(7.09974814698911E-30,-7.88860905221012E-30,
1.));
#12993=DIRECTION('ref_axis',(-0.84125353283118,0.5406408174556,1.02375922574407E-29));
#12994=DIRECTION('center_axis',(-7.09974814698911E-30,7.88860905221012E-30,
-1.));
#12995=DIRECTION('ref_axis',(-0.755749574354257,0.654860733945286,1.05315719538472E-29));
#12996=DIRECTION('center_axis',(-7.09974814698911E-30,7.88860905221012E-30,
-1.));
#12997=DIRECTION('ref_axis',(0.755749574354257,-0.654860733945286,-1.05315719538472E-29));
#12998=DIRECTION('center_axis',(7.09974814698911E-30,-7.88860905221012E-30,
1.));
#12999=DIRECTION('ref_axis',(-0.755749574354257,0.654860733945286,1.05315719538472E-29));
#13000=DIRECTION('center_axis',(7.09974814698911E-30,-7.88860905221012E-30,
1.));
#13001=DIRECTION('ref_axis',(-0.755749574354257,0.654860733945286,1.05315719538472E-29));
#13002=DIRECTION('center_axis',(-7.09974814698911E-30,7.88860905221012E-30,
-1.));
#13003=DIRECTION('ref_axis',(-0.654860733945284,0.755749574354259,1.06111592158189E-29));
#13004=DIRECTION('center_axis',(-7.09974814698911E-30,7.88860905221012E-30,
-1.));
#13005=DIRECTION('ref_axis',(0.654860733945284,-0.75574957435426,-1.06111592158189E-29));
#13006=DIRECTION('center_axis',(7.09974814698911E-30,-7.88860905221012E-30,
1.));
#13007=DIRECTION('ref_axis',(-0.654860733945284,0.755749574354259,1.06111592158189E-29));
#13008=DIRECTION('center_axis',(7.09974814698911E-30,-7.88860905221012E-30,
1.));
#13009=DIRECTION('ref_axis',(-0.654860733945284,0.755749574354259,1.06111592158189E-29));
#13010=DIRECTION('center_axis',(-7.09974814698911E-30,7.88860905221012E-30,
-1.));
#13011=DIRECTION('ref_axis',(-0.540640817455596,0.841253532831182,1.04747338762128E-29));
#13012=DIRECTION('center_axis',(-7.09974814698911E-30,7.88860905221012E-30,
-1.));
#13013=DIRECTION('ref_axis',(0.540640817455596,-0.841253532831182,-1.04747338762128E-29));
#13014=DIRECTION('center_axis',(7.09974814698911E-30,-7.88860905221012E-30,
1.));
#13015=DIRECTION('ref_axis',(-0.540640817455596,0.841253532831182,1.04747338762128E-29));
#13016=DIRECTION('center_axis',(7.09974814698911E-30,-7.88860905221012E-30,
1.));
#13017=DIRECTION('ref_axis',(-0.540640817455596,0.841253532831182,1.04747338762128E-29));
#13018=DIRECTION('center_axis',(-7.09974814698911E-30,7.88860905221012E-30,
-1.));
#13019=DIRECTION('ref_axis',(-0.415415013001884,0.909631995354519,1.01250731615252E-29));
#13020=DIRECTION('center_axis',(-7.09974814698911E-30,7.88860905221012E-30,
-1.));
#13021=DIRECTION('ref_axis',(0.415415013001884,-0.909631995354519,-1.01250731615252E-29));
#13022=DIRECTION('center_axis',(7.09974814698911E-30,-7.88860905221012E-30,
1.));
#13023=DIRECTION('ref_axis',(-0.415415013001883,0.90963199535452,1.01250731615252E-29));
#13024=DIRECTION('center_axis',(7.09974814698911E-30,-7.88860905221012E-30,
1.));
#13025=DIRECTION('ref_axis',(-0.415415013001883,0.90963199535452,1.01250731615252E-29));
#13026=DIRECTION('center_axis',(-7.09974814698911E-30,7.88860905221012E-30,
-1.));
#13027=DIRECTION('ref_axis',(-0.281732556841427,0.959492973614498,9.56929515556876E-30));
#13028=DIRECTION('center_axis',(-7.09974814698911E-30,7.88860905221012E-30,
-1.));
#13029=DIRECTION('ref_axis',(0.281732556841427,-0.959492973614498,-9.56929515556876E-30));
#13030=DIRECTION('center_axis',(7.09974814698911E-30,-7.88860905221012E-30,
1.));
#13031=DIRECTION('ref_axis',(-0.281732556841426,0.959492973614498,9.56929515556875E-30));
#13032=DIRECTION('center_axis',(7.09974814698911E-30,-7.88860905221012E-30,
1.));
#13033=DIRECTION('ref_axis',(-0.281732556841426,0.959492973614498,9.56929515556875E-30));
#13034=DIRECTION('center_axis',(-7.09974814698911E-30,7.88860905221012E-30,
-1.));
#13035=DIRECTION('ref_axis',(-0.142314838273282,0.989821441880933,8.81871389581339E-30));
#13036=DIRECTION('center_axis',(-7.09974814698911E-30,7.88860905221012E-30,
-1.));
#13037=DIRECTION('ref_axis',(0.142314838273282,-0.989821441880933,-8.81871389581339E-30));
#13038=DIRECTION('center_axis',(7.09974814698911E-30,-7.88860905221012E-30,
1.));
#13039=DIRECTION('ref_axis',(-0.142314838273281,0.989821441880933,8.81871389581338E-30));
#13040=DIRECTION('center_axis',(7.09974814698911E-30,-7.88860905221012E-30,
1.));
#13041=DIRECTION('ref_axis',(-0.142314838273281,0.989821441880933,8.81871389581338E-30));
#13042=DIRECTION('center_axis',(-7.09974814698911E-30,7.88860905221012E-30,
-1.));
#13043=DIRECTION('ref_axis',(3.85494105772623E-15,1.,7.88860905221009E-30));
#13044=DIRECTION('center_axis',(-7.09974814698911E-30,7.88860905221012E-30,
-1.));
#13045=DIRECTION('ref_axis',(-3.85494105772623E-15,-1.,-7.88860905221009E-30));
#13046=DIRECTION('center_axis',(7.09974814698911E-30,-7.88860905221012E-30,
1.));
#13047=DIRECTION('ref_axis',(3.85494105772623E-15,1.,7.88860905221009E-30));
#13048=DIRECTION('center_axis',(7.09974814698911E-30,-7.88860905221012E-30,
1.));
#13049=DIRECTION('ref_axis',(3.85494105772623E-15,1.,7.88860905221009E-30));
#13050=DIRECTION('center_axis',(-7.09974814698911E-30,7.88860905221012E-30,
-1.));
#13051=DIRECTION('ref_axis',(0.142314838273289,0.989821441880932,6.79791487717376E-30));
#13052=DIRECTION('center_axis',(-7.09974814698911E-30,7.88860905221012E-30,
-1.));
#13053=DIRECTION('ref_axis',(-0.142314838273289,-0.989821441880932,-6.79791487717376E-30));
#13054=DIRECTION('center_axis',(7.09974814698911E-30,-7.88860905221012E-30,
1.));
#13055=DIRECTION('ref_axis',(0.142314838273288,0.989821441880932,6.79791487717376E-30));
#13056=DIRECTION('center_axis',(7.09974814698911E-30,-7.88860905221012E-30,
1.));
#13057=DIRECTION('ref_axis',(0.142314838273288,0.989821441880932,6.79791487717376E-30));
#13058=DIRECTION('center_axis',(-7.09974814698911E-30,7.88860905221012E-30,
-1.));
#13059=DIRECTION('ref_axis',(0.281732556841434,0.959492973614496,5.56883475880585E-30));
#13060=DIRECTION('center_axis',(-7.09974814698911E-30,7.88860905221012E-30,
-1.));
#13061=DIRECTION('ref_axis',(-0.281732556841434,-0.959492973614496,-5.56883475880585E-30));
#13062=DIRECTION('center_axis',(7.09974814698911E-30,-7.88860905221012E-30,
1.));
#13063=DIRECTION('ref_axis',(0.281732556841434,0.959492973614496,5.56883475880585E-30));
#13064=DIRECTION('center_axis',(7.09974814698911E-30,-7.88860905221012E-30,
1.));
#13065=DIRECTION('ref_axis',(0.281732556841434,0.959492973614496,5.56883475880585E-30));
#13066=DIRECTION('center_axis',(-7.09974814698911E-30,7.88860905221012E-30,
-1.));
#13067=DIRECTION('ref_axis',(0.415415013001891,0.909631995354516,4.22638922394196E-30));
#13068=DIRECTION('center_axis',(-7.09974814698911E-30,7.88860905221012E-30,
-1.));
#13069=DIRECTION('ref_axis',(-0.415415013001891,-0.909631995354516,-4.22638922394196E-30));
#13070=DIRECTION('center_axis',(7.09974814698911E-30,-7.88860905221012E-30,
1.));
#13071=DIRECTION('ref_axis',(0.415415013001891,0.909631995354516,4.22638922394196E-30));
#13072=DIRECTION('center_axis',(7.09974814698911E-30,-7.88860905221012E-30,
1.));
#13073=DIRECTION('ref_axis',(0.415415013001891,0.909631995354516,4.22638922394196E-30));
#13074=DIRECTION('center_axis',(-7.09974814698911E-30,7.88860905221012E-30,
-1.));
#13075=DIRECTION('ref_axis',(0.0473042560766741,0.998880527068694,7.54392966348545E-30));
#13076=DIRECTION('center_axis',(-7.09974814698911E-30,7.88860905221012E-30,
-1.));
#13077=DIRECTION('ref_axis',(-0.646029139287098,-0.76331274795589,-1.43483166863767E-30));
#13078=DIRECTION('center_axis',(7.09974814698911E-30,-7.88860905221012E-30,
1.));
#13079=DIRECTION('ref_axis',(0.27333986172383,-0.961917522448155,-9.52883545183607E-30));
#13080=DIRECTION('center_axis',(7.09974814698911E-30,-7.88860905221012E-30,
1.));
#13081=DIRECTION('ref_axis',(0.27333986172383,-0.961917522448155,-9.52883545183607E-30));
#13082=DIRECTION('center_axis',(-7.09974814698911E-30,7.88860905221012E-30,
-1.));
#13083=DIRECTION('ref_axis',(0.654860733945289,0.755749574354255,1.31246665109093E-30));
#13084=DIRECTION('center_axis',(-7.09974814698911E-30,7.88860905221012E-30,
-1.));
#13085=DIRECTION('ref_axis',(-0.654860733945289,-0.755749574354255,-1.31246665109092E-30));
#13086=DIRECTION('center_axis',(7.09974814698911E-30,-7.88860905221012E-30,
1.));
#13087=DIRECTION('ref_axis',(0.654860733945288,0.755749574354255,1.31246665109094E-30));
#13088=DIRECTION('center_axis',(7.09974814698911E-30,-7.88860905221012E-30,
1.));
#13089=DIRECTION('ref_axis',(0.654860733945288,0.755749574354255,1.31246665109094E-30));
#13090=DIRECTION('center_axis',(-7.09974814698911E-30,7.88860905221012E-30,
-1.));
#13091=DIRECTION('ref_axis',(0.755749574354262,0.654860733945281,-1.99691326371774E-31));
#13092=DIRECTION('center_axis',(-7.09974814698911E-30,7.88860905221012E-30,
-1.));
#13093=DIRECTION('ref_axis',(-0.755749574354262,-0.654860733945281,1.99691326371774E-31));
#13094=DIRECTION('center_axis',(7.09974814698911E-30,-7.88860905221012E-30,
1.));
#13095=DIRECTION('ref_axis',(0.755749574354263,0.65486073394528,-1.99691326371783E-31));
#13096=DIRECTION('center_axis',(7.09974814698911E-30,-7.88860905221012E-30,
1.));
#13097=DIRECTION('ref_axis',(0.755749574354263,0.65486073394528,-1.99691326371783E-31));
#13098=DIRECTION('center_axis',(-7.09974814698911E-30,7.88860905221012E-30,
-1.));
#13099=DIRECTION('ref_axis',(0.841253532831184,0.540640817455593,-1.70778416429177E-30));
#13100=DIRECTION('center_axis',(-7.09974814698911E-30,7.88860905221012E-30,
-1.));
#13101=DIRECTION('ref_axis',(-0.841253532831185,-0.540640817455593,1.70778416429178E-30));
#13102=DIRECTION('center_axis',(7.09974814698911E-30,-7.88860905221012E-30,
1.));
#13103=DIRECTION('ref_axis',(0.841253532831184,0.540640817455592,-1.70778416429178E-30));
#13104=DIRECTION('center_axis',(7.09974814698911E-30,-7.88860905221012E-30,
1.));
#13105=DIRECTION('ref_axis',(0.841253532831184,0.540640817455592,-1.70778416429178E-30));
#13106=DIRECTION('center_axis',(-7.09974814698911E-30,7.88860905221012E-30,
-1.));
#13107=DIRECTION('ref_axis',(0.909631995354521,0.415415013001881,-3.18111144146964E-30));
#13108=DIRECTION('center_axis',(-7.09974814698911E-30,7.88860905221012E-30,
-1.));
#13109=DIRECTION('ref_axis',(-0.909631995354521,-0.415415013001881,3.18111144146964E-30));
#13110=DIRECTION('center_axis',(7.09974814698911E-30,-7.88860905221012E-30,
1.));
#13111=DIRECTION('ref_axis',(0.909631995354522,0.415415013001879,-3.18111144146966E-30));
#13112=DIRECTION('center_axis',(7.09974814698911E-30,-7.88860905221012E-30,
1.));
#13113=DIRECTION('ref_axis',(0.909631995354522,0.415415013001879,-3.18111144146966E-30));
#13114=DIRECTION('center_axis',(-7.09974814698911E-30,7.88860905221012E-30,
-1.));
#13115=DIRECTION('ref_axis',(0.959492973614499,0.281732556841423,-4.58968046326706E-30));
#13116=DIRECTION('center_axis',(-7.09974814698911E-30,7.88860905221012E-30,
-1.));
#13117=DIRECTION('ref_axis',(-0.959492973614499,-0.281732556841423,4.58968046326706E-30));
#13118=DIRECTION('center_axis',(7.09974814698911E-30,-7.88860905221012E-30,
1.));
#13119=DIRECTION('ref_axis',(0.9594929736145,0.281732556841422,-4.58968046326707E-30));
#13120=DIRECTION('center_axis',(7.09974814698911E-30,-7.88860905221012E-30,
1.));
#13121=DIRECTION('ref_axis',(0.9594929736145,0.281732556841422,-4.58968046326707E-30));
#13122=DIRECTION('center_axis',(-7.09974814698911E-30,7.88860905221012E-30,
-1.));
#13123=DIRECTION('ref_axis',(0.989821441880934,0.142314838273278,-5.90481682637785E-30));
#13124=DIRECTION('center_axis',(-7.09974814698911E-30,7.88860905221012E-30,
-1.));
#13125=DIRECTION('ref_axis',(-0.989821441880934,-0.142314838273278,5.90481682637784E-30));
#13126=DIRECTION('center_axis',(7.09974814698911E-30,-7.88860905221012E-30,
1.));
#13127=DIRECTION('ref_axis',(0.989821441880934,0.142314838273277,-5.90481682637786E-30));
#13128=DIRECTION('center_axis',(7.09974814698911E-30,-7.88860905221012E-30,
1.));
#13129=DIRECTION('ref_axis',(0.989821441880934,0.142314838273277,-5.90481682637786E-30));
#13130=DIRECTION('center_axis',(-7.09974814698911E-30,7.88860905221012E-30,
-1.));
#13131=DIRECTION('ref_axis',(1.,1.0890276736257E-58,-7.09974814698911E-30));
#13132=DIRECTION('center_axis',(-7.09974814698911E-30,7.88860905221012E-30,
-1.));
#13133=DIRECTION('ref_axis',(-1.,-1.0890276736257E-58,7.09974814698911E-30));
#13134=DIRECTION('center_axis',(7.09974814698911E-30,-7.88860905221012E-30,
1.));
#13135=DIRECTION('ref_axis',(1.,1.0890276736257E-58,-7.0997481469891E-30));
#13136=DIRECTION('center_axis',(7.09974814698911E-30,-7.88860905221012E-30,
1.));
#13137=DIRECTION('ref_axis',(1.,1.0890276736257E-58,-7.0997481469891E-30));
#13138=DIRECTION('center_axis',(-7.09974814698911E-30,7.88860905221012E-30,
-1.));
#13139=DIRECTION('ref_axis',(0.989821441880932,-0.142314838273293,-8.15014906931075E-30));
#13140=DIRECTION('center_axis',(-7.09974814698911E-30,7.88860905221012E-30,
-1.));
#13141=DIRECTION('ref_axis',(-0.989821441880932,0.142314838273293,8.15014906931075E-30));
#13142=DIRECTION('center_axis',(7.09974814698911E-30,-7.88860905221012E-30,
1.));
#13143=DIRECTION('ref_axis',(0.989821441880932,-0.142314838273292,-8.15014906931074E-30));
#13144=DIRECTION('center_axis',(7.09974814698911E-30,-7.88860905221012E-30,
1.));
#13145=DIRECTION('ref_axis',(0.989821441880932,-0.142314838273292,-8.15014906931074E-30));
#13146=DIRECTION('center_axis',(-7.09974814698911E-30,7.88860905221012E-30,
-1.));
#13147=DIRECTION('ref_axis',(0.959492973614495,-0.281732556841437,-9.03463645967024E-30));
#13148=DIRECTION('center_axis',(-7.09974814698911E-30,7.88860905221012E-30,
-1.));
#13149=DIRECTION('ref_axis',(-0.959492973614495,0.281732556841437,9.03463645967024E-30));
#13150=DIRECTION('center_axis',(7.09974814698911E-30,-7.88860905221012E-30,
1.));
#13151=DIRECTION('ref_axis',(0.959492973614495,-0.281732556841437,-9.03463645967025E-30));
#13152=DIRECTION('center_axis',(7.09974814698911E-30,-7.88860905221012E-30,
1.));
#13153=DIRECTION('ref_axis',(0.959492973614495,-0.281732556841437,-9.03463645967025E-30));
#13154=DIRECTION('center_axis',(-7.09974814698911E-30,7.88860905221012E-30,
-1.));
#13155=DIRECTION('ref_axis',(0.909631995354515,-0.415415013001894,-9.73520470545095E-30));
#13156=DIRECTION('center_axis',(-7.09974814698911E-30,7.88860905221012E-30,
-1.));
#13157=DIRECTION('ref_axis',(-0.909631995354515,0.415415013001894,9.73520470545095E-30));
#13158=DIRECTION('center_axis',(7.09974814698911E-30,-7.88860905221012E-30,
1.));
#13159=DIRECTION('ref_axis',(0.909631995354515,-0.415415013001894,-9.73520470545095E-30));
#13160=DIRECTION('center_axis',(7.09974814698911E-30,-7.88860905221012E-30,
1.));
#13161=DIRECTION('ref_axis',(0.909631995354515,-0.415415013001894,-9.73520470545095E-30));
#13162=DIRECTION('center_axis',(-7.09974814698911E-30,7.88860905221012E-30,
-1.));
#13163=DIRECTION('ref_axis',(0.841253532831177,-0.540640817455604,-1.02375922574407E-29));
#13164=DIRECTION('center_axis',(-7.09974814698911E-30,7.88860905221012E-30,
-1.));
#13165=DIRECTION('ref_axis',(-0.841253532831177,0.540640817455605,1.02375922574407E-29));
#13166=DIRECTION('center_axis',(7.09974814698911E-30,-7.88860905221012E-30,
1.));
#13167=DIRECTION('ref_axis',(0.841253532831177,-0.540640817455604,-1.02375922574407E-29));
#13168=DIRECTION('center_axis',(7.09974814698911E-30,-7.88860905221012E-30,
1.));
#13169=DIRECTION('ref_axis',(0.841253532831177,-0.540640817455604,-1.02375922574407E-29));
#13170=DIRECTION('center_axis',(-7.09974814698911E-30,7.88860905221012E-30,
-1.));
#13171=DIRECTION('ref_axis',(0.755749574354253,-0.654860733945292,-1.05315719538472E-29));
#13172=DIRECTION('center_axis',(-7.09974814698911E-30,7.88860905221012E-30,
-1.));
#13173=DIRECTION('ref_axis',(-0.755749574354252,0.654860733945292,1.05315719538472E-29));
#13174=DIRECTION('center_axis',(7.09974814698911E-30,-7.88860905221012E-30,
1.));
#13175=DIRECTION('ref_axis',(0.755749574354253,-0.654860733945291,-1.05315719538472E-29));
#13176=DIRECTION('center_axis',(7.09974814698911E-30,-7.88860905221012E-30,
1.));
#13177=DIRECTION('ref_axis',(0.755749574354253,-0.654860733945291,-1.05315719538472E-29));
#13178=DIRECTION('center_axis',(-7.09974814698911E-30,7.88860905221012E-30,
-1.));
#13179=DIRECTION('ref_axis',(0.654860733945278,-0.755749574354264,-1.06111592158189E-29));
#13180=DIRECTION('center_axis',(-7.09974814698911E-30,7.88860905221012E-30,
-1.));
#13181=DIRECTION('ref_axis',(-0.654860733945278,0.755749574354264,1.06111592158189E-29));
#13182=DIRECTION('center_axis',(7.09974814698911E-30,-7.88860905221012E-30,
1.));
#13183=DIRECTION('ref_axis',(0.654860733945278,-0.755749574354264,-1.06111592158189E-29));
#13184=DIRECTION('center_axis',(7.09974814698911E-30,-7.88860905221012E-30,
1.));
#13185=DIRECTION('ref_axis',(0.654860733945278,-0.755749574354264,-1.06111592158189E-29));
#13186=DIRECTION('center_axis',(-7.09974814698911E-30,7.88860905221012E-30,
-1.));
#13187=DIRECTION('ref_axis',(0.540640817455589,-0.841253532831186,-1.04747338762128E-29));
#13188=DIRECTION('center_axis',(-7.09974814698911E-30,7.88860905221012E-30,
-1.));
#13189=DIRECTION('ref_axis',(-0.540640817455589,0.841253532831186,1.04747338762128E-29));
#13190=DIRECTION('center_axis',(7.09974814698911E-30,-7.88860905221012E-30,
1.));
#13191=DIRECTION('ref_axis',(0.540640817455589,-0.841253532831187,-1.04747338762128E-29));
#13192=DIRECTION('center_axis',(7.09974814698911E-30,-7.88860905221012E-30,
1.));
#13193=DIRECTION('ref_axis',(0.540640817455589,-0.841253532831187,-1.04747338762128E-29));
#13194=DIRECTION('center_axis',(-7.09974814698911E-30,7.88860905221012E-30,
-1.));
#13195=DIRECTION('ref_axis',(0.415415013001877,-0.909631995354522,-1.01250731615252E-29));
#13196=DIRECTION('center_axis',(-7.09974814698911E-30,7.88860905221012E-30,
-1.));
#13197=DIRECTION('ref_axis',(-0.415415013001877,0.909631995354522,1.01250731615252E-29));
#13198=DIRECTION('center_axis',(7.09974814698911E-30,-7.88860905221012E-30,
1.));
#13199=DIRECTION('ref_axis',(0.415415013001879,-0.909631995354522,-1.01250731615252E-29));
#13200=DIRECTION('center_axis',(7.09974814698911E-30,-7.88860905221012E-30,
1.));
#13201=DIRECTION('ref_axis',(0.415415013001879,-0.909631995354522,-1.01250731615252E-29));
#13202=DIRECTION('center_axis',(-7.09974814698911E-30,7.88860905221012E-30,
-1.));
#13203=DIRECTION('ref_axis',(0.281732556841419,-0.9594929736145,-9.56929515556872E-30));
#13204=DIRECTION('center_axis',(-7.09974814698911E-30,7.88860905221012E-30,
-1.));
#13205=DIRECTION('ref_axis',(-0.28173255684142,0.9594929736145,9.56929515556872E-30));
#13206=DIRECTION('center_axis',(7.09974814698911E-30,-7.88860905221012E-30,
1.));
#13207=DIRECTION('ref_axis',(0.281732556841418,-0.959492973614501,-9.56929515556872E-30));
#13208=DIRECTION('center_axis',(7.09974814698911E-30,-7.88860905221012E-30,
1.));
#13209=DIRECTION('ref_axis',(0.281732556841418,-0.959492973614501,-9.56929515556872E-30));
#13210=DIRECTION('center_axis',(-7.09974814698911E-30,7.88860905221012E-30,
-1.));
#13211=DIRECTION('ref_axis',(0.142314838273275,-0.989821441880934,-8.81871389581334E-30));
#13212=DIRECTION('center_axis',(-7.09974814698911E-30,7.88860905221012E-30,
-1.));
#13213=DIRECTION('ref_axis',(-0.142314838273275,0.989821441880934,8.81871389581335E-30));
#13214=DIRECTION('center_axis',(7.09974814698911E-30,-7.88860905221012E-30,
1.));
#13215=DIRECTION('ref_axis',(0.142314838273273,-0.989821441880935,-8.81871389581334E-30));
#13216=DIRECTION('center_axis',(7.09974814698911E-30,-7.88860905221012E-30,
1.));
#13217=DIRECTION('ref_axis',(0.142314838273273,-0.989821441880935,-8.81871389581334E-30));
#13218=DIRECTION('center_axis',(-7.09974814698911E-30,7.88860905221012E-30,
-1.));
#13219=DIRECTION('ref_axis',(-1.04083408558608E-14,-1.,-7.88860905221005E-30));
#13220=DIRECTION('center_axis',(-7.09974814698911E-30,7.88860905221012E-30,
-1.));
#13221=DIRECTION('ref_axis',(1.04083408558608E-14,1.,7.88860905221005E-30));
#13222=DIRECTION('center_axis',(7.09974814698911E-30,-7.88860905221012E-30,
1.));
#13223=DIRECTION('ref_axis',(-1.15648231731787E-14,-1.,-7.88860905221003E-30));
#13224=DIRECTION('center_axis',(7.09974814698911E-30,-7.88860905221012E-30,
1.));
#13225=DIRECTION('ref_axis',(-1.15648231731787E-14,-1.,-7.88860905221003E-30));
#13226=DIRECTION('center_axis',(-7.09974814698911E-30,7.88860905221012E-30,
-1.));
#13227=DIRECTION('ref_axis',(-0.142314838273296,-0.989821441880931,-6.7979148771737E-30));
#13228=DIRECTION('center_axis',(-7.09974814698911E-30,7.88860905221012E-30,
-1.));
#13229=DIRECTION('ref_axis',(0.142314838273296,0.989821441880931,6.7979148771737E-30));
#13230=DIRECTION('center_axis',(7.09974814698911E-30,-7.88860905221012E-30,
1.));
#13231=DIRECTION('ref_axis',(-0.142314838273296,-0.989821441880931,-6.7979148771737E-30));
#13232=DIRECTION('center_axis',(7.09974814698911E-30,-7.88860905221012E-30,
1.));
#13233=DIRECTION('ref_axis',(-0.142314838273296,-0.989821441880931,-6.7979148771737E-30));
#13234=DIRECTION('center_axis',(-7.09974814698911E-30,7.88860905221012E-30,
-1.));
#13235=DIRECTION('ref_axis',(-0.281732556841441,-0.959492973614494,-5.56883475880578E-30));
#13236=DIRECTION('center_axis',(-7.09974814698911E-30,7.88860905221012E-30,
-1.));
#13237=DIRECTION('ref_axis',(0.281732556841441,0.959492973614494,5.56883475880578E-30));
#13238=DIRECTION('center_axis',(7.09974814698911E-30,-7.88860905221012E-30,
1.));
#13239=DIRECTION('ref_axis',(-0.281732556841441,-0.959492973614494,-5.56883475880578E-30));
#13240=DIRECTION('center_axis',(7.09974814698911E-30,-7.88860905221012E-30,
1.));
#13241=DIRECTION('ref_axis',(-0.281732556841441,-0.959492973614494,-5.56883475880578E-30));
#13242=DIRECTION('center_axis',(-7.09974814698911E-30,7.88860905221012E-30,
-1.));
#13243=DIRECTION('ref_axis',(-0.415415013001897,-0.909631995354514,-4.22638922394189E-30));
#13244=DIRECTION('center_axis',(-7.09974814698911E-30,7.88860905221012E-30,
-1.));
#13245=DIRECTION('ref_axis',(0.415415013001897,0.909631995354513,4.22638922394189E-30));
#13246=DIRECTION('center_axis',(7.09974814698911E-30,-7.88860905221012E-30,
1.));
#13247=DIRECTION('ref_axis',(-0.415415013001898,-0.909631995354513,-4.22638922394188E-30));
#13248=DIRECTION('center_axis',(7.09974814698911E-30,-7.88860905221012E-30,
1.));
#13249=DIRECTION('ref_axis',(-0.415415013001898,-0.909631995354513,-4.22638922394188E-30));
#13250=DIRECTION('center_axis',(-7.09974814698911E-30,7.88860905221012E-30,
-1.));
#13251=DIRECTION('ref_axis',(-0.0473042560766785,-0.998880527068694,-7.54392966348542E-30));
#13252=DIRECTION('center_axis',(-7.09974814698911E-30,7.88860905221012E-30,
-1.));
#13253=DIRECTION('ref_axis',(0.646029139287104,0.763312747955885,1.43483166863759E-30));
#13254=DIRECTION('center_axis',(7.49417859959961E-30,-7.88860905221012E-30,
1.));
#13255=DIRECTION('ref_axis',(-0.273339861723828,0.961917522448156,9.63664901721228E-30));
#13256=DIRECTION('center_axis',(7.49417859959961E-30,-7.88860905221012E-30,
1.));
#13257=DIRECTION('ref_axis',(-0.273339861723828,0.961917522448156,9.63664901721228E-30));
#13258=DIRECTION('center_axis',(-7.09974814698911E-30,7.88860905221012E-30,
-1.));
#13259=DIRECTION('ref_axis',(-0.654860733945295,-0.75574957435425,-1.31246665109085E-30));
#13260=DIRECTION('center_axis',(-7.09974814698911E-30,7.88860905221012E-30,
-1.));
#13261=DIRECTION('ref_axis',(0.654860733945295,0.75574957435425,1.31246665109085E-30));
#13262=DIRECTION('center_axis',(7.09974814698911E-30,-7.88860905221012E-30,
1.));
#13263=DIRECTION('ref_axis',(-0.654860733945294,-0.75574957435425,-1.31246665109085E-30));
#13264=DIRECTION('center_axis',(7.09974814698911E-30,-7.88860905221012E-30,
1.));
#13265=DIRECTION('ref_axis',(-0.654860733945294,-0.75574957435425,-1.31246665109085E-30));
#13266=DIRECTION('center_axis',(-7.09974814698911E-30,7.88860905221012E-30,
-1.));
#13267=DIRECTION('ref_axis',(-0.755749574354266,-0.654860733945276,1.99691326371847E-31));
#13268=DIRECTION('center_axis',(-7.09974814698911E-30,7.88860905221012E-30,
-1.));
#13269=DIRECTION('ref_axis',(0.755749574354267,0.654860733945276,-1.99691326371846E-31));
#13270=DIRECTION('center_axis',(7.09974814698911E-30,-7.88860905221012E-30,
1.));
#13271=DIRECTION('ref_axis',(-0.755749574354267,-0.654860733945275,1.99691326371857E-31));
#13272=DIRECTION('center_axis',(7.09974814698911E-30,-7.88860905221012E-30,
1.));
#13273=DIRECTION('ref_axis',(-0.755749574354267,-0.654860733945275,1.99691326371857E-31));
#13274=DIRECTION('center_axis',(-7.09974814698911E-30,7.88860905221012E-30,
-1.));
#13275=DIRECTION('ref_axis',(-0.841253532831189,-0.540640817455586,1.70778416429186E-30));
#13276=DIRECTION('center_axis',(-7.09974814698911E-30,7.88860905221012E-30,
-1.));
#13277=DIRECTION('ref_axis',(0.841253532831188,0.540640817455586,-1.70778416429185E-30));
#13278=DIRECTION('center_axis',(7.09974814698911E-30,-7.88860905221012E-30,
1.));
#13279=DIRECTION('ref_axis',(-0.841253532831189,-0.540640817455585,1.70778416429187E-30));
#13280=DIRECTION('center_axis',(7.09974814698911E-30,-7.88860905221012E-30,
1.));
#13281=DIRECTION('ref_axis',(-0.841253532831189,-0.540640817455585,1.70778416429187E-30));
#13282=DIRECTION('center_axis',(-7.09974814698911E-30,7.88860905221012E-30,
-1.));
#13283=DIRECTION('ref_axis',(-0.909631995354524,-0.415415013001874,3.18111144146971E-30));
#13284=DIRECTION('center_axis',(-7.09974814698911E-30,7.88860905221012E-30,
-1.));
#13285=DIRECTION('ref_axis',(0.909631995354524,0.415415013001874,-3.18111144146971E-30));
#13286=DIRECTION('center_axis',(7.09974814698911E-30,-7.88860905221012E-30,
1.));
#13287=DIRECTION('ref_axis',(-0.909631995354523,-0.415415013001875,3.1811114414697E-30));
#13288=DIRECTION('center_axis',(7.09974814698911E-30,-7.88860905221012E-30,
1.));
#13289=DIRECTION('ref_axis',(-0.909631995354523,-0.415415013001875,3.1811114414697E-30));
#13290=DIRECTION('center_axis',(-7.09974814698911E-30,7.88860905221012E-30,
-1.));
#13291=DIRECTION('ref_axis',(-0.959492973614501,-0.281732556841416,4.58968046326713E-30));
#13292=DIRECTION('center_axis',(-7.09974814698911E-30,7.88860905221012E-30,
-1.));
#13293=DIRECTION('ref_axis',(0.959492973614501,0.281732556841416,-4.58968046326713E-30));
#13294=DIRECTION('center_axis',(7.09974814698911E-30,-7.88860905221012E-30,
1.));
#13295=DIRECTION('ref_axis',(-0.959492973614502,-0.281732556841414,4.58968046326714E-30));
#13296=DIRECTION('center_axis',(7.09974814698911E-30,-7.88860905221012E-30,
1.));
#13297=DIRECTION('ref_axis',(-0.959492973614502,-0.281732556841414,4.58968046326714E-30));
#13298=DIRECTION('center_axis',(-7.09974814698911E-30,7.88860905221012E-30,
-1.));
#13299=DIRECTION('ref_axis',(-0.989821441880935,-0.142314838273271,5.90481682637791E-30));
#13300=DIRECTION('center_axis',(-7.09974814698911E-30,7.88860905221012E-30,
-1.));
#13301=DIRECTION('ref_axis',(0.989821441880935,0.142314838273271,-5.90481682637791E-30));
#13302=DIRECTION('center_axis',(7.09974814698911E-30,-7.88860905221012E-30,
1.));
#13303=DIRECTION('ref_axis',(-0.989821441880934,-0.142314838273273,5.90481682637789E-30));
#13304=DIRECTION('center_axis',(7.09974814698911E-30,-7.88860905221012E-30,
1.));
#13305=DIRECTION('ref_axis',(-0.989821441880934,-0.142314838273273,5.90481682637789E-30));
#17301=CARTESIAN_POINT('',(0.,0.,0.));
#17302=CARTESIAN_POINT('Origin',(0.,0.,-6.93889390390723E-15));
#17303=CARTESIAN_POINT('',(-3.54343684303821,-43.3554385900939,6.16441400296896));
#17304=CARTESIAN_POINT('',(-3.84642767658917,-41.3213624427943,0.));
#17305=CARTESIAN_POINT('Ctrl Pts',(-3.54343684303822,-43.3554385900939,
6.16441400296899));
#17306=CARTESIAN_POINT('Ctrl Pts',(-3.55141066631791,-42.7078411106921,
5.27531660683076));
#17307=CARTESIAN_POINT('Ctrl Pts',(-3.57572362730238,-42.2030493088126,
4.29109868658263));
#17308=CARTESIAN_POINT('Ctrl Pts',(-3.6760022876941,-41.5111240838458,2.19783870908455));
#17309=CARTESIAN_POINT('Ctrl Pts',(-3.75038336645554,-41.3303027940034,
1.10199792653041));
#17310=CARTESIAN_POINT('Ctrl Pts',(-3.84642767658919,-41.3213624427943,
1.38777878078145E-15));
#17311=CARTESIAN_POINT('',(-3.54327233497679,-43.3554520350116,-6.16441400296897));
#17312=CARTESIAN_POINT('Ctrl Pts',(-3.54327233497681,-43.3554520350116,
-6.16441400296899));
#17313=CARTESIAN_POINT('Ctrl Pts',(-3.55068393228085,-42.7074736895779,
-5.27472971793057));
#17314=CARTESIAN_POINT('Ctrl Pts',(-3.57665600754489,-42.2023811348684,
-4.28982003626222));
#17315=CARTESIAN_POINT('Ctrl Pts',(-3.67659250957593,-41.5108986473516,
-2.19678068827402));
#17316=CARTESIAN_POINT('Ctrl Pts',(-3.74909596947971,-41.3304226322436,
-1.10143125928569));
#17317=CARTESIAN_POINT('Ctrl Pts',(-3.84642767658919,-41.3213624427943,
-1.38777878078145E-15));
#17318=CARTESIAN_POINT('',(-1.48664137583835,-43.4745891000668,-6.16441400296897));
#17319=CARTESIAN_POINT('Origin',(-5.20417042793042E-15,1.73472347597681E-15,
-6.16441400296897));
#17320=CARTESIAN_POINT('',(-2.07336642434586,-41.448174286335,0.));
#17321=CARTESIAN_POINT('Ctrl Pts',(-2.07336642434585,-41.4481742863349,
9.0205620750794E-16));
#17322=CARTESIAN_POINT('Ctrl Pts',(-2.06122214993793,-41.4487817806634,
-0.137010845842713));
#17323=CARTESIAN_POINT('Ctrl Pts',(-2.04906663309419,-41.4520669390525,
-0.273849719833661));
#17324=CARTESIAN_POINT('Ctrl Pts',(-2.02470703660086,-41.4639867448445,
-0.547496131359158));
#17325=CARTESIAN_POINT('Ctrl Pts',(-2.01251001184278,-41.4726232572572,
-0.684223919449433));
#17326=CARTESIAN_POINT('Ctrl Pts',(-1.97587807515071,-41.5065536416689,
-1.09397285879738));
#17327=CARTESIAN_POINT('Ctrl Pts',(-1.95143443912056,-41.5398552486479,
-1.36621764182242));
#17328=CARTESIAN_POINT('Ctrl Pts',(-1.87808530350882,-41.6716267136228,
-2.17875768609682));
#17329=CARTESIAN_POINT('Ctrl Pts',(-1.82935412691929,-41.8017662331319,
-2.71300426676783));
#17330=CARTESIAN_POINT('Ctrl Pts',(-1.73185220830973,-42.144880341048,-3.75889728641896));
#17331=CARTESIAN_POINT('Ctrl Pts',(-1.68324609183627,-42.3577123750293,
-4.26878718252178));
#17332=CARTESIAN_POINT('Ctrl Pts',(-1.58505547146646,-42.8607776274967,
-5.24984087225669));
#17333=CARTESIAN_POINT('Ctrl Pts',(-1.53586728286777,-43.1500457179623,
-5.71948809643066));
#17334=CARTESIAN_POINT('Ctrl Pts',(-1.48664137583835,-43.4745891000668,
-6.16441400296899));
#17335=CARTESIAN_POINT('',(-1.48703027021499,-43.4745757998335,6.16441400296896));
#17336=CARTESIAN_POINT('Ctrl Pts',(-2.07336642434584,-41.4481742863349,
-2.77555756156289E-16));
#17337=CARTESIAN_POINT('Ctrl Pts',(-1.97732270203172,-41.4529786916566,
1.09861960926666));
#17338=CARTESIAN_POINT('Ctrl Pts',(-1.87861834962005,-41.630211988073,2.18971594132761));
#17339=CARTESIAN_POINT('Ctrl Pts',(-1.68194342719021,-42.3167003895122,
4.28292314717353));
#17340=CARTESIAN_POINT('Ctrl Pts',(-1.58640053900951,-42.8234325995621,
5.27177304443354));
#17341=CARTESIAN_POINT('Ctrl Pts',(-1.48703027021497,-43.4745757998335,
6.16441400296898));
#17342=CARTESIAN_POINT('Origin',(-1.73472347597681E-15,-1.73472347597681E-15,
6.16441400296896));
#17343=CARTESIAN_POINT('Origin',(0.,0.,-6.93889390390723E-15));
#17344=CARTESIAN_POINT('',(-9.67749199640668,-42.4098590973784,6.16441400296896));
#17345=CARTESIAN_POINT('',(-9.68791960221031,-40.3533668208876,0.));
#17346=CARTESIAN_POINT('Ctrl Pts',(-9.67749199640668,-42.4098590973784,
6.164414002969));
#17347=CARTESIAN_POINT('Ctrl Pts',(-9.59322192711545,-41.767718433188,5.27531660683078));
#17348=CARTESIAN_POINT('Ctrl Pts',(-9.54544805356732,-41.2646045888915,
4.29109868658267));
#17349=CARTESIAN_POINT('Ctrl Pts',(-9.54623479529778,-40.5654510237051,
2.19783870908455));
#17350=CARTESIAN_POINT('Ctrl Pts',(-9.59412522930581,-40.375884702676,1.1019979265304));
#17351=CARTESIAN_POINT('Ctrl Pts',(-9.68791960221032,-40.3533668208876,
1.11022302462516E-15));
#17352=CARTESIAN_POINT('',(-9.67733107621878,-42.4098958173827,-6.16441400296897));
#17353=CARTESIAN_POINT('Ctrl Pts',(-9.67733107621879,-42.4098958173827,
-6.164414002969));
#17354=CARTESIAN_POINT('Ctrl Pts',(-9.59245030071221,-41.7674581769263,
-5.2747297179302));
#17355=CARTESIAN_POINT('Ctrl Pts',(-9.5462758524577,-41.2638105244509,-4.28982003626219));
#17356=CARTESIAN_POINT('Ctrl Pts',(-9.54678692660889,-40.5651438845136,
-2.19678068831833));
#17357=CARTESIAN_POINT('Ctrl Pts',(-9.59286799090522,-40.3761865368352,
-1.10143125952358));
#17358=CARTESIAN_POINT('Ctrl Pts',(-9.68791960221033,-40.3533668208876,
-2.22044604925031E-15));
#17359=CARTESIAN_POINT('',(-7.65858862696402,-42.8205093412368,-6.16441400296901));
#17360=CARTESIAN_POINT('Origin',(-5.20417042793042E-15,1.73472347597681E-15,
-6.16441400296897));
#17361=CARTESIAN_POINT('',(-7.95095276397625,-40.7312208280702,0.));
#17362=CARTESIAN_POINT('Ctrl Pts',(-7.95095276397622,-40.7312208280702,
2.46330733588707E-15));
#17363=CARTESIAN_POINT('Ctrl Pts',(-7.93901575180353,-40.7335509968694,
-0.137043042087696));
#17364=CARTESIAN_POINT('Ctrl Pts',(-7.92744885398147,-40.7385344220979,
-0.273914065095848));
#17365=CARTESIAN_POINT('Ctrl Pts',(-7.90502864323289,-40.7538057116238,
-0.547624684008695));
#17366=CARTESIAN_POINT('Ctrl Pts',(-7.8941825814094,-40.7640944186137,-0.684384502473543));
#17367=CARTESIAN_POINT('Ctrl Pts',(-7.86274596139053,-40.8029092867107,
-1.09422919239435));
#17368=CARTESIAN_POINT('Ctrl Pts',(-7.8432869311216,-40.8393666280175,-1.36653715783867));
#17369=CARTESIAN_POINT('Ctrl Pts',(-7.78942904928734,-40.9802981987834,
-2.17926357855915));
#17370=CARTESIAN_POINT('Ctrl Pts',(-7.75971205509762,-41.1161093962788,
-2.71362913030393));
#17371=CARTESIAN_POINT('Ctrl Pts',(-7.7120439733908,-41.4696829616657,-3.75949691623912));
#17372=CARTESIAN_POINT('Ctrl Pts',(-7.69422964590224,-41.6872426581296,
-4.26925519586819));
#17373=CARTESIAN_POINT('Ctrl Pts',(-7.66864299491693,-42.1990770319903,
-5.25006061967085));
#17374=CARTESIAN_POINT('Ctrl Pts',(-7.66112555224713,-42.4923406106851,
-5.71959225708845));
#17375=CARTESIAN_POINT('Ctrl Pts',(-7.658588626964,-42.8205093412367,-6.16441400296904));
#17376=CARTESIAN_POINT('',(-7.65897167013779,-42.82044083094,6.16441400296896));
#17377=CARTESIAN_POINT('Ctrl Pts',(-7.95095276397622,-40.7312208280702,
-1.38777878078145E-15));
#17378=CARTESIAN_POINT('Ctrl Pts',(-7.85657036643801,-40.7496447782814,
1.09861960926659));
#17379=CARTESIAN_POINT('Ctrl Pts',(-7.7840936099301,-40.9391211892399,2.18971594132748));
#17380=CARTESIAN_POINT('Ctrl Pts',(-7.68711804045607,-41.646611888365,4.28292314717352));
#17381=CARTESIAN_POINT('Ctrl Pts',(-7.66466315363669,-42.1617834658437,
5.27177304443355));
#17382=CARTESIAN_POINT('Ctrl Pts',(-7.65897167013776,-42.8204408309399,
6.16441400296899));
#17383=CARTESIAN_POINT('Origin',(-1.73472347597681E-15,-1.73472347597681E-15,
6.16441400296896));
#17384=CARTESIAN_POINT('Origin',(0.,0.,-6.93889390390723E-15));
#17385=CARTESIAN_POINT('',(-15.6145413203107,-40.6009371733746,6.16441400296896));
#17386=CARTESIAN_POINT('',(-15.3321934223835,-38.563893020008,0.));
#17387=CARTESIAN_POINT('Ctrl Pts',(-15.6145413203107,-40.6009371733746,
6.16441400296898));
#17388=CARTESIAN_POINT('Ctrl Pts',(-15.4397428540445,-39.9773254565378,
5.27531660683075));
#17389=CARTESIAN_POINT('Ctrl Pts',(-15.3208546842607,-39.4861315168337,
4.29109868658265));
#17390=CARTESIAN_POINT('Ctrl Pts',(-15.2221334915371,-38.7939823618226,
2.19783870908461));
#17391=CARTESIAN_POINT('Ctrl Pts',(-15.2425583696598,-38.5995300332388,
1.10199792653054));
#17392=CARTESIAN_POINT('Ctrl Pts',(-15.3321934223835,-38.563893020008,2.4980018054066E-15));
#17393=CARTESIAN_POINT('',(-15.6143872638446,-40.6009964209586,-6.16441400296898));
#17394=CARTESIAN_POINT('Ctrl Pts',(-15.6143872638446,-40.6009964209586,
-6.164414002969));
#17395=CARTESIAN_POINT('Ctrl Pts',(-15.4389420434457,-39.9771776635648,
-5.27472971844796));
#17396=CARTESIAN_POINT('Ctrl Pts',(-15.3215610503336,-39.4852277273297,
-4.28982003740452));
#17397=CARTESIAN_POINT('Ctrl Pts',(-15.2474291081464,-38.9669376181131,
-2.72134440716479));
#17398=CARTESIAN_POINT('Ctrl Pts',(-15.2397722663402,-38.8316218835454,
-2.18467279509807));
#17399=CARTESIAN_POINT('Ctrl Pts',(-15.254622909041,-38.6871163772095,-1.36905841490953));
#17400=CARTESIAN_POINT('Ctrl Pts',(-15.2639410255199,-38.6487537976598,
-1.09600303225455));
#17401=CARTESIAN_POINT('Ctrl Pts',(-15.2845639945731,-38.6059048579417,
-0.685230045232502));
#17402=CARTESIAN_POINT('Ctrl Pts',(-15.2925374872687,-38.5940776984981,
-0.548230322286331));
#17403=CARTESIAN_POINT('Ctrl Pts',(-15.3107058126117,-38.5753161429334,
-0.274077591982354));
#17404=CARTESIAN_POINT('Ctrl Pts',(-15.3208934838215,-38.5683856381055,
-0.137016510472968));
#17405=CARTESIAN_POINT('Ctrl Pts',(-15.3321934223835,-38.563893020008,-1.2490009027033E-15));
#17406=CARTESIAN_POINT('',(-13.6746290992012,-41.2947274963679,-6.16441400296901));
#17407=CARTESIAN_POINT('Origin',(-5.20417042793042E-15,1.73472347597681E-15,
-6.16441400296897));
#17408=CARTESIAN_POINT('',(-13.6666806339864,-39.1850971728874,0.));
#17409=CARTESIAN_POINT('Ctrl Pts',(-13.6666806339864,-39.1850971728873,
1.70002900645727E-15));
#17410=CARTESIAN_POINT('Ctrl Pts',(-13.6551967409802,-39.1891024378853,
-0.137043042092346));
#17411=CARTESIAN_POINT('Ctrl Pts',(-13.6444567928547,-39.1956812802236,
-0.273914065098134));
#17412=CARTESIAN_POINT('Ctrl Pts',(-13.6244381186219,-39.2139878587089,
-0.547624684011075));
#17413=CARTESIAN_POINT('Ctrl Pts',(-13.6151666897398,-39.2257153970312,
-0.684384502476133));
#17414=CARTESIAN_POINT('Ctrl Pts',(-13.5895739808594,-39.268609083232,-1.09422919239856));
#17415=CARTESIAN_POINT('Ctrl Pts',(-13.5755014360926,-39.3074646501175,
-1.36653715784331));
#17416=CARTESIAN_POINT('Ctrl Pts',(-13.5422484035402,-39.4546265164425,
-2.17926357856199));
#17417=CARTESIAN_POINT('Ctrl Pts',(-13.5321618341116,-39.5932845209921,
-2.71362913030486));
#17418=CARTESIAN_POINT('Ctrl Pts',(-13.5352977095238,-39.9500430926316,
-3.75949691623844));
#17419=CARTESIAN_POINT('Ctrl Pts',(-13.5486266792216,-40.1679235882157,
-4.26925519586768));
#17420=CARTESIAN_POINT('Ctrl Pts',(-13.5961420895942,-40.6781895862498,
-5.25006061967041));
#17421=CARTESIAN_POINT('Ctrl Pts',(-13.6304369224277,-40.9695380082016,
-5.71959225708826));
#17422=CARTESIAN_POINT('Ctrl Pts',(-13.6746290992012,-41.2947274963679,
-6.16441400296904));
#17423=CARTESIAN_POINT('',(-13.674998493507,-41.2946051706828,6.16441400296896));
#17424=CARTESIAN_POINT('Ctrl Pts',(-13.6666806339864,-39.1850971728873,
-2.22044604925031E-15));
#17425=CARTESIAN_POINT('Ctrl Pts',(-13.5758809146616,-39.216765609492,1.09861960926666));
#17426=CARTESIAN_POINT('Ctrl Pts',(-13.5311071718143,-39.4146279416704,
2.1897159413276));
#17427=CARTESIAN_POINT('Ctrl Pts',(-13.5358050982361,-40.1287184680819,
4.28292314717352));
#17428=CARTESIAN_POINT('Ctrl Pts',(-13.5868953295191,-40.641842005304,5.2717730444335));
#17429=CARTESIAN_POINT('Ctrl Pts',(-13.674998493507,-41.2946051706828,6.16441400296898));
#17430=CARTESIAN_POINT('Origin',(-1.73472347597681E-15,-1.73472347597681E-15,
6.16441400296896));
#17431=CARTESIAN_POINT('Origin',(0.,0.,-6.93889390390723E-15));
#17432=CARTESIAN_POINT('',(-21.2337236115519,-37.9654972519553,6.16441400296896));
#17433=CARTESIAN_POINT('',(-20.6643479988718,-35.9893695663251,0.));
#17434=CARTESIAN_POINT('Ctrl Pts',(-21.2337236115519,-37.9654972519553,
6.16441400296898));
#17435=CARTESIAN_POINT('Ctrl Pts',(-20.9719551410068,-37.3731094186791,
5.27531660683075));
#17436=CARTESIAN_POINT('Ctrl Pts',(-20.784372895279,-36.9038346756933,4.29109868658264));
#17437=CARTESIAN_POINT('Ctrl Pts',(-20.5881534468967,-36.2327800916602,
2.19783870908455));
#17438=CARTESIAN_POINT('Ctrl Pts',(-20.5806969775162,-36.0374002441775,
1.10199792653042));
#17439=CARTESIAN_POINT('Ctrl Pts',(-20.6643479988717,-35.9893695663251,
2.22044604925031E-15));
#17440=CARTESIAN_POINT('',(-21.2335795549793,-37.9655778209995,-6.16441400296897));
#17441=CARTESIAN_POINT('Ctrl Pts',(-21.2335795549793,-37.9655778209995,
-6.16441400296899));
#17442=CARTESIAN_POINT('Ctrl Pts',(-20.9711414482259,-37.373077096907,-5.27472971792917));
#17443=CARTESIAN_POINT('Ctrl Pts',(-20.7849434486971,-36.9028395585411,
-4.28982003626091));
#17444=CARTESIAN_POINT('Ctrl Pts',(-20.5885966819103,-36.2323298404348,
-2.19678068843132));
#17445=CARTESIAN_POINT('Ctrl Pts',(-20.5795757025526,-36.0380440569569,
-1.10143126012878));
#17446=CARTESIAN_POINT('Ctrl Pts',(-20.6643479988717,-35.9893695663251,
-5.55111512312578E-16));
#17447=CARTESIAN_POINT('',(-19.4122935573269,-38.9283040838433,-6.16441400296902));
#17448=CARTESIAN_POINT('Origin',(-5.20417042793042E-15,1.73472347597681E-15,
-6.16441400296897));
#17449=CARTESIAN_POINT('',(-19.1041942977411,-36.8412779397534,0.));
#17450=CARTESIAN_POINT('Ctrl Pts',(-19.1041942977411,-36.8412779397534,
1.66533453693773E-15));
#17451=CARTESIAN_POINT('Ctrl Pts',(-19.0175901854858,-36.8861868538853,
-1.09924021646038));
#17452=CARTESIAN_POINT('Ctrl Pts',(-19.0022157487917,-37.0882313865091,
-2.19104319734134));
#17453=CARTESIAN_POINT('Ctrl Pts',(-19.0830118167184,-37.6171355518865,
-3.75949691436112));
#17454=CARTESIAN_POINT('Ctrl Pts',(-19.1272127442119,-37.8309014280932,
-4.26925519440142));
#17455=CARTESIAN_POINT('Ctrl Pts',(-19.2468629392382,-38.3292115063353,
-5.25006061898198));
#17456=CARTESIAN_POINT('Ctrl Pts',(-19.322271903712,-38.6127137580402,-5.71959225676187));
#17457=CARTESIAN_POINT('Ctrl Pts',(-19.4122935573269,-38.9283040838433,
-6.16441400296904));
#17458=CARTESIAN_POINT('',(-19.4126417829876,-38.9281304329582,6.16441400296896));
#17459=CARTESIAN_POINT('Ctrl Pts',(-19.1041942977411,-36.8412779397534,
5.55111512312578E-16));
#17460=CARTESIAN_POINT('Ctrl Pts',(-19.0188256770704,-36.8855461847065,
1.09861960926669));
#17461=CARTESIAN_POINT('Ctrl Pts',(-19.0026664121712,-37.0877665316095,
2.18971594132765));
#17462=CARTESIAN_POINT('Ctrl Pts',(-19.1089421982546,-37.7939200614567,
4.28292314717352));
#17463=CARTESIAN_POINT('Ctrl Pts',(-19.2325374978632,-38.2945498429305,
5.27177304443354));
#17464=CARTESIAN_POINT('Ctrl Pts',(-19.4126417829876,-38.9281304329582,
6.16441400296899));
#17465=CARTESIAN_POINT('Origin',(-1.73472347597681E-15,-1.73472347597681E-15,
6.16441400296896));
#17466=CARTESIAN_POINT('Origin',(0.,0.,-6.93889390390723E-15));
#17467=CARTESIAN_POINT('',(-26.4206485230644,-34.5571892899393,6.16441400296896));
#17468=CARTESIAN_POINT('',(-25.5758360411617,-32.6822063330434,0.));
#17469=CARTESIAN_POINT('Ctrl Pts',(-26.4206485230644,-34.5571892899393,
6.16441400296898));
#17470=CARTESIAN_POINT('Ctrl Pts',(-26.0772388994227,-34.0080846482038,
5.27531660683074));
#17471=CARTESIAN_POINT('Ctrl Pts',(-25.8247812113314,-33.5702821824271,
4.29109868658261));
#17472=CARTESIAN_POINT('Ctrl Pts',(-25.5350579694094,-32.9339829055412,
2.19783870908459));
#17473=CARTESIAN_POINT('Ctrl Pts',(-25.4998719447394,-32.7416529094253,
1.1019979265305));
#17474=CARTESIAN_POINT('Ctrl Pts',(-25.5758360411617,-32.6822063330433,
8.32667268468867E-16));
#17475=CARTESIAN_POINT('',(-26.4205173989538,-34.5572895402921,-6.16441400296898));
#17476=CARTESIAN_POINT('Ctrl Pts',(-26.4205173989538,-34.5572895402921,
-6.16441400296899));
#17477=CARTESIAN_POINT('Ctrl Pts',(-26.0764288890034,-34.0081684559713,
-5.27472971793099));
#17478=CARTESIAN_POINT('Ctrl Pts',(-25.825204337397,-33.5692159959191,-4.2898200362617));
#17479=CARTESIAN_POINT('Ctrl Pts',(-25.5354326154955,-32.9334741583167,
-2.1967806884535));
#17480=CARTESIAN_POINT('Ctrl Pts',(-25.498853706854,-32.7424497431807,-1.10143126024324));
#17481=CARTESIAN_POINT('Ctrl Pts',(-25.5758360411617,-32.6822063330433,
-1.94289029309402E-15));
#17482=CARTESIAN_POINT('',(-24.7547796990836,-35.7694126601185,-6.16441400296902));
#17483=CARTESIAN_POINT('Origin',(-5.20417042793042E-15,1.73472347597681E-15,
-6.16441400296897));
#17484=CARTESIAN_POINT('',(-24.1528016575408,-33.7474765292385,0.));
#17485=CARTESIAN_POINT('Ctrl Pts',(-24.1528016575407,-33.7474765292384,
7.63278329429795E-16));
#17486=CARTESIAN_POINT('Ctrl Pts',(-24.1429113564378,-33.7545549394024,
-0.137043042102339));
#17487=CARTESIAN_POINT('Ctrl Pts',(-24.1344599257467,-33.7638930854468,
-0.273914065100194));
#17488=CARTESIAN_POINT('Ctrl Pts',(-24.1204097076412,-33.7870980311517,
-0.547624684011823));
#17489=CARTESIAN_POINT('Ctrl Pts',(-24.1148178661299,-33.8009625851348,
-0.684384502477576));
#17490=CARTESIAN_POINT('Ctrl Pts',(-24.1023463896684,-33.8493290749669,
-1.09422919240133));
#17491=CARTESIAN_POINT('Ctrl Pts',(-24.0997907600507,-33.8905754123975,
-1.36653715784733));
#17492=CARTESIAN_POINT('Ctrl Pts',(-24.1093449978383,-34.0411446510019,
-2.17926357856575));
#17493=CARTESIAN_POINT('Ctrl Pts',(-24.1387314794962,-34.1770277470944,
-2.71362913030714));
#17494=CARTESIAN_POINT('Ctrl Pts',(-24.2422508344842,-34.5184516116601,
-3.75949691623867));
#17495=CARTESIAN_POINT('Ctrl Pts',(-24.3164239163555,-34.7237512115516,
-4.26925519586687));
#17496=CARTESIAN_POINT('Ctrl Pts',(-24.5057731630367,-35.199961213288,-5.25006061966791));
#17497=CARTESIAN_POINT('Ctrl Pts',(-24.6207611500201,-35.4698460060844,
-5.71959225708702));
#17498=CARTESIAN_POINT('Ctrl Pts',(-24.7547796990836,-35.7694126601185,
-6.16441400296905));
#17499=CARTESIAN_POINT('',(-24.7550996672026,-35.7691912190766,6.16441400296896));
#17500=CARTESIAN_POINT('Ctrl Pts',(-24.1528016575407,-33.7474765292384,
0.));
#17501=CARTESIAN_POINT('Ctrl Pts',(-24.0746019944582,-33.8034434087318,
1.09861960926657));
#17502=CARTESIAN_POINT('Ctrl Pts',(-24.087386163541,-34.0059051472517,2.18971594132744));
#17503=CARTESIAN_POINT('Ctrl Pts',(-24.2930763407555,-34.6897464310456,
4.28292314717365));
#17504=CARTESIAN_POINT('Ctrl Pts',(-24.486660664809,-35.1676910781175,5.2717730444337));
#17505=CARTESIAN_POINT('Ctrl Pts',(-24.7550996672026,-35.7691912190766,
6.16441400296898));
#17506=CARTESIAN_POINT('Origin',(-1.73472347597681E-15,-1.73472347597681E-15,
6.16441400296896));
#17507=CARTESIAN_POINT('Origin',(0.,0.,-6.93889390390723E-15));
#17508=CARTESIAN_POINT('',(-31.069725221506,-30.4453966086848,6.16441400296896));
#17509=CARTESIAN_POINT('',(-29.9666738162742,-28.7097276265211,0.));
#17510=CARTESIAN_POINT('Ctrl Pts',(-31.069725221506,-30.4453966086848,6.164414002969));
#17511=CARTESIAN_POINT('Ctrl Pts',(-30.6516652743934,-29.9507533455087,
5.27531660683074));
#17512=CARTESIAN_POINT('Ctrl Pts',(-30.3394714544404,-29.5533355526261,
4.29109868658259));
#17513=CARTESIAN_POINT('Ctrl Pts',(-29.9621423486912,-28.9647448012293,
2.19783870908461));
#17514=CARTESIAN_POINT('Ctrl Pts',(-29.899943054726,-28.7793799405673,1.10199792653053));
#17515=CARTESIAN_POINT('Ctrl Pts',(-29.9666738162742,-28.7097276265211,
1.11022302462516E-15));
#17516=CARTESIAN_POINT('',(-31.069609699158,-30.4455144995448,-6.16441400296898));
#17517=CARTESIAN_POINT('Ctrl Pts',(-31.0696096991579,-30.4455144995448,
-6.164414002969));
#17518=CARTESIAN_POINT('Ctrl Pts',(-30.6508754357951,-29.9509515767416,
-5.27472971793068));
#17519=CARTESIAN_POINT('Ctrl Pts',(-30.3397385395325,-29.5522200012418,
-4.28982003626194));
#17520=CARTESIAN_POINT('Ctrl Pts',(-29.9624407791487,-28.9641879146137,
-2.19678068845436));
#17521=CARTESIAN_POINT('Ctrl Pts',(-29.8990485823063,-28.7803135740586,
-1.10143126024342));
#17522=CARTESIAN_POINT('Ctrl Pts',(-29.9666738162742,-28.7097276265211,
-1.38777878078145E-15));
#17523=CARTESIAN_POINT('',(-29.5933299130507,-31.8823591451032,-6.16441400296901));
#17524=CARTESIAN_POINT('Origin',(-5.20417042793042E-15,1.73472347597681E-15,
-6.16441400296897));
#17525=CARTESIAN_POINT('',(-28.7097276265213,-29.9666738162741,0.));
#17526=CARTESIAN_POINT('Ctrl Pts',(-28.7097276265212,-29.9666738162741,
3.81639164714898E-16));
#17527=CARTESIAN_POINT('Ctrl Pts',(-28.7009453572214,-29.97508771503,-0.137043042104982));
#17528=CARTESIAN_POINT('Ctrl Pts',(-28.6939089066536,-29.9855335762034,
-0.273914065099642));
#17529=CARTESIAN_POINT('Ctrl Pts',(-28.6833041076052,-30.0105018835366,
-0.547624684008771));
#17530=CARTESIAN_POINT('Ctrl Pts',(-28.6797423147354,-30.0250211183715,
-0.684384502473487));
#17531=CARTESIAN_POINT('Ctrl Pts',(-28.674281049099,-30.0746701832321,-1.09422919239485));
#17532=CARTESIAN_POINT('Ctrl Pts',(-28.677621397945,-30.1158603964369,-1.36653715783935));
#17533=CARTESIAN_POINT('Ctrl Pts',(-28.7085066242031,-30.2635373474942,
-2.17926357855851));
#17534=CARTESIAN_POINT('Ctrl Pts',(-28.7569321746901,-30.3938552172152,
-2.71362913030275));
#17535=CARTESIAN_POINT('Ctrl Pts',(-28.9079875339794,-30.7170715388663,
-3.75949691623764));
#17536=CARTESIAN_POINT('Ctrl Pts',(-29.0106228201944,-30.9097255546857,
-4.26925519586596));
#17537=CARTESIAN_POINT('Ctrl Pts',(-29.2658165139508,-31.3541412178217,
-5.25006061967079));
#17538=CARTESIAN_POINT('Ctrl Pts',(-29.418042699661,-31.6049144758011,-5.71959225708859));
#17539=CARTESIAN_POINT('Ctrl Pts',(-29.5933299130507,-31.8823591451032,
-6.16441400296904));
#17540=CARTESIAN_POINT('',(-29.5936151100058,-31.8820944218042,6.16441400296897));
#17541=CARTESIAN_POINT('Ctrl Pts',(-28.7097276265212,-29.966673816274,0.));
#17542=CARTESIAN_POINT('Ctrl Pts',(-28.640288840658,-30.0332000060364,1.09861960926665));
#17543=CARTESIAN_POINT('Ctrl Pts',(-28.6817561949068,-30.2317815990284,
2.18971594132759));
#17544=CARTESIAN_POINT('Ctrl Pts',(-28.9826735044057,-30.8793896002663,
4.28292314717353));
#17545=CARTESIAN_POINT('Ctrl Pts',(-29.2423060343175,-31.3249195382003,
5.27177304443354));
#17546=CARTESIAN_POINT('Ctrl Pts',(-29.5936151100058,-31.8820944218042,
6.16441400296899));
#17547=CARTESIAN_POINT('Origin',(-1.73472347597681E-15,-1.73472347597681E-15,
6.16441400296896));
#17548=CARTESIAN_POINT('Origin',(0.,0.,-6.93889390390723E-15));
#17549=CARTESIAN_POINT('',(-35.0863119121265,-25.7138234497512,6.16441400296896));
#17550=CARTESIAN_POINT('',(-33.7474765292386,-24.1528016575407,0.));
#17551=CARTESIAN_POINT('Ctrl Pts',(-35.0863119121264,-25.7138234497512,
6.164414002969));
#17552=CARTESIAN_POINT('Ctrl Pts',(-34.602112136481,-25.2837110755395,5.27531660683076));
#17553=CARTESIAN_POINT('Ctrl Pts',(-34.2365375505477,-24.9347682357558,
4.29109868658263));
#17554=CARTESIAN_POINT('Ctrl Pts',(-33.7792839134372,-24.4058680201909,
2.19783870908452));
#17555=CARTESIAN_POINT('Ctrl Pts',(-33.691337548434,-24.2312417889978,1.10199792653034));
#17556=CARTESIAN_POINT('Ctrl Pts',(-33.7474765292385,-24.1528016575406,
2.77555756156289E-16));
#17557=CARTESIAN_POINT('',(-35.0862143432467,-25.7139565811984,-6.16441400296897));
#17558=CARTESIAN_POINT('Ctrl Pts',(-35.0862143432467,-25.7139565811983,
-6.164414002969));
#17559=CARTESIAN_POINT('Ctrl Pts',(-34.6013585485437,-25.2840196948202,
-5.27472971793046));
#17560=CARTESIAN_POINT('Ctrl Pts',(-34.2366431575829,-24.9336260289062,
-4.28982003626259));
#17561=CARTESIAN_POINT('Ctrl Pts',(-33.7795000530746,-24.4052743307777,
-2.19678068842248));
#17562=CARTESIAN_POINT('Ctrl Pts',(-33.6905850503741,-24.2322932161148,
-1.10143126006778));
#17563=CARTESIAN_POINT('Ctrl Pts',(-33.7474765292385,-24.1528016575406,
-1.94289029309402E-15));
#17564=CARTESIAN_POINT('',(-33.8294452700949,-27.3462727390344,-6.16441400296902));
#17565=CARTESIAN_POINT('Origin',(-5.20417042793042E-15,1.73472347597681E-15,
-6.16441400296897));
#17566=CARTESIAN_POINT('',(-32.6822063330435,-25.5758360411616,1.04083408558608E-14));
#17567=CARTESIAN_POINT('Ctrl Pts',(-32.6822063330434,-25.5758360411615,
1.35308431126191E-14));
#17568=CARTESIAN_POINT('Ctrl Pts',(-32.6747108772234,-25.5854141457942,
-0.137043042106718));
#17569=CARTESIAN_POINT('Ctrl Pts',(-32.6692326486208,-25.5967550744865,
-0.273914065103458));
#17570=CARTESIAN_POINT('Ctrl Pts',(-32.6622891517574,-25.6229784607124,
-0.547624684015696));
#17571=CARTESIAN_POINT('Ctrl Pts',(-32.6608299153614,-25.6378568066473,
-0.684384502481298));
#17572=CARTESIAN_POINT('Ctrl Pts',(-32.6624900361727,-25.6877777347498,
-1.09422919240422));
#17573=CARTESIAN_POINT('Ctrl Pts',(-32.6716583636155,-25.7280733097688,
-1.36653715784883));
#17574=CARTESIAN_POINT('Ctrl Pts',(-32.7232458442116,-25.8698516964151,
-2.17926357856531));
#17575=CARTESIAN_POINT('Ctrl Pts',(-32.7897246589715,-25.9919514437395,
-2.71362913030676));
#17576=CARTESIAN_POINT('Ctrl Pts',(-32.9852409710453,-26.2903804702531,
-3.7594969162393));
#17577=CARTESIAN_POINT('Ctrl Pts',(-33.1142491031337,-26.4664670218237,
-4.26925519586842));
#17578=CARTESIAN_POINT('Ctrl Pts',(-33.4300922362676,-26.8700413250523,
-5.25006061967152));
#17579=CARTESIAN_POINT('Ctrl Pts',(-33.6164577345519,-27.0965980278499,
-5.71959225708876));
#17580=CARTESIAN_POINT('Ctrl Pts',(-33.8294452700949,-27.3462727390344,
-6.16441400296905));
#17581=CARTESIAN_POINT('',(-33.829689890108,-27.345970122472,6.16441400296896));
#17582=CARTESIAN_POINT('Ctrl Pts',(-32.6822063330434,-25.5758360411615,
9.99200722162641E-15));
#17583=CARTESIAN_POINT('Ctrl Pts',(-32.6229419978348,-25.651567259815,1.09861960926662));
#17584=CARTESIAN_POINT('Ctrl Pts',(-32.692248381499,-25.8422261587078,2.18971594132752));
#17585=CARTESIAN_POINT('Ctrl Pts',(-33.0822670146348,-26.4404174460317,
4.28292314717354));
#17586=CARTESIAN_POINT('Ctrl Pts',(-33.4026623808143,-26.8444629700938,
5.27177304443356));
#17587=CARTESIAN_POINT('Ctrl Pts',(-33.829689890108,-27.345970122472,6.164414002969));
#17588=CARTESIAN_POINT('Origin',(-1.73472347597681E-15,-1.73472347597681E-15,
6.16441400296896));
#17589=CARTESIAN_POINT('Origin',(0.,0.,-6.93889390390723E-15));
#17590=CARTESIAN_POINT('',(-38.3886424727843,-20.4587909979242,6.16441400296896));
#17591=CARTESIAN_POINT('',(-36.8412779397535,-19.104194297741,3.46944695195361E-15));
#17592=CARTESIAN_POINT('Ctrl Pts',(-38.3886424727843,-20.4587909979242,
6.16441400296899));
#17593=CARTESIAN_POINT('Ctrl Pts',(-37.8481597797212,-20.101965360274,5.27531660683071));
#17594=CARTESIAN_POINT('Ctrl Pts',(-37.4366464721472,-19.8086009435392,
4.29109868658253));
#17595=CARTESIAN_POINT('Ctrl Pts',(-36.9087766691165,-19.3501581469729,
2.19783870908465));
#17596=CARTESIAN_POINT('Ctrl Pts',(-36.7968735674502,-19.1898254317353,
1.10199792653061));
#17597=CARTESIAN_POINT('Ctrl Pts',(-36.8412779397534,-19.1041942977409,
3.05311331771918E-15));
#17598=CARTESIAN_POINT('',(-38.3885648435901,-20.4589366597944,-6.16441400296897));
#17599=CARTESIAN_POINT('Ctrl Pts',(-38.3885648435901,-20.4589366597944,
-6.16441400296899));
#17600=CARTESIAN_POINT('Ctrl Pts',(-37.8474577833227,-20.1023780850071,
-5.27472971793101));
#17601=CARTESIAN_POINT('Ctrl Pts',(-37.4365884512732,-19.807455333257,-4.28982003626108));
#17602=CARTESIAN_POINT('Ctrl Pts',(-36.9089061179334,-19.3495397405838,
-2.19678068837342));
#17603=CARTESIAN_POINT('Ctrl Pts',(-36.796278362415,-19.1909732484813,-1.10143125981476));
#17604=CARTESIAN_POINT('Ctrl Pts',(-36.8412779397534,-19.1041942977409,
2.4980018054066E-15));
#17605=CARTESIAN_POINT('',(-37.37689067751,-22.2534950801323,-6.16441400296901));
#17606=CARTESIAN_POINT('Origin',(-5.20417042793042E-15,1.73472347597681E-15,
-6.16441400296897));
#17607=CARTESIAN_POINT('',(-35.9893695663252,-20.6643479988716,0.));
#17608=CARTESIAN_POINT('Ctrl Pts',(-35.9893695663251,-20.6643479988716,
2.46330733588707E-15));
#17609=CARTESIAN_POINT('Ctrl Pts',(-35.9833135098508,-20.6748953267903,
-0.137043042103492));
#17610=CARTESIAN_POINT('Ctrl Pts',(-35.9795050241501,-20.6869004543967,
-0.273914065100136));
#17611=CARTESIAN_POINT('Ctrl Pts',(-35.9763641790442,-20.7138450869921,
-0.547624684010087));
#17612=CARTESIAN_POINT('Ctrl Pts',(-35.9770372049667,-20.7287796638086,
-0.684384502474728));
#17613=CARTESIAN_POINT('Ctrl Pts',(-35.9857849169524,-20.7779562090156,
-1.09422919239792));
#17614=CARTESIAN_POINT('Ctrl Pts',(-36.0005945822839,-20.8165368441443,
-1.36653715784288));
#17615=CARTESIAN_POINT('Ctrl Pts',(-36.071834144877,-20.9495304672835,-2.17926357856208));
#17616=CARTESIAN_POINT('Ctrl Pts',(-36.15501290695,-21.0609264934646,-2.71362913030558));
#17617=CARTESIAN_POINT('Ctrl Pts',(-36.3910100235187,-21.3284930704613,
-3.75949691623798));
#17618=CARTESIAN_POINT('Ctrl Pts',(-36.5437647679417,-21.4844275433842,
-4.26925519586578));
#17619=CARTESIAN_POINT('Ctrl Pts',(-36.9138276850818,-21.8389448777016,
-5.25006061966817));
#17620=CARTESIAN_POINT('Ctrl Pts',(-37.1305386318308,-22.0366729841827,
-5.71959225708717));
#17621=CARTESIAN_POINT('Ctrl Pts',(-37.3768906775099,-22.2534950801323,
-6.16441400296905));
#17622=CARTESIAN_POINT('',(-37.3770897408172,-22.253160730712,6.16441400296896));
#17623=CARTESIAN_POINT('Ctrl Pts',(-35.9893695663251,-20.6643479988716,
-1.11022302462516E-15));
#17624=CARTESIAN_POINT('Ctrl Pts',(-35.9414861327318,-20.7477425771951,
1.09861960926678));
#17625=CARTESIAN_POINT('Ctrl Pts',(-36.0372206677032,-20.9265975166223,
2.18971594132783));
#17626=CARTESIAN_POINT('Ctrl Pts',(-36.508400969826,-21.4631946404635,4.28292314717348));
#17627=CARTESIAN_POINT('Ctrl Pts',(-36.8830368465616,-21.8175305489547,
5.27177304443343));
#17628=CARTESIAN_POINT('Ctrl Pts',(-37.3770897408172,-22.253160730712,6.16441400296898));
#17629=CARTESIAN_POINT('Origin',(-1.73472347597681E-15,-1.73472347597681E-15,
6.16441400296896));
#17630=CARTESIAN_POINT('Origin',(0.,0.,-6.93889390390723E-15));
#17631=CARTESIAN_POINT('',(-40.9094909763995,-14.7872765596607,6.16441400296896));
#17632=CARTESIAN_POINT('',(-39.1850971728874,-13.6666806339863,0.));
#17633=CARTESIAN_POINT('Ctrl Pts',(-40.9094909763995,-14.7872765596607,
6.16441400296899));
#17634=CARTESIAN_POINT('Ctrl Pts',(-40.3237280349261,-14.5110015995545,
5.27531660683078));
#17635=CARTESIAN_POINT('Ctrl Pts',(-39.8746532299474,-14.2791876594002,
4.29109868658268));
#17636=CARTESIAN_POINT('Ctrl Pts',(-39.2869131679351,-13.9005348551307,
2.19783870908458));
#17637=CARTESIAN_POINT('Ctrl Pts',(-39.1533313540539,-13.7577595675694,
1.10199792653047));
#17638=CARTESIAN_POINT('Ctrl Pts',(-39.1850971728874,-13.6666806339863,
5.55111512312578E-16));
#17639=CARTESIAN_POINT('',(-40.9094348672063,-14.7874317866831,-6.16441400296897));
#17640=CARTESIAN_POINT('Ctrl Pts',(-40.9094348672063,-14.7874317866831,
-6.16441400296899));
#17641=CARTESIAN_POINT('Ctrl Pts',(-40.3230919206938,-14.5115100278443,
-5.27472971793063));
#17642=CARTESIAN_POINT('Ctrl Pts',(-39.8744327623002,-14.2780619670101,
-4.28982003626127));
#17643=CARTESIAN_POINT('Ctrl Pts',(-39.2869532907287,-13.8999043207298,
-2.19678068831752));
#17644=CARTESIAN_POINT('Ctrl Pts',(-39.1529055587102,-13.7589804076816,
-1.10143125951959));
#17645=CARTESIAN_POINT('Ctrl Pts',(-39.1850971728874,-13.6666806339863,
-1.38777878078145E-15));
#17646=CARTESIAN_POINT('',(-40.1634503767788,-16.7077004351894,-6.16441400296902));
#17647=CARTESIAN_POINT('Origin',(-5.20417042793042E-15,1.73472347597681E-15,
-6.16441400296897));
#17648=CARTESIAN_POINT('',(-38.5638930200081,-15.3321934223834,0.));
#17649=CARTESIAN_POINT('Ctrl Pts',(-38.563893020008,-15.3321934223834,8.67361737988404E-16));
#17650=CARTESIAN_POINT('Ctrl Pts',(-38.5593996467226,-15.3434952604117,
-0.137043042096665));
#17651=CARTESIAN_POINT('Ctrl Pts',(-38.5573384337076,-15.3559201971581,
-0.273914065096707));
#17652=CARTESIAN_POINT('Ctrl Pts',(-38.5580641789047,-15.3830375611115,
-0.547624684006058));
#17653=CARTESIAN_POINT('Ctrl Pts',(-38.5608557662775,-15.397724343896,-0.684384502470298));
#17654=CARTESIAN_POINT('Ctrl Pts',(-38.5765129912447,-15.4451554135661,
-1.09422919239245));
#17655=CARTESIAN_POINT('Ctrl Pts',(-38.5966625123853,-15.481235718332,-1.36653715783741));
#17656=CARTESIAN_POINT('Ctrl Pts',(-38.6861039249185,-15.6027372113193,
-2.17926357855849));
#17657=CARTESIAN_POINT('Ctrl Pts',(-38.7842893545795,-15.7011618144977,
-2.71362913030383));
#17658=CARTESIAN_POINT('Ctrl Pts',(-39.0559630549181,-15.9324190580551,
-3.75949691623976));
#17659=CARTESIAN_POINT('Ctrl Pts',(-39.2293547655943,-16.0650270761305,
-4.26925519586824));
#17660=CARTESIAN_POINT('Ctrl Pts',(-39.646104052922,-16.3632704909573,-5.25006061967103));
#17661=CARTESIAN_POINT('Ctrl Pts',(-39.8887488381972,-16.5281448270819,
-5.71959225708847));
#17662=CARTESIAN_POINT('Ctrl Pts',(-40.1634503767788,-16.7077004351894,
-6.16441400296903));
#17663=CARTESIAN_POINT('',(-40.1635998310294,-16.707341159291,6.16441400296896));
#17664=CARTESIAN_POINT('Ctrl Pts',(-38.563893020008,-15.3321934223834,-1.38777878078145E-15));
#17665=CARTESIAN_POINT('Ctrl Pts',(-38.5283652566534,-15.4215536872524,
1.09861960926663));
#17666=CARTESIAN_POINT('Ctrl Pts',(-38.6485790638755,-15.584963696422,2.18971594132755));
#17667=CARTESIAN_POINT('Ctrl Pts',(-39.191329162806,-16.0490430867576,4.28292314717361));
#17668=CARTESIAN_POINT('Ctrl Pts',(-39.6125790440083,-16.3464561224017,
5.27177304443367));
#17669=CARTESIAN_POINT('Ctrl Pts',(-40.1635998310294,-16.707341159291,6.16441400296898));
#17670=CARTESIAN_POINT('Origin',(-1.73472347597681E-15,-1.73472347597681E-15,
6.16441400296896));
#17671=CARTESIAN_POINT('Origin',(0.,0.,-6.93889390390723E-15));
#17672=CARTESIAN_POINT('',(-42.5975402169652,-8.81473581362673,6.16441400296896));
#17673=CARTESIAN_POINT('',(-40.7312208280702,-7.95095276397609,0.));
#17674=CARTESIAN_POINT('Ctrl Pts',(-42.5975458454602,-8.81473754185287,
6.16442208586936));
#17675=CARTESIAN_POINT('Ctrl Pts',(-41.9784270998641,-8.62463742076724,
5.27532468973115));
#17676=CARTESIAN_POINT('Ctrl Pts',(-41.5009270369901,-8.45909129229262,
4.29109868658267));
#17677=CARTESIAN_POINT('Ctrl Pts',(-40.8652814087566,-8.1679367594703,2.19783870908461));
#17678=CARTESIAN_POINT('Ctrl Pts',(-40.712740223173,-8.04562539271016,1.10199792653052));
#17679=CARTESIAN_POINT('Ctrl Pts',(-40.7312208280702,-7.95095276397607,
5.55111512312578E-16));
#17680=CARTESIAN_POINT('',(-42.5975067699919,-8.81489744582999,-6.16441400296896));
#17681=CARTESIAN_POINT('Ctrl Pts',(-42.5975067699918,-8.81489744582997,
-6.16441400296899));
#17682=CARTESIAN_POINT('Ctrl Pts',(-41.9778641887521,-8.62522947425753,
-5.27472971793024));
#17683=CARTESIAN_POINT('Ctrl Pts',(-41.5005486106554,-8.45800843364591,
-4.28982003626188));
#17684=CARTESIAN_POINT('Ctrl Pts',(-40.8652313887449,-8.16730693291995,
-2.19678068827478));
#17685=CARTESIAN_POINT('Ctrl Pts',(-40.7124925054799,-8.04689440340105,
-1.10143125929045));
#17686=CARTESIAN_POINT('Ctrl Pts',(-40.7312208280702,-7.95095276397607,
-1.38777878078145E-15));
#17687=CARTESIAN_POINT('',(-42.1323980482118,-10.8217851903945,-6.16441400296901));
#17688=CARTESIAN_POINT('Origin',(-5.20417042793042E-15,1.73472347597681E-15,
-6.16441400296897));
#17689=CARTESIAN_POINT('',(-40.3533668208877,-9.68791960221017,1.04083408558608E-14));
#17690=CARTESIAN_POINT('Ctrl Pts',(-40.3533668208876,-9.68791960221017,
1.2038980923279E-14));
#17691=CARTESIAN_POINT('Ctrl Pts',(-40.3505276029147,-9.69974587751488,
-0.137043042091313));
#17692=CARTESIAN_POINT('Ctrl Pts',(-40.3502556229396,-9.71233768751765,
-0.273914065097098));
#17693=CARTESIAN_POINT('Ctrl Pts',(-40.3548331843628,-9.73907575149574,
-0.547624684009998));
#17694=CARTESIAN_POINT('Ctrl Pts',(-40.3596865045181,-9.75321575970265,
-0.684384502475249));
#17695=CARTESIAN_POINT('Ctrl Pts',(-40.3819345065204,-9.79793579403437,
-1.09422919239669));
#17696=CARTESIAN_POINT('Ctrl Pts',(-40.4070136973265,-9.8307812774791,-1.36653715784155));
#17697=CARTESIAN_POINT('Ctrl Pts',(-40.5128361905684,-9.93831722029971,
-2.17926357856093));
#17698=CARTESIAN_POINT('Ctrl Pts',(-40.62402951561,-10.0217667593921,-2.7136291303046));
#17699=CARTESIAN_POINT('Ctrl Pts',(-40.9258493066162,-10.2120069389282,
-3.75949691623883));
#17700=CARTESIAN_POINT('Ctrl Pts',(-41.1163482283345,-10.3185889853199,
-4.26925519586717));
#17701=CARTESIAN_POINT('Ctrl Pts',(-41.5713000721685,-10.5544871047827,
-5.25006061967));
#17702=CARTESIAN_POINT('Ctrl Pts',(-41.8349391478766,-10.6831513045169,
-5.71959225708799));
#17703=CARTESIAN_POINT('Ctrl Pts',(-42.1323980482118,-10.8217851903945,
-6.16441400296903));
#17704=CARTESIAN_POINT('',(-42.1324948509394,-10.8214083018602,6.16441400296896));
#17705=CARTESIAN_POINT('Ctrl Pts',(-40.3533668208876,-9.68791960221018,
8.60422844084496E-15));
#17706=CARTESIAN_POINT('Ctrl Pts',(-40.33091797058,-9.78142643632573,1.09861960926666));
#17707=CARTESIAN_POINT('Ctrl Pts',(-40.4731638436058,-9.92606495868674,
2.18971594132761));
#17708=CARTESIAN_POINT('Ctrl Pts',(-41.0764349124918,-10.3081792974238,
4.2829231471735));
#17709=CARTESIAN_POINT('Ctrl Pts',(-41.5357233653636,-10.5426149884832,
5.27177304443348));
#17710=CARTESIAN_POINT('Ctrl Pts',(-42.1324948509394,-10.8214083018602,
6.16441400296899));
#17711=CARTESIAN_POINT('Origin',(-1.73472347597681E-15,-1.73472347597681E-15,
6.16441400296896));
#17712=CARTESIAN_POINT('Origin',(0.,0.,-6.93889390390723E-15));
#17713=CARTESIAN_POINT('',(-43.4184263798756,-2.66275246602631,6.16441400296896));
#17714=CARTESIAN_POINT('',(-41.448174286335,-2.0733664243457,0.));
#17715=CARTESIAN_POINT('Ctrl Pts',(-43.4184263798755,-2.66275246602631,
6.16441400296899));
#17716=CARTESIAN_POINT('Ctrl Pts',(-42.7785553024261,-2.56269707422304,
5.27531660683071));
#17717=CARTESIAN_POINT('Ctrl Pts',(-42.2823616483505,-2.46679222047884,
4.29109868658253));
#17718=CARTESIAN_POINT('Ctrl Pts',(-41.611750365836,-2.26906302577168,2.19783870908463));
#17719=CARTESIAN_POINT('Ctrl Pts',(-41.4433551071959,-2.16970548652307,
1.10199792653057));
#17720=CARTESIAN_POINT('Ctrl Pts',(-41.4481742863349,-2.07336642434569,
1.11022302462516E-15));
#17721=CARTESIAN_POINT('',(-43.4184162760053,-2.66291721304384,-6.16441400296897));
#17722=CARTESIAN_POINT('Ctrl Pts',(-43.4184220936431,-2.66291811752308,
-6.16442208610002));
#17723=CARTESIAN_POINT('Ctrl Pts',(-42.7780940137297,-2.56336502615921,
-5.27473780106136));
#17724=CARTESIAN_POINT('Ctrl Pts',(-42.2818329669972,-2.46577423945546,
-4.28982003626243));
#17725=CARTESIAN_POINT('Ctrl Pts',(-41.6116112212699,-2.26844672853033,
-2.19678068820493));
#17726=CARTESIAN_POINT('Ctrl Pts',(-41.4432905099648,-2.17099683438165,
-1.10143125891921));
#17727=CARTESIAN_POINT('Ctrl Pts',(-41.4481742863349,-2.07336642434569,
2.77555756156289E-16));
#17728=CARTESIAN_POINT('',(-43.2436515951817,-4.7155696065853,-6.16441400296901));
#17729=CARTESIAN_POINT('Origin',(-5.20417042793042E-15,1.73472347597681E-15,
-6.16441400296897));
#17730=CARTESIAN_POINT('',(-41.3213624427943,-3.84642767658903,0.));
#17731=CARTESIAN_POINT('Ctrl Pts',(-41.3213624427943,-3.84642767658904,
1.83880688453542E-15));
#17732=CARTESIAN_POINT('Ctrl Pts',(-41.320235178424,-3.85853764030828,-0.137043042087949));
#17733=CARTESIAN_POINT('Ctrl Pts',(-41.3217579682172,-3.87103999062632,
-0.27391406509514));
#17734=CARTESIAN_POINT('Ctrl Pts',(-41.3300941599161,-3.89685444475066,
-0.547624684006307));
#17735=CARTESIAN_POINT('Ctrl Pts',(-41.3369104132512,-3.91015982858841,
-0.684384502470434));
#17736=CARTESIAN_POINT('Ctrl Pts',(-41.3652962871257,-3.95125845664314,
-1.09422919239298));
#17737=CARTESIAN_POINT('Ctrl Pts',(-41.3947946075951,-3.98020047944156,
-1.36653715783799));
#17738=CARTESIAN_POINT('Ctrl Pts',(-41.5148439407502,-4.07158175040666,
-2.17926357855872));
#17739=CARTESIAN_POINT('Ctrl Pts',(-41.6367815857305,-4.13835743344657,
-2.71362913030384));
#17740=CARTESIAN_POINT('Ctrl Pts',(-41.9626032868359,-4.28370780751825,
-3.7594969162383));
#17741=CARTESIAN_POINT('Ctrl Pts',(-42.1663314109023,-4.36209417912445,
-4.26925519586628));
#17742=CARTESIAN_POINT('Ctrl Pts',(-42.6502243036723,-4.53084479779167,
-5.25006061966883));
#17743=CARTESIAN_POINT('Ctrl Pts',(-42.9294907385031,-4.62067962906769,
-5.71959225708739));
#17744=CARTESIAN_POINT('Ctrl Pts',(-43.2436515951816,-4.7155696065853,-6.16441400296904));
#17745=CARTESIAN_POINT('',(-43.2436937757663,-4.71518277776806,6.16441400296896));
#17746=CARTESIAN_POINT('Ctrl Pts',(-41.3213624427943,-3.84642767658904,
-8.32667268468867E-16));
#17747=CARTESIAN_POINT('Ctrl Pts',(-41.3124494993889,-3.94217755045996,
1.09861960926659));
#17748=CARTESIAN_POINT('Ctrl Pts',(-41.4738317224467,-4.06510016280015,
2.18971594132748));
#17749=CARTESIAN_POINT('Ctrl Pts',(-42.1253429020158,-4.3574707039288,4.28292314717357));
#17750=CARTESIAN_POINT('Ctrl Pts',(-42.6133201381353,-4.5241566157904,5.2717730444336));
#17751=CARTESIAN_POINT('Ctrl Pts',(-43.2436937757662,-4.71518277776806,
6.16441400296899));
#17752=CARTESIAN_POINT('Origin',(-1.73472347597681E-15,-1.73472347597681E-15,
6.16441400296896));
#17753=CARTESIAN_POINT('Origin',(0.,0.,-6.93889390390723E-15));
#17754=CARTESIAN_POINT('',(-43.3554385900939,3.54343684303835,6.16441400296897));
#17755=CARTESIAN_POINT('',(-41.3213624427943,3.84642767658933,0.));
#17756=CARTESIAN_POINT('Ctrl Pts',(-43.3554444774928,3.54343677054778,6.16442208586936));
#17757=CARTESIAN_POINT('Ctrl Pts',(-42.7078469980911,3.55141059382748,5.27532468973115));
#17758=CARTESIAN_POINT('Ctrl Pts',(-42.2030493088126,3.57572362730252,4.2910986865827));
#17759=CARTESIAN_POINT('Ctrl Pts',(-41.5111240838457,3.67600228769425,2.19783870908447));
#17760=CARTESIAN_POINT('Ctrl Pts',(-41.3303027940033,3.7503833664557,1.10199792653022));
#17761=CARTESIAN_POINT('Ctrl Pts',(-41.3213624427943,3.84642767658933,1.94289029309402E-15));
#17762=CARTESIAN_POINT('',(-43.3554520350115,3.54327233497867,-6.16441400296897));
#17763=CARTESIAN_POINT('Ctrl Pts',(-43.3554579221549,3.54327226764192,-6.16442208610002));
#17764=CARTESIAN_POINT('Ctrl Pts',(-42.707479577098,3.55068386494164,-5.27473780157895));
#17765=CARTESIAN_POINT('Ctrl Pts',(-42.2023811354534,3.57665600751496,-4.28982003740415));
#17766=CARTESIAN_POINT('Ctrl Pts',(-41.6842000357502,3.65154612751076,-2.72134440716138));
#17767=CARTESIAN_POINT('Ctrl Pts',(-41.5522083575935,3.68232228947575,-2.18467279509217));
#17768=CARTESIAN_POINT('Ctrl Pts',(-41.4177402491549,3.73728328257893,-1.36905841490162));
#17769=CARTESIAN_POINT('Ctrl Pts',(-41.3835568404079,3.75703193749213,-1.09600303224686));
#17770=CARTESIAN_POINT('Ctrl Pts',(-41.3482537456227,3.78889147274118,-0.685230045226319));
#17771=CARTESIAN_POINT('Ctrl Pts',(-41.3391520617229,3.79987407882911,-0.548230322281482));
#17772=CARTESIAN_POINT('Ctrl Pts',(-41.3262690897369,3.82259220036053,-0.274077591980457));
#17773=CARTESIAN_POINT('Ctrl Pts',(-41.322489517709,3.83431974815085,-0.137016510473668));
#17774=CARTESIAN_POINT('Ctrl Pts',(-41.3213624427943,3.84642767658934,-1.66533453693773E-15));
#17775=CARTESIAN_POINT('',(-43.4745891000669,1.48664137583784,-6.16441400296901));
#17776=CARTESIAN_POINT('Origin',(-5.20417042793042E-15,1.73472347597681E-15,
-6.16441400296897));
#17777=CARTESIAN_POINT('',(-41.4481742863349,2.07336642434601,0.));
#17778=CARTESIAN_POINT('Ctrl Pts',(-41.4481742863349,2.07336642434599,1.2490009027033E-15));
#17779=CARTESIAN_POINT('Ctrl Pts',(-41.4487819234188,2.06121929614942,-0.137043042079584));
#17780=CARTESIAN_POINT('Ctrl Pts',(-41.452068483371,2.04906091731251,-0.273914065091576));
#17781=CARTESIAN_POINT('Ctrl Pts',(-41.4639936045221,2.0246955808817,-0.547624684002258));
#17782=CARTESIAN_POINT('Ctrl Pts',(-41.4726340317754,2.01249568065706,-0.68438450246554));
#17783=CARTESIAN_POINT('Ctrl Pts',(-41.5065799229875,1.97585510842473,-1.09422919238728));
#17784=CARTESIAN_POINT('Ctrl Pts',(-41.5398968723813,1.95140572239379,-1.36653715783194));
#17785=CARTESIAN_POINT('Ctrl Pts',(-41.67172918722,1.87803938243819,-2.17926357855389));
#17786=CARTESIAN_POINT('Ctrl Pts',(-41.8019288533266,1.82929691579476,-2.71362913030093));
#17787=CARTESIAN_POINT('Ctrl Pts',(-42.1451196742907,1.73179526165578,-3.75949691623917));
#17788=CARTESIAN_POINT('Ctrl Pts',(-42.3579296836043,1.68320028532058,-4.2692551958683));
#17789=CARTESIAN_POINT('Ctrl Pts',(-42.8609129614465,1.58503244341179,-5.25006061967115));
#17790=CARTESIAN_POINT('Ctrl Pts',(-43.1501216961234,1.535855758695,-5.71959225708858));
#17791=CARTESIAN_POINT('Ctrl Pts',(-43.4745891000668,1.48664137583782,-6.16441400296904));
#17792=CARTESIAN_POINT('',(-43.4745757998335,1.48703027021514,6.16441400296896));
#17793=CARTESIAN_POINT('Ctrl Pts',(-41.4481742863349,2.07336642434599,-2.77555756156289E-16));
#17794=CARTESIAN_POINT('Ctrl Pts',(-41.4529786916566,1.97732270203186,1.09861960926673));
#17795=CARTESIAN_POINT('Ctrl Pts',(-41.6302119880731,1.87861834962018,2.18971594132774));
#17796=CARTESIAN_POINT('Ctrl Pts',(-42.3167003895122,1.68194342719036,4.28292314717356));
#17797=CARTESIAN_POINT('Ctrl Pts',(-42.8234325995621,1.58640053900966,5.27177304443357));
#17798=CARTESIAN_POINT('Ctrl Pts',(-43.4745757998335,1.48703027021513,6.16441400296899));
#17799=CARTESIAN_POINT('Origin',(-1.73472347597681E-15,-1.73472347597681E-15,
6.16441400296896));
#17800=CARTESIAN_POINT('Origin',(0.,0.,-6.93889390390723E-15));
#17801=CARTESIAN_POINT('',(-42.4098590973784,9.67749199640682,6.16441400296896));
#17802=CARTESIAN_POINT('',(-40.3533668208876,9.68791960221045,0.));
#17803=CARTESIAN_POINT('Ctrl Pts',(-42.4098649351686,9.67749276251832,6.16442208586937));
#17804=CARTESIAN_POINT('Ctrl Pts',(-41.7677242709781,9.59322269322707,5.27532468973104));
#17805=CARTESIAN_POINT('Ctrl Pts',(-41.2646045888914,9.54544805356745,4.29109868658242));
#17806=CARTESIAN_POINT('Ctrl Pts',(-40.5654510237052,9.54623479529791,2.19783870908471));
#17807=CARTESIAN_POINT('Ctrl Pts',(-40.375884702676,9.59412522930591,1.10199792653074));
#17808=CARTESIAN_POINT('Ctrl Pts',(-40.3533668208875,9.68791960221046,8.32667268468867E-16));
#17809=CARTESIAN_POINT('',(-42.4098958173841,9.67733107621259,-6.16441400296897));
#17810=CARTESIAN_POINT('Ctrl Pts',(-42.4098958173841,9.6773310762126,-6.164414002969));
#17811=CARTESIAN_POINT('Ctrl Pts',(-41.7674581769275,9.59245030070757,-5.27472971793047));
#17812=CARTESIAN_POINT('Ctrl Pts',(-41.263810524451,9.54627585245725,-4.28982003626203));
#17813=CARTESIAN_POINT('Ctrl Pts',(-40.5651438845123,9.54678692661234,-2.19678068831686));
#17814=CARTESIAN_POINT('Ctrl Pts',(-40.3761865368333,9.59286799091328,-1.1014312595142));
#17815=CARTESIAN_POINT('Ctrl Pts',(-40.3533668208875,9.68791960221045,-2.77555756156289E-16));
#17816=CARTESIAN_POINT('',(-42.8205093412364,7.65858862696565,-6.16441400296902));
#17817=CARTESIAN_POINT('Origin',(-5.20417042793042E-15,1.73472347597681E-15,
-6.16441400296897));
#17818=CARTESIAN_POINT('',(-40.7312208280702,7.95095276397637,0.));
#17819=CARTESIAN_POINT('Ctrl Pts',(-40.7312208280702,7.95095276397635,1.66533453693773E-15));
#17820=CARTESIAN_POINT('Ctrl Pts',(-40.7499114176564,7.85520442356475,-1.0992402164504));
#17821=CARTESIAN_POINT('Ctrl Pts',(-40.939440247702,7.78353023681697,-2.19104319733171));
#17822=CARTESIAN_POINT('Ctrl Pts',(-41.4696829608985,7.71204397345954,-3.75949691436094));
#17823=CARTESIAN_POINT('Ctrl Pts',(-41.6872426574349,7.69422964594872,-4.26925519440169));
#17824=CARTESIAN_POINT('Ctrl Pts',(-42.1990770315599,7.66864299493069,-5.25006061898242));
#17825=CARTESIAN_POINT('Ctrl Pts',(-42.4923406104441,7.66112555225126,-5.7195922567623));
#17826=CARTESIAN_POINT('Ctrl Pts',(-42.8205093412364,7.65858862696564,-6.16441400296903));
#17827=CARTESIAN_POINT('',(-42.82044083094,7.65897167013792,6.16441400296897));
#17828=CARTESIAN_POINT('Ctrl Pts',(-40.7312208280702,7.95095276397636,0.));
#17829=CARTESIAN_POINT('Ctrl Pts',(-40.7496447782814,7.85657036643813,1.09861960926664));
#17830=CARTESIAN_POINT('Ctrl Pts',(-40.9391211892399,7.78409360993022,2.18971594132758));
#17831=CARTESIAN_POINT('Ctrl Pts',(-41.646611888365,7.68711804045621,4.28292314717358));
#17832=CARTESIAN_POINT('Ctrl Pts',(-42.1617834658437,7.66466315363683,5.27177304443359));
#17833=CARTESIAN_POINT('Ctrl Pts',(-42.8204408309399,7.6589716701379,6.16441400296898));
#17834=CARTESIAN_POINT('Origin',(-1.73472347597681E-15,-1.73472347597681E-15,
6.16441400296896));
#17835=CARTESIAN_POINT('Origin',(0.,0.,-6.93889390390723E-15));
#17836=CARTESIAN_POINT('',(-40.6009371733746,15.6145413203108,6.16441400296896));
#17837=CARTESIAN_POINT('',(-38.563893020008,15.3321934223837,0.));
#17838=CARTESIAN_POINT('Ctrl Pts',(-40.6009428427155,15.6145429094286,6.16442208586937));
#17839=CARTESIAN_POINT('Ctrl Pts',(-39.9773311258786,15.4397444431623,5.27532468973107));
#17840=CARTESIAN_POINT('Ctrl Pts',(-39.4861315168336,15.3208546842608,4.29109868658248));
#17841=CARTESIAN_POINT('Ctrl Pts',(-38.7939823618226,15.2221334915372,2.19783870908464));
#17842=CARTESIAN_POINT('Ctrl Pts',(-38.5995300332387,15.24255836966,1.1019979265306));
#17843=CARTESIAN_POINT('Ctrl Pts',(-38.5638930200079,15.3321934223837,2.77555756156289E-15));
#17844=CARTESIAN_POINT('',(-40.6009964209562,15.6143872638508,-6.16441400296897));
#17845=CARTESIAN_POINT('Ctrl Pts',(-40.6010020885999,15.6143888578416,-6.16442208610002));
#17846=CARTESIAN_POINT('Ctrl Pts',(-39.9772648207974,15.4389665558936,-5.27485402124692));
#17847=CARTESIAN_POINT('Ctrl Pts',(-39.4853557749724,15.3215914526481,-4.29007656912573));
#17848=CARTESIAN_POINT('Ctrl Pts',(-38.7936501568704,15.2226313606678,-2.19706468916282));
#17849=CARTESIAN_POINT('Ctrl Pts',(-38.60001241506,15.2413450715728,-1.10157448566469));
#17850=CARTESIAN_POINT('Ctrl Pts',(-38.5638930200079,15.3321934223837,5.55111512312578E-16));
#17851=CARTESIAN_POINT('',(-41.2947274963707,13.6746290991927,-6.16441400296902));
#17852=CARTESIAN_POINT('Origin',(-5.20417042793042E-15,1.73472347597681E-15,
-6.16441400296897));
#17853=CARTESIAN_POINT('',(-39.1850971728873,13.6666806339866,0.));
#17854=CARTESIAN_POINT('Ctrl Pts',(-39.1850971728873,13.6666806339865,2.08166817117217E-15));
#17855=CARTESIAN_POINT('Ctrl Pts',(-39.189102437885,13.6551967409812,-0.137043042091231));
#17856=CARTESIAN_POINT('Ctrl Pts',(-39.195681280223,13.6444567928563,-0.273914065094698));
#17857=CARTESIAN_POINT('Ctrl Pts',(-39.2139878587076,13.6244381186245,-0.547624684004344));
#17858=CARTESIAN_POINT('Ctrl Pts',(-39.2257153970297,13.6151666897426,-0.684384502468343));
#17859=CARTESIAN_POINT('Ctrl Pts',(-39.2686090832299,13.5895739808625,-1.0942291923894));
#17860=CARTESIAN_POINT('Ctrl Pts',(-39.3074646501152,13.5755014360956,-1.36653715783395));
#17861=CARTESIAN_POINT('Ctrl Pts',(-39.4546265164404,13.5422484035419,-2.17926357855595));
#17862=CARTESIAN_POINT('Ctrl Pts',(-39.593284520991,13.5321618341122,-2.71362913030224));
#17863=CARTESIAN_POINT('Ctrl Pts',(-39.9500430926314,13.5352977095237,-3.75949691623775));
#17864=CARTESIAN_POINT('Ctrl Pts',(-40.1679235882143,13.5486266792222,-4.26925519586518));
#17865=CARTESIAN_POINT('Ctrl Pts',(-40.6781895862499,13.5961420895901,-5.25006061966842));
#17866=CARTESIAN_POINT('Ctrl Pts',(-40.9695380082035,13.6304369224201,-5.71959225708742));
#17867=CARTESIAN_POINT('Ctrl Pts',(-41.2947274963707,13.6746290991927,-6.16441400296904));
#17868=CARTESIAN_POINT('',(-41.2946051706828,13.6749984935072,6.16441400296896));
#17869=CARTESIAN_POINT('Ctrl Pts',(-39.1850971728873,13.6666806339865,-8.32667268468867E-16));
#17870=CARTESIAN_POINT('Ctrl Pts',(-39.2167656094919,13.5758809146617,1.09861960926663));
#17871=CARTESIAN_POINT('Ctrl Pts',(-39.4146279416703,13.5311071718144,2.18971594132755));
#17872=CARTESIAN_POINT('Ctrl Pts',(-40.1287184680819,13.5358050982362,4.2829231471736));
#17873=CARTESIAN_POINT('Ctrl Pts',(-40.6418420053041,13.5868953295193,5.27177304443364));
#17874=CARTESIAN_POINT('Ctrl Pts',(-41.2946051706828,13.6749984935071,6.16441400296898));
#17875=CARTESIAN_POINT('Origin',(-1.73472347597681E-15,-1.73472347597681E-15,
6.16441400296896));
#17876=CARTESIAN_POINT('Origin',(0.,0.,-6.93889390390723E-15));
#17877=CARTESIAN_POINT('',(-37.9654972519552,21.2337236115521,6.16441400296896));
#17878=CARTESIAN_POINT('',(-35.989369566325,20.6643479988719,0.));
#17879=CARTESIAN_POINT('Ctrl Pts',(-37.9654972519552,21.2337236115521,6.16441400296898));
#17880=CARTESIAN_POINT('Ctrl Pts',(-37.373109418679,20.9719551410069,5.27531660683082));
#17881=CARTESIAN_POINT('Ctrl Pts',(-36.9038346756933,20.7843728952792,4.2910986865828));
#17882=CARTESIAN_POINT('Ctrl Pts',(-36.2327800916601,20.5881534468968,2.19783870908457));
#17883=CARTESIAN_POINT('Ctrl Pts',(-36.0374002441774,20.5806969775163,1.10199792653046));
#17884=CARTESIAN_POINT('Ctrl Pts',(-35.989369566325,20.6643479988719,1.66533453693773E-15));
#17885=CARTESIAN_POINT('',(-37.9655778209999,21.2335795549786,-6.16441400296897));
#17886=CARTESIAN_POINT('Ctrl Pts',(-37.9655778209998,21.2335795549787,-6.164414002969));
#17887=CARTESIAN_POINT('Ctrl Pts',(-37.3731544963908,20.9711757310147,-5.27484593906402));
#17888=CARTESIAN_POINT('Ctrl Pts',(-36.9029619776899,20.7849917652438,-4.29007657121778));
#17889=CARTESIAN_POINT('Ctrl Pts',(-36.2323804143448,20.5885989707591,-2.19706469153212));
#17890=CARTESIAN_POINT('Ctrl Pts',(-36.0380503864369,20.5795646790257,-1.10157448711653));
#17891=CARTESIAN_POINT('Ctrl Pts',(-35.989369566325,20.6643479988719,-2.4980018054066E-15));
#17892=CARTESIAN_POINT('',(-38.92830408384,19.4122935573335,-6.16441400296897));
#17893=CARTESIAN_POINT('Origin',(-5.20417042793042E-15,1.73472347597681E-15,
-6.16441400296897));
#17894=CARTESIAN_POINT('',(-36.8412779397533,19.1041942977412,0.));
#17895=CARTESIAN_POINT('Ctrl Pts',(-36.8412779397533,19.1041942977412,1.56125112837913E-15));
#17896=CARTESIAN_POINT('Ctrl Pts',(-36.8468754499426,19.0933998394437,-0.137010845862136));
#17897=CARTESIAN_POINT('Ctrl Pts',(-36.85491331931,19.0837074965195,-0.273849719843199));
#17898=CARTESIAN_POINT('Ctrl Pts',(-36.8758752981302,19.0665008944353,-0.547496131370911));
#17899=CARTESIAN_POINT('Ctrl Pts',(-36.8887981733475,19.0589938273842,-0.684223919463285));
#17900=CARTESIAN_POINT('Ctrl Pts',(-36.9348797930799,19.0397674368009,-1.09397285881179));
#17901=CARTESIAN_POINT('Ctrl Pts',(-36.9753262536641,19.0313667108818,-1.36621764183654));
#17902=CARTESIAN_POINT('Ctrl Pts',(-37.1256601264042,19.0193858351339,-2.17875768610691));
#17903=CARTESIAN_POINT('Ctrl Pts',(-37.2642828595668,19.0291203079234,-2.71300426677318));
#17904=CARTESIAN_POINT('Ctrl Pts',(-37.6168941909717,19.082964194744,-3.75889728641727));
#17905=CARTESIAN_POINT('Ctrl Pts',(-37.8306847292239,19.127164138192,-4.26878718251841));
#17906=CARTESIAN_POINT('Ctrl Pts',(-38.3290788364577,19.2468276666523,-5.24984087225394));
#17907=CARTESIAN_POINT('Ctrl Pts',(-38.6126451863175,19.32225227825,-5.71949644942051));
#17908=CARTESIAN_POINT('Ctrl Pts',(-38.9283097929753,19.4122951858561,-6.1644220499366));
#17909=CARTESIAN_POINT('',(-38.9281304329582,19.4126417829877,6.16441400296896));
#17910=CARTESIAN_POINT('Ctrl Pts',(-36.8412779397533,19.1041942977412,-1.11022302462516E-15));
#17911=CARTESIAN_POINT('Ctrl Pts',(-36.8855461847064,19.0188256770705,1.09861960926665));
#17912=CARTESIAN_POINT('Ctrl Pts',(-37.0877665316094,19.0026664121713,2.18971594132759));
#17913=CARTESIAN_POINT('Ctrl Pts',(-37.7939200614566,19.1089421982548,4.28292314717358));
#17914=CARTESIAN_POINT('Ctrl Pts',(-38.2945498429305,19.2325374978634,5.27177304443359));
#17915=CARTESIAN_POINT('Ctrl Pts',(-38.9281304329581,19.4126417829877,6.16441400296898));
#17916=CARTESIAN_POINT('Origin',(-1.73472347597681E-15,-1.73472347597681E-15,
6.16441400296896));
#17917=CARTESIAN_POINT('Origin',(0.,0.,-6.93889390390723E-15));
#17918=CARTESIAN_POINT('',(-34.5571892899392,26.4206485230646,6.16441400296896));
#17919=CARTESIAN_POINT('',(-32.6822063330433,25.5758360411618,0.));
#17920=CARTESIAN_POINT('Ctrl Pts',(-34.5571892899392,26.4206485230645,6.16441400296899));
#17921=CARTESIAN_POINT('Ctrl Pts',(-34.0080846482037,26.0772388994228,5.27531660683079));
#17922=CARTESIAN_POINT('Ctrl Pts',(-33.570282182427,25.8247812113316,4.29109868658273));
#17923=CARTESIAN_POINT('Ctrl Pts',(-32.9339829055411,25.5350579694094,2.19783870908454));
#17924=CARTESIAN_POINT('Ctrl Pts',(-32.7416529094252,25.4998719447395,1.10199792653037));
#17925=CARTESIAN_POINT('Ctrl Pts',(-32.6822063330432,25.5758360411618,2.22044604925031E-15));
#17926=CARTESIAN_POINT('',(-34.5572895403017,26.4205173989413,-6.16441400296897));
#17927=CARTESIAN_POINT('Ctrl Pts',(-34.5572895403017,26.4205173989413,-6.16441400296899));
#17928=CARTESIAN_POINT('Ctrl Pts',(-34.0082401881207,26.0764738375471,-5.27484593811451));
#17929=CARTESIAN_POINT('Ctrl Pts',(-33.5693302919162,25.8252695836891,-4.29007656912472));
#17930=CARTESIAN_POINT('Ctrl Pts',(-32.9335238913029,25.5354420784063,-2.19706468924495));
#17931=CARTESIAN_POINT('Ctrl Pts',(-32.7424575770002,25.4988436963698,-1.10157448610462));
#17932=CARTESIAN_POINT('Ctrl Pts',(-32.6822063330432,25.5758360411618,-2.22044604925031E-15));
#17933=CARTESIAN_POINT('',(-35.7694126601179,24.7547796990844,-6.16441400296897));
#17934=CARTESIAN_POINT('Origin',(-5.20417042793042E-15,1.73472347597681E-15,
-6.16441400296897));
#17935=CARTESIAN_POINT('',(-33.7474765292384,24.1528016575409,0.));
#17936=CARTESIAN_POINT('Ctrl Pts',(-33.7474765292383,24.1528016575408,1.59594559789866E-15));
#17937=CARTESIAN_POINT('Ctrl Pts',(-33.7545532764259,24.14291368003,-0.137010845725497));
#17938=CARTESIAN_POINT('Ctrl Pts',(-33.7638886960774,24.1344638992668,-0.273849719561638));
#17939=CARTESIAN_POINT('Ctrl Pts',(-33.7870860669391,24.1204156362138,-0.547496130807132));
#17940=CARTESIAN_POINT('Ctrl Pts',(-33.8009457729327,24.114824097178,-0.684223918759467));
#17941=CARTESIAN_POINT('Ctrl Pts',(-33.8492945488111,24.102351501781,-1.09397285769029));
#17942=CARTESIAN_POINT('Ctrl Pts',(-33.8905248706266,24.0997924146199,-1.3662176404398));
#17943=CARTESIAN_POINT('Ctrl Pts',(-34.0410336174364,24.1093282276174,-2.17875768389756));
#17944=CARTESIAN_POINT('Ctrl Pts',(-34.1768600108832,24.1386916892626,-2.7130042640453));
#17945=CARTESIAN_POINT('Ctrl Pts',(-34.5182194830287,24.2421693473779,-3.75889728380116));
#17946=CARTESIAN_POINT('Ctrl Pts',(-34.7235436341634,24.3163449650229,-4.268787180477));
#17947=CARTESIAN_POINT('Ctrl Pts',(-35.1998349126634,24.5057193681843,-5.24984087129627));
#17948=CARTESIAN_POINT('Ctrl Pts',(-35.4697758584422,24.6207297677425,-5.71948809597562));
#17949=CARTESIAN_POINT('Ctrl Pts',(-35.7694126601179,24.7547796990843,-6.164414002969));
#17950=CARTESIAN_POINT('',(-35.7691912190766,24.7550996672027,6.16441400296896));
#17951=CARTESIAN_POINT('Ctrl Pts',(-33.7474765292383,24.1528016575408,-1.94289029309402E-15));
#17952=CARTESIAN_POINT('Ctrl Pts',(-33.8034434087317,24.0746019944583,1.09861960926657));
#17953=CARTESIAN_POINT('Ctrl Pts',(-34.0059051472516,24.0873861635411,2.18971594132745));
#17954=CARTESIAN_POINT('Ctrl Pts',(-34.6897464310455,24.2930763407556,4.28292314717356));
#17955=CARTESIAN_POINT('Ctrl Pts',(-35.1676910781174,24.4866606648091,5.27177304443356));
#17956=CARTESIAN_POINT('Ctrl Pts',(-35.7691912190765,24.7550996672027,6.16441400296898));
#17957=CARTESIAN_POINT('Origin',(-1.73472347597681E-15,-1.73472347597681E-15,
6.16441400296896));
#17958=CARTESIAN_POINT('Origin',(0.,0.,-6.93889390390723E-15));
#17959=CARTESIAN_POINT('',(-30.4453966086847,31.0697252215061,6.16441400296896));
#17960=CARTESIAN_POINT('',(-28.709727626521,29.9666738162743,0.));
#17961=CARTESIAN_POINT('Ctrl Pts',(-30.4453966086847,31.0697252215061,6.16441400296899));
#17962=CARTESIAN_POINT('Ctrl Pts',(-29.9507533455086,30.6516652743936,5.27531660683076));
#17963=CARTESIAN_POINT('Ctrl Pts',(-29.553335552626,30.3394714544405,4.29109868658263));
#17964=CARTESIAN_POINT('Ctrl Pts',(-28.9647448012292,29.9621423486913,2.19783870908456));
#17965=CARTESIAN_POINT('Ctrl Pts',(-28.7793799405672,29.8999430547261,1.10199792653042));
#17966=CARTESIAN_POINT('Ctrl Pts',(-28.709727626521,29.9666738162743,8.32667268468867E-16));
#17967=CARTESIAN_POINT('',(-30.4455144995497,31.0696096991531,-6.16441400296897));
#17968=CARTESIAN_POINT('Ctrl Pts',(-30.4455144995497,31.0696096991531,-6.164414002969));
#17969=CARTESIAN_POINT('Ctrl Pts',(-29.9510161819033,30.650930135392,-5.27484593811665));
#17970=CARTESIAN_POINT('Ctrl Pts',(-29.5523238483592,30.3398193877234,-4.29007656912482));
#17971=CARTESIAN_POINT('Ctrl Pts',(-28.964235794694,29.9624572234644,-2.19706468924138));
#17972=CARTESIAN_POINT('Ctrl Pts',(-28.7803227527792,29.8990397885854,-1.10157448608512));
#17973=CARTESIAN_POINT('Ctrl Pts',(-28.709727626521,29.9666738162743,-1.66533453693773E-15));
#17974=CARTESIAN_POINT('',(-31.8823591451153,29.5933299130377,-6.16441400296897));
#17975=CARTESIAN_POINT('Origin',(-5.20417042793042E-15,1.73472347597681E-15,
-6.16441400296897));
#17976=CARTESIAN_POINT('',(-29.966673816274,28.7097276265214,0.));
#17977=CARTESIAN_POINT('Ctrl Pts',(-29.966673816274,28.7097276265213,3.46944695195361E-15));
#17978=CARTESIAN_POINT('Ctrl Pts',(-29.9750857383085,28.700947420486,-0.137010845869001));
#17979=CARTESIAN_POINT('Ctrl Pts',(-29.9855286660442,28.6939122150399,-0.273849719844409));
#17980=CARTESIAN_POINT('Ctrl Pts',(-30.0104891974366,28.683308273128,-0.547496131370688));
#17981=CARTESIAN_POINT('Ctrl Pts',(-30.0250035906016,28.6797460897162,-0.684223919463375));
#17982=CARTESIAN_POINT('Ctrl Pts',(-30.0746352811261,28.6742811955938,-1.09397285881368));
#17983=CARTESIAN_POINT('Ctrl Pts',(-30.1158101338558,28.677615842858,-1.36621764183967));
#17984=CARTESIAN_POINT('Ctrl Pts',(-30.2634298311996,28.7084742231121,-2.17875768611005));
#17985=CARTESIAN_POINT('Ctrl Pts',(-30.3936948517388,28.7568689184108,-2.71300426677516));
#17986=CARTESIAN_POINT('Ctrl Pts',(-30.7168533707347,28.9078738414552,-3.75889728641947));
#17987=CARTESIAN_POINT('Ctrl Pts',(-30.9095313269425,29.0105151315892,-4.26878718252155));
#17988=CARTESIAN_POINT('Ctrl Pts',(-31.3540238590941,29.2657452924843,-5.24984087225396));
#17989=CARTESIAN_POINT('Ctrl Pts',(-31.604849508625,29.4180016539176,-5.71948809642924));
#17990=CARTESIAN_POINT('Ctrl Pts',(-31.8823591451152,29.5933299130376,-6.16441400296899));
#17991=CARTESIAN_POINT('',(-31.8820944218041,29.5936151100059,6.16441400296896));
#17992=CARTESIAN_POINT('Ctrl Pts',(-29.966673816274,28.7097276265213,-1.66533453693773E-15));
#17993=CARTESIAN_POINT('Ctrl Pts',(-30.0332000060363,28.6402888406582,1.09861960926661));
#17994=CARTESIAN_POINT('Ctrl Pts',(-30.2317815990283,28.6817561949069,2.18971594132752));
#17995=CARTESIAN_POINT('Ctrl Pts',(-30.8793896002662,28.9826735044058,4.28292314717356));
#17996=CARTESIAN_POINT('Ctrl Pts',(-31.3249195382002,29.2423060343176,5.27177304443357));
#17997=CARTESIAN_POINT('Ctrl Pts',(-31.8820944218041,29.5936151100059,6.16441400296898));
#17998=CARTESIAN_POINT('Origin',(-1.73472347597681E-15,-1.73472347597681E-15,
6.16441400296896));
#17999=CARTESIAN_POINT('Origin',(0.,0.,-6.93889390390723E-15));
#18000=CARTESIAN_POINT('',(-25.7138234497511,35.0863119121265,6.16441400296896));
#18001=CARTESIAN_POINT('',(-24.1528016575405,33.7474765292386,0.));
#18002=CARTESIAN_POINT('Ctrl Pts',(-25.7138234497511,35.0863119121265,6.16441400296898));
#18003=CARTESIAN_POINT('Ctrl Pts',(-25.2837110755394,34.6021121364811,5.2753166068308));
#18004=CARTESIAN_POINT('Ctrl Pts',(-24.9347682357557,34.2365375505478,4.29109868658277));
#18005=CARTESIAN_POINT('Ctrl Pts',(-24.4058680201908,33.7792839134373,2.19783870908457));
#18006=CARTESIAN_POINT('Ctrl Pts',(-24.2312417889977,33.691337548434,1.10199792653045));
#18007=CARTESIAN_POINT('Ctrl Pts',(-24.1528016575405,33.7474765292386,8.32667268468867E-16));
#18008=CARTESIAN_POINT('',(-25.7139565811841,35.0862143432572,-6.16441400296897));
#18009=CARTESIAN_POINT('Ctrl Pts',(-25.713956581184,35.0862143432571,-6.164414002969));
#18010=CARTESIAN_POINT('Ctrl Pts',(-25.2840758578099,34.6014218856657,-5.27484593811654));
#18011=CARTESIAN_POINT('Ctrl Pts',(-24.9337173131132,34.2367379618409,-4.29007656912594));
#18012=CARTESIAN_POINT('Ctrl Pts',(-24.4053193832555,33.7795231440466,-2.19706468921581));
#18013=CARTESIAN_POINT('Ctrl Pts',(-24.2323035529049,33.6905776524152,-1.10157448595032));
#18014=CARTESIAN_POINT('Ctrl Pts',(-24.1528016575405,33.7474765292386,-2.77555756156289E-16));
#18015=CARTESIAN_POINT('',(-27.3462727390392,33.829445270091,-6.16441400296897));
#18016=CARTESIAN_POINT('Origin',(-5.20417042793042E-15,1.73472347597681E-15,
-6.16441400296897));
#18017=CARTESIAN_POINT('',(-25.5758360411614,32.6822063330436,0.));
#18018=CARTESIAN_POINT('Ctrl Pts',(-25.5758360411614,32.6822063330435,2.60208521396521E-15));
#18019=CARTESIAN_POINT('Ctrl Pts',(-25.5854118955599,32.6747126381701,-0.137010845868782));
#18020=CARTESIAN_POINT('Ctrl Pts',(-25.5967497434736,32.6692352245436,-0.273849719843329));
#18021=CARTESIAN_POINT('Ctrl Pts',(-25.6229653109245,32.662291469459,-0.54749613136761));
#18022=CARTESIAN_POINT('Ctrl Pts',(-25.6378389200515,32.6608311574538,-0.684223919459034));
#18023=CARTESIAN_POINT('Ctrl Pts',(-25.6877431670541,32.6624852140826,-1.09397285880905));
#18024=CARTESIAN_POINT('Ctrl Pts',(-25.7280243493679,32.6716457119514,-1.36621764183439));
#18025=CARTESIAN_POINT('Ctrl Pts',(-25.8697498856529,32.7231984717371,-2.17875768610485));
#18026=CARTESIAN_POINT('Ctrl Pts',(-25.991801712879,32.7896392241448,-2.71300426677193));
#18027=CARTESIAN_POINT('Ctrl Pts',(-26.290180702901,32.9850973871755,-3.7588972864174));
#18028=CARTESIAN_POINT('Ctrl Pts',(-26.4662900967129,33.1141148691595,-4.26878718251803));
#18029=CARTESIAN_POINT('Ctrl Pts',(-26.8699352967195,33.4300050378598,-5.24984087225432));
#18030=CARTESIAN_POINT('Ctrl Pts',(-27.0965395633502,33.6164078608134,-5.71948809642964));
#18031=CARTESIAN_POINT('Ctrl Pts',(-27.3462727390392,33.829445270091,-6.164414002969));
#18032=CARTESIAN_POINT('',(-27.3459701224718,33.8296898901081,6.16441400296896));
#18033=CARTESIAN_POINT('Ctrl Pts',(-25.5758360411614,32.6822063330435,-1.66533453693773E-15));
#18034=CARTESIAN_POINT('Ctrl Pts',(-25.6515672598148,32.6229419978349,1.09861960926661));
#18035=CARTESIAN_POINT('Ctrl Pts',(-25.8422261587077,32.6922483814991,2.18971594132752));
#18036=CARTESIAN_POINT('Ctrl Pts',(-26.4404174460316,33.0822670146349,4.2829231471735));
#18037=CARTESIAN_POINT('Ctrl Pts',(-26.8444629700937,33.4026623808144,5.27177304443351));
#18038=CARTESIAN_POINT('Ctrl Pts',(-27.3459701224718,33.829689890108,6.16441400296898));
#18039=CARTESIAN_POINT('Origin',(-1.73472347597681E-15,-1.73472347597681E-15,
6.16441400296896));
#18040=CARTESIAN_POINT('Origin',(0.,0.,-6.93889390390723E-15));
#18041=CARTESIAN_POINT('',(-20.4587909979241,38.3886424727844,6.16441400296896));
#18042=CARTESIAN_POINT('',(-19.1041942977416,36.8412779397542,-3.46944695195361E-15));
#18043=CARTESIAN_POINT('Ctrl Pts',(-20.458790997924,38.3886424727844,6.16441400296899));
#18044=CARTESIAN_POINT('Ctrl Pts',(-20.1019653602739,37.8481597797213,5.2753166068308));
#18045=CARTESIAN_POINT('Ctrl Pts',(-19.8086009435391,37.4366464721473,4.29109868658275));
#18046=CARTESIAN_POINT('Ctrl Pts',(-19.3501581469722,36.9087766691158,2.19783870908188));
#18047=CARTESIAN_POINT('Ctrl Pts',(-19.1898254317347,36.7968735674505,1.10199792652465));
#18048=CARTESIAN_POINT('Ctrl Pts',(-19.1041942977408,36.8412779397535,2.72004641033163E-14));
#18049=CARTESIAN_POINT('',(-20.4589366597763,38.3885648435998,-6.16441400296897));
#18050=CARTESIAN_POINT('Ctrl Pts',(-20.4589366597763,38.3885648435998,-6.16441400296901));
#18051=CARTESIAN_POINT('Ctrl Pts',(-20.1024246625312,37.8475284685869,-5.27484593811536));
#18052=CARTESIAN_POINT('Ctrl Pts',(-19.8075321962687,37.4366952816587,-4.29007656912531));
#18053=CARTESIAN_POINT('Ctrl Pts',(-19.3495810482861,36.9089353855174,-2.19706468916458));
#18054=CARTESIAN_POINT('Ctrl Pts',(-19.1909845328821,36.7962725108431,-1.10157448568023));
#18055=CARTESIAN_POINT('Ctrl Pts',(-19.1041942977408,36.8412779397535,-3.13638004456607E-14));
#18056=CARTESIAN_POINT('',(-22.2534950801163,37.3768906775195,-6.16441400296897));
#18057=CARTESIAN_POINT('Origin',(-5.20417042793042E-15,1.73472347597681E-15,
-6.16441400296897));
#18058=CARTESIAN_POINT('',(-20.6643479988715,35.9893695663253,0.));
#18059=CARTESIAN_POINT('Ctrl Pts',(-20.6643479988715,35.9893695663252,2.63677968348475E-15));
#18060=CARTESIAN_POINT('Ctrl Pts',(-20.6748928488527,35.983314932631,-0.137010845869154));
#18061=CARTESIAN_POINT('Ctrl Pts',(-20.6868948110568,35.9795068151698,-0.273849719847874));
#18062=CARTESIAN_POINT('Ctrl Pts',(-20.7138317412126,35.9763646017424,-0.5474961313763));
#18063=CARTESIAN_POINT('Ctrl Pts',(-20.7287617825115,35.9770358888855,-0.68422391946899));
#18064=CARTESIAN_POINT('Ctrl Pts',(-20.7779226794341,35.9857752244446,-1.09397285881967));
#18065=CARTESIAN_POINT('Ctrl Pts',(-20.8164901826204,36.0005750915999,-1.36621764184467));
#18066=CARTESIAN_POINT('Ctrl Pts',(-20.9494364346273,36.0717727653988,-2.1787576861109));
#18067=CARTESIAN_POINT('Ctrl Pts',(-21.0607904453043,36.1549070327976,-2.71300426677424));
#18068=CARTESIAN_POINT('Ctrl Pts',(-21.3283157705729,36.390839471264,-3.75889728641524));
#18069=CARTESIAN_POINT('Ctrl Pts',(-21.4842715225984,36.5436067212097,-4.26878718251598));
#18070=CARTESIAN_POINT('Ctrl Pts',(-21.8388523381951,36.9137262848343,-5.24984087225303));
#18071=CARTESIAN_POINT('Ctrl Pts',(-22.0366222125189,37.1304809453829,-5.71948809642907));
#18072=CARTESIAN_POINT('Ctrl Pts',(-22.2534950801163,37.3768906775195,-6.16441400296901));
#18073=CARTESIAN_POINT('',(-22.2531607307118,37.3770897408173,6.16441400296896));
#18074=CARTESIAN_POINT('Ctrl Pts',(-20.6643479988715,35.9893695663252,-5.55111512312578E-16));
#18075=CARTESIAN_POINT('Ctrl Pts',(-20.747742577195,35.9414861327319,1.09861960926664));
#18076=CARTESIAN_POINT('Ctrl Pts',(-20.9265975166221,36.0372206677032,2.18971594132757));
#18077=CARTESIAN_POINT('Ctrl Pts',(-21.4631946404634,36.5084009698261,4.28292314717356));
#18078=CARTESIAN_POINT('Ctrl Pts',(-21.8175305489547,36.8830368465618,5.27177304443358));
#18079=CARTESIAN_POINT('Ctrl Pts',(-22.2531607307118,37.3770897408172,6.16441400296897));
#18080=CARTESIAN_POINT('Origin',(-1.73472347597681E-15,-1.73472347597681E-15,
6.16441400296896));
#18081=CARTESIAN_POINT('Origin',(0.,0.,-6.93889390390723E-15));
#18082=CARTESIAN_POINT('',(-14.7872765596605,40.9094909763996,6.16441400296896));
#18083=CARTESIAN_POINT('',(-13.6666806339862,39.1850971728874,0.));
#18084=CARTESIAN_POINT('Ctrl Pts',(-14.7872765596605,40.9094909763996,6.16441400296899));
#18085=CARTESIAN_POINT('Ctrl Pts',(-14.5110015995543,40.3237280349262,5.27531660683078));
#18086=CARTESIAN_POINT('Ctrl Pts',(-14.2791876594001,39.8746532299474,4.29109868658268));
#18087=CARTESIAN_POINT('Ctrl Pts',(-13.9005348551306,39.2869131679352,2.19783870908465));
#18088=CARTESIAN_POINT('Ctrl Pts',(-13.7577595675692,39.153331354054,1.10199792653061));
#18089=CARTESIAN_POINT('Ctrl Pts',(-13.6666806339861,39.1850971728874,-5.55111512312578E-16));
#18090=CARTESIAN_POINT('',(-14.7874317866676,40.9094348672119,-6.16441400296897));
#18091=CARTESIAN_POINT('Ctrl Pts',(-14.7874317866676,40.9094348672119,-6.164414002969));
#18092=CARTESIAN_POINT('Ctrl Pts',(-14.5115460717139,40.3231685151577,-5.27484593811608));
#18093=CARTESIAN_POINT('Ctrl Pts',(-14.2781228441205,39.8745494440526,-4.29007656912554));
#18094=CARTESIAN_POINT('Ctrl Pts',(-13.8999410427714,39.2869881391078,-2.19706468910641));
#18095=CARTESIAN_POINT('Ctrl Pts',(-13.7589924099841,39.1529013726383,-1.1015744853717));
#18096=CARTESIAN_POINT('Ctrl Pts',(-13.6666806339861,39.1850971728874,-8.32667268468867E-16));
#18097=CARTESIAN_POINT('',(-16.7077004351661,40.1634503767885,-6.16441400296897));
#18098=CARTESIAN_POINT('Origin',(-5.20417042793042E-15,1.73472347597681E-15,
-6.16441400296897));
#18099=CARTESIAN_POINT('',(-15.3321934223833,38.5638930200081,0.));
#18100=CARTESIAN_POINT('Ctrl Pts',(-15.3321934223833,38.5638930200081,1.2490009027033E-15));
#18101=CARTESIAN_POINT('Ctrl Pts',(-15.3434926052115,38.5594007023744,-0.137010845860815));
#18102=CARTESIAN_POINT('Ctrl Pts',(-15.3559143563672,38.5573394033676,-0.273849719841542));
#18103=CARTESIAN_POINT('Ctrl Pts',(-15.3830242910103,38.5580626980003,-0.547496131368016));
#18104=CARTESIAN_POINT('Ctrl Pts',(-15.3977068318951,38.5608519188208,-0.684223919460011));
#18105=CARTESIAN_POINT('Ctrl Pts',(-15.4451236046443,38.5764986256395,-1.09397285880962));
#18106=CARTESIAN_POINT('Ctrl Pts',(-15.4811923055565,38.5966365794654,-1.36621764183523));
#18107=CARTESIAN_POINT('Ctrl Pts',(-15.6026528709759,38.6860297879581,-2.17875768610564));
#18108=CARTESIAN_POINT('Ctrl Pts',(-15.7010422185607,38.7841651964068,-2.71300426677201));
#18109=CARTESIAN_POINT('Ctrl Pts',(-15.9322678349351,39.0557690062366,-3.75889728641666));
#18110=CARTESIAN_POINT('Ctrl Pts',(-16.0648951358121,39.2291761234751,-4.26878718251826));
#18111=CARTESIAN_POINT('Ctrl Pts',(-16.3631933241338,39.6459905150347,-5.2498408722538));
#18112=CARTESIAN_POINT('Ctrl Pts',(-16.5281027818355,39.8886845133532,-5.71948809642935));
#18113=CARTESIAN_POINT('Ctrl Pts',(-16.7077004351661,40.1634503767885,-6.16441400296899));
#18114=CARTESIAN_POINT('',(-16.7073411592909,40.1635998310295,6.16441400296896));
#18115=CARTESIAN_POINT('Ctrl Pts',(-15.3321934223833,38.5638930200081,-1.38777878078145E-15));
#18116=CARTESIAN_POINT('Ctrl Pts',(-15.4215536872523,38.5283652566535,1.09861960926664));
#18117=CARTESIAN_POINT('Ctrl Pts',(-15.5849636964219,38.6485790638755,2.18971594132757));
#18118=CARTESIAN_POINT('Ctrl Pts',(-16.0490430867575,39.1913291628061,4.28292314717355));
#18119=CARTESIAN_POINT('Ctrl Pts',(-16.3464561224015,39.6125790440083,5.27177304443356));
#18120=CARTESIAN_POINT('Ctrl Pts',(-16.7073411592909,40.1635998310294,6.16441400296897));
#18121=CARTESIAN_POINT('Origin',(-1.73472347597681E-15,-1.73472347597681E-15,
6.16441400296896));
#18122=CARTESIAN_POINT('Origin',(0.,0.,-6.93889390390723E-15));
#18123=CARTESIAN_POINT('',(-8.81473581362657,42.5975402169653,6.16441400296896));
#18124=CARTESIAN_POINT('',(-7.95095276397595,40.7312208280703,0.));
#18125=CARTESIAN_POINT('Ctrl Pts',(-8.81473754185273,42.5975458454602,6.16442208586935));
#18126=CARTESIAN_POINT('Ctrl Pts',(-8.62463742076709,41.9784270998641,5.27532468973107));
#18127=CARTESIAN_POINT('Ctrl Pts',(-8.45909129229247,41.5009270369901,4.29109868658251));
#18128=CARTESIAN_POINT('Ctrl Pts',(-8.16793675947019,40.8652814087567,2.19783870908467));
#18129=CARTESIAN_POINT('Ctrl Pts',(-8.04562539271004,40.712740223173,1.10199792653066));
#18130=CARTESIAN_POINT('Ctrl Pts',(-7.95095276397594,40.7312208280702,2.77555756156289E-15));
#18131=CARTESIAN_POINT('',(-8.81489744582791,42.5975067699923,-6.16441400296897));
#18132=CARTESIAN_POINT('Ctrl Pts',(-8.8148974458279,42.5975067699923,-6.164414002969));
#18133=CARTESIAN_POINT('Ctrl Pts',(-8.62525425073438,41.9779451331706,-5.27484593811627));
#18134=CARTESIAN_POINT('Ctrl Pts',(-8.45805208556847,41.500672768472,-4.29007656912508));
#18135=CARTESIAN_POINT('Ctrl Pts',(-8.16733832174611,40.8652711085092,-2.19706468906603));
#18136=CARTESIAN_POINT('Ctrl Pts',(-8.046906879285,40.7124900701204,-1.10157448515744));
#18137=CARTESIAN_POINT('Ctrl Pts',(-7.95095276397593,40.7312208280702,-1.38777878078145E-15));
#18138=CARTESIAN_POINT('',(-10.8217851903811,42.1323980482153,-6.16441400296897));
#18139=CARTESIAN_POINT('Origin',(-5.20417042793042E-15,1.73472347597681E-15,
-6.16441400296897));
#18140=CARTESIAN_POINT('',(-9.68791960221003,40.3533668208877,1.04083408558608E-14));
#18141=CARTESIAN_POINT('Ctrl Pts',(-9.68791960221003,40.3533668208876,1.21777588013572E-14));
#18142=CARTESIAN_POINT('Ctrl Pts',(-9.6997430991055,40.3505282699472,-0.137010845855937));
#18143=CARTESIAN_POINT('Ctrl Pts',(-9.71233176817975,40.3502557514989,-0.273849719840574));
#18144=CARTESIAN_POINT('Ctrl Pts',(-9.7390628272182,40.3548298299997,-0.547496131367697));
#18145=CARTESIAN_POINT('Ctrl Pts',(-9.75319897349705,40.3596802040055,-0.68422391945948));
#18146=CARTESIAN_POINT('Ctrl Pts',(-9.79790635331839,40.3819157602545,-1.09397285880777));
#18147=CARTESIAN_POINT('Ctrl Pts',(-9.83074199722052,40.4069818500838,-1.36621764183255));
#18148=CARTESIAN_POINT('Ctrl Pts',(-9.93824428920808,40.5127508053321,-2.17875768610361));
#18149=CARTESIAN_POINT('Ctrl Pts',(-10.0216660503199,40.6238896009114,-2.71300426677103));
#18150=CARTESIAN_POINT('Ctrl Pts',(-10.2118848710492,40.9256357117768,-3.75889728641691));
#18151=CARTESIAN_POINT('Ctrl Pts',(-10.3184838113872,41.1161526274701,-4.26878718251867));
#18152=CARTESIAN_POINT('Ctrl Pts',(-10.5544268815369,41.5711767079492,-5.24984087225478));
#18153=CARTESIAN_POINT('Ctrl Pts',(-10.6831188416198,41.8348694941026,-5.71948809642984));
#18154=CARTESIAN_POINT('Ctrl Pts',(-10.8217851903811,42.1323980482152,-6.164414002969));
#18155=CARTESIAN_POINT('',(-10.82140830186,42.1324948509394,6.16441400296896));
#18156=CARTESIAN_POINT('Ctrl Pts',(-9.68791960221004,40.3533668208876,9.15933995315754E-15));
#18157=CARTESIAN_POINT('Ctrl Pts',(-9.78142643632559,40.3309179705801,1.09861960926654));
#18158=CARTESIAN_POINT('Ctrl Pts',(-9.92606495868656,40.4731638436057,2.18971594132738));
#18159=CARTESIAN_POINT('Ctrl Pts',(-10.3081792974237,41.0764349124918,4.2829231471736));
#18160=CARTESIAN_POINT('Ctrl Pts',(-10.5426149884832,41.5357233653637,5.27177304443365));
#18161=CARTESIAN_POINT('Ctrl Pts',(-10.82140830186,42.1324948509394,6.16441400296898));
#18162=CARTESIAN_POINT('Origin',(-1.73472347597681E-15,-1.73472347597681E-15,
6.16441400296896));
#18163=CARTESIAN_POINT('Origin',(0.,0.,-6.93889390390723E-15));
#18164=CARTESIAN_POINT('',(-2.66275246602648,43.4184263798755,6.16441400296896));
#18165=CARTESIAN_POINT('',(-2.07336642434587,41.448174286335,0.));
#18166=CARTESIAN_POINT('Ctrl Pts',(-2.66275246602647,43.4184263798755,6.16441400296898));
#18167=CARTESIAN_POINT('Ctrl Pts',(-2.56269707422321,42.7785553024261,5.27531660683073));
#18168=CARTESIAN_POINT('Ctrl Pts',(-2.46679222047902,42.2823616483505,4.29109868658259));
#18169=CARTESIAN_POINT('Ctrl Pts',(-2.26906302577184,41.611750365836,2.19783870908463));
#18170=CARTESIAN_POINT('Ctrl Pts',(-2.16970548652324,41.4433551071959,1.1019979265306));
#18171=CARTESIAN_POINT('Ctrl Pts',(-2.07336642434585,41.4481742863349,1.38777878078145E-15));
#18172=CARTESIAN_POINT('',(-2.66291721304304,43.4184162760053,-6.16441400296898));
#18173=CARTESIAN_POINT('Ctrl Pts',(-2.66291721304302,43.4184162760053,-6.16441400296899));
#18174=CARTESIAN_POINT('Ctrl Pts',(-2.56337712638027,42.7781718426724,-5.27484593811571));
#18175=CARTESIAN_POINT('Ctrl Pts',(-2.46579977756426,42.2819620733826,-4.29007656912569));
#18176=CARTESIAN_POINT('Ctrl Pts',(-2.26847214514445,41.6116550038393,-2.197064688993));
#18177=CARTESIAN_POINT('Ctrl Pts',(-2.17100952986355,41.4432898748974,-1.1015744847684));
#18178=CARTESIAN_POINT('Ctrl Pts',(-2.07336642434585,41.4481742863349,-1.66533453693773E-15));
#18179=CARTESIAN_POINT('',(-4.71556960658337,43.2436515951818,-6.16441400296897));
#18180=CARTESIAN_POINT('Origin',(-5.20417042793042E-15,1.73472347597681E-15,
-6.16441400296897));
#18181=CARTESIAN_POINT('',(-3.84642767658888,41.3213624427944,0.));
#18182=CARTESIAN_POINT('Ctrl Pts',(-3.8464276765889,41.3213624427943,2.35922392732846E-15));
#18183=CARTESIAN_POINT('Ctrl Pts',(-3.85853479525186,41.3202354432581,-0.137010845849856));
#18184=CARTESIAN_POINT('Ctrl Pts',(-3.87103411324552,41.321757253058,-0.273849719835895));
#18185=CARTESIAN_POINT('Ctrl Pts',(-3.89684212940387,41.3300890003785,-0.547496131360071));
#18186=CARTESIAN_POINT('Ctrl Pts',(-3.91014410990392,41.3369017879418,-0.684223919450046));
#18187=CARTESIAN_POINT('Ctrl Pts',(-3.95123198346989,41.3652735418179,-1.09397285879913));
#18188=CARTESIAN_POINT('Ctrl Pts',(-3.98016613134168,41.3947574943464,-1.36621764182406));
#18189=CARTESIAN_POINT('Ctrl Pts',(-4.07152171324077,41.5147490454345,-2.17875768609805));
#18190=CARTESIAN_POINT('Ctrl Pts',(-4.13827766138895,41.6366287627654,-2.71300426676847));
#18191=CARTESIAN_POINT('Ctrl Pts',(-4.28361737982964,41.9623744940143,-3.75889728641876));
#18192=CARTESIAN_POINT('Ctrl Pts',(-4.36201791261577,42.1661228331631,-4.26878718252147));
#18193=CARTESIAN_POINT('Ctrl Pts',(-4.53080274409615,42.6500936244629,-5.24984087225698));
#18194=CARTESIAN_POINT('Ctrl Pts',(-4.62065740937212,42.9294171737523,-5.71948809643096));
#18195=CARTESIAN_POINT('Ctrl Pts',(-4.71556960658338,43.2436515951818,-6.164414002969));
#18196=CARTESIAN_POINT('',(-4.71518277776789,43.2436937757662,6.16441400296896));
#18197=CARTESIAN_POINT('Ctrl Pts',(-3.84642767658889,41.3213624427943,-1.66533453693773E-15));
#18198=CARTESIAN_POINT('Ctrl Pts',(-3.94217755045982,41.3124494993889,1.09861960926671));
#18199=CARTESIAN_POINT('Ctrl Pts',(-4.06510016280003,41.4738317224468,2.18971594132769));
#18200=CARTESIAN_POINT('Ctrl Pts',(-4.35747070392864,42.1253429020159,4.28292314717349));
#18201=CARTESIAN_POINT('Ctrl Pts',(-4.52415661579022,42.6133201381352,5.27177304443345));
#18202=CARTESIAN_POINT('Ctrl Pts',(-4.71518277776791,43.2436937757662,6.16441400296897));
#18203=CARTESIAN_POINT('Origin',(-1.73472347597681E-15,-1.73472347597681E-15,
6.16441400296896));
#18204=CARTESIAN_POINT('Origin',(0.,0.,-6.93889390390723E-15));
#18205=CARTESIAN_POINT('',(3.54343684303851,43.3554385900939,6.16441400296897));
#18206=CARTESIAN_POINT('',(3.84642767658947,41.3213624427943,0.));
#18207=CARTESIAN_POINT('Ctrl Pts',(3.54343684303853,43.3554385900938,6.16441400296898));
#18208=CARTESIAN_POINT('Ctrl Pts',(3.55141066631822,42.7078411106921,5.27531660683074));
#18209=CARTESIAN_POINT('Ctrl Pts',(3.57572362730268,42.2030493088126,4.29109868658261));
#18210=CARTESIAN_POINT('Ctrl Pts',(3.67600228769439,41.5111240838458,2.1978387090846));
#18211=CARTESIAN_POINT('Ctrl Pts',(3.75038336645583,41.3303027940033,1.10199792653051));
#18212=CARTESIAN_POINT('Ctrl Pts',(3.84642767658948,41.3213624427942,2.77555756156289E-16));
#18213=CARTESIAN_POINT('',(3.54327233497914,43.3554520350114,-6.16441400296898));
#18214=CARTESIAN_POINT('Ctrl Pts',(3.54327233497913,43.3554520350114,-6.16441400296901));
#18215=CARTESIAN_POINT('Ctrl Pts',(3.55068296410195,42.7075583355186,-5.27484593811621));
#18216=CARTESIAN_POINT('Ctrl Pts',(3.57664910313154,42.2025125615888,-4.29007656912535));
#18217=CARTESIAN_POINT('Ctrl Pts',(3.6765735825726,41.5109456014396,-2.19706468906318));
#18218=CARTESIAN_POINT('Ctrl Pts',(3.74908331283908,41.3304238103958,-1.1015744851416));
#18219=CARTESIAN_POINT('Ctrl Pts',(3.84642767658949,41.3213624427942,-8.32667268468867E-16));
#18220=CARTESIAN_POINT('',(1.48664137583834,43.4745891000668,-6.16441400296897));
#18221=CARTESIAN_POINT('Origin',(-5.20417042793042E-15,1.73472347597681E-15,
-6.16441400296897));
#18222=CARTESIAN_POINT('',(2.07336642434584,41.448174286335,0.));
#18223=CARTESIAN_POINT('Ctrl Pts',(2.07336642434582,41.4481742863349,1.80411241501588E-15));
#18224=CARTESIAN_POINT('Ctrl Pts',(2.06122214993787,41.4487817806634,-0.137010845843175));
#18225=CARTESIAN_POINT('Ctrl Pts',(2.04906663309415,41.4520669390525,-0.273849719833891));
#18226=CARTESIAN_POINT('Ctrl Pts',(2.02470703660085,41.4639867448445,-0.547496131359161));
#18227=CARTESIAN_POINT('Ctrl Pts',(2.01251001184276,41.4726232572572,-0.684223919449438));
#18228=CARTESIAN_POINT('Ctrl Pts',(1.97587807515069,41.5065536416689,-1.09397285879738));
#18229=CARTESIAN_POINT('Ctrl Pts',(1.95143443912054,41.5398552486479,-1.36621764182242));
#18230=CARTESIAN_POINT('Ctrl Pts',(1.8780853035088,41.6716267136228,-2.17875768609688));
#18231=CARTESIAN_POINT('Ctrl Pts',(1.82935412691927,41.8017662331319,-2.71300426676794));
#18232=CARTESIAN_POINT('Ctrl Pts',(1.73185220830974,42.144880341048,-3.75889728641881));
#18233=CARTESIAN_POINT('Ctrl Pts',(1.68324609183628,42.3577123750292,-4.26878718252151));
#18234=CARTESIAN_POINT('Ctrl Pts',(1.58505547146645,42.8607776274967,-5.24984087225669));
#18235=CARTESIAN_POINT('Ctrl Pts',(1.53586728286775,43.1500457179624,-5.7194880964307));
#18236=CARTESIAN_POINT('Ctrl Pts',(1.48664137583833,43.4745891000668,-6.164414002969));
#18237=CARTESIAN_POINT('',(1.48703027021497,43.4745757998335,6.16441400296896));
#18238=CARTESIAN_POINT('Ctrl Pts',(2.07336642434583,41.4481742863349,-2.22044604925031E-15));
#18239=CARTESIAN_POINT('Ctrl Pts',(1.97732270203171,41.4529786916566,1.09861960926666));
#18240=CARTESIAN_POINT('Ctrl Pts',(1.87861834962003,41.630211988073,2.18971594132761));
#18241=CARTESIAN_POINT('Ctrl Pts',(1.6819434271902,42.3167003895122,4.28292314717354));
#18242=CARTESIAN_POINT('Ctrl Pts',(1.58640053900949,42.8234325995621,5.27177304443355));
#18243=CARTESIAN_POINT('Ctrl Pts',(1.48703027021496,43.4745757998335,6.16441400296897));
#18244=CARTESIAN_POINT('Origin',(-1.73472347597681E-15,-1.73472347597681E-15,
6.16441400296896));
#18245=CARTESIAN_POINT('Origin',(0.,0.,-6.93889390390723E-15));
#18246=CARTESIAN_POINT('',(9.67749199640695,42.4098590973783,6.16441400296896));
#18247=CARTESIAN_POINT('',(9.68791960221059,40.3533668208876,0.));
#18248=CARTESIAN_POINT('Ctrl Pts',(9.67749199640696,42.4098590973783,6.164414002969));
#18249=CARTESIAN_POINT('Ctrl Pts',(9.59322192711572,41.7677184331879,5.27531660683075));
#18250=CARTESIAN_POINT('Ctrl Pts',(9.54544805356759,41.2646045888914,4.29109868658259));
#18251=CARTESIAN_POINT('Ctrl Pts',(9.54623479529805,40.5654510237051,2.19783870908456));
#18252=CARTESIAN_POINT('Ctrl Pts',(9.59412522930608,40.3758847026759,1.10199792653043));
#18253=CARTESIAN_POINT('Ctrl Pts',(9.6879196022106,40.3533668208875,1.38777878078145E-15));
#18254=CARTESIAN_POINT('',(9.67733107622405,42.4098958173815,-6.16441400296897));
#18255=CARTESIAN_POINT('Ctrl Pts',(9.67733107622405,42.4098958173815,-6.16441400296901));
#18256=CARTESIAN_POINT('Ctrl Pts',(9.59246138876394,41.767542099079,-5.2748459381158));
#18257=CARTESIAN_POINT('Ctrl Pts',(9.54628772229279,41.2639415960375,-4.29007656912554));
#18258=CARTESIAN_POINT('Ctrl Pts',(9.54677487451954,40.5651930542696,-2.19706468910642));
#18259=CARTESIAN_POINT('Ctrl Pts',(9.59285563076488,40.376189504222,-1.10157448537283));
#18260=CARTESIAN_POINT('Ctrl Pts',(9.68791960221059,40.3533668208875,0.));
#18261=CARTESIAN_POINT('',(7.6585886269646,42.8205093412366,-6.16441400296898));
#18262=CARTESIAN_POINT('Origin',(-5.20417042793042E-15,1.73472347597681E-15,
-6.16441400296897));
#18263=CARTESIAN_POINT('',(7.95095276397653,40.7312208280702,0.));
#18264=CARTESIAN_POINT('Ctrl Pts',(7.95095276397649,40.7312208280701,2.98372437868011E-15));
#18265=CARTESIAN_POINT('Ctrl Pts',(7.93901855622804,40.7335504494307,-0.137010845850136));
#18266=CARTESIAN_POINT('Ctrl Pts',(7.92745429180435,40.738532080058,-0.273849719836056));
#18267=CARTESIAN_POINT('Ctrl Pts',(7.90503900611341,40.7537972914492,-0.547496131360746));
#18268=CARTESIAN_POINT('Ctrl Pts',(7.89419523334797,40.7640817142243,-0.684223919451336));
#18269=CARTESIAN_POINT('Ctrl Pts',(7.86276495412265,40.8028800043923,-1.09397285879932));
#18270=CARTESIAN_POINT('Ctrl Pts',(7.84330943187384,40.8393213411377,-1.36621764182423));
#18271=CARTESIAN_POINT('Ctrl Pts',(7.78945991942847,40.9801902329702,-2.17875768609855));
#18272=CARTESIAN_POINT('Ctrl Pts',(7.75974554062361,41.1159402893316,-2.71300426676885));
#18273=CARTESIAN_POINT('Ctrl Pts',(7.71206627973686,41.4694379601366,-3.75889728641854));
#18274=CARTESIAN_POINT('Ctrl Pts',(7.6942440599413,41.6870210424949,-4.26878718252084));
#18275=CARTESIAN_POINT('Ctrl Pts',(7.66864652855301,42.1989397983105,-5.24984087225615));
#18276=CARTESIAN_POINT('Ctrl Pts',(7.66112614630197,42.4922637658111,-5.71948809643045));
#18277=CARTESIAN_POINT('Ctrl Pts',(7.65858862696456,42.8205093412366,-6.164414002969));
#18278=CARTESIAN_POINT('',(7.65897167013808,42.8204408309399,6.16441400296896));
#18279=CARTESIAN_POINT('Ctrl Pts',(7.95095276397651,40.7312208280701,2.77555756156289E-16));
#18280=CARTESIAN_POINT('Ctrl Pts',(7.85657036643829,40.7496447782813,1.09861960926667));
#18281=CARTESIAN_POINT('Ctrl Pts',(7.78409360993039,40.9391211892399,2.18971594132763));
#18282=CARTESIAN_POINT('Ctrl Pts',(7.68711804045638,41.646611888365,4.28292314717352));
#18283=CARTESIAN_POINT('Ctrl Pts',(7.66466315363699,42.1617834658436,5.27177304443353));
#18284=CARTESIAN_POINT('Ctrl Pts',(7.65897167013807,42.8204408309399,6.16441400296898));
#18285=CARTESIAN_POINT('Origin',(-1.73472347597681E-15,-1.73472347597681E-15,
6.16441400296896));
#18286=CARTESIAN_POINT('Origin',(0.,0.,-6.93889390390723E-15));
#18287=CARTESIAN_POINT('',(15.6145413203109,40.6009371733745,6.16441400296896));
#18288=CARTESIAN_POINT('',(15.3321934223838,38.5638930200079,0.));
#18289=CARTESIAN_POINT('Ctrl Pts',(15.6145413203109,40.6009371733745,6.16441400296897));
#18290=CARTESIAN_POINT('Ctrl Pts',(15.4397428540447,39.9773254565376,5.27531660683071));
#18291=CARTESIAN_POINT('Ctrl Pts',(15.320854684261,39.4861315168335,4.29109868658256));
#18292=CARTESIAN_POINT('Ctrl Pts',(15.2221334915373,38.7939823618225,2.1978387090846));
#18293=CARTESIAN_POINT('Ctrl Pts',(15.2425583696601,38.5995300332387,1.10199792653053));
#18294=CARTESIAN_POINT('Ctrl Pts',(15.3321934223838,38.5638930200079,2.4980018054066E-15));
#18295=CARTESIAN_POINT('',(15.6143872638506,40.6009964209563,-6.16441400296898));
#18296=CARTESIAN_POINT('Ctrl Pts',(15.6143872638506,40.6009964209562,-6.16441400296901));
#18297=CARTESIAN_POINT('Ctrl Pts',(15.4389649620045,39.9772591535156,-5.27484593863204));
#18298=CARTESIAN_POINT('Ctrl Pts',(15.321591452786,39.4853557755399,-4.29007657026461));
#18299=CARTESIAN_POINT('Ctrl Pts',(15.2474362658641,38.9670300715335,-2.72168992255469));
#18300=CARTESIAN_POINT('Ctrl Pts',(15.2397716853914,38.8316817981346,-2.18495234743865));
#18301=CARTESIAN_POINT('Ctrl Pts',(15.2546174490221,38.6871424443347,-1.36923477589022));
#18302=CARTESIAN_POINT('Ctrl Pts',(15.2639350598672,38.648771103302,-1.09614446426196));
#18303=CARTESIAN_POINT('Ctrl Pts',(15.2845589828127,38.6059128200838,-0.685318587195841));
#18304=CARTESIAN_POINT('Ctrl Pts',(15.2925330768462,38.5940831817694,-0.548301186445323));
#18305=CARTESIAN_POINT('Ctrl Pts',(15.3107031781166,38.5753179353705,-0.274113036182014));
#18306=CARTESIAN_POINT('Ctrl Pts',(15.3208920224688,38.5683862191086,-0.137034229960439));
#18307=CARTESIAN_POINT('Ctrl Pts',(15.3321934223838,38.5638930200079,3.46944695195361E-17));
#18308=CARTESIAN_POINT('',(13.6746290992085,41.2947274963655,-6.16441400296897));
#18309=CARTESIAN_POINT('Origin',(-5.20417042793042E-15,1.73472347597681E-15,
-6.16441400296897));
#18310=CARTESIAN_POINT('',(13.6666806339867,39.1850971728872,0.));
#18311=CARTESIAN_POINT('Ctrl Pts',(13.6666806339867,39.1850971728872,1.83880688453542E-15));
#18312=CARTESIAN_POINT('Ctrl Pts',(13.6551994389513,39.1891014969075,-0.137010845854186));
#18313=CARTESIAN_POINT('Ctrl Pts',(13.6444618420215,39.1956781881393,-0.273849719837921));
#18314=CARTESIAN_POINT('Ctrl Pts',(13.6244471777075,39.2139780494479,-0.547496131363585));
#18315=CARTESIAN_POINT('Ctrl Pts',(13.6151774048766,39.2257010213957,-0.684223919454799));
#18316=CARTESIAN_POINT('Ctrl Pts',(13.5895886129639,39.2685773960179,-1.09397285880287));
#18317=CARTESIAN_POINT('Ctrl Pts',(13.5755172628236,39.3074166220021,-1.36621764182792));
#18318=CARTESIAN_POINT('Ctrl Pts',(13.5422635943279,39.4545152562871,-2.17875768610036));
#18319=CARTESIAN_POINT('Ctrl Pts',(13.5321709123718,39.5931123698236,-2.71300426676916));
#18320=CARTESIAN_POINT('Ctrl Pts',(13.5352849214684,39.9497974103412,-3.75889728641716));
#18321=CARTESIAN_POINT('Ctrl Pts',(13.5486094073549,40.1677021769759,-4.26878718251941));
#18322=CARTESIAN_POINT('Ctrl Pts',(13.5961260568799,40.6780532465201,-5.2498408722557));
#18323=CARTESIAN_POINT('Ctrl Pts',(13.6304265742773,40.9694618609525,-5.71948809643038));
#18324=CARTESIAN_POINT('Ctrl Pts',(13.6746290992085,41.2947274963655,-6.16441400296901));
#18325=CARTESIAN_POINT('',(13.6749984935073,41.2946051706827,6.16441400296896));
#18326=CARTESIAN_POINT('Ctrl Pts',(13.6666806339867,39.1850971728872,-8.32667268468867E-16));
#18327=CARTESIAN_POINT('Ctrl Pts',(13.5758809146619,39.2167656094919,1.0986196092667));
#18328=CARTESIAN_POINT('Ctrl Pts',(13.5311071718145,39.4146279416703,2.18971594132769));
#18329=CARTESIAN_POINT('Ctrl Pts',(13.5358050982364,40.1287184680818,4.28292314717347));
#18330=CARTESIAN_POINT('Ctrl Pts',(13.5868958926851,40.6418470803382,5.27178170541197));
#18331=CARTESIAN_POINT('Ctrl Pts',(13.6749992876916,41.2946110548517,6.16442204944812));
#18332=CARTESIAN_POINT('Origin',(-1.73472347597681E-15,-1.73472347597681E-15,
6.16441400296896));
#18333=CARTESIAN_POINT('Origin',(0.,0.,-6.93889390390723E-15));
#18334=CARTESIAN_POINT('',(21.2337236115522,37.9654972519551,6.16441400296897));
#18335=CARTESIAN_POINT('',(20.664347998872,35.989369566325,0.));
#18336=CARTESIAN_POINT('Ctrl Pts',(21.2337236115522,37.9654972519551,6.16441400296898));
#18337=CARTESIAN_POINT('Ctrl Pts',(20.971955141007,37.3731094186789,5.27531660683071));
#18338=CARTESIAN_POINT('Ctrl Pts',(20.7843728952793,36.9038346756932,4.29109868658253));
#18339=CARTESIAN_POINT('Ctrl Pts',(20.588153446897,36.2327800916601,2.19783870908462));
#18340=CARTESIAN_POINT('Ctrl Pts',(20.5806969775164,36.0374002441774,1.10199792653056));
#18341=CARTESIAN_POINT('Ctrl Pts',(20.664347998872,35.9893695663249,-2.77555756156289E-16));
#18342=CARTESIAN_POINT('',(21.2335795549855,37.965577820996,-6.16441400296897));
#18343=CARTESIAN_POINT('Ctrl Pts',(21.2335819393416,37.9655832041028,-6.16442208610002));
#18344=CARTESIAN_POINT('Ctrl Pts',(20.9711781152475,37.3731598792073,-5.27485402176265));
#18345=CARTESIAN_POINT('Ctrl Pts',(20.7849917650648,36.9029619772348,-4.29007657026496));
#18346=CARTESIAN_POINT('Ctrl Pts',(20.6378259322843,36.4004654649649,-2.72168992255382));
#18347=CARTESIAN_POINT('Ctrl Pts',(20.6109772985515,36.2675856253627,-2.18495234743789));
#18348=CARTESIAN_POINT('Ctrl Pts',(20.6051018589552,36.1224047013253,-1.36923477588968));
#18349=CARTESIAN_POINT('Ctrl Pts',(20.6088638187637,36.0830978909367,-1.0961444642612));
#18350=CARTESIAN_POINT('Ctrl Pts',(20.6231784502659,36.0377407529866,-0.685318587194771));
#18351=CARTESIAN_POINT('Ctrl Pts',(20.6293878464561,36.0248966914307,-0.548301186444714));
#18352=CARTESIAN_POINT('Ctrl Pts',(20.644702429288,36.0037365731592,-0.274113036178763));
#18353=CARTESIAN_POINT('Ctrl Pts',(20.6538010798168,35.9954253880384,-0.137034229958601));
#18354=CARTESIAN_POINT('Ctrl Pts',(20.664347998872,35.9893695663249,2.42861286636753E-16));
#18355=CARTESIAN_POINT('',(19.4122935573318,38.9283040838408,-6.16441400296897));
#18356=CARTESIAN_POINT('Origin',(-5.20417042793042E-15,1.73472347597681E-15,
-6.16441400296897));
#18357=CARTESIAN_POINT('',(19.1041942977414,36.8412779397533,0.));
#18358=CARTESIAN_POINT('Ctrl Pts',(19.1041942977413,36.8412779397532,1.38777878078145E-15));
#18359=CARTESIAN_POINT('Ctrl Pts',(19.0176106207021,36.8861762571209,-1.09898083807772));
#18360=CARTESIAN_POINT('Ctrl Pts',(19.0022226489713,37.0881362268422,-2.19052946959247));
#18361=CARTESIAN_POINT('Ctrl Pts',(19.082964194596,37.6168941902153,-3.75889728453982));
#18362=CARTESIAN_POINT('Ctrl Pts',(19.1271641380397,37.8306847285466,-4.26878718105547));
#18363=CARTESIAN_POINT('Ctrl Pts',(19.246827666541,38.3290788360445,-5.24984087156839));
#18364=CARTESIAN_POINT('Ctrl Pts',(19.3222522781826,38.6126451860877,-5.71949644909548));
#18365=CARTESIAN_POINT('Ctrl Pts',(19.4122951858544,38.9283097929761,-6.16442204993663));
#18366=CARTESIAN_POINT('',(19.4126417829878,38.9281304329581,6.16441400296896));
#18367=CARTESIAN_POINT('Ctrl Pts',(19.1041942977413,36.8412779397532,-5.55111512312578E-16));
#18368=CARTESIAN_POINT('Ctrl Pts',(19.0188256770706,36.8855461847064,1.0986196092667));
#18369=CARTESIAN_POINT('Ctrl Pts',(19.0026664121714,37.0877665316094,2.18971594132768));
#18370=CARTESIAN_POINT('Ctrl Pts',(19.1089421982549,37.7939200614565,4.2829231471735));
#18371=CARTESIAN_POINT('Ctrl Pts',(19.2325374978635,38.2945498429304,5.2717730444335));
#18372=CARTESIAN_POINT('Ctrl Pts',(19.4126417829878,38.9281304329581,6.16441400296897));
#18373=CARTESIAN_POINT('Origin',(-1.73472347597681E-15,-1.73472347597681E-15,
6.16441400296896));
#18374=CARTESIAN_POINT('Origin',(0.,0.,-6.93889390390723E-15));
#18375=CARTESIAN_POINT('',(26.4206485230646,34.5571892899391,6.16441400296896));
#18376=CARTESIAN_POINT('',(25.5758360411619,32.6822063330432,0.));
#18377=CARTESIAN_POINT('Ctrl Pts',(26.4206485230647,34.5571892899391,6.16441400296897));
#18378=CARTESIAN_POINT('Ctrl Pts',(26.0772388994229,34.0080846482036,5.2753166068307));
#18379=CARTESIAN_POINT('Ctrl Pts',(25.8247812113316,33.5702821824269,4.2910986865825));
#18380=CARTESIAN_POINT('Ctrl Pts',(25.5350579694096,32.933982905541,2.19783870908455));
#18381=CARTESIAN_POINT('Ctrl Pts',(25.4998719447396,32.7416529094252,1.10199792653042));
#18382=CARTESIAN_POINT('Ctrl Pts',(25.5758360411619,32.6822063330431,1.11022302462516E-15));
#18383=CARTESIAN_POINT('',(26.4205173989462,34.5572895402979,-6.16441400296898));
#18384=CARTESIAN_POINT('Ctrl Pts',(26.420520525129,34.5572945292832,-6.16442208610004));
#18385=CARTESIAN_POINT('Ctrl Pts',(26.0764769637365,34.0082451771012,-5.27485402124597));
#18386=CARTESIAN_POINT('Ctrl Pts',(25.8252695836875,33.5693302919173,-4.29007656912465));
#18387=CARTESIAN_POINT('Ctrl Pts',(25.5354420784007,32.9335238913062,-2.19706468924219));
#18388=CARTESIAN_POINT('Ctrl Pts',(25.4988436963722,32.7424575769983,-1.10157448609152));
#18389=CARTESIAN_POINT('Ctrl Pts',(25.5758360411619,32.6822063330431,-1.66533453693773E-15));
#18390=CARTESIAN_POINT('',(24.7547796990912,35.7694126601132,-6.16441400296897));
#18391=CARTESIAN_POINT('Origin',(-5.20417042793042E-15,1.73472347597681E-15,
-6.16441400296897));
#18392=CARTESIAN_POINT('',(24.152801657541,33.7474765292383,0.));
#18393=CARTESIAN_POINT('Ctrl Pts',(24.152801657541,33.7474765292382,1.11022302462516E-15));
#18394=CARTESIAN_POINT('Ctrl Pts',(24.0734889742688,33.8042399884658,-1.09898083808803));
#18395=CARTESIAN_POINT('Ctrl Pts',(24.0869995303267,34.0063342336128,-2.19052946960189));
#18396=CARTESIAN_POINT('Ctrl Pts',(24.2421693474788,34.5182194833125,-3.75889728453595));
#18397=CARTESIAN_POINT('Ctrl Pts',(24.3163449651184,34.723543634418,-4.26878718104901));
#18398=CARTESIAN_POINT('Ctrl Pts',(24.5057193682513,35.1998349128155,-5.24984087156284));
#18399=CARTESIAN_POINT('Ctrl Pts',(24.6207297677859,35.4697758585235,-5.71948809610186));
#18400=CARTESIAN_POINT('Ctrl Pts',(24.7547796990912,35.7694126601132,-6.16441400296901));
#18401=CARTESIAN_POINT('',(24.7550996672029,35.7691912190764,6.16441400296897));
#18402=CARTESIAN_POINT('Ctrl Pts',(24.152801657541,33.7474765292382,8.32667268468867E-16));
#18403=CARTESIAN_POINT('Ctrl Pts',(24.0746019944585,33.8034434087317,1.09861960926675));
#18404=CARTESIAN_POINT('Ctrl Pts',(24.0873861635413,34.0059051472516,2.18971594132777));
#18405=CARTESIAN_POINT('Ctrl Pts',(24.2930763407557,34.6897464310454,4.28292314717347));
#18406=CARTESIAN_POINT('Ctrl Pts',(24.4866606648092,35.1676910781172,5.27177304443343));
#18407=CARTESIAN_POINT('Ctrl Pts',(24.7550996672028,35.7691912190764,6.16441400296897));
#18408=CARTESIAN_POINT('Origin',(-1.73472347597681E-15,-1.73472347597681E-15,
6.16441400296896));
#18409=CARTESIAN_POINT('Origin',(0.,0.,-6.93889390390723E-15));
#18410=CARTESIAN_POINT('',(31.0697252215062,30.4453966086846,6.16441400296896));
#18411=CARTESIAN_POINT('',(29.9666738162744,28.7097276265209,0.));
#18412=CARTESIAN_POINT('Ctrl Pts',(31.0697252215062,30.4453966086846,6.16441400296899));
#18413=CARTESIAN_POINT('Ctrl Pts',(30.6516652743936,29.9507533455085,5.27531660683076));
#18414=CARTESIAN_POINT('Ctrl Pts',(30.3394714544406,29.5533355526259,4.29109868658263));
#18415=CARTESIAN_POINT('Ctrl Pts',(29.9621423486914,28.9647448012291,2.19783870908459));
#18416=CARTESIAN_POINT('Ctrl Pts',(29.8999430547262,28.7793799405671,1.1019979265305));
#18417=CARTESIAN_POINT('Ctrl Pts',(29.9666738162744,28.7097276265209,8.32667268468867E-16));
#18418=CARTESIAN_POINT('',(31.0696096991581,30.4455144995447,-6.16441400296899));
#18419=CARTESIAN_POINT('Ctrl Pts',(31.0696096991581,30.4455144995446,-6.16441400296901));
#18420=CARTESIAN_POINT('Ctrl Pts',(30.6509301353917,29.9510161819023,-5.27484593811529));
#18421=CARTESIAN_POINT('Ctrl Pts',(30.3398193877248,29.5523238483581,-4.29007656912537));
#18422=CARTESIAN_POINT('Ctrl Pts',(29.9624572234713,28.9642357946874,-2.19706468924242));
#18423=CARTESIAN_POINT('Ctrl Pts',(29.8990397885865,28.7803227527781,-1.10157448608938));
#18424=CARTESIAN_POINT('Ctrl Pts',(29.9666738162744,28.7097276265209,-1.94289029309402E-15));
#18425=CARTESIAN_POINT('',(29.5933299130458,31.8823591451078,-6.16441400296898));
#18426=CARTESIAN_POINT('Origin',(-5.20417042793042E-15,1.73472347597681E-15,
-6.16441400296897));
#18427=CARTESIAN_POINT('',(28.7097276265215,29.9666738162739,0.));
#18428=CARTESIAN_POINT('Ctrl Pts',(28.7097276265214,29.9666738162739,1.38777878078145E-15));
#18429=CARTESIAN_POINT('Ctrl Pts',(28.7009474204864,29.9750857383081,-0.137010845867973));
#18430=CARTESIAN_POINT('Ctrl Pts',(28.6939122150404,29.9855286660437,-0.273849719843528));
#18431=CARTESIAN_POINT('Ctrl Pts',(28.6833082731284,30.0104891974361,-0.547496131369053));
#18432=CARTESIAN_POINT('Ctrl Pts',(28.6797460897164,30.0250035906012,-0.684223919461066));
#18433=CARTESIAN_POINT('Ctrl Pts',(28.6742811955932,30.0746352811264,-1.09397285881146));
#18434=CARTESIAN_POINT('Ctrl Pts',(28.6776158428565,30.1158101338568,-1.36621764183717));
#18435=CARTESIAN_POINT('Ctrl Pts',(28.708474223108,30.2634298312027,-2.17875768610757));
#18436=CARTESIAN_POINT('Ctrl Pts',(28.7568689184051,30.3936948517435,-2.71300426677357));
#18437=CARTESIAN_POINT('Ctrl Pts',(28.907873841452,30.7168533707375,-3.75889728641903));
#18438=CARTESIAN_POINT('Ctrl Pts',(29.010515131592,30.9095313269397,-4.26878718252163));
#18439=CARTESIAN_POINT('Ctrl Pts',(29.2657452924933,31.3540238590871,-5.24984087225568));
#18440=CARTESIAN_POINT('Ctrl Pts',(29.4180016539271,31.6048495086171,-5.71948809643018));
#18441=CARTESIAN_POINT('Ctrl Pts',(29.5933299130457,31.8823591451077,-6.16441400296901));
#18442=CARTESIAN_POINT('',(29.593615110006,31.882094421804,6.16441400296896));
#18443=CARTESIAN_POINT('Ctrl Pts',(28.7097276265214,29.9666738162739,-8.32667268468867E-16));
#18444=CARTESIAN_POINT('Ctrl Pts',(28.6402888406582,30.0332000060362,1.09861960926672));
#18445=CARTESIAN_POINT('Ctrl Pts',(28.6817561949071,30.2317815990283,2.18971594132772));
#18446=CARTESIAN_POINT('Ctrl Pts',(28.9826735044059,30.8793896002661,4.28292314717346));
#18447=CARTESIAN_POINT('Ctrl Pts',(29.2423060343177,31.3249195382,5.27177304443341));
#18448=CARTESIAN_POINT('Ctrl Pts',(29.593615110006,31.882094421804,6.16441400296897));
#18449=CARTESIAN_POINT('Origin',(-1.73472347597681E-15,-1.73472347597681E-15,
6.16441400296896));
#18450=CARTESIAN_POINT('Origin',(0.,0.,-6.93889390390723E-15));
#18451=CARTESIAN_POINT('',(35.0863119121266,25.713823449751,6.16441400296896));
#18452=CARTESIAN_POINT('',(33.7474765292387,24.1528016575404,0.));
#18453=CARTESIAN_POINT('Ctrl Pts',(35.0863119121266,25.713823449751,6.16441400296898));
#18454=CARTESIAN_POINT('Ctrl Pts',(34.6021121364811,25.2837110755392,5.2753166068307));
#18455=CARTESIAN_POINT('Ctrl Pts',(34.2365375505478,24.9347682357555,4.2910986865825));
#18456=CARTESIAN_POINT('Ctrl Pts',(33.7792839134374,24.4058680201907,2.19783870908459));
#18457=CARTESIAN_POINT('Ctrl Pts',(33.6913375484341,24.2312417889975,1.10199792653051));
#18458=CARTESIAN_POINT('Ctrl Pts',(33.7474765292387,24.1528016575404,1.38777878078145E-15));
#18459=CARTESIAN_POINT('',(35.0862143432449,25.7139565812008,-6.16441400296898));
#18460=CARTESIAN_POINT('Ctrl Pts',(35.0862143432449,25.7139565812008,-6.16441400296901));
#18461=CARTESIAN_POINT('Ctrl Pts',(34.601421885651,25.2840758578288,-5.27484593811562));
#18462=CARTESIAN_POINT('Ctrl Pts',(34.2367379618438,24.933717313109,-4.29007656912498));
#18463=CARTESIAN_POINT('Ctrl Pts',(33.7795231440548,24.4053193832426,-2.19706468921364));
#18464=CARTESIAN_POINT('Ctrl Pts',(33.6905776524145,24.232303552906,-1.10157448593714));
#18465=CARTESIAN_POINT('Ctrl Pts',(33.7474765292387,24.1528016575404,5.55111512312578E-16));
#18466=CARTESIAN_POINT('',(33.8294452700945,27.346272739035,-6.16441400296899));
#18467=CARTESIAN_POINT('Origin',(-5.20417042793042E-15,1.73472347597681E-15,
-6.16441400296897));
#18468=CARTESIAN_POINT('',(32.6822063330436,25.5758360411613,0.));
#18469=CARTESIAN_POINT('Ctrl Pts',(32.6822063330436,25.5758360411613,3.12250225675825E-15));
#18470=CARTESIAN_POINT('Ctrl Pts',(32.6747126381706,25.5854118955592,-0.13701084587003));
#18471=CARTESIAN_POINT('Ctrl Pts',(32.6692352245446,25.5967497434724,-0.273849719845774));
#18472=CARTESIAN_POINT('Ctrl Pts',(32.6622914694609,25.6229653109225,-0.547496131372112));
#18473=CARTESIAN_POINT('Ctrl Pts',(32.6608311574562,25.637838920049,-0.684223919464382));
#18474=CARTESIAN_POINT('Ctrl Pts',(32.6624852140865,25.6877431670502,-1.09397285881505));
#18475=CARTESIAN_POINT('Ctrl Pts',(32.6716457119561,25.7280243493632,-1.36621764184054));
#18476=CARTESIAN_POINT('Ctrl Pts',(32.7231984717437,25.8697498856463,-2.17875768610944));
#18477=CARTESIAN_POINT('Ctrl Pts',(32.7896392241513,25.991801712872,-2.7130042667745));
#18478=CARTESIAN_POINT('Ctrl Pts',(32.9850973871782,26.290180702898,-3.75889728641806));
#18479=CARTESIAN_POINT('Ctrl Pts',(33.1141148691575,26.4662900967167,-4.26878718251969));
#18480=CARTESIAN_POINT('Ctrl Pts',(33.4300050378579,26.8699352967219,-5.24984087225438));
#18481=CARTESIAN_POINT('Ctrl Pts',(33.6164113967186,27.0965438053519,-5.7194964494206));
#18482=CARTESIAN_POINT('Ctrl Pts',(33.8294491231113,27.3462772557344,-6.16442204993664));
#18483=CARTESIAN_POINT('',(33.8296898901082,27.3459701224717,6.16441400296896));
#18484=CARTESIAN_POINT('Ctrl Pts',(32.6822063330436,25.5758360411613,-2.22044604925031E-15));
#18485=CARTESIAN_POINT('Ctrl Pts',(32.622941997835,25.6515672598147,1.0986196092667));
#18486=CARTESIAN_POINT('Ctrl Pts',(32.6922483814993,25.8422261587076,2.18971594132768));
#18487=CARTESIAN_POINT('Ctrl Pts',(33.082267014635,26.4404174460315,4.2829231471735));
#18488=CARTESIAN_POINT('Ctrl Pts',(33.4026623808145,26.8444629700935,5.27177304443349));
#18489=CARTESIAN_POINT('Ctrl Pts',(33.8296898901081,27.3459701224717,6.16441400296898));
#18490=CARTESIAN_POINT('Origin',(-1.73472347597681E-15,-1.73472347597681E-15,
6.16441400296896));
#18491=CARTESIAN_POINT('Origin',(0.,0.,-6.93889390390723E-15));
#18492=CARTESIAN_POINT('',(38.3886424727845,20.4587909979239,6.16441400296896));
#18493=CARTESIAN_POINT('',(36.8412779397543,19.1041942977414,6.93889390390723E-15));
#18494=CARTESIAN_POINT('Ctrl Pts',(38.3886424727844,20.4587909979239,6.16441400296899));
#18495=CARTESIAN_POINT('Ctrl Pts',(37.8481597797213,20.1019653602737,5.27531660683076));
#18496=CARTESIAN_POINT('Ctrl Pts',(37.4366464721474,19.808600943539,4.29109868658265));
#18497=CARTESIAN_POINT('Ctrl Pts',(36.9087766691159,19.3501581469721,2.19783870908195));
#18498=CARTESIAN_POINT('Ctrl Pts',(36.7968735674506,19.1898254317345,1.10199792652477));
#18499=CARTESIAN_POINT('Ctrl Pts',(36.8412779397536,19.1041942977407,3.33066907387547E-14));
#18500=CARTESIAN_POINT('',(38.3885648435948,20.4589366597857,-6.16441400296898));
#18501=CARTESIAN_POINT('Ctrl Pts',(38.3885648435948,20.4589366597857,-6.16441400296902));
#18502=CARTESIAN_POINT('Ctrl Pts',(37.8475284685813,20.1024246625415,-5.27484593811522));
#18503=CARTESIAN_POINT('Ctrl Pts',(37.4366952816589,19.8075321962687,-4.29007656912551));
#18504=CARTESIAN_POINT('Ctrl Pts',(36.9089353855233,19.3495810482744,-2.19706468916407));
#18505=CARTESIAN_POINT('Ctrl Pts',(36.7962725108494,19.19098453287,-1.10157448567205));
#18506=CARTESIAN_POINT('Ctrl Pts',(36.8412779397536,19.1041942977407,-2.02615701994091E-14));
#18507=CARTESIAN_POINT('',(37.3768906775087,22.2534950801344,-6.16441400296898));
#18508=CARTESIAN_POINT('Origin',(-5.20417042793042E-15,1.73472347597681E-15,
-6.16441400296897));
#18509=CARTESIAN_POINT('',(35.9893695663253,20.6643479988714,0.));
#18510=CARTESIAN_POINT('Ctrl Pts',(35.9893695663253,20.6643479988713,1.94289029309402E-15));
#18511=CARTESIAN_POINT('Ctrl Pts',(35.9833149326307,20.6748928488533,-0.137010845865106));
#18512=CARTESIAN_POINT('Ctrl Pts',(35.9795068151691,20.6868948110578,-0.273849719841543));
#18513=CARTESIAN_POINT('Ctrl Pts',(35.9763646017412,20.7138317412138,-0.547496131366511));
#18514=CARTESIAN_POINT('Ctrl Pts',(35.9770358888841,20.7287617825126,-0.684223919458269));
#18515=CARTESIAN_POINT('Ctrl Pts',(35.985775224443,20.7779226794343,-1.09397285880729));
#18516=CARTESIAN_POINT('Ctrl Pts',(36.0005750915987,20.8164901826193,-1.36621764183265));
#18517=CARTESIAN_POINT('Ctrl Pts',(36.0717727653998,20.9494364346224,-2.17875768610445));
#18518=CARTESIAN_POINT('Ctrl Pts',(36.1549070328013,21.0607904452962,-2.71300426677191));
#18519=CARTESIAN_POINT('Ctrl Pts',(36.390839471268,21.3283157705684,-3.75889728641864));
#18520=CARTESIAN_POINT('Ctrl Pts',(36.5436067212089,21.4842715226041,-4.2687871825207));
#18521=CARTESIAN_POINT('Ctrl Pts',(36.9137262848261,21.8388523382117,-5.24984087225524));
#18522=CARTESIAN_POINT('Ctrl Pts',(37.1304809453721,22.0366222125383,-5.71948809642998));
#18523=CARTESIAN_POINT('Ctrl Pts',(37.3768906775087,22.2534950801344,-6.16441400296901));
#18524=CARTESIAN_POINT('',(37.3770897408174,22.2531607307117,6.16441400296896));
#18525=CARTESIAN_POINT('Ctrl Pts',(35.9893695663253,20.6643479988713,2.77555756156289E-16));
#18526=CARTESIAN_POINT('Ctrl Pts',(35.9414861327319,20.7477425771949,1.09861960926664));
#18527=CARTESIAN_POINT('Ctrl Pts',(36.0372206677033,20.9265975166219,2.18971594132757));
#18528=CARTESIAN_POINT('Ctrl Pts',(36.5084009698262,21.4631946404632,4.28292314717355));
#18529=CARTESIAN_POINT('Ctrl Pts',(36.8830368465619,21.8175305489545,5.27177304443358));
#18530=CARTESIAN_POINT('Ctrl Pts',(37.3770897408173,22.2531607307117,6.16441400296898));
#18531=CARTESIAN_POINT('Origin',(-1.73472347597681E-15,-1.73472347597681E-15,
6.16441400296896));
#18532=CARTESIAN_POINT('Origin',(0.,0.,-6.93889390390723E-15));
#18533=CARTESIAN_POINT('',(40.9094909763996,14.7872765596604,6.16441400296896));
#18534=CARTESIAN_POINT('',(39.1850971728875,13.666680633986,0.));
#18535=CARTESIAN_POINT('Ctrl Pts',(40.9094909763996,14.7872765596603,6.16441400296898));
#18536=CARTESIAN_POINT('Ctrl Pts',(40.3237280349262,14.5110015995542,5.27531660683077));
#18537=CARTESIAN_POINT('Ctrl Pts',(39.8746532299475,14.2791876593999,4.29109868658268));
#18538=CARTESIAN_POINT('Ctrl Pts',(39.2869131679352,13.9005348551303,2.19783870908451));
#18539=CARTESIAN_POINT('Ctrl Pts',(39.153331354054,13.757759567569,1.10199792653032));
#18540=CARTESIAN_POINT('Ctrl Pts',(39.1850971728875,13.666680633986,1.66533453693773E-15));
#18541=CARTESIAN_POINT('',(40.9094348672085,14.7874317866772,-6.16441400296898));
#18542=CARTESIAN_POINT('Ctrl Pts',(40.9094348672084,14.7874317866772,-6.164414002969));
#18543=CARTESIAN_POINT('Ctrl Pts',(40.3231685151537,14.5115460717244,-5.27484593811583));
#18544=CARTESIAN_POINT('Ctrl Pts',(39.8745494440533,14.2781228441186,-4.29007656912527));
#18545=CARTESIAN_POINT('Ctrl Pts',(39.2869881391103,13.8999410427645,-2.1970646891068));
#18546=CARTESIAN_POINT('Ctrl Pts',(39.1529013726389,13.7589924099824,-1.10157448537221));
#18547=CARTESIAN_POINT('Ctrl Pts',(39.1850971728875,13.666680633986,-8.32667268468867E-16));
#18548=CARTESIAN_POINT('',(40.1634503767828,16.7077004351798,-6.16441400296898));
#18549=CARTESIAN_POINT('Origin',(-5.20417042793042E-15,1.73472347597681E-15,
-6.16441400296897));
#18550=CARTESIAN_POINT('',(38.5638930200082,15.3321934223831,0.));
#18551=CARTESIAN_POINT('Ctrl Pts',(38.5638930200081,15.3321934223831,1.38777878078145E-16));
#18552=CARTESIAN_POINT('Ctrl Pts',(38.5594007023748,15.3434926052104,-0.137010845860786));
#18553=CARTESIAN_POINT('Ctrl Pts',(38.5573394033684,15.3559143563653,-0.273849719841182));
#18554=CARTESIAN_POINT('Ctrl Pts',(38.5580626980017,15.3830242910068,-0.54749613136722));
#18555=CARTESIAN_POINT('Ctrl Pts',(38.5608519188225,15.3977068318908,-0.684223919458968));
#18556=CARTESIAN_POINT('Ctrl Pts',(38.5764986256418,15.4451236046381,-1.09397285880846));
#18557=CARTESIAN_POINT('Ctrl Pts',(38.5966365794681,15.4811923055493,-1.36621764183395));
#18558=CARTESIAN_POINT('Ctrl Pts',(38.6860297879615,15.602652870967,-2.17875768610512));
#18559=CARTESIAN_POINT('Ctrl Pts',(38.7841651964102,15.7010422185523,-2.7130042667723));
#18560=CARTESIAN_POINT('Ctrl Pts',(39.0557690062388,15.9322678349323,-3.75889728641943));
#18561=CARTESIAN_POINT('Ctrl Pts',(39.2291761234756,16.0648951358156,-4.26878718252243));
#18562=CARTESIAN_POINT('Ctrl Pts',(39.6459905150316,16.3631933241455,-5.24984087225649));
#18563=CARTESIAN_POINT('Ctrl Pts',(39.8886845133482,16.5281027818499,-5.71948809643058));
#18564=CARTESIAN_POINT('Ctrl Pts',(40.1634503767828,16.7077004351798,-6.164414002969));
#18565=CARTESIAN_POINT('',(40.1635998310295,16.7073411592907,6.16441400296896));
#18566=CARTESIAN_POINT('Ctrl Pts',(38.5638930200081,15.3321934223831,-8.32667268468867E-16));
#18567=CARTESIAN_POINT('Ctrl Pts',(38.5283652566535,15.4215536872522,1.0986196092665));
#18568=CARTESIAN_POINT('Ctrl Pts',(38.6485790638755,15.5849636964217,2.18971594132732));
#18569=CARTESIAN_POINT('Ctrl Pts',(39.1913291628061,16.0490430867574,4.28292314717371));
#18570=CARTESIAN_POINT('Ctrl Pts',(39.6125790440085,16.3464561224015,5.27177304443379));
#18571=CARTESIAN_POINT('Ctrl Pts',(40.1635998310295,16.7073411592907,6.16441400296898));
#18572=CARTESIAN_POINT('Origin',(-1.73472347597681E-15,-1.73472347597681E-15,
6.16441400296896));
#18573=CARTESIAN_POINT('Origin',(0.,0.,-6.93889390390723E-15));
#18574=CARTESIAN_POINT('',(42.5975402169653,8.81473581362642,6.16441400296896));
#18575=CARTESIAN_POINT('',(40.7312208280703,7.9509527639758,0.));
#18576=CARTESIAN_POINT('Ctrl Pts',(42.5975402169653,8.8147358136264,6.16441400296897));
#18577=CARTESIAN_POINT('Ctrl Pts',(41.9783611257759,8.62461716345458,5.27522994637944));
#18578=CARTESIAN_POINT('Ctrl Pts',(41.5008344149426,8.45905891928459,4.29090746118671));
#18579=CARTESIAN_POINT('Ctrl Pts',(40.865251830097,8.16791310841239,2.19762693960535));
#18580=CARTESIAN_POINT('Ctrl Pts',(40.7127420143401,8.04561621690129,1.10189111929206));
#18581=CARTESIAN_POINT('Ctrl Pts',(40.7312208280703,7.95095276397578,3.05311331771918E-15));
#18582=CARTESIAN_POINT('',(42.5975067699923,8.81489744582799,-6.16441400296898));
#18583=CARTESIAN_POINT('Ctrl Pts',(42.5975067699923,8.81489744582797,-6.164414002969));
#18584=CARTESIAN_POINT('Ctrl Pts',(41.9779451331701,8.62525425073588,-5.27484593811595));
#18585=CARTESIAN_POINT('Ctrl Pts',(41.5006727684721,8.45805208556826,-4.29007656912516));
#18586=CARTESIAN_POINT('Ctrl Pts',(40.8652711085094,8.16733832174138,-2.19706468906351));
#18587=CARTESIAN_POINT('Ctrl Pts',(40.7124900701213,8.04690687928061,-1.10157448514352));
#18588=CARTESIAN_POINT('Ctrl Pts',(40.7312208280703,7.95095276397578,-1.38777878078145E-15));
#18589=CARTESIAN_POINT('',(42.1323980482129,10.8217851903902,-6.16441400296898));
#18590=CARTESIAN_POINT('Origin',(-5.20417042793042E-15,1.73472347597681E-15,
-6.16441400296897));
#18591=CARTESIAN_POINT('',(40.3533668208877,9.68791960220985,0.));
#18592=CARTESIAN_POINT('Ctrl Pts',(40.3533668208877,9.68791960220986,1.17961196366423E-15));
#18593=CARTESIAN_POINT('Ctrl Pts',(40.3505282699472,9.69974309910533,-0.137010845854389));
#18594=CARTESIAN_POINT('Ctrl Pts',(40.3502557514989,9.71233176817958,-0.273849719838591));
#18595=CARTESIAN_POINT('Ctrl Pts',(40.3548298299996,9.73906282721793,-0.547496131365122));
#18596=CARTESIAN_POINT('Ctrl Pts',(40.3596802040054,9.75319897349669,-0.684223919456776));
#18597=CARTESIAN_POINT('Ctrl Pts',(40.3819157602544,9.79790635331761,-1.09397285880488));
#18598=CARTESIAN_POINT('Ctrl Pts',(40.4069818500837,9.83074199721934,-1.36621764183001));
#18599=CARTESIAN_POINT('Ctrl Pts',(40.5127508053323,9.9382442892057,-2.17875768610251));
#18600=CARTESIAN_POINT('Ctrl Pts',(40.623889600912,10.0216660503167,-2.71300426677077));
#18601=CARTESIAN_POINT('Ctrl Pts',(40.9256357117777,10.2118848710475,-3.75889728641811));
#18602=CARTESIAN_POINT('Ctrl Pts',(41.1161526274704,10.3184838113887,-4.26878718252017));
#18603=CARTESIAN_POINT('Ctrl Pts',(41.5711767079479,10.5544268815438,-5.24984087225546));
#18604=CARTESIAN_POINT('Ctrl Pts',(41.8348694941005,10.683118841629,-5.71948809643011));
#18605=CARTESIAN_POINT('Ctrl Pts',(42.1323980482129,10.8217851903902,-6.164414002969));
#18606=CARTESIAN_POINT('',(42.1324948509395,10.8214083018598,6.16441400296896));
#18607=CARTESIAN_POINT('Ctrl Pts',(40.3533668208877,9.68791960220987,-5.55111512312578E-16));
#18608=CARTESIAN_POINT('Ctrl Pts',(40.3309179705801,9.78142643632542,1.09861960926657));
#18609=CARTESIAN_POINT('Ctrl Pts',(40.4731638436058,9.92606495868641,2.18971594132745));
#18610=CARTESIAN_POINT('Ctrl Pts',(41.0764349124919,10.3081792974235,4.2829231471736));
#18611=CARTESIAN_POINT('Ctrl Pts',(41.5357233653638,10.542614988483,5.27177304443365));
#18612=CARTESIAN_POINT('Ctrl Pts',(42.1324948509395,10.8214083018599,6.16441400296898));
#18613=CARTESIAN_POINT('Origin',(-1.73472347597681E-15,-1.73472347597681E-15,
6.16441400296896));
#18614=CARTESIAN_POINT('Origin',(0.,0.,-6.93889390390723E-15));
#18615=CARTESIAN_POINT('',(43.4184263798756,2.66275246602602,6.16441400296896));
#18616=CARTESIAN_POINT('',(41.448174286335,2.07336642434544,0.));
#18617=CARTESIAN_POINT('Ctrl Pts',(43.4184263798756,2.66275246602601,6.16441400296898));
#18618=CARTESIAN_POINT('Ctrl Pts',(42.7784929341,2.5626873218093,5.27522994637943));
#18619=CARTESIAN_POINT('Ctrl Pts',(42.2822653619025,2.46677335847309,4.29090746118668));
#18620=CARTESIAN_POINT('Ctrl Pts',(41.611717722348,2.26904382492961,2.19762693960537));
#18621=CARTESIAN_POINT('Ctrl Pts',(41.4433555742777,2.16969614920107,1.10189111929209));
#18622=CARTESIAN_POINT('Ctrl Pts',(41.4481742863349,2.07336642434542,1.11022302462516E-15));
#18623=CARTESIAN_POINT('',(43.4184162760054,2.6629172130419,-6.16441400296898));
#18624=CARTESIAN_POINT('Ctrl Pts',(43.4184162760054,2.66291721304189,-6.16441400296901));
#18625=CARTESIAN_POINT('Ctrl Pts',(42.7781718430444,2.56337712643548,-5.27484593863236));
#18626=CARTESIAN_POINT('Ctrl Pts',(42.2819620739562,2.46579977767809,-4.29007657026531));
#18627=CARTESIAN_POINT('Ctrl Pts',(41.7796712516364,2.31793342925177,-2.72168992254993));
#18628=CARTESIAN_POINT('Ctrl Pts',(41.6533701498395,2.26867967212385,-2.18495234742919));
#18629=CARTESIAN_POINT('Ctrl Pts',(41.5280596821275,2.19513167299008,-1.36923477587661));
#18630=CARTESIAN_POINT('Ctrl Pts',(41.4970265580502,2.17071604491098,-1.09614446424856));
#18631=CARTESIAN_POINT('Ctrl Pts',(41.4666087795881,2.1341518904505,-0.685318587183261));
#18632=CARTESIAN_POINT('Ctrl Pts',(41.4591607204606,2.12198419003006,-0.548301186434216));
#18633=CARTESIAN_POINT('Ctrl Pts',(41.4496393847912,2.09766071948028,-0.274113036173078));
#18634=CARTESIAN_POINT('Ctrl Pts',(41.447566672806,2.08551308166182,-0.137034229955334));
#18635=CARTESIAN_POINT('Ctrl Pts',(41.4481742863349,2.07336642434541,-2.0122792321331E-15));
#18636=CARTESIAN_POINT('',(43.2436515951818,4.71556960658337,-6.16441400296898));
#18637=CARTESIAN_POINT('Origin',(-5.20417042793042E-15,1.73472347597681E-15,
-6.16441400296897));
#18638=CARTESIAN_POINT('',(41.3213624427944,3.84642767658874,0.));
#18639=CARTESIAN_POINT('Ctrl Pts',(41.3213624427943,3.84642767658874,1.73472347597681E-16));
#18640=CARTESIAN_POINT('Ctrl Pts',(41.3202354432581,3.85853479525182,-0.137010845851213));
#18641=CARTESIAN_POINT('Ctrl Pts',(41.321757253058,3.87103411324551,-0.273849719837603));
#18642=CARTESIAN_POINT('Ctrl Pts',(41.3300890003786,3.89684212940388,-0.547496131362626));
#18643=CARTESIAN_POINT('Ctrl Pts',(41.336901787942,3.91014410990395,-0.684223919453106));
#18644=CARTESIAN_POINT('Ctrl Pts',(41.3652735418183,3.95123198346985,-1.09397285880268));
#18645=CARTESIAN_POINT('Ctrl Pts',(41.3947574943469,3.98016613134156,-1.36621764182791));
#18646=CARTESIAN_POINT('Ctrl Pts',(41.5147490454351,4.0715217132403,-2.17875768610036));
#18647=CARTESIAN_POINT('Ctrl Pts',(41.6366287627659,4.13827766138837,-2.71300426676958));
#18648=CARTESIAN_POINT('Ctrl Pts',(41.9623744940145,4.2836173798294,-3.75889728641934));
#18649=CARTESIAN_POINT('Ctrl Pts',(42.1661228331635,4.36201791261592,-4.26878718252248));
#18650=CARTESIAN_POINT('Ctrl Pts',(42.6500936244634,4.53080274409635,-5.24984087225778));
#18651=CARTESIAN_POINT('Ctrl Pts',(42.9294171737525,4.6206574093722,-5.71948809643132));
#18652=CARTESIAN_POINT('Ctrl Pts',(43.2436515951818,4.71556960658337,-6.16441400296901));
#18653=CARTESIAN_POINT('',(43.2436937757662,4.71518277776774,6.16441400296896));
#18654=CARTESIAN_POINT('Ctrl Pts',(41.3213624427943,3.84642767658874,-8.32667268468867E-16));
#18655=CARTESIAN_POINT('Ctrl Pts',(41.3124474863202,3.94219917643307,1.09886774242324));
#18656=CARTESIAN_POINT('Ctrl Pts',(41.4739046363274,4.06515557324188,2.190207356141));
#18657=CARTESIAN_POINT('Ctrl Pts',(42.1255613966704,4.35754593773624,4.28336653879353));
#18658=CARTESIAN_POINT('Ctrl Pts',(42.613461821837,4.52419955110993,5.27197367572233));
#18659=CARTESIAN_POINT('Ctrl Pts',(43.2436937757662,4.71518277776774,6.16441400296897));
#18660=CARTESIAN_POINT('Origin',(-1.73472347597681E-15,-1.73472347597681E-15,
6.16441400296896));
#18661=CARTESIAN_POINT('Origin',(0.,0.,-6.93889390390723E-15));
#18662=CARTESIAN_POINT('',(43.3554385900938,-3.54343684303869,6.16441400296896));
#18663=CARTESIAN_POINT('',(41.3213624427943,-3.84642767658963,0.));
#18664=CARTESIAN_POINT('Ctrl Pts',(43.3554444774928,-3.5434367705481,6.16442208586934));
#18665=CARTESIAN_POINT('Ctrl Pts',(42.7077838766714,-3.55141137103749,5.27523802927978));
#18666=CARTESIAN_POINT('Ctrl Pts',(42.2029513180785,-3.57572859433001,4.29090746118662));
#18667=CARTESIAN_POINT('Ctrl Pts',(41.5110890400568,-3.67601664744674,2.19762693960542));
#18668=CARTESIAN_POINT('Ctrl Pts',(41.3303019274915,-3.75039267520991,1.10189111929219));
#18669=CARTESIAN_POINT('Ctrl Pts',(41.3213624427942,-3.84642767658964,5.55111512312578E-16));
#18670=CARTESIAN_POINT('',(43.3554520350114,-3.54327233497894,-6.16441400296897));
#18671=CARTESIAN_POINT('Ctrl Pts',(43.3554520350114,-3.54327233497896,-6.16441400296899));
#18672=CARTESIAN_POINT('Ctrl Pts',(42.7075583358946,-3.55068296409579,-5.27484593863224));
#18673=CARTESIAN_POINT('Ctrl Pts',(42.2025125621728,-3.57664910310152,-4.29007657026532));
#18674=CARTESIAN_POINT('Ctrl Pts',(41.6842907607187,-3.6515269481625,-2.7216899225514));
#18675=CARTESIAN_POINT('Ctrl Pts',(41.5522656815471,-3.68230485218473,-2.18495234743192));
#18676=CARTESIAN_POINT('Ctrl Pts',(41.4177637221115,-3.73727069978806,-1.36923477588026));
#18677=CARTESIAN_POINT('Ctrl Pts',(41.3835717643297,-3.75702133794349,-1.09614446425197));
#18678=CARTESIAN_POINT('Ctrl Pts',(41.3482599732647,-3.78888442081007,-0.68531858718678));
#18679=CARTESIAN_POINT('Ctrl Pts',(41.3391560803224,-3.79986830225437,-0.548301186437842));
#18680=CARTESIAN_POINT('Ctrl Pts',(41.3262700673438,-3.82258916759967,-0.274113036173981));
#18681=CARTESIAN_POINT('Ctrl Pts',(41.3224896634664,-3.8343181823096,-0.137034229955792));
#18682=CARTESIAN_POINT('Ctrl Pts',(41.3213624427942,-3.84642767658964,-4.85722573273506E-16));
#18683=CARTESIAN_POINT('',(43.4745891000668,-1.48664137583804,-6.16441400296898));
#18684=CARTESIAN_POINT('Origin',(-5.20417042793042E-15,1.73472347597681E-15,
-6.16441400296897));
#18685=CARTESIAN_POINT('',(41.4481742863349,-2.07336642434629,1.04083408558608E-14));
#18686=CARTESIAN_POINT('Ctrl Pts',(41.4481742863349,-2.07336642434628,1.11022302462516E-14));
#18687=CARTESIAN_POINT('Ctrl Pts',(41.4530470730269,-1.97595570634813,-1.09898083808598));
#18688=CARTESIAN_POINT('Ctrl Pts',(41.6303639287926,-1.87806111146117,-2.19052946960028));
#18689=CARTESIAN_POINT('Ctrl Pts',(42.1448803402979,-1.73185220848821,-3.75889728453942));
#18690=CARTESIAN_POINT('Ctrl Pts',(42.3577123743482,-1.68324609198078,-4.26878718105493));
#18691=CARTESIAN_POINT('Ctrl Pts',(42.8607776270729,-1.58505547153932,-5.24984087156854));
#18692=CARTESIAN_POINT('Ctrl Pts',(43.1500457177245,-1.53586728290387,-5.71948809610463));
#18693=CARTESIAN_POINT('Ctrl Pts',(43.4745891000668,-1.48664137583802,-6.164414002969));
#18694=CARTESIAN_POINT('',(43.4745757998335,-1.48703027021543,6.16441400296897));
#18695=CARTESIAN_POINT('Ctrl Pts',(41.4481742863349,-2.07336642434627,7.7715611723761E-15));
#18696=CARTESIAN_POINT('Ctrl Pts',(41.4529797767749,-1.97730100969043,1.09886774242324));
#18697=CARTESIAN_POINT('Ctrl Pts',(41.6302920455235,-1.87857387990399,2.19020735614099));
#18698=CARTESIAN_POINT('Ctrl Pts',(42.3169273670934,-1.68190005418599,4.2833665387936));
#18699=CARTESIAN_POINT('Ctrl Pts',(42.8235789514612,-1.58637820440283,5.27197367572244));
#18700=CARTESIAN_POINT('Ctrl Pts',(43.4745757998334,-1.48703027021542,6.16441400296898));
#18701=CARTESIAN_POINT('Origin',(-1.73472347597681E-15,-1.73472347597681E-15,
6.16441400296896));
#18702=CARTESIAN_POINT('Origin',(0.,0.,-6.93889390390723E-15));
#18703=CARTESIAN_POINT('',(42.4098590973783,-9.6774919964071,6.16441400296896));
#18704=CARTESIAN_POINT('',(40.3533668208875,-9.68791960221073,0.));
#18705=CARTESIAN_POINT('Ctrl Pts',(42.4098590973783,-9.67749199640711,6.16441400296899));
#18706=CARTESIAN_POINT('Ctrl Pts',(41.7676558436448,-9.59321371330007,5.27522994637944));
#18707=CARTESIAN_POINT('Ctrl Pts',(41.26450688868,-9.54543902450228,4.29090746118668));
#18708=CARTESIAN_POINT('Ctrl Pts',(40.5654142930054,-9.54624402163765,2.19762693960537));
#18709=CARTESIAN_POINT('Ctrl Pts',(40.3758825202101,-9.59413431999296,1.10189111929208));
#18710=CARTESIAN_POINT('Ctrl Pts',(40.3533668208875,-9.68791960221072,1.38777878078145E-15));
#18711=CARTESIAN_POINT('',(42.4098958173846,-9.67733107621065,-6.16441400296897));
#18712=CARTESIAN_POINT('Ctrl Pts',(42.4098958173845,-9.67733107621065,-6.16441400296901));
#18713=CARTESIAN_POINT('Ctrl Pts',(41.7675420990818,-9.59246138875226,-5.27484593811599));
#18714=CARTESIAN_POINT('Ctrl Pts',(41.2639415960371,-9.54628772229384,-4.29007656912504));
#18715=CARTESIAN_POINT('Ctrl Pts',(40.5651930542684,-9.54677487452529,-2.19706468910702));
#18716=CARTESIAN_POINT('Ctrl Pts',(40.3761895042215,-9.59285563076689,-1.10157448537428));
#18717=CARTESIAN_POINT('Ctrl Pts',(40.3533668208875,-9.68791960221073,-8.32667268468867E-16));
#18718=CARTESIAN_POINT('',(42.8205093412358,-7.65858862696908,-6.16441400296897));
#18719=CARTESIAN_POINT('Origin',(-5.20417042793042E-15,1.73472347597681E-15,
-6.16441400296897));
#18720=CARTESIAN_POINT('',(40.7312208280701,-7.95095276397668,0.));
#18721=CARTESIAN_POINT('Ctrl Pts',(40.7312208280701,-7.95095276397666,2.4980018054066E-15));
#18722=CARTESIAN_POINT('Ctrl Pts',(40.7499070073971,-7.85522701648535,-1.09898083808689));
#18723=CARTESIAN_POINT('Ctrl Pts',(40.93935088668,-7.78356366707505,-2.19052946960111));
#18724=CARTESIAN_POINT('Ctrl Pts',(41.4694379593684,-7.71206627980807,-3.75889728453886));
#18725=CARTESIAN_POINT('Ctrl Pts',(41.6870210418007,-7.69424405998532,-4.26878718105426));
#18726=CARTESIAN_POINT('Ctrl Pts',(42.1989397978802,-7.66864652856466,-5.24984087156736));
#18727=CARTESIAN_POINT('Ctrl Pts',(42.4922637655696,-7.66112614630714,-5.71948809610396));
#18728=CARTESIAN_POINT('Ctrl Pts',(42.8205093412358,-7.65858862696907,-6.16441400296899));
#18729=CARTESIAN_POINT('',(42.8204408309399,-7.65897167013825,6.16441400296896));
#18730=CARTESIAN_POINT('Ctrl Pts',(40.7312208280701,-7.95095276397667,-1.11022302462516E-15));
#18731=CARTESIAN_POINT('Ctrl Pts',(40.7496489394968,-7.85654904932192,1.09886774242332));
#18732=CARTESIAN_POINT('Ctrl Pts',(40.9392067605215,-7.78406098621475,2.19020735614115));
#18733=CARTESIAN_POINT('Ctrl Pts',(41.6468427282638,-7.68710741120429,4.28336653879352));
#18734=CARTESIAN_POINT('Ctrl Pts',(42.1619315066373,-7.66466187441098,5.27197367572231));
#18735=CARTESIAN_POINT('Ctrl Pts',(42.8204408309398,-7.65897167013822,6.16441400296896));
#18736=CARTESIAN_POINT('Origin',(-1.73472347597681E-15,-1.73472347597681E-15,
6.16441400296896));
#18737=CARTESIAN_POINT('Origin',(0.,0.,-6.93889390390723E-15));
#18738=CARTESIAN_POINT('',(40.6009371733745,-15.6145413203111,6.16441400296896));
#18739=CARTESIAN_POINT('',(38.5638930200078,-15.332193422384,1.04083408558608E-14));
#18740=CARTESIAN_POINT('Ctrl Pts',(40.6009371733744,-15.6145413203111,6.16441400296898));
#18741=CARTESIAN_POINT('Ctrl Pts',(39.9772646730137,-15.4397258164132,5.27522994637943));
#18742=CARTESIAN_POINT('Ctrl Pts',(39.4860360960394,-15.3208318429088,4.29090746118668));
#18743=CARTESIAN_POINT('Ctrl Pts',(38.7939446919434,-15.2221373966425,2.19762693960533));
#18744=CARTESIAN_POINT('Ctrl Pts',(38.5995265792476,-15.2425670572197,1.10189111929201));
#18745=CARTESIAN_POINT('Ctrl Pts',(38.5638930200078,-15.332193422384,1.19348975147204E-14));
#18746=CARTESIAN_POINT('',(40.600996420953,-15.614387263859,-6.16441400296897));
#18747=CARTESIAN_POINT('Ctrl Pts',(40.6010020885968,-15.6143888578498,-6.16442208610001));
#18748=CARTESIAN_POINT('Ctrl Pts',(39.9772648207935,-15.4389665559052,-5.27485402124762));
#18749=CARTESIAN_POINT('Ctrl Pts',(39.485355774973,-15.3215914526464,-4.29007656912584));
#18750=CARTESIAN_POINT('Ctrl Pts',(38.793650156874,-15.2226313606578,-2.19706468916126));
#18751=CARTESIAN_POINT('Ctrl Pts',(38.6000124150605,-15.2413450715717,-1.10157448565927));
#18752=CARTESIAN_POINT('Ctrl Pts',(38.5638930200078,-15.332193422384,8.88178419700125E-15));
#18753=CARTESIAN_POINT('',(41.2947274963709,-13.6746290991923,-6.16441400296897));
#18754=CARTESIAN_POINT('Origin',(-5.20417042793042E-15,1.73472347597681E-15,
-6.16441400296897));
#18755=CARTESIAN_POINT('',(39.1850971728872,-13.6666806339868,0.));
#18756=CARTESIAN_POINT('Ctrl Pts',(39.1850971728872,-13.6666806339868,1.04083408558608E-16));
#18757=CARTESIAN_POINT('Ctrl Pts',(39.189101496907,-13.6551994389527,-0.137010845854338));
#18758=CARTESIAN_POINT('Ctrl Pts',(39.1956781881385,-13.6444618420239,-0.273849719838171));
#18759=CARTESIAN_POINT('Ctrl Pts',(39.2139780494464,-13.6244471777117,-0.547496131363631));
#18760=CARTESIAN_POINT('Ctrl Pts',(39.225701021394,-13.6151774048816,-0.684223919454616));
#18761=CARTESIAN_POINT('Ctrl Pts',(39.2685773960156,-13.5895886129705,-1.09397285880303));
#18762=CARTESIAN_POINT('Ctrl Pts',(39.3074166219997,-13.5755172628307,-1.36621764182805));
#18763=CARTESIAN_POINT('Ctrl Pts',(39.4545152562845,-13.5422635943353,-2.17875768610048));
#18764=CARTESIAN_POINT('Ctrl Pts',(39.5931123698217,-13.5321709123776,-2.71300426676969));
#18765=CARTESIAN_POINT('Ctrl Pts',(39.9497974103409,-13.53528492147,-3.7588972864178));
#18766=CARTESIAN_POINT('Ctrl Pts',(40.1677021769761,-13.5486094073543,-4.26878718251924));
#18767=CARTESIAN_POINT('Ctrl Pts',(40.6780532465233,-13.5961260568701,-5.24984087225545));
#18768=CARTESIAN_POINT('Ctrl Pts',(40.9694618609575,-13.6304265742619,-5.71948809643021));
#18769=CARTESIAN_POINT('Ctrl Pts',(41.2947274963708,-13.6746290991923,-6.164414002969));
#18770=CARTESIAN_POINT('',(41.2946051706827,-13.6749984935074,6.16441400296896));
#18771=CARTESIAN_POINT('Ctrl Pts',(39.1850971728872,-13.6666806339868,1.66533453693773E-15));
#18772=CARTESIAN_POINT('Ctrl Pts',(39.2167727620941,-13.5758604067257,1.09886774242333));
#18773=CARTESIAN_POINT('Ctrl Pts',(39.4147172847985,-13.5310870582244,2.19020735614118));
#18774=CARTESIAN_POINT('Ctrl Pts',(40.1289484710636,-13.5358274291177,4.28336653879346));
#18775=CARTESIAN_POINT('Ctrl Pts',(40.6419887213086,-13.5869151317157,5.27197367572221));
#18776=CARTESIAN_POINT('Ctrl Pts',(41.2946051706827,-13.6749984935074,6.16441400296898));
#18777=CARTESIAN_POINT('Origin',(-1.73472347597681E-15,-1.73472347597681E-15,
6.16441400296896));
#18778=CARTESIAN_POINT('Origin',(0.,0.,-6.93889390390723E-15));
#18779=CARTESIAN_POINT('',(37.9654972519551,-21.2337236115523,6.16441400296896));
#18780=CARTESIAN_POINT('',(35.9893695663249,-20.6643479988721,0.));
#18781=CARTESIAN_POINT('Ctrl Pts',(37.965497251955,-21.2337236115523,6.16441400296898));
#18782=CARTESIAN_POINT('Ctrl Pts',(37.3730516785514,-20.9719296263966,5.27522994637944));
#18783=CARTESIAN_POINT('Ctrl Pts',(36.9037434768085,-20.7843367066242,4.29090746118667));
#18784=CARTESIAN_POINT('Ctrl Pts',(36.2327422494516,-20.588151951271,2.19762693960533));
#18785=CARTESIAN_POINT('Ctrl Pts',(36.0373955889743,-20.580705085095,1.101891119292));
#18786=CARTESIAN_POINT('Ctrl Pts',(35.9893695663249,-20.6643479988721,8.32667268468867E-16));
#18787=CARTESIAN_POINT('',(37.9655778209991,-21.23357955498,-6.16441400296898));
#18788=CARTESIAN_POINT('Ctrl Pts',(37.965577820999,-21.23357955498,-6.164414002969));
#18789=CARTESIAN_POINT('Ctrl Pts',(37.3731544963901,-20.9711757310157,-5.27484593906386));
#18790=CARTESIAN_POINT('Ctrl Pts',(36.9029619776889,-20.7849917652452,-4.29007657121741));
#18791=CARTESIAN_POINT('Ctrl Pts',(36.2323804143473,-20.5885989707562,-2.19706469153443));
#18792=CARTESIAN_POINT('Ctrl Pts',(36.038050386442,-20.5795646790169,-1.10157448713195));
#18793=CARTESIAN_POINT('Ctrl Pts',(35.9893695663249,-20.6643479988721,5.55111512312578E-16));
#18794=CARTESIAN_POINT('',(38.9283040838375,-19.4122935573384,-6.16441400296897));
#18795=CARTESIAN_POINT('Origin',(-5.20417042793042E-15,1.73472347597681E-15,
-6.16441400296897));
#18796=CARTESIAN_POINT('',(36.8412779397532,-19.1041942977415,0.));
#18797=CARTESIAN_POINT('Ctrl Pts',(36.8412779397531,-19.1041942977415,4.5102810375397E-16));
#18798=CARTESIAN_POINT('Ctrl Pts',(36.8468754499427,-19.0933998394435,-0.137010845862249));
#18799=CARTESIAN_POINT('Ctrl Pts',(36.8549133193103,-19.083707496519,-0.273849719841702));
#18800=CARTESIAN_POINT('Ctrl Pts',(36.8758752981308,-19.0665008944338,-0.547496131366671));
#18801=CARTESIAN_POINT('Ctrl Pts',(36.8887981733482,-19.0589938273821,-0.684223919457815));
#18802=CARTESIAN_POINT('Ctrl Pts',(36.9348797930813,-19.0397674367968,-1.09397285880578));
#18803=CARTESIAN_POINT('Ctrl Pts',(36.9753262536659,-19.0313667108765,-1.36621764182999));
#18804=CARTESIAN_POINT('Ctrl Pts',(37.1256601264072,-19.0193858351252,-2.17875768610118));
#18805=CARTESIAN_POINT('Ctrl Pts',(37.2642828595705,-19.0291203079137,-2.71300426676973));
#18806=CARTESIAN_POINT('Ctrl Pts',(37.6168941909741,-19.0829641947397,-3.75889728641827));
#18807=CARTESIAN_POINT('Ctrl Pts',(37.8306847292225,-19.1271641381968,-4.2687871825209));
#18808=CARTESIAN_POINT('Ctrl Pts',(38.3290788364555,-19.2468276666622,-5.24984087225791));
#18809=CARTESIAN_POINT('Ctrl Pts',(38.6126398587854,-19.3222508240785,-5.71948809643139));
#18810=CARTESIAN_POINT('Ctrl Pts',(38.9283040838375,-19.4122935573384,-6.16441400296899));
#18811=CARTESIAN_POINT('',(38.928130432958,-19.412641782988,6.16441400296896));
#18812=CARTESIAN_POINT('Ctrl Pts',(36.8412779397531,-19.1041942977415,-8.32667268468867E-16));
#18813=CARTESIAN_POINT('Ctrl Pts',(36.885556183089,-19.0188063957971,1.09886774242324));
#18814=CARTESIAN_POINT('Ctrl Pts',(37.0878578278155,-19.0026592181615,2.19020735614101));
#18815=CARTESIAN_POINT('Ctrl Pts',(37.7941445453238,-19.1089970346771,4.2833665387935));
#18816=CARTESIAN_POINT('Ctrl Pts',(38.2946922474313,-19.2325779783665,5.27197367572228));
#18817=CARTESIAN_POINT('Ctrl Pts',(38.928130432958,-19.412641782988,6.16441400296895));
#18818=CARTESIAN_POINT('Origin',(-1.73472347597681E-15,-1.73472347597681E-15,
6.16441400296896));
#18819=CARTESIAN_POINT('Origin',(0.,0.,-6.93889390390723E-15));
#18820=CARTESIAN_POINT('',(34.557189289939,-26.4206485230648,6.16441400296897));
#18821=CARTESIAN_POINT('',(32.682206333043,-25.575836041162,0.));
#18822=CARTESIAN_POINT('Ctrl Pts',(34.557189289939,-26.4206485230648,6.16441400296899));
#18823=CARTESIAN_POINT('Ctrl Pts',(34.008031126895,-26.0772054272376,5.27522994637943));
#18824=CARTESIAN_POINT('Ctrl Pts',(33.5701970619979,-25.8247324120704,4.29090746118663));
#18825=CARTESIAN_POINT('Ctrl Pts',(32.9339456613615,-25.5350511034992,2.19762693960548));
#18826=CARTESIAN_POINT('Ctrl Pts',(32.7416471477766,-25.4998793072902,1.10189111929232));
#18827=CARTESIAN_POINT('Ctrl Pts',(32.682206333043,-25.575836041162,-2.77555756156289E-16));
#18828=CARTESIAN_POINT('',(34.5572895402933,-26.4205173989522,-6.16441400296897));
#18829=CARTESIAN_POINT('Ctrl Pts',(34.5572895402933,-26.4205173989522,-6.164414002969));
#18830=CARTESIAN_POINT('Ctrl Pts',(34.0082401881097,-26.0764738375632,-5.274845938116));
#18831=CARTESIAN_POINT('Ctrl Pts',(33.5693302919201,-25.8252695836844,-4.29007656912555));
#18832=CARTESIAN_POINT('Ctrl Pts',(32.9335238913098,-25.5354420783965,-2.197064689243));
#18833=CARTESIAN_POINT('Ctrl Pts',(32.7424575769921,-25.4988436963802,-1.1015744860932));
#18834=CARTESIAN_POINT('Ctrl Pts',(32.682206333043,-25.575836041162,1.94289029309402E-15));
#18835=CARTESIAN_POINT('',(35.7694126601179,-24.7547796990844,-6.16441400296897));
#18836=CARTESIAN_POINT('Origin',(-5.20417042793042E-15,1.73472347597681E-15,
-6.16441400296897));
#18837=CARTESIAN_POINT('',(33.7474765292382,-24.1528016575411,0.));
#18838=CARTESIAN_POINT('Ctrl Pts',(33.7474765292382,-24.1528016575411,2.77555756156289E-16));
#18839=CARTESIAN_POINT('Ctrl Pts',(33.754553276426,-24.1429136800298,-0.13701084572592));
#18840=CARTESIAN_POINT('Ctrl Pts',(33.7638886960778,-24.1344638992664,-0.273849719562642));
#18841=CARTESIAN_POINT('Ctrl Pts',(33.7870860669397,-24.1204156362131,-0.547496130807772));
#18842=CARTESIAN_POINT('Ctrl Pts',(33.8009457729332,-24.1148240971771,-0.684223918759634));
#18843=CARTESIAN_POINT('Ctrl Pts',(33.849294548812,-24.1023515017802,-1.09397285769292));
#18844=CARTESIAN_POINT('Ctrl Pts',(33.8905248706275,-24.0997924146194,-1.36621764044298));
#18845=CARTESIAN_POINT('Ctrl Pts',(34.0410336174366,-24.1093282276182,-2.17875768389983));
#18846=CARTESIAN_POINT('Ctrl Pts',(34.1768600108824,-24.1386916892646,-2.71300426404658));
#18847=CARTESIAN_POINT('Ctrl Pts',(34.5182194830272,-24.2421693473793,-3.75889728379987));
#18848=CARTESIAN_POINT('Ctrl Pts',(34.723543634163,-24.3163449650217,-4.2687871804743));
#18849=CARTESIAN_POINT('Ctrl Pts',(35.1998349126628,-24.5057193681818,-5.24984087129297));
#18850=CARTESIAN_POINT('Ctrl Pts',(35.4697758584417,-24.6207297677412,-5.71948809597396));
#18851=CARTESIAN_POINT('Ctrl Pts',(35.7694126601179,-24.7547796990843,-6.164414002969));
#18852=CARTESIAN_POINT('',(35.7691912190763,-24.755099667203,6.16441400296896));
#18853=CARTESIAN_POINT('Ctrl Pts',(33.7474765292382,-24.1528016575411,8.32667268468867E-16));
#18854=CARTESIAN_POINT('Ctrl Pts',(33.8034560493565,-24.0745843323587,1.09886774242322));
#18855=CARTESIAN_POINT('Ctrl Pts',(34.0059965380084,-24.0873920355607,2.19020735614096));
#18856=CARTESIAN_POINT('Ctrl Pts',(34.689960825954,-24.2931625664075,4.28336653879352));
#18857=CARTESIAN_POINT('Ctrl Pts',(35.1678262721695,-24.4867209995526,5.27197367572231));
#18858=CARTESIAN_POINT('Ctrl Pts',(35.7691912190763,-24.755099667203,6.16441400296897));
#18859=CARTESIAN_POINT('Origin',(-1.73472347597681E-15,-1.73472347597681E-15,
6.16441400296896));
#18860=CARTESIAN_POINT('Origin',(0.,0.,-6.93889390390723E-15));
#18861=CARTESIAN_POINT('',(30.4453966086845,-31.0697252215063,6.16441400296896));
#18862=CARTESIAN_POINT('',(28.7097276265208,-29.9666738162745,0.));
#18863=CARTESIAN_POINT('Ctrl Pts',(30.4453966086845,-31.0697252215063,6.16441400296898));
#18864=CARTESIAN_POINT('Ctrl Pts',(29.9507051325582,-30.6516245260304,5.27522994637932));
#18865=CARTESIAN_POINT('Ctrl Pts',(29.5532582434591,-30.3394110379853,4.29090746118637));
#18866=CARTESIAN_POINT('Ctrl Pts',(28.9647089132626,-29.9621302522667,2.19762693960548));
#18867=CARTESIAN_POINT('Ctrl Pts',(28.7793731897637,-29.8999495223686,1.10189111929233));
#18868=CARTESIAN_POINT('Ctrl Pts',(28.7097276265208,-29.9666738162744,-5.55111512312578E-16));
#18869=CARTESIAN_POINT('',(30.44551449954,-31.0696096991627,-6.16441400296898));
#18870=CARTESIAN_POINT('Ctrl Pts',(30.4455144995399,-31.0696096991627,-6.164414002969));
#18871=CARTESIAN_POINT('Ctrl Pts',(29.9510161818958,-30.6509301353986,-5.27484593811587));
#18872=CARTESIAN_POINT('Ctrl Pts',(29.552323848359,-30.3398193877237,-4.29007656912524));
#18873=CARTESIAN_POINT('Ctrl Pts',(28.9642357946952,-29.9624572234643,-2.19706468924339));
#18874=CARTESIAN_POINT('Ctrl Pts',(28.7803227527825,-29.8990397885823,-1.10157448609764));
#18875=CARTESIAN_POINT('Ctrl Pts',(28.7097276265208,-29.9666738162745,-2.77555756156289E-16));
#18876=CARTESIAN_POINT('',(31.882359145105,-29.5933299130488,-6.16441400296898));
#18877=CARTESIAN_POINT('Origin',(-5.20417042793042E-15,1.73472347597681E-15,
-6.16441400296897));
#18878=CARTESIAN_POINT('',(29.9666738162738,-28.7097276265216,0.));
#18879=CARTESIAN_POINT('Ctrl Pts',(29.9666738162737,-28.7097276265215,2.42861286636753E-16));
#18880=CARTESIAN_POINT('Ctrl Pts',(29.9750857383069,-28.7009474204877,-0.137010845870293));
#18881=CARTESIAN_POINT('Ctrl Pts',(29.9855286660416,-28.6939122150426,-0.273849719845077));
#18882=CARTESIAN_POINT('Ctrl Pts',(30.0104891974329,-28.6833082731318,-0.54749613137037));
#18883=CARTESIAN_POINT('Ctrl Pts',(30.0250035905977,-28.6797460897202,-0.68422391946205));
#18884=CARTESIAN_POINT('Ctrl Pts',(30.0746352811228,-28.6742811955971,-1.09397285881242));
#18885=CARTESIAN_POINT('Ctrl Pts',(30.115810133854,-28.6776158428596,-1.36621764183756));
#18886=CARTESIAN_POINT('Ctrl Pts',(30.263429831203,-28.7084742231074,-2.17875768610662));
#18887=CARTESIAN_POINT('Ctrl Pts',(30.3936948517472,-28.7568689184009,-2.71300426677264));
#18888=CARTESIAN_POINT('Ctrl Pts',(30.7168533707401,-28.907873841448,-3.75889728641653));
#18889=CARTESIAN_POINT('Ctrl Pts',(30.9095313269346,-29.0105151315945,-4.26878718251739));
#18890=CARTESIAN_POINT('Ctrl Pts',(31.3540238590801,-29.2657452924991,-5.24984087225377));
#18891=CARTESIAN_POINT('Ctrl Pts',(31.6048495086121,-29.4180016539316,-5.71948809642935));
#18892=CARTESIAN_POINT('Ctrl Pts',(31.8823591451049,-29.5933299130488,-6.16441400296902));
#18893=CARTESIAN_POINT('',(31.8820944218039,-29.5936151100062,6.16441400296897));
#18894=CARTESIAN_POINT('Ctrl Pts',(29.9666738162737,-28.7097276265215,-1.11022302462516E-15));
#18895=CARTESIAN_POINT('Ctrl Pts',(30.0332150315766,-28.6402731572817,1.09886774242332));
#18896=CARTESIAN_POINT('Ctrl Pts',(30.2318712238835,-28.6817750134187,2.19020735614117));
#18897=CARTESIAN_POINT('Ctrl Pts',(30.879589541754,-28.9827893639817,4.28336653879344));
#18898=CARTESIAN_POINT('Ctrl Pts',(31.3250447696425,-29.24238499506,5.27197367572218));
#18899=CARTESIAN_POINT('Ctrl Pts',(31.8820944218039,-29.5936151100061,6.16441400296897));
#18900=CARTESIAN_POINT('Origin',(-1.73472347597681E-15,-1.73472347597681E-15,
6.16441400296896));
#18901=CARTESIAN_POINT('Origin',(0.,0.,-6.93889390390723E-15));
#18902=CARTESIAN_POINT('',(25.7138234497508,-35.0863119121267,6.16441400296896));
#18903=CARTESIAN_POINT('',(24.1528016575403,-33.7474765292388,0.));
#18904=CARTESIAN_POINT('Ctrl Pts',(25.7138234497508,-35.0863119121267,6.16441400296899));
#18905=CARTESIAN_POINT('Ctrl Pts',(25.283669152424,-34.6020649414593,5.27522994637943));
#18906=CARTESIAN_POINT('Ctrl Pts',(24.9347003116427,-34.2364667468035,4.29090746118665));
#18907=CARTESIAN_POINT('Ctrl Pts',(24.4058342190125,-33.7792668327467,2.19762693960535));
#18908=CARTESIAN_POINT('Ctrl Pts',(24.231234186466,-33.6913429895057,1.10189111929205));
#18909=CARTESIAN_POINT('Ctrl Pts',(24.1528016575402,-33.7474765292388,1.94289029309402E-15));
#18910=CARTESIAN_POINT('',(25.7139565811959,-35.0862143432485,-6.16441400296897));
#18911=CARTESIAN_POINT('Ctrl Pts',(25.7139565811959,-35.0862143432484,-6.164414002969));
#18912=CARTESIAN_POINT('Ctrl Pts',(25.2840758578255,-34.6014218856529,-5.27484593811503));
#18913=CARTESIAN_POINT('Ctrl Pts',(24.9337173131074,-34.2367379618448,-4.29007656912494));
#18914=CARTESIAN_POINT('Ctrl Pts',(24.4053193832454,-33.7795231440541,-2.19706468921654));
#18915=CARTESIAN_POINT('Ctrl Pts',(24.2323035529173,-33.6905776524064,-1.10157448595652));
#18916=CARTESIAN_POINT('Ctrl Pts',(24.1528016575402,-33.7474765292388,-1.94289029309402E-15));
#18917=CARTESIAN_POINT('',(27.3462727390257,-33.829445270102,-6.16441400296897));
#18918=CARTESIAN_POINT('Origin',(-5.20417042793042E-15,1.73472347597681E-15,
-6.16441400296897));
#18919=CARTESIAN_POINT('',(25.5758360411612,-32.6822063330437,0.));
#18920=CARTESIAN_POINT('Ctrl Pts',(25.5758360411612,-32.6822063330437,7.63278329429795E-16));
#18921=CARTESIAN_POINT('Ctrl Pts',(25.5854118955597,-32.6747126381702,-0.137010845871668));
#18922=CARTESIAN_POINT('Ctrl Pts',(25.5967497434736,-32.6692352245437,-0.273849719849249));
#18923=CARTESIAN_POINT('Ctrl Pts',(25.6229653109251,-32.6622914694593,-0.547496131378874));
#18924=CARTESIAN_POINT('Ctrl Pts',(25.6378389200524,-32.6608311574542,-0.684223919472369));
#18925=CARTESIAN_POINT('Ctrl Pts',(25.6877431670554,-32.6624852140835,-1.09397285882336));
#18926=CARTESIAN_POINT('Ctrl Pts',(25.7280243493695,-32.6716457119525,-1.36621764184875));
#18927=CARTESIAN_POINT('Ctrl Pts',(25.8697498856548,-32.7231984717385,-2.17875768611436));
#18928=CARTESIAN_POINT('Ctrl Pts',(25.9918017128807,-32.7896392241452,-2.71300426677627));
#18929=CARTESIAN_POINT('Ctrl Pts',(26.2901807029013,-32.9850973871748,-3.75889728641619));
#18930=CARTESIAN_POINT('Ctrl Pts',(26.4662900967122,-33.1141148691595,-4.26878718251706));
#18931=CARTESIAN_POINT('Ctrl Pts',(26.8699352967115,-33.4300050378656,-5.24984087225354));
#18932=CARTESIAN_POINT('Ctrl Pts',(27.0965395633376,-33.6164078608233,-5.7194880964293));
#18933=CARTESIAN_POINT('Ctrl Pts',(27.3462727390257,-33.8294452701019,-6.164414002969));
#18934=CARTESIAN_POINT('',(27.3459701224716,-33.8296898901083,6.16441400296896));
#18935=CARTESIAN_POINT('Ctrl Pts',(25.5758360411612,-32.6822063330437,5.55111512312578E-16));
#18936=CARTESIAN_POINT('Ctrl Pts',(25.651584364394,-32.62292861245,1.09886774242327));
#18937=CARTESIAN_POINT('Ctrl Pts',(25.8423121931576,-32.6922797634123,2.19020735614105));
#18938=CARTESIAN_POINT('Ctrl Pts',(26.4405988638666,-33.0824101495678,4.28336653879351));
#18939=CARTESIAN_POINT('Ctrl Pts',(26.8445756895753,-33.4027583601428,5.2719736757223));
#18940=CARTESIAN_POINT('Ctrl Pts',(27.3459701224716,-33.8296898901082,6.16441400296898));
#18941=CARTESIAN_POINT('Origin',(-1.73472347597681E-15,-1.73472347597681E-15,
6.16441400296896));
#18942=CARTESIAN_POINT('Origin',(0.,0.,-6.93889390390723E-15));
#18943=CARTESIAN_POINT('',(20.4587909979238,-38.3886424727845,6.16441400296896));
#18944=CARTESIAN_POINT('',(19.1041942977406,-36.8412779397537,0.));
#18945=CARTESIAN_POINT('Ctrl Pts',(20.4587909979237,-38.3886424727845,6.16441400296898));
#18946=CARTESIAN_POINT('Ctrl Pts',(20.1019305804272,-37.8481070987954,5.27522994637938));
#18947=CARTESIAN_POINT('Ctrl Pts',(19.8085437872191,-37.4365667224739,4.29090746118653));
#18948=CARTESIAN_POINT('Ctrl Pts',(19.3501271206775,-36.9087549518735,2.19762693960539));
#18949=CARTESIAN_POINT('Ctrl Pts',(19.1898171322411,-36.7968778711866,1.10189111929213));
#18950=CARTESIAN_POINT('Ctrl Pts',(19.1041942977406,-36.8412779397536,2.77555756156289E-16));
#18951=CARTESIAN_POINT('',(20.4589366597946,-38.38856484359,-6.16441400296897));
#18952=CARTESIAN_POINT('Ctrl Pts',(20.4589366597946,-38.38856484359,-6.16441400296901));
#18953=CARTESIAN_POINT('Ctrl Pts',(20.1024246625473,-37.8475284685787,-5.27484593811585));
#18954=CARTESIAN_POINT('Ctrl Pts',(19.8075321962676,-37.4366952816592,-4.29007656912457));
#18955=CARTESIAN_POINT('Ctrl Pts',(19.3495810482794,-36.9089353855215,-2.19706468916629));
#18956=CARTESIAN_POINT('Ctrl Pts',(19.1909845328796,-36.7962725108444,-1.1015744856864));
#18957=CARTESIAN_POINT('Ctrl Pts',(19.1041942977406,-36.8412779397536,-2.22044604925031E-15));
#18958=CARTESIAN_POINT('',(22.2534950801302,-37.3768906775112,-6.16441400296897));
#18959=CARTESIAN_POINT('Origin',(-5.20417042793042E-15,1.73472347597681E-15,
-6.16441400296897));
#18960=CARTESIAN_POINT('',(20.6643479988712,-35.9893695663254,0.));
#18961=CARTESIAN_POINT('Ctrl Pts',(20.6643479988712,-35.9893695663254,1.04083408558608E-15));
#18962=CARTESIAN_POINT('Ctrl Pts',(20.6748928488534,-35.9833149326307,-0.137010845868849));
#18963=CARTESIAN_POINT('Ctrl Pts',(20.6868948110582,-35.9795068151691,-0.273849719849772));
#18964=CARTESIAN_POINT('Ctrl Pts',(20.7138317412147,-35.9763646017415,-0.547496131381827));
#18965=CARTESIAN_POINT('Ctrl Pts',(20.7287617825137,-35.9770358888848,-0.684223919476415));
#18966=CARTESIAN_POINT('Ctrl Pts',(20.7779226794355,-35.9857752244448,-1.09397285882839));
#18967=CARTESIAN_POINT('Ctrl Pts',(20.8164901826204,-36.0005750916014,-1.36621764185478));
#18968=CARTESIAN_POINT('Ctrl Pts',(20.9494364346222,-36.0717727654041,-2.17875768611945));
#18969=CARTESIAN_POINT('Ctrl Pts',(21.0607904452947,-36.1549070328049,-2.71300426677922));
#18970=CARTESIAN_POINT('Ctrl Pts',(21.3283157705668,-36.3908394712685,-3.7588972864172));
#18971=CARTESIAN_POINT('Ctrl Pts',(21.4842715226045,-36.5436067212075,-4.26878718251819));
#18972=CARTESIAN_POINT('Ctrl Pts',(21.8388523382101,-36.913726284825,-5.24984087225241));
#18973=CARTESIAN_POINT('Ctrl Pts',(22.0366222125346,-37.1304809453732,-5.71948809642862));
#18974=CARTESIAN_POINT('Ctrl Pts',(22.2534950801302,-37.3768906775112,-6.164414002969));
#18975=CARTESIAN_POINT('',(22.2531607307116,-37.3770897408175,6.16441400296896));
#18976=CARTESIAN_POINT('Ctrl Pts',(20.6643479988712,-35.9893695663254,-5.55111512312578E-16));
#18977=CARTESIAN_POINT('Ctrl Pts',(20.7477614126131,-35.9414753178263,1.09886774242329));
#18978=CARTESIAN_POINT('Ctrl Pts',(20.9266782092534,-36.0372639741726,2.19020735614109));
#18979=CARTESIAN_POINT('Ctrl Pts',(21.4633538415015,-36.5085684663016,4.2833665387935));
#18980=CARTESIAN_POINT('Ctrl Pts',(21.8176284618318,-36.8831478906138,5.27197367572225));
#18981=CARTESIAN_POINT('Ctrl Pts',(22.2531607307115,-37.3770897408174,6.16441400296898));
#18982=CARTESIAN_POINT('Origin',(-1.73472347597681E-15,-1.73472347597681E-15,
6.16441400296896));
#18983=CARTESIAN_POINT('Origin',(0.,0.,-6.93889390390723E-15));
#18984=CARTESIAN_POINT('',(14.7872765596602,-40.9094909763997,6.16441400296897));
#18985=CARTESIAN_POINT('',(13.6666806339858,-39.1850971728875,0.));
#18986=CARTESIAN_POINT('Ctrl Pts',(14.7872790713139,-40.9094963016524,6.16442208586935));
#18987=CARTESIAN_POINT('Ctrl Pts',(14.5109771826475,-40.3236762657807,5.27523802927974));
#18988=CARTESIAN_POINT('Ctrl Pts',(14.2791424344108,-39.8745661578182,4.2909074611865));
#18989=CARTESIAN_POINT('Ctrl Pts',(13.9005072353241,-39.2868872562402,2.19762693960545));
#18990=CARTESIAN_POINT('Ctrl Pts',(13.7577507400665,-39.1533344328433,1.10189111929226));
#18991=CARTESIAN_POINT('Ctrl Pts',(13.6666806339858,-39.1850971728875,2.77555756156289E-16));
#18992=CARTESIAN_POINT('',(14.787431786677,-40.9094348672085,-6.16441400296898));
#18993=CARTESIAN_POINT('Ctrl Pts',(14.787431786677,-40.9094348672085,-6.164414002969));
#18994=CARTESIAN_POINT('Ctrl Pts',(14.5115460717211,-40.3231685151554,-5.27484593811647));
#18995=CARTESIAN_POINT('Ctrl Pts',(14.2781228441197,-39.8745494440528,-4.29007656912508));
#18996=CARTESIAN_POINT('Ctrl Pts',(13.8999410427704,-39.2869881391093,-2.19706468910962));
#18997=CARTESIAN_POINT('Ctrl Pts',(13.7589924099839,-39.1529013726384,-1.1015744853883));
#18998=CARTESIAN_POINT('Ctrl Pts',(13.6666806339858,-39.1850971728875,-8.32667268468867E-16));
#18999=CARTESIAN_POINT('',(16.7077004351884,-40.1634503767792,-6.16441400296897));
#19000=CARTESIAN_POINT('Origin',(-5.20417042793042E-15,1.73472347597681E-15,
-6.16441400296897));
#19001=CARTESIAN_POINT('',(15.332193422383,-38.5638930200082,0.));
#19002=CARTESIAN_POINT('Ctrl Pts',(15.332193422383,-38.5638930200082,-4.16333634234434E-16));
#19003=CARTESIAN_POINT('Ctrl Pts',(15.3434926052103,-38.5594007023748,-0.137010845862397));
#19004=CARTESIAN_POINT('Ctrl Pts',(15.3559143563653,-38.5573394033684,-0.27384971984452));
#19005=CARTESIAN_POINT('Ctrl Pts',(15.3830242910069,-38.558062698002,-0.547496131373093));
#19006=CARTESIAN_POINT('Ctrl Pts',(15.397706831891,-38.5608519188229,-0.684223919465796));
#19007=CARTESIAN_POINT('Ctrl Pts',(15.4451236046383,-38.5764986256427,-1.09397285881666));
#19008=CARTESIAN_POINT('Ctrl Pts',(15.4811923055495,-38.5966365794692,-1.36621764184235));
#19009=CARTESIAN_POINT('Ctrl Pts',(15.602652870967,-38.6860297879631,-2.17875768611168));
#19010=CARTESIAN_POINT('Ctrl Pts',(15.701042218552,-38.7841651964116,-2.71300426677608));
#19011=CARTESIAN_POINT('Ctrl Pts',(15.9322678349316,-39.0557690062386,-3.75889728641793));
#19012=CARTESIAN_POINT('Ctrl Pts',(16.0648951358144,-39.2291761234743,-4.2687871825184));
#19013=CARTESIAN_POINT('Ctrl Pts',(16.3631933241489,-39.6459905150278,-5.24984087225277));
#19014=CARTESIAN_POINT('Ctrl Pts',(16.5281027818572,-39.8886845133437,-5.71948809642874));
#19015=CARTESIAN_POINT('Ctrl Pts',(16.7077004351884,-40.1634503767792,-6.164414002969));
#19016=CARTESIAN_POINT('',(16.7073411592906,-40.1635998310296,6.16441400296896));
#19017=CARTESIAN_POINT('Ctrl Pts',(15.332193422383,-38.5638930200082,0.));
#19018=CARTESIAN_POINT('Ctrl Pts',(15.4215738700746,-38.5283572323875,1.09886774242323));
#19019=CARTESIAN_POINT('Ctrl Pts',(15.5850374045654,-38.6486334133062,2.19020735614099));
#19020=CARTESIAN_POINT('Ctrl Pts',(16.0491768301248,-39.191517611079,4.28336653879356));
#19021=CARTESIAN_POINT('Ctrl Pts',(16.3465372354506,-39.6127028922473,5.27197367572238));
#19022=CARTESIAN_POINT('Ctrl Pts',(16.7073411592906,-40.1635998310296,6.16441400296899));
#19023=CARTESIAN_POINT('Origin',(-1.73472347597681E-15,-1.73472347597681E-15,
6.16441400296896));
#19024=CARTESIAN_POINT('Origin',(0.,0.,-6.93889390390723E-15));
#19025=CARTESIAN_POINT('',(2.66275246602648,-43.4184263798756,6.16441400296896));
#19026=CARTESIAN_POINT('',(2.07336642434585,-41.4481742863349,0.));
#19027=CARTESIAN_POINT('Ctrl Pts',(2.66275246602646,-43.4184263798755,6.16441400296898));
#19028=CARTESIAN_POINT('Ctrl Pts',(2.5626970742232,-42.7785553024261,5.27531660683072));
#19029=CARTESIAN_POINT('Ctrl Pts',(2.466792220479,-42.2823616483505,4.29109868658257));
#19030=CARTESIAN_POINT('Ctrl Pts',(2.26906302577183,-41.611750365836,2.19783870908466));
#19031=CARTESIAN_POINT('Ctrl Pts',(2.16970548652323,-41.4433551071959,1.10199792653062));
#19032=CARTESIAN_POINT('Ctrl Pts',(2.07336642434584,-41.4481742863349,0.));
#19033=CARTESIAN_POINT('',(2.66291721304303,-43.4184162760053,-6.16441400296897));
#19034=CARTESIAN_POINT('Ctrl Pts',(2.662917213043,-43.4184162760053,-6.164414002969));
#19035=CARTESIAN_POINT('Ctrl Pts',(2.56337712638025,-42.7781718426724,-5.27484593811569));
#19036=CARTESIAN_POINT('Ctrl Pts',(2.46579977756423,-42.2819620733826,-4.29007656912562));
#19037=CARTESIAN_POINT('Ctrl Pts',(2.26847214514444,-41.6116550038394,-2.19706468899303));
#19038=CARTESIAN_POINT('Ctrl Pts',(2.17100952986354,-41.4432898748974,-1.10157448476846));
#19039=CARTESIAN_POINT('Ctrl Pts',(2.07336642434584,-41.4481742863349,-1.94289029309402E-15));
#19040=CARTESIAN_POINT('',(4.71556960657991,-43.2436515951822,-6.16441400296899));
#19041=CARTESIAN_POINT('Origin',(-5.20417042793042E-15,1.73472347597681E-15,
-6.16441400296897));
#19042=CARTESIAN_POINT('',(3.84642767658858,-41.3213624427944,0.));
#19043=CARTESIAN_POINT('Ctrl Pts',(3.8464276765886,-41.3213624427943,1.38777878078145E-15));
#19044=CARTESIAN_POINT('Ctrl Pts',(3.94354036378048,-41.3123226409659,-1.09898083808903));
#19045=CARTESIAN_POINT('Ctrl Pts',(4.06567335249903,-41.4739028133711,-2.19052946960313));
#19046=CARTESIAN_POINT('Ctrl Pts',(4.2836173795468,-41.9623744932969,-3.75889728453861));
#19047=CARTESIAN_POINT('Ctrl Pts',(4.36201791237544,-42.1661228325091,-4.26878718105355));
#19048=CARTESIAN_POINT('Ctrl Pts',(4.53080274396104,-42.6500936240533,-5.24984087156751));
#19049=CARTESIAN_POINT('Ctrl Pts',(4.62065740929872,-42.9294171735218,-5.71948809610405));
#19050=CARTESIAN_POINT('Ctrl Pts',(4.71556960657992,-43.2436515951822,-6.16441400296901));
#19051=CARTESIAN_POINT('',(4.71518277776759,-43.2436937757663,6.16441400296896));
#19052=CARTESIAN_POINT('Ctrl Pts',(3.8464276765886,-41.3213624427943,-1.94289029309402E-15));
#19053=CARTESIAN_POINT('Ctrl Pts',(3.94219917643291,-41.3124474863202,1.09886774242318));
#19054=CARTESIAN_POINT('Ctrl Pts',(4.06515557324172,-41.4739046363273,2.19020735614089));
#19055=CARTESIAN_POINT('Ctrl Pts',(4.3575459377361,-42.1255613966704,4.28336653879355));
#19056=CARTESIAN_POINT('Ctrl Pts',(4.52420114711007,-42.6134666723851,5.27198233656275));
#19057=CARTESIAN_POINT('Ctrl Pts',(4.71518449972428,-43.2436994581107,6.16442204944812));
#19058=CARTESIAN_POINT('Origin',(-1.73472347597681E-15,-1.73472347597681E-15,
6.16441400296896));
#19059=CARTESIAN_POINT('Origin',(0.,0.,-6.93889390390723E-15));
#19060=CARTESIAN_POINT('',(8.81473581362626,-42.5975402169653,6.16441400296897));
#19061=CARTESIAN_POINT('',(7.95095276397613,-40.7312208280712,0.));
#19062=CARTESIAN_POINT('Ctrl Pts',(8.81473754185242,-42.5975458454603,6.16442208586935));
#19063=CARTESIAN_POINT('Ctrl Pts',(8.6246188916806,-41.9783667542709,5.27523802927979));
#19064=CARTESIAN_POINT('Ctrl Pts',(8.45905891928443,-41.5008344149427,4.29090746118661));
#19065=CARTESIAN_POINT('Ctrl Pts',(8.16791310841188,-40.8652518300962,2.19762693960268));
#19066=CARTESIAN_POINT('Ctrl Pts',(8.04561621690065,-40.7127420143402,1.10189111928629));
#19067=CARTESIAN_POINT('Ctrl Pts',(7.95095276397564,-40.7312208280703,2.66453525910038E-14));
#19068=CARTESIAN_POINT('',(8.81489744582342,-42.5975067699932,-6.16441400296899));
#19069=CARTESIAN_POINT('Ctrl Pts',(8.81489744582339,-42.5975067699932,-6.16441400296902));
#19070=CARTESIAN_POINT('Ctrl Pts',(8.62525425083943,-41.9779451335314,-5.27484593863276));
#19071=CARTESIAN_POINT('Ctrl Pts',(8.45805208576314,-41.5006727690235,-4.29007657026494));
#19072=CARTESIAN_POINT('Ctrl Pts',(8.24020736641904,-41.0245381184933,-2.72168992255145));
#19073=CARTESIAN_POINT('Ctrl Pts',(8.17348042064547,-40.9065321202818,-2.18495234743267));
#19074=CARTESIAN_POINT('Ctrl Pts',(8.08284749514825,-40.7929641040503,-1.36923477588193));
#19075=CARTESIAN_POINT('Ctrl Pts',(8.05426390892374,-40.7657215585915,-1.09614446425365));
#19076=CARTESIAN_POINT('Ctrl Pts',(8.01374302361062,-40.740817010984,-0.68531858718774));
#19077=CARTESIAN_POINT('Ctrl Pts',(8.00063920350535,-40.7351764066767,-0.548301186438288));
#19078=CARTESIAN_POINT('Ctrl Pts',(7.97520828346697,-40.7292135752535,-0.274113036175805));
#19079=CARTESIAN_POINT('Ctrl Pts',(7.96288931341435,-40.7288907495992,-0.137034229957148));
#19080=CARTESIAN_POINT('Ctrl Pts',(7.95095276397563,-40.7312208280703,-2.77208811461094E-14));
#19081=CARTESIAN_POINT('',(10.821785190392,-42.1323980482125,-6.16441400296898));
#19082=CARTESIAN_POINT('Origin',(-5.20417042793042E-15,1.73472347597681E-15,
-6.16441400296897));
#19083=CARTESIAN_POINT('',(9.68791960220972,-40.3533668208878,0.));
#19084=CARTESIAN_POINT('Ctrl Pts',(9.68791960220971,-40.3533668208877,6.93889390390723E-17));
#19085=CARTESIAN_POINT('Ctrl Pts',(9.69974309910563,-40.3505282699471,-0.137010845854286));
#19086=CARTESIAN_POINT('Ctrl Pts',(9.71233176818024,-40.3502557514988,-0.273849719837571));
#19087=CARTESIAN_POINT('Ctrl Pts',(9.73906282721921,-40.3548298299992,-0.547496131362149));
#19088=CARTESIAN_POINT('Ctrl Pts',(9.75319897349823,-40.3596802040047,-0.684223919452797));
#19089=CARTESIAN_POINT('Ctrl Pts',(9.79790635332026,-40.3819157602534,-1.09397285880181));
#19090=CARTESIAN_POINT('Ctrl Pts',(9.83074199722253,-40.4069818500826,-1.36621764182707));
#19091=CARTESIAN_POINT('Ctrl Pts',(9.93824428920984,-40.5127508053307,-2.17875768609988));
#19092=CARTESIAN_POINT('Ctrl Pts',(10.0216660503208,-40.6238896009105,-2.71300426676926));
#19093=CARTESIAN_POINT('Ctrl Pts',(10.2118848710489,-40.9256357117772,-3.75889728641769));
#19094=CARTESIAN_POINT('Ctrl Pts',(10.3184838113865,-41.1161526274705,-4.26878718251922));
#19095=CARTESIAN_POINT('Ctrl Pts',(10.554426881542,-41.5711767079482,-5.24984087225529));
#19096=CARTESIAN_POINT('Ctrl Pts',(10.6831188416295,-41.8348694941004,-5.7194880964301));
#19097=CARTESIAN_POINT('Ctrl Pts',(10.821785190392,-42.1323980482124,-6.164414002969));
#19098=CARTESIAN_POINT('',(10.8214083018597,-42.1324948509395,6.16441400296896));
#19099=CARTESIAN_POINT('Ctrl Pts',(9.68791960220971,-40.3533668208877,8.32667268468867E-16));
#19100=CARTESIAN_POINT('Ctrl Pts',(9.7814475556879,-40.3309129003046,1.0988677424233));
#19101=CARTESIAN_POINT('Ctrl Pts',(9.92613018185704,-40.4732281296003,2.19020735614111));
#19102=CARTESIAN_POINT('Ctrl Pts',(10.3082848604908,-41.0766404762988,4.2833665387935));
#19103=CARTESIAN_POINT('Ctrl Pts',(10.5426776504761,-41.5358574965965,5.27197367572226));
#19104=CARTESIAN_POINT('Ctrl Pts',(10.8214083018597,-42.1324948509395,6.16441400296897));
#19105=CARTESIAN_POINT('Origin',(-1.73472347597681E-15,-1.73472347597681E-15,
6.16441400296896));
#19106=CARTESIAN_POINT('Origin',(-1.73472347597681E-15,-1.73472347597681E-15,
11.35));
#19107=CARTESIAN_POINT('',(-42.3548619717231,-1.97942721139887,10.4489096280657));
#19108=CARTESIAN_POINT('',(-42.3779453595728,0.399648641330071,10.4701702229062));
#19109=CARTESIAN_POINT('Ctrl Pts',(-42.3548619717231,-1.97942721139887,
10.4489096280657));
#19110=CARTESIAN_POINT('Ctrl Pts',(-42.277687969919,-1.85081682220853,10.5320034604966));
#19111=CARTESIAN_POINT('Ctrl Pts',(-42.2140016405931,-1.7066924272665,10.6017906159603));
#19112=CARTESIAN_POINT('Ctrl Pts',(-42.113822889283,-1.38567030932352,10.7137049327917));
#19113=CARTESIAN_POINT('Ctrl Pts',(-42.0800217201965,-1.20911028675503,
10.7529995432141));
#19114=CARTESIAN_POINT('Ctrl Pts',(-42.0461300361259,-0.795750669329885,
10.796977768321));
#19115=CARTESIAN_POINT('Ctrl Pts',(-42.0584163598968,-0.559888029352842,
10.7884683253291));
#19116=CARTESIAN_POINT('Ctrl Pts',(-42.1278479976902,-0.194142158176164,
10.7219357482004));
#19117=CARTESIAN_POINT('Ctrl Pts',(-42.1656814408185,-0.0597157582366805,
10.6844661413473));
#19118=CARTESIAN_POINT('Ctrl Pts',(-42.2599040956416,0.186267410922271,
10.5898537840786));
#19119=CARTESIAN_POINT('Ctrl Pts',(-42.3148062568321,0.297900855882757,
10.5342660162233));
#19120=CARTESIAN_POINT('Ctrl Pts',(-42.3779453595727,0.399648641330068,
10.4701702229062));
#19121=CARTESIAN_POINT('',(-43.4414564579485,-2.25607198756206,9.34999999998968));
#19122=CARTESIAN_POINT('Ctrl Pts',(-43.4414564579485,-2.25607198756207,
9.34999999998968));
#19123=CARTESIAN_POINT('Ctrl Pts',(-43.2405264867435,-2.19180199692552,
9.55399283494864));
#19124=CARTESIAN_POINT('Ctrl Pts',(-43.0384692598565,-2.13460442092698,
9.7586494941231));
#19125=CARTESIAN_POINT('Ctrl Pts',(-42.8353155147913,-2.08446078316056,
9.96399986478615));
#19126=CARTESIAN_POINT('Ctrl Pts',(-42.6758357073823,-2.04509701119951,
10.1252040678109));
#19127=CARTESIAN_POINT('Ctrl Pts',(-42.5156798721484,-2.01008129874976,
10.2868360245461));
#19128=CARTESIAN_POINT('Ctrl Pts',(-42.3548619717231,-1.97942721139887,
10.4489096280657));
#19129=CARTESIAN_POINT('',(-43.1481717937249,-5.52134683388194,9.34999999999062));
#19130=CARTESIAN_POINT('Origin',(0.,0.,9.34999999999998));
#19131=CARTESIAN_POINT('',(-42.0034749115207,-5.63542964579464,10.4701702229062));
#19132=CARTESIAN_POINT('Ctrl Pts',(-42.0034749115207,-5.63542964579464,
10.4701702229062));
#19133=CARTESIAN_POINT('Ctrl Pts',(-42.2104648788784,-5.62758774458413,
10.2660612053905));
#19134=CARTESIAN_POINT('Ctrl Pts',(-42.4175418687078,-5.61278982655376,
10.0627475751685));
#19135=CARTESIAN_POINT('Ctrl Pts',(-42.6246751679979,-5.59105439750503,
9.86020040449357));
#19136=CARTESIAN_POINT('Ctrl Pts',(-42.7991408439574,-5.57274692915372,
9.68959756484101));
#19137=CARTESIAN_POINT('Ctrl Pts',(-42.9736466844289,-5.54951680903796,
9.51953800447466));
#19138=CARTESIAN_POINT('Ctrl Pts',(-43.1481717937249,-5.52134683388194,
9.34999999999062));
#19139=CARTESIAN_POINT('',(-41.6420486840548,-7.98700482807827,10.4489096280657));
#19140=CARTESIAN_POINT('Ctrl Pts',(-41.6420486840548,-7.98700482807827,
10.4489096280657));
#19141=CARTESIAN_POINT('Ctrl Pts',(-41.5731662587823,-7.82301570651097,
10.547449245225));
#19142=CARTESIAN_POINT('Ctrl Pts',(-41.526239540548,-7.64031704551109,10.6271602259564));
#19143=CARTESIAN_POINT('Ctrl Pts',(-41.4764846370605,-7.22632801333186,
10.7492445866574));
#19144=CARTESIAN_POINT('Ctrl Pts',(-41.4810105474699,-6.99569328456079,
10.7838550844415));
#19145=CARTESIAN_POINT('Ctrl Pts',(-41.5511566965011,-6.53884015808524,
10.7881210903218));
#19146=CARTESIAN_POINT('Ctrl Pts',(-41.6161107996091,-6.31689994183735,
10.7577447440201));
#19147=CARTESIAN_POINT('Ctrl Pts',(-41.7881771403425,-5.9346381788992,10.6429386483201));
#19148=CARTESIAN_POINT('Ctrl Pts',(-41.8881138550115,-5.77289556463321,
10.5662273743849));
#19149=CARTESIAN_POINT('Ctrl Pts',(-42.0034749115207,-5.63542964579464,
10.4701702229062));
#19150=CARTESIAN_POINT('',(-42.6782125485707,-8.41547227788435,9.34999999999061));
#19151=CARTESIAN_POINT('Ctrl Pts',(-42.6782125485707,-8.41547227788435,
9.34999999999062));
#19152=CARTESIAN_POINT('Ctrl Pts',(-42.4884743280784,-8.32326114672641,
9.55399283494986));
#19153=CARTESIAN_POINT('Ctrl Pts',(-42.2966138161963,-8.23789001801298,
9.75864949412459));
#19154=CARTESIAN_POINT('Ctrl Pts',(-42.1026640670313,-8.15934497780424,
9.96399986478792));
#19155=CARTESIAN_POINT('Ctrl Pts',(-41.9504095829518,-8.09768552928488,
10.125204067812));
#19156=CARTESIAN_POINT('Ctrl Pts',(-41.7968671586498,-8.04023367450976,
10.2868360245467));
#19157=CARTESIAN_POINT('Ctrl Pts',(-41.6420486840548,-7.98700482807828,
10.4489096280657));
#19158=CARTESIAN_POINT('',(-41.9232160376754,-11.6057725748497,9.34999999999155));
#19159=CARTESIAN_POINT('Origin',(0.,0.,9.34999999999998));
#19160=CARTESIAN_POINT('',(-40.7739348422943,-11.5557868365701,10.4701702229111));
#19161=CARTESIAN_POINT('Ctrl Pts',(-40.7739348422943,-11.55578683657,10.4701702229111));
#19162=CARTESIAN_POINT('Ctrl Pts',(-40.9799339692222,-11.5774824983432,
10.2660612053103));
#19163=CARTESIAN_POINT('Ctrl Pts',(-41.1870091772698,-11.592305330102,10.0627475750051));
#19164=CARTESIAN_POINT('Ctrl Pts',(-41.395127432389,-11.600269278368,9.86020040424831));
#19165=CARTESIAN_POINT('Ctrl Pts',(-41.5704227236394,-11.6069772080976,
9.68959756467802));
#19166=CARTESIAN_POINT('Ctrl Pts',(-41.7464583369743,-11.6088183075708,
9.51953800439386));
#19167=CARTESIAN_POINT('Ctrl Pts',(-41.9232160376754,-11.6057725748497,
9.34999999999155));
#19168=CARTESIAN_POINT('',(-40.0815233709313,-13.831990059078,10.4489096280657));
#19169=CARTESIAN_POINT('Ctrl Pts',(-40.0815233709313,-13.831990059078,10.4489096280657));
#19170=CARTESIAN_POINT('Ctrl Pts',(-40.0366801547422,-13.659867119103,10.5474492452249));
#19171=CARTESIAN_POINT('Ctrl Pts',(-40.0162318132297,-13.4723496987262,
10.6271602259563));
#19172=CARTESIAN_POINT('Ctrl Pts',(-40.0259001250805,-13.0554936169285,
10.7492445866574));
#19173=CARTESIAN_POINT('Ctrl Pts',(-40.063202712373,-12.8278505213564,10.7838550844415));
#19174=CARTESIAN_POINT('Ctrl Pts',(-40.1976518535585,-12.3856303388355,
10.7881210903218));
#19175=CARTESIAN_POINT('Ctrl Pts',(-40.2935302035346,-12.1751930866566,
10.7577447440202));
#19176=CARTESIAN_POINT('Ctrl Pts',(-40.51824667799,-11.8213097907414,10.6429386483196));
#19177=CARTESIAN_POINT('Ctrl Pts',(-40.6401845549915,-11.6754359604617,
10.5662273743844));
#19178=CARTESIAN_POINT('Ctrl Pts',(-40.7739348422891,-11.5557868365682,
10.4701702229063));
#19179=CARTESIAN_POINT('',(-41.0461633055059,-14.4035578208467,9.34999999999155));
#19180=CARTESIAN_POINT('Ctrl Pts',(-41.0461633055059,-14.4035578208467,
9.34999999999155));
#19181=CARTESIAN_POINT('Ctrl Pts',(-40.8714793587379,-14.2852827018841,
9.55399283494871));
#19182=CARTESIAN_POINT('Ctrl Pts',(-40.6937212886046,-14.1734759304475,
9.75864949412134));
#19183=CARTESIAN_POINT('Ctrl Pts',(-40.51292379293,-14.0681284383109,9.96399986478255));
#19184=CARTESIAN_POINT('Ctrl Pts',(-40.3709940944081,-13.9854285217927,
10.1252040678084));
#19185=CARTESIAN_POINT('Ctrl Pts',(-40.2271907620149,-13.906710078777,10.2868360245449));
#19186=CARTESIAN_POINT('Ctrl Pts',(-40.0815233709313,-13.831990059078,10.4489096280657));
#19187=CARTESIAN_POINT('',(-39.8448244996705,-17.4539382544775,9.34999999999249));
#19188=CARTESIAN_POINT('Origin',(0.,0.,9.34999999999998));
#19189=CARTESIAN_POINT('',(-38.7143550419872,-17.2409015314864,10.4701702229062));
#19190=CARTESIAN_POINT('Ctrl Pts',(-38.7143550419872,-17.2409015314864,
10.4701702229062));
#19191=CARTESIAN_POINT('Ctrl Pts',(-38.9151697801539,-17.2916930951193,
10.2660612053907));
#19192=CARTESIAN_POINT('Ctrl Pts',(-39.1180277521749,-17.3358349265527,
10.0627475751689));
#19193=CARTESIAN_POINT('Ctrl Pts',(-39.3228942754451,-17.3733361291179,
9.86020040449417));
#19194=CARTESIAN_POINT('Ctrl Pts',(-39.4954506755326,-17.4049229028392,
9.68959756484204));
#19195=CARTESIAN_POINT('Ctrl Pts',(-39.6694324844552,-17.4317977424317,
9.51953800447611));
#19196=CARTESIAN_POINT('Ctrl Pts',(-39.8448244996705,-17.4539382544775,
9.34999999999249));
#19197=CARTESIAN_POINT('',(-37.7050538275441,-19.3953958606403,10.4489096280657));
#19198=CARTESIAN_POINT('Ctrl Pts',(-37.7050538275441,-19.3953958606403,
10.4489096280657));
#19199=CARTESIAN_POINT('Ctrl Pts',(-37.6851626990029,-19.2186430289538,
10.547449245225));
#19200=CARTESIAN_POINT('Ctrl Pts',(-37.6916090034773,-19.0301241631233,
10.6271602259564));
#19201=CARTESIAN_POINT('Ctrl Pts',(-37.7605037117183,-18.6188870194189,
10.7492445866574));
#19202=CARTESIAN_POINT('Ctrl Pts',(-37.8298236027884,-18.3988697140032,
10.7838550844415));
#19203=CARTESIAN_POINT('Ctrl Pts',(-38.025838739333,-17.9802848030953,10.7881210903218));
#19204=CARTESIAN_POINT('Ctrl Pts',(-38.150689529462,-17.7856344105889,10.7577447440201));
#19205=CARTESIAN_POINT('Ctrl Pts',(-38.4234815582465,-17.4673336250894,
10.6429386483201));
#19206=CARTESIAN_POINT('Ctrl Pts',(-38.564938294045,-17.3402981493132,10.5662273743849));
#19207=CARTESIAN_POINT('Ctrl Pts',(-38.7143550419872,-17.2409015314864,
10.4701702229062));
#19208=CARTESIAN_POINT('',(-38.5785325449017,-20.0984284630072,9.34999999999249));
#19209=CARTESIAN_POINT('Ctrl Pts',(-38.5785325449017,-20.0984284630072,
9.34999999999249));
#19210=CARTESIAN_POINT('Ctrl Pts',(-38.4224589332633,-19.956497096582,9.55399283495215));
#19211=CARTESIAN_POINT('Ctrl Pts',(-38.2624219465708,-19.8205307458622,
9.75864949412731));
#19212=CARTESIAN_POINT('Ctrl Pts',(-38.0984572200175,-19.6905253729384,
9.96399986479107));
#19213=CARTESIAN_POINT('Ctrl Pts',(-37.9697415864275,-19.5884685202376,
10.1252040678142));
#19214=CARTESIAN_POINT('Ctrl Pts',(-37.8386047670999,-19.4900859694782,
10.2868360245478));
#19215=CARTESIAN_POINT('Ctrl Pts',(-37.7050538275441,-19.3953958606403,
10.4489096280657));
#19216=CARTESIAN_POINT('',(-36.9553072378377,-22.9467920842455,9.34999999999342));
#19217=CARTESIAN_POINT('Origin',(0.,0.,9.34999999999998));
#19218=CARTESIAN_POINT('',(-35.866662616011,-22.575041189878,10.4701702229062));
#19219=CARTESIAN_POINT('Ctrl Pts',(-35.866662616011,-22.575041189878,10.4701702229062));
#19220=CARTESIAN_POINT('Ctrl Pts',(-36.0582049565313,-22.6538946856141,
10.2660612053895));
#19221=CARTESIAN_POINT('Ctrl Pts',(-36.2527160892939,-22.7264569163318,
10.0627475751663));
#19222=CARTESIAN_POINT('Ctrl Pts',(-36.4501603891734,-22.7927319568543,
9.86020040449035));
#19223=CARTESIAN_POINT('Ctrl Pts',(-36.6164651473186,-22.8485545589344,
9.68959756483981));
#19224=CARTESIAN_POINT('Ctrl Pts',(-36.7848513838357,-22.8999160444089,
9.51953800447548));
#19225=CARTESIAN_POINT('Ctrl Pts',(-36.9553072378377,-22.9467920842455,
9.34999999999343));
#19226=CARTESIAN_POINT('',(-34.5610181206245,-24.5639673341829,10.4489096280657));
#19227=CARTESIAN_POINT('Ctrl Pts',(-34.5610181206245,-24.5639673341829,
10.4489096280657));
#19228=CARTESIAN_POINT('Ctrl Pts',(-34.5664840057471,-24.386182788725,10.547449245225));
#19229=CARTESIAN_POINT('Ctrl Pts',(-34.5996937280388,-24.2005001779056,
10.6271602259564));
#19230=CARTESIAN_POINT('Ctrl Pts',(-34.7264123350862,-23.8032535746304,
10.7492445866574));
#19231=CARTESIAN_POINT('Ctrl Pts',(-34.8263383768538,-23.5953409772319,
10.7838550844415));
#19232=CARTESIAN_POINT('Ctrl Pts',(-35.0799292058383,-23.2089125196238,
10.7881210903218));
#19233=CARTESIAN_POINT('Ctrl Pts',(-35.2312108340732,-23.034011507456,10.7577447440201));
#19234=CARTESIAN_POINT('Ctrl Pts',(-35.5465251581488,-22.7577729184597,
10.6429386483201));
#19235=CARTESIAN_POINT('Ctrl Pts',(-35.7046211015307,-22.6521618731347,
10.5662273743849));
#19236=CARTESIAN_POINT('Ctrl Pts',(-35.866662616011,-22.575041189878,10.4701702229062));
#19237=CARTESIAN_POINT('',(-35.3255541129844,-25.3841530607422,9.34999999999342));
#19238=CARTESIAN_POINT('Ctrl Pts',(-35.3255541129844,-25.3841530607421,
9.34999999999342));
#19239=CARTESIAN_POINT('Ctrl Pts',(-35.1912680451325,-25.2214547601811,
9.55399283495167));
#19240=CARTESIAN_POINT('Ctrl Pts',(-35.0522100334246,-25.0640967129866,
9.7586494941254));
#19241=CARTESIAN_POINT('Ctrl Pts',(-34.9084159249933,-24.912079993766,9.96399986478771));
#19242=CARTESIAN_POINT('Ctrl Pts',(-34.7955346354467,-24.7927437880933,
10.1252040678119));
#19243=CARTESIAN_POINT('Ctrl Pts',(-34.6797338966557,-24.6766999146096,
10.2868360245467));
#19244=CARTESIAN_POINT('Ctrl Pts',(-34.5610181206245,-24.5639673341829,
10.4489096280657));
#19245=CARTESIAN_POINT('',(-33.3134864909484,-27.9725154002619,9.34999999999436));
#19246=CARTESIAN_POINT('Origin',(0.,0.,9.34999999999998));
#19247=CARTESIAN_POINT('',(-32.2888283700867,-27.4496181106866,10.4701702229062));
#19248=CARTESIAN_POINT('Ctrl Pts',(-32.2888283700867,-27.4496181106866,
10.4701702229062));
#19249=CARTESIAN_POINT('Ctrl Pts',(-32.4671990632674,-27.5549283087462,
10.266061205391));
#19250=CARTESIAN_POINT('Ctrl Pts',(-32.6494036710296,-27.6544337809821,
10.0627475751695));
#19251=CARTESIAN_POINT('Ctrl Pts',(-32.8354063509525,-27.7481334907575,
9.86020040449504));
#19252=CARTESIAN_POINT('Ctrl Pts',(-32.9920739818655,-27.8270555339981,
9.68959756484325));
#19253=CARTESIAN_POINT('Ctrl Pts',(-33.1514367877901,-27.9018580936256,
9.51953800447765));
#19254=CARTESIAN_POINT('Ctrl Pts',(-33.3134864909484,-27.9725154002619,
9.34999999999436));
#19255=CARTESIAN_POINT('',(-30.7134197505151,-29.2324872694338,10.4489096280657));
#19256=CARTESIAN_POINT('Ctrl Pts',(-30.7134197505151,-29.2324872694338,
10.4489096280657));
#19257=CARTESIAN_POINT('Ctrl Pts',(-30.7441313796426,-29.0572901908618,
10.547449245225));
#19258=CARTESIAN_POINT('Ctrl Pts',(-30.8034284655748,-28.8782237975454,
10.6271602259564));
#19259=CARTESIAN_POINT('Ctrl Pts',(-30.9853913460153,-28.5030545299773,
10.7492445866574));
#19260=CARTESIAN_POINT('Ctrl Pts',(-31.1138893324329,-28.3114791415085,
10.7838550844415));
#19261=CARTESIAN_POINT('Ctrl Pts',(-31.4198934758748,-27.9650737062297,
10.7881210903218));
#19262=CARTESIAN_POINT('Ctrl Pts',(-31.5945262845248,-27.8134825546352,
10.7577447440201));
#19263=CARTESIAN_POINT('Ctrl Pts',(-31.945944013545,-27.5849295832079,10.6429386483201));
#19264=CARTESIAN_POINT('Ctrl Pts',(-32.1174607870141,-27.5028929046598,
10.5662273743849));
#19265=CARTESIAN_POINT('Ctrl Pts',(-32.2888283700867,-27.4496181106866,
10.4701702229062));
#19266=CARTESIAN_POINT('',(-31.3534492698128,-30.1531295040128,9.34999999999437));
#19267=CARTESIAN_POINT('Ctrl Pts',(-31.3534492698128,-30.1531295040128,
9.34999999999436));
#19268=CARTESIAN_POINT('Ctrl Pts',(-31.2436844228208,-29.9729763375018,
9.55399283498594));
#19269=CARTESIAN_POINT('Ctrl Pts',(-31.1284362061847,-29.7974299498614,
9.7586494941933));
#19270=CARTESIAN_POINT('Ctrl Pts',(-31.0077399492325,-29.6264965063399,
9.96399986488942));
#19271=CARTESIAN_POINT('Ctrl Pts',(-30.912990941281,-29.4923102887359,10.1252040678799));
#19272=CARTESIAN_POINT('Ctrl Pts',(-30.8148836521473,-29.360967411178,10.2868360245808));
#19273=CARTESIAN_POINT('Ctrl Pts',(-30.7134197505151,-29.2324872694338,
10.4489096280657));
#19274=CARTESIAN_POINT('',(-28.9934992272654,-32.428798968802,9.34999999999529));
#19275=CARTESIAN_POINT('Origin',(0.,0.,9.34999999999998));
#19276=CARTESIAN_POINT('',(-28.0536866918425,-31.7653999649279,10.4701702229111));
#19277=CARTESIAN_POINT('Ctrl Pts',(-28.0536866918425,-31.7653999649279,
10.4701702229111));
#19278=CARTESIAN_POINT('Ctrl Pts',(-28.2152546248138,-31.8950230534185,
10.2660612053112));
#19279=CARTESIAN_POINT('Ctrl Pts',(-28.3814435472657,-32.0194461227552,
10.0627475750071));
#19280=CARTESIAN_POINT('Ctrl Pts',(-28.5522181291298,-32.1386630459438,
9.86020040425125));
#19281=CARTESIAN_POINT('Ctrl Pts',(-28.6960593315701,-32.2390779050844,
9.68959756468124));
#19282=CARTESIAN_POINT('Ctrl Pts',(-28.8431545396677,-32.3357987744151,
9.51953800439734));
#19283=CARTESIAN_POINT('Ctrl Pts',(-28.9934992272654,-32.4287989688019,
9.34999999999529));
#19284=CARTESIAN_POINT('',(-26.2405847244738,-33.3059180634111,10.4489096280657));
#19285=CARTESIAN_POINT('Ctrl Pts',(-26.2405847244738,-33.3059180634111,
10.4489096280657));
#19286=CARTESIAN_POINT('Ctrl Pts',(-26.2959168974022,-33.136874959018,10.5474492452249));
#19287=CARTESIAN_POINT('Ctrl Pts',(-26.3800942293039,-32.9680700585877,
10.6271602259563));
#19288=CARTESIAN_POINT('Ctrl Pts',(-26.6135971436294,-32.6226154911157,
10.7492445866574));
#19289=CARTESIAN_POINT('Ctrl Pts',(-26.7680512262512,-32.4512772340281,
10.7838550844415));
#19290=CARTESIAN_POINT('Ctrl Pts',(-27.120239322233,-32.1519466367898,10.7881210903218));
#19291=CARTESIAN_POINT('Ctrl Pts',(-27.3146682909135,-32.0267513044625,
10.7577447440202));
#19292=CARTESIAN_POINT('Ctrl Pts',(-27.6950355733221,-31.8505366300091,
10.6429386483196));
#19293=CARTESIAN_POINT('Ctrl Pts',(-27.8764815899833,-31.7937443484396,
10.5662273743844));
#19294=CARTESIAN_POINT('Ctrl Pts',(-28.0536866918392,-31.7653999649236,
10.4701702229063));
#19295=CARTESIAN_POINT('',(-26.7430786153894,-34.3082751850266,9.34999999999529));
#19296=CARTESIAN_POINT('Ctrl Pts',(-26.7430786153894,-34.3082751850266,
9.3499999999953));
#19297=CARTESIAN_POINT('Ctrl Pts',(-26.6600694850412,-34.1143345515736,
9.55399283495525));
#19298=CARTESIAN_POINT('Ctrl Pts',(-26.5709771848575,-33.9241734417595,
9.7586494941307));
#19299=CARTESIAN_POINT('Ctrl Pts',(-26.4758358071583,-33.7378029859668,
9.96399986479476));
#19300=CARTESIAN_POINT('Ctrl Pts',(-26.4011478973347,-33.5914984008048,
10.1252040678166));
#19301=CARTESIAN_POINT('Ctrl Pts',(-26.3227312393088,-33.4475302813445,
10.286836024549));
#19302=CARTESIAN_POINT('Ctrl Pts',(-26.2405847244738,-33.3059180634111,
10.4489096280657));
#19303=CARTESIAN_POINT('',(-24.0832879296629,-36.2249257072707,9.34999999999623));
#19304=CARTESIAN_POINT('Origin',(0.,0.,9.34999999999998));
#19305=CARTESIAN_POINT('',(-23.2474528526981,-35.4345298797237,10.4701702229062));
#19306=CARTESIAN_POINT('Ctrl Pts',(-23.2474528526981,-35.4345298797237,
10.4701702229062));
#19307=CARTESIAN_POINT('Ctrl Pts',(-23.3889289681449,-35.5858271062694,
10.2660612053881));
#19308=CARTESIAN_POINT('Ctrl Pts',(-23.5357190779423,-35.732634877731,10.0627475751637));
#19309=CARTESIAN_POINT('Ctrl Pts',(-23.6877890835939,-35.8749421014862,
9.86020040448638));
#19310=CARTESIAN_POINT('Ctrl Pts',(-23.8158756656119,-35.9948056196677,
9.68959756483812));
#19311=CARTESIAN_POINT('Ctrl Pts',(-23.9477088417672,-36.1114758408148,
9.51953800447604));
#19312=CARTESIAN_POINT('Ctrl Pts',(-24.0832879296629,-36.2249257072707,
9.34999999999623));
#19313=CARTESIAN_POINT('',(-21.2335670650398,-36.7013364119537,10.4489096280657));
#19314=CARTESIAN_POINT('Ctrl Pts',(-21.2335670650398,-36.7013364119537,
10.4489096280657));
#19315=CARTESIAN_POINT('Ctrl Pts',(-21.3123933782931,-36.5418885118649,
10.547449245225));
#19316=CARTESIAN_POINT('Ctrl Pts',(-21.4197373484343,-36.3867814853002,
10.6271602259564));
#19317=CARTESIAN_POINT('Ctrl Pts',(-21.7000268506759,-36.0780740767093,
10.7492445866574));
#19318=CARTESIAN_POINT('Ctrl Pts',(-21.8772927897884,-35.9304609038185,
10.7838550844415));
#19319=CARTESIAN_POINT('Ctrl Pts',(-22.2684953043027,-35.6842986523824,
10.7881210903218));
#19320=CARTESIAN_POINT('Ctrl Pts',(-22.4787624198982,-35.5880477552548,
10.7577447440201));
#19321=CARTESIAN_POINT('Ctrl Pts',(-22.8803360747106,-35.4677586003878,
10.6429386483201));
#19322=CARTESIAN_POINT('Ctrl Pts',(-23.0680176169133,-35.4373668428729,
10.5662273743849));
#19323=CARTESIAN_POINT('Ctrl Pts',(-23.2474528526981,-35.4345298797237,
10.4701702229062));
#19324=CARTESIAN_POINT('',(-21.5882960010271,-37.7650033201689,9.34999999999623));
#19325=CARTESIAN_POINT('Ctrl Pts',(-21.5882960010271,-37.7650033201689,
9.34999999999623));
#19326=CARTESIAN_POINT('Ctrl Pts',(-21.5337324138217,-37.5612232917665,
9.55399283495411));
#19327=CARTESIAN_POINT('Ctrl Pts',(-21.4726096923831,-37.3603185915706,
9.75864949412748));
#19328=CARTESIAN_POINT('Ctrl Pts',(-21.4049599980022,-37.1623050885155,
9.96399986478943));
#19329=CARTESIAN_POINT('Ctrl Pts',(-21.351853616785,-37.0068604752673,10.125204067813));
#19330=CARTESIAN_POINT('Ctrl Pts',(-21.2947239269072,-36.8531978896717,
10.2868360245472));
#19331=CARTESIAN_POINT('Ctrl Pts',(-21.2335670650398,-36.7013364119537,
10.4489096280657));
#19332=CARTESIAN_POINT('',(-18.6828103402799,-39.2836174223986,9.34999999999716));
#19333=CARTESIAN_POINT('Origin',(0.,0.,9.34999999999998));
#19334=CARTESIAN_POINT('',(-17.9679679135938,-38.3823149509186,10.4701702229062));
#19335=CARTESIAN_POINT('Ctrl Pts',(-17.9679679135938,-38.3823149509186,
10.4701702229062));
#19336=CARTESIAN_POINT('Ctrl Pts',(-18.0864721658495,-38.5522063403393,
10.2660612053891));
#19337=CARTESIAN_POINT('Ctrl Pts',(-18.2108752397297,-38.7184102311019,
10.0627475751655));
#19338=CARTESIAN_POINT('Ctrl Pts',(-18.341144962456,-38.8809107907692,9.86020040448914));
#19339=CARTESIAN_POINT('Ctrl Pts',(-18.4508694505502,-39.0177828923699,
9.68959756484026));
#19340=CARTESIAN_POINT('Ctrl Pts',(-18.5647568514065,-39.1520273960344,
9.51953800447757));
#19341=CARTESIAN_POINT('Ctrl Pts',(-18.6828103402799,-39.2836174223986,
9.34999999999716));
#19342=CARTESIAN_POINT('',(-15.7942952127126,-39.3496213890633,10.4489096280657));
#19343=CARTESIAN_POINT('Ctrl Pts',(-15.7942952127126,-39.3496213890633,
10.4489096280657));
#19344=CARTESIAN_POINT('Ctrl Pts',(-15.8950109898693,-39.2030145927148,
10.547449245225));
#19345=CARTESIAN_POINT('Ctrl Pts',(-16.0233363845722,-39.064762971785,10.6271602259564));
#19346=CARTESIAN_POINT('Ctrl Pts',(-16.3447065887524,-38.7990871146754,
10.7492445866574));
#19347=CARTESIAN_POINT('Ctrl Pts',(-16.5411757610281,-38.6782040045002,
10.7838550844415));
#19348=CARTESIAN_POINT('Ctrl Pts',(-16.9634289390143,-38.4902212524323,
10.7881210903218));
#19349=CARTESIAN_POINT('Ctrl Pts',(-17.1852537694115,-38.4248741812053,
10.7577447440201));
#19350=CARTESIAN_POINT('Ctrl Pts',(-17.5998589150602,-38.3629592862316,
10.6429386483201));
#19351=CARTESIAN_POINT('Ctrl Pts',(-17.7899553278333,-38.3595867413123,
10.5662273743849));
#19352=CARTESIAN_POINT('Ctrl Pts',(-17.9679679135938,-38.3823149509187,
10.4701702229062));
#19353=CARTESIAN_POINT('',(-15.994037935589,-40.4529448929888,9.34999999999716));
#19354=CARTESIAN_POINT('Ctrl Pts',(-15.994037935589,-40.4529448929888,9.34999999999716));
#19355=CARTESIAN_POINT('Ctrl Pts',(-15.9690306488124,-40.2434738433598,
9.55399283495553));
#19356=CARTESIAN_POINT('Ctrl Pts',(-15.937121788463,-40.0359153931143,9.75864949412937));
#19357=CARTESIAN_POINT('Ctrl Pts',(-15.8983409300912,-39.8302898266929,
9.9639998647918));
#19358=CARTESIAN_POINT('Ctrl Pts',(-15.8678971702567,-39.6688695894216,
10.1252040678146));
#19359=CARTESIAN_POINT('Ctrl Pts',(-15.8332174442655,-39.5086406648094,
10.286836024548));
#19360=CARTESIAN_POINT('Ctrl Pts',(-15.7942952127126,-39.3496213890633,
10.4489096280657));
#19361=CARTESIAN_POINT('',(-12.902004609145,-41.5426079714041,9.3499999999981));
#19362=CARTESIAN_POINT('Origin',(0.,0.,9.34999999999998));
#19363=CARTESIAN_POINT('',(-12.3227069631095,-40.5487467751691,10.4701702229062));
#19364=CARTESIAN_POINT('Ctrl Pts',(-12.3227069631095,-40.5487467751691,
10.4701702229062));
#19365=CARTESIAN_POINT('Ctrl Pts',(-12.4158269473359,-40.7337738287013,
10.266061205391));
#19366=CARTESIAN_POINT('Ctrl Pts',(-12.5153104974631,-40.9159904068405,
10.0627475751694));
#19367=CARTESIAN_POINT('Ctrl Pts',(-12.6211280213761,-41.0953762596368,
9.86020040449486));
#19368=CARTESIAN_POINT('Ctrl Pts',(-12.7102567413884,-41.2464706233757,
9.68959756484438));
#19369=CARTESIAN_POINT('Ctrl Pts',(-12.8038799478888,-41.3955565785931,
9.5195380044801));
#19370=CARTESIAN_POINT('Ctrl Pts',(-12.902004609145,-41.5426079714041,9.3499999999981));
#19371=CARTESIAN_POINT('',(-10.0334970568407,-41.1968615496291,10.4489096280657));
#19372=CARTESIAN_POINT('Ctrl Pts',(-10.0334970568407,-41.1968615496291,
10.4489096280657));
#19373=CARTESIAN_POINT('Ctrl Pts',(-10.1540520151182,-41.0660803486156,
10.547449245225));
#19374=CARTESIAN_POINT('Ctrl Pts',(-10.3007464994067,-40.9474985376379,
10.6271602259564));
#19375=CARTESIAN_POINT('Ctrl Pts',(-10.6566552349236,-40.7302626263145,
10.7492445866574));
#19376=CARTESIAN_POINT('Ctrl Pts',(-10.8683280945852,-40.6385704103799,
10.7838550844415));
#19377=CARTESIAN_POINT('Ctrl Pts',(-11.313036079017,-40.5125939444148,10.7881210903218));
#19378=CARTESIAN_POINT('Ctrl Pts',(-11.5419029103591,-40.4794809770132,
10.7577447440201));
#19379=CARTESIAN_POINT('Ctrl Pts',(-11.9610993817012,-40.4772007506467,
10.6429386483201));
#19380=CARTESIAN_POINT('Ctrl Pts',(-12.1497408502734,-40.5009160736121,
10.5662273743849));
#19381=CARTESIAN_POINT('Ctrl Pts',(-12.3227069631095,-40.5487467751691,
10.4701702229062));
#19382=CARTESIAN_POINT('',(-10.0741873807793,-42.3173811644473,9.3499999999981));
#19383=CARTESIAN_POINT('Ctrl Pts',(-10.0741873807793,-42.3173811644473,
9.3499999999981));
#19384=CARTESIAN_POINT('Ctrl Pts',(-10.0792454706754,-42.1064833200987,
9.55399283495567));
#19385=CARTESIAN_POINT('Ctrl Pts',(-10.0772000437945,-41.8964964113029,
9.75864949412871));
#19386=CARTESIAN_POINT('Ctrl Pts',(-10.0680774878737,-41.6874447250736,
9.96399986479033));
#19387=CARTESIAN_POINT('Ctrl Pts',(-10.0609160965793,-41.5233349143112,
10.1252040678136));
#19388=CARTESIAN_POINT('Ctrl Pts',(-10.0493923136875,-41.3598014495242,
10.2868360245475));
#19389=CARTESIAN_POINT('Ctrl Pts',(-10.0334970568407,-41.1968615496291,
10.4489096280657));
#19390=CARTESIAN_POINT('',(-6.8585512704771,-42.9559108211003,9.34999999999904));
#19391=CARTESIAN_POINT('Origin',(0.,0.,9.34999999999998));
#19392=CARTESIAN_POINT('',(-6.42659123460866,-41.8897230480067,10.4701702229062));
#19393=CARTESIAN_POINT('Ctrl Pts',(-6.42659123460866,-41.8897230480067,
10.4701702229062));
#19394=CARTESIAN_POINT('Ctrl Pts',(-6.49243129646439,-42.0861191484173,
10.2660612053897));
#19395=CARTESIAN_POINT('Ctrl Pts',(-6.56497012464666,-42.2806390098741,
10.0627475751668));
#19396=CARTESIAN_POINT('Ctrl Pts',(-6.64418131011379,-42.4732583771454,
9.86020040449103));
#19397=CARTESIAN_POINT('Ctrl Pts',(-6.7108998583293,-42.635499157494,9.68959756484215));
#19398=CARTESIAN_POINT('Ctrl Pts',(-6.7823529719748,-42.7963916041418,9.51953800447945));
#19399=CARTESIAN_POINT('Ctrl Pts',(-6.85855127047709,-42.9559108211003,
9.34999999999904));
#19400=CARTESIAN_POINT('',(-4.06844583510776,-42.2054524109828,10.4489096280657));
#19401=CARTESIAN_POINT('Ctrl Pts',(-4.06844583510776,-42.2054524109828,
10.4489096280657));
#19402=CARTESIAN_POINT('Ctrl Pts',(-4.20638582320732,-42.093159133415,10.547449245225));
#19403=CARTESIAN_POINT('Ctrl Pts',(-4.36846312041316,-41.9966611160993,
10.6271602259564));
#19404=CARTESIAN_POINT('Ctrl Pts',(-4.75166511176766,-41.8322874472601,
10.7492445866574));
#19405=CARTESIAN_POINT('Ctrl Pts',(-4.97423260980666,-41.7716527146639,
10.7838550844415));
#19406=CARTESIAN_POINT('Ctrl Pts',(-5.4323424285529,-41.7102470523626,10.7881210903217));
#19407=CARTESIAN_POINT('Ctrl Pts',(-5.66359219215121,-41.7100422733127,
10.7577447440201));
#19408=CARTESIAN_POINT('Ctrl Pts',(-6.078846357893,-41.7674431343866,10.6429386483201));
#19409=CARTESIAN_POINT('Ctrl Pts',(-6.26219268596132,-41.8177635496503,
10.5662273743849));
#19410=CARTESIAN_POINT('Ctrl Pts',(-6.42659123460866,-41.8897230480067,
10.4701702229062));
#19411=CARTESIAN_POINT('',(-3.9492554224545,-43.3203575886476,9.34999999999904));
#19412=CARTESIAN_POINT('Ctrl Pts',(-3.9492554224545,-43.3203575886476,9.34999999999904));
#19413=CARTESIAN_POINT('Ctrl Pts',(-3.98427592089977,-43.1123262215076,
9.5539928349595));
#19414=CARTESIAN_POINT('Ctrl Pts',(-4.01213556648031,-42.9041855820685,
9.75864949413545));
#19415=CARTESIAN_POINT('Ctrl Pts',(-4.03285702194169,-42.6959634655039,
9.96399986480001));
#19416=CARTESIAN_POINT('Ctrl Pts',(-4.04912378446205,-42.5325048837476,
10.1252040678201));
#19417=CARTESIAN_POINT('Ctrl Pts',(-4.06099053565725,-42.3689959485411,
10.2868360245508));
#19418=CARTESIAN_POINT('Ctrl Pts',(-4.06844583510776,-42.2054524109828,
10.4489096280657));
#19419=CARTESIAN_POINT('',(-0.675477606371088,-43.4947552010963,9.34999999999998));
#19420=CARTESIAN_POINT('Origin',(0.,0.,9.34999999999998));
#19421=CARTESIAN_POINT('',(-0.399648641329914,-42.3779453595728,10.4701702229062));
#19422=CARTESIAN_POINT('Ctrl Pts',(-0.399648641329913,-42.3779453595728,
10.4701702229062));
#19423=CARTESIAN_POINT('Ctrl Pts',(-0.436868467022045,-42.581712448616,
10.2660612053897));
#19424=CARTESIAN_POINT('Ctrl Pts',(-0.48098589190162,-42.7845757299589,
10.0627475751667));
#19425=CARTESIAN_POINT('Ctrl Pts',(-0.53197822761229,-42.9865074368548,
9.86020040449092));
#19426=CARTESIAN_POINT('Ctrl Pts',(-0.57492840679043,-43.1565918793901,
9.68959756484239));
#19427=CARTESIAN_POINT('Ctrl Pts',(-0.622756848241735,-43.326015511231,
9.51953800448004));
#19428=CARTESIAN_POINT('Ctrl Pts',(-0.675477606371083,-43.4947552010963,
9.34999999999997));
#19429=CARTESIAN_POINT('',(1.97942721139903,-42.3548619717231,10.4489096280657));
#19430=CARTESIAN_POINT('Ctrl Pts',(1.97942721139902,-42.3548619717231,10.4489096280657));
#19431=CARTESIAN_POINT('Ctrl Pts',(1.82691025384907,-42.2633425849052,10.5474492452249));
#19432=CARTESIAN_POINT('Ctrl Pts',(1.65274957010464,-42.1908927826067,10.6271602259564));
#19433=CARTESIAN_POINT('Ctrl Pts',(1.25005521039315,-42.0827275301346,10.7492445866574));
#19434=CARTESIAN_POINT('Ctrl Pts',(1.02112390640523,-42.0543846291766,10.7838550844415));
#19435=CARTESIAN_POINT('Ctrl Pts',(0.558938048174549,-42.0587998127441,
10.7881210903218));
#19436=CARTESIAN_POINT('Ctrl Pts',(0.330012930637701,-42.0915073907569,
10.7577447440201));
#19437=CARTESIAN_POINT('Ctrl Pts',(-0.0728455521833925,-42.2074208232701,
10.6429386483201));
#19438=CARTESIAN_POINT('Ctrl Pts',(-0.247164337235464,-42.2833219522895,
10.5662273743849));
#19439=CARTESIAN_POINT('Ctrl Pts',(-0.399648641329906,-42.3779453595728,
10.4701702229062));
#19440=CARTESIAN_POINT('',(2.25607198755898,-43.4414564579384,9.34999999999998));
#19441=CARTESIAN_POINT('Ctrl Pts',(2.25607198755898,-43.4414564579384,9.34999999999998));
#19442=CARTESIAN_POINT('Ctrl Pts',(2.19180199691216,-43.2405264867004,9.55399283499235));
#19443=CARTESIAN_POINT('Ctrl Pts',(2.13460442090562,-43.0384692597801,9.75864949420051));
#19444=CARTESIAN_POINT('Ctrl Pts',(2.08446078313353,-42.8353155146812,9.96399986489744));
#19445=CARTESIAN_POINT('Ctrl Pts',(2.04509701118354,-42.6758357073085,10.1252040678853));
#19446=CARTESIAN_POINT('Ctrl Pts',(2.01008129874285,-42.5156798721113,10.2868360245835));
#19447=CARTESIAN_POINT('Ctrl Pts',(1.97942721139903,-42.3548619717231,10.4489096280657));
#19448=CARTESIAN_POINT('',(5.52134683388117,-43.148171793727,9.34999999998873));
#19449=CARTESIAN_POINT('Origin',(0.,0.,9.34999999999998));
#19450=CARTESIAN_POINT('',(5.63542964579419,-42.0034749115208,10.4701702229062));
#19451=CARTESIAN_POINT('Ctrl Pts',(5.6354296457942,-42.0034749115208,10.4701702229062));
#19452=CARTESIAN_POINT('Ctrl Pts',(5.62758774458367,-42.2104648788786,10.2660612053904));
#19453=CARTESIAN_POINT('Ctrl Pts',(5.61278982655329,-42.4175418687082,10.0627475751682));
#19454=CARTESIAN_POINT('Ctrl Pts',(5.59105439750453,-42.6246751679985,9.86020040449308));
#19455=CARTESIAN_POINT('Ctrl Pts',(5.57274692915316,-42.7991408439585,9.68959756484005));
#19456=CARTESIAN_POINT('Ctrl Pts',(5.54951680903731,-42.9736466844305,9.51953800447324));
#19457=CARTESIAN_POINT('Ctrl Pts',(5.52134683388117,-43.148171793727,9.34999999998873));
#19458=CARTESIAN_POINT('',(7.98700482807783,-41.6420486840549,10.4489096280657));
#19459=CARTESIAN_POINT('Ctrl Pts',(7.98700482807783,-41.6420486840549,10.4489096280657));
#19460=CARTESIAN_POINT('Ctrl Pts',(7.82301570651054,-41.5731662587824,10.547449245225));
#19461=CARTESIAN_POINT('Ctrl Pts',(7.64031704551066,-41.5262395405481,10.6271602259564));
#19462=CARTESIAN_POINT('Ctrl Pts',(7.22632801333144,-41.4764846370606,10.7492445866574));
#19463=CARTESIAN_POINT('Ctrl Pts',(6.99569328456037,-41.4810105474699,10.7838550844415));
#19464=CARTESIAN_POINT('Ctrl Pts',(6.53884015808481,-41.5511566965012,10.7881210903218));
#19465=CARTESIAN_POINT('Ctrl Pts',(6.31689994183693,-41.6161107996092,10.7577447440201));
#19466=CARTESIAN_POINT('Ctrl Pts',(5.93463817889873,-41.7881771403425,10.6429386483201));
#19467=CARTESIAN_POINT('Ctrl Pts',(5.77289556463275,-41.8881138550116,10.5662273743849));
#19468=CARTESIAN_POINT('Ctrl Pts',(5.63542964579419,-42.0034749115208,10.4701702229062));
#19469=CARTESIAN_POINT('',(8.41547227788475,-42.6782125485726,9.34999999998873));
#19470=CARTESIAN_POINT('Ctrl Pts',(8.41547227788475,-42.6782125485725,9.34999999998873));
#19471=CARTESIAN_POINT('Ctrl Pts',(8.32326114671144,-42.4884743280488,9.55399283498187));
#19472=CARTESIAN_POINT('Ctrl Pts',(8.23789001798488,-42.2966138161343,9.75864949419081));
#19473=CARTESIAN_POINT('Ctrl Pts',(8.15934497776531,-42.1026640669364,9.96399986488852));
#19474=CARTESIAN_POINT('Ctrl Pts',(8.09768552926051,-41.950409582888,10.1252040678793));
#19475=CARTESIAN_POINT('Ctrl Pts',(8.04023367449823,-41.7968671586176,10.2868360245805));
#19476=CARTESIAN_POINT('Ctrl Pts',(7.98700482807784,-41.642048684055,10.4489096280657));
#19477=CARTESIAN_POINT('',(11.6057725748491,-41.9232160376785,9.34999999998873));
#19478=CARTESIAN_POINT('Origin',(0.,0.,9.34999999999998));
#19479=CARTESIAN_POINT('',(11.5557868365676,-40.7739348422894,10.4701702229062));
#19480=CARTESIAN_POINT('Ctrl Pts',(11.5557868365676,-40.7739348422894,10.4701702229062));
#19481=CARTESIAN_POINT('Ctrl Pts',(11.577482498333,-40.9799339691365,10.2660612053909));
#19482=CARTESIAN_POINT('Ctrl Pts',(11.592305330089,-41.1870091771008,10.0627475751691));
#19483=CARTESIAN_POINT('Ctrl Pts',(11.6002692783576,-41.3951274321352,9.8602004044945));
#19484=CARTESIAN_POINT('Ctrl Pts',(11.6069772080954,-41.5704227234707,9.689597564841));
#19485=CARTESIAN_POINT('Ctrl Pts',(11.6088183075718,-41.7464583368912,9.51953800447371));
#19486=CARTESIAN_POINT('Ctrl Pts',(11.6057725748491,-41.9232160376785,9.34999999998873));
#19487=CARTESIAN_POINT('',(13.8319900590775,-40.0815233709314,10.4489096280657));
#19488=CARTESIAN_POINT('Ctrl Pts',(13.8319900590775,-40.0815233709314,10.4489096280657));
#19489=CARTESIAN_POINT('Ctrl Pts',(13.6598671191025,-40.0366801547423,10.547449245225));
#19490=CARTESIAN_POINT('Ctrl Pts',(13.4723496987256,-40.0162318132298,10.6271602259564));
#19491=CARTESIAN_POINT('Ctrl Pts',(13.0554936169279,-40.0259001250807,10.7492445866574));
#19492=CARTESIAN_POINT('Ctrl Pts',(12.8278505213559,-40.0632027123732,10.7838550844415));
#19493=CARTESIAN_POINT('Ctrl Pts',(12.385630338835,-40.1976518535586,10.7881210903218));
#19494=CARTESIAN_POINT('Ctrl Pts',(12.1751930866561,-40.2935302035348,10.7577447440201));
#19495=CARTESIAN_POINT('Ctrl Pts',(11.8213097907425,-40.5182466779892,10.6429386483201));
#19496=CARTESIAN_POINT('Ctrl Pts',(11.6754359604618,-40.640184554991,10.5662273743849));
#19497=CARTESIAN_POINT('Ctrl Pts',(11.5557868365676,-40.7739348422894,10.4701702229062));
#19498=CARTESIAN_POINT('',(14.4035578208479,-41.0461633055085,9.34999999998873));
#19499=CARTESIAN_POINT('Ctrl Pts',(14.4035578208479,-41.0461633055085,9.34999999998873));
#19500=CARTESIAN_POINT('Ctrl Pts',(14.2852827018644,-40.8714793587097,9.55399283498179));
#19501=CARTESIAN_POINT('Ctrl Pts',(14.1734759304092,-40.6937212885446,9.75864949419063));
#19502=CARTESIAN_POINT('Ctrl Pts',(14.0681284382562,-40.5129237928371,9.96399986488825));
#19503=CARTESIAN_POINT('Ctrl Pts',(13.9854285217579,-40.3709940943454,10.1252040678792));
#19504=CARTESIAN_POINT('Ctrl Pts',(13.9067100787601,-40.2271907619831,10.2868360245804));
#19505=CARTESIAN_POINT('Ctrl Pts',(13.8319900590775,-40.0815233709314,10.4489096280657));
#19506=CARTESIAN_POINT('',(17.4539382544776,-39.8448244996745,9.34999999998873));
#19507=CARTESIAN_POINT('Origin',(0.,0.,9.34999999999998));
#19508=CARTESIAN_POINT('',(17.240901531486,-38.7143550419874,10.4701702229062));
#19509=CARTESIAN_POINT('Ctrl Pts',(17.240901531486,-38.7143550419874,10.4701702229062));
#19510=CARTESIAN_POINT('Ctrl Pts',(17.291693095119,-38.9151697801545,10.2660612053903));
#19511=CARTESIAN_POINT('Ctrl Pts',(17.3358349265524,-39.1180277521759,10.0627475751681));
#19512=CARTESIAN_POINT('Ctrl Pts',(17.3733361291177,-39.3228942754465,9.86020040449296));
#19513=CARTESIAN_POINT('Ctrl Pts',(17.4049229028391,-39.4954506755349,9.68959756483997));
#19514=CARTESIAN_POINT('Ctrl Pts',(17.4317977424317,-39.6694324844584,9.5195380044732));
#19515=CARTESIAN_POINT('Ctrl Pts',(17.4539382544776,-39.8448244996745,9.34999999998873));
#19516=CARTESIAN_POINT('',(19.3953958606399,-37.7050538275443,10.4489096280657));
#19517=CARTESIAN_POINT('Ctrl Pts',(19.3953958606399,-37.7050538275443,10.4489096280657));
#19518=CARTESIAN_POINT('Ctrl Pts',(19.2186430289534,-37.6851626990031,10.5474492452249));
#19519=CARTESIAN_POINT('Ctrl Pts',(19.0301241631229,-37.6916090034775,10.6271602259564));
#19520=CARTESIAN_POINT('Ctrl Pts',(18.6188870194185,-37.7605037117185,10.7492445866574));
#19521=CARTESIAN_POINT('Ctrl Pts',(18.3988697140028,-37.8298236027886,10.7838550844415));
#19522=CARTESIAN_POINT('Ctrl Pts',(17.9802848030949,-38.0258387393331,10.7881210903218));
#19523=CARTESIAN_POINT('Ctrl Pts',(17.7856344105885,-38.1506895294622,10.7577447440201));
#19524=CARTESIAN_POINT('Ctrl Pts',(17.467333625089,-38.4234815582466,10.6429386483201));
#19525=CARTESIAN_POINT('Ctrl Pts',(17.3402981493128,-38.5649382940451,10.5662273743849));
#19526=CARTESIAN_POINT('Ctrl Pts',(17.240901531486,-38.7143550419874,10.4701702229062));
#19527=CARTESIAN_POINT('',(20.0984284630094,-38.5785325449048,9.34999999998873));
#19528=CARTESIAN_POINT('Ctrl Pts',(20.0984284630094,-38.5785325449048,9.34999999998873));
#19529=CARTESIAN_POINT('Ctrl Pts',(19.9564970965836,-38.4224589332658,9.55399283494912));
#19530=CARTESIAN_POINT('Ctrl Pts',(19.8205307458633,-38.2624219465728,9.75864949412501));
#19531=CARTESIAN_POINT('Ctrl Pts',(19.690525372939,-38.098457220019,9.9639998647895));
#19532=CARTESIAN_POINT('Ctrl Pts',(19.5884685202378,-37.9697415864286,10.1252040678131));
#19533=CARTESIAN_POINT('Ctrl Pts',(19.4900859694781,-37.8386047671006,10.2868360245473));
#19534=CARTESIAN_POINT('Ctrl Pts',(19.3953958606399,-37.7050538275443,10.4489096280657));
#19535=CARTESIAN_POINT('',(22.9467920842464,-36.9553072378427,9.34999999998873));
#19536=CARTESIAN_POINT('Origin',(0.,0.,9.34999999999998));
#19537=CARTESIAN_POINT('',(22.5750411898809,-35.8666626160155,10.4701702229111));
#19538=CARTESIAN_POINT('Ctrl Pts',(22.5750411898809,-35.8666626160155,10.4701702229111));
#19539=CARTESIAN_POINT('Ctrl Pts',(22.6538946856459,-36.0582049566081,10.2660612053122));
#19540=CARTESIAN_POINT('Ctrl Pts',(22.7264569163886,-36.2527160894467,10.0627475750089));
#19541=CARTESIAN_POINT('Ctrl Pts',(22.7927319569317,-36.450160389405,9.86020040425393));
#19542=CARTESIAN_POINT('Ctrl Pts',(22.848554558982,-36.6164651474763,9.68959756468081));
#19543=CARTESIAN_POINT('Ctrl Pts',(22.8999160444311,-36.7848513839179,9.51953800439383));
#19544=CARTESIAN_POINT('Ctrl Pts',(22.9467920842464,-36.9553072378427,9.34999999998873));
#19545=CARTESIAN_POINT('',(24.5639673341825,-34.5610181206248,10.4489096280657));
#19546=CARTESIAN_POINT('Ctrl Pts',(24.5639673341825,-34.5610181206248,10.4489096280657));
#19547=CARTESIAN_POINT('Ctrl Pts',(24.3861827887247,-34.5664840057473,10.5474492452249));
#19548=CARTESIAN_POINT('Ctrl Pts',(24.2005001779053,-34.5996937280391,10.6271602259563));
#19549=CARTESIAN_POINT('Ctrl Pts',(23.8032535746301,-34.7264123350864,10.7492445866574));
#19550=CARTESIAN_POINT('Ctrl Pts',(23.5953409772316,-34.826338376854,10.7838550844415));
#19551=CARTESIAN_POINT('Ctrl Pts',(23.2089125196235,-35.0799292058385,10.7881210903218));
#19552=CARTESIAN_POINT('Ctrl Pts',(23.0340115074557,-35.2312108340733,10.7577447440202));
#19553=CARTESIAN_POINT('Ctrl Pts',(22.7577729184581,-35.5465251581505,10.6429386483196));
#19554=CARTESIAN_POINT('Ctrl Pts',(22.652161873134,-35.7046211015317,10.5662273743844));
#19555=CARTESIAN_POINT('Ctrl Pts',(22.5750411898777,-35.8666626160111,10.4701702229063));
#19556=CARTESIAN_POINT('',(25.3841530607455,-35.3255541129878,9.34999999998873));
#19557=CARTESIAN_POINT('Ctrl Pts',(25.3841530607455,-35.3255541129878,9.34999999998873));
#19558=CARTESIAN_POINT('Ctrl Pts',(25.2214547601852,-35.1912680451366,9.55399283494599));
#19559=CARTESIAN_POINT('Ctrl Pts',(25.0640967129913,-35.0522100334294,9.75864949411873));
#19560=CARTESIAN_POINT('Ctrl Pts',(24.9120799937713,-34.908415924999,9.96399986478005));
#19561=CARTESIAN_POINT('Ctrl Pts',(24.7927437880966,-34.7955346354507,10.1252040678068));
#19562=CARTESIAN_POINT('Ctrl Pts',(24.676699914611,-34.6797338966578,10.2868360245441));
#19563=CARTESIAN_POINT('Ctrl Pts',(24.5639673341825,-34.5610181206248,10.4489096280657));
#19564=CARTESIAN_POINT('',(27.9725154002639,-33.3134864909541,9.34999999998873));
#19565=CARTESIAN_POINT('Origin',(0.,0.,9.34999999999998));
#19566=CARTESIAN_POINT('',(27.4496181106863,-32.288828370087,10.4701702229062));
#19567=CARTESIAN_POINT('Ctrl Pts',(27.4496181106863,-32.288828370087,10.4701702229062));
#19568=CARTESIAN_POINT('Ctrl Pts',(27.5549283087466,-32.4671990632689,10.2660612053897));
#19569=CARTESIAN_POINT('Ctrl Pts',(27.654433780983,-32.6494036710323,10.0627475751668));
#19570=CARTESIAN_POINT('Ctrl Pts',(27.748133490759,-32.8354063509565,9.86020040449105));
#19571=CARTESIAN_POINT('Ctrl Pts',(27.8270555339998,-32.99207398187,9.68959756483871));
#19572=CARTESIAN_POINT('Ctrl Pts',(27.9018580936275,-33.1514367877952,9.51953800447257));
#19573=CARTESIAN_POINT('Ctrl Pts',(27.9725154002639,-33.3134864909541,9.34999999998873));
#19574=CARTESIAN_POINT('',(29.2324872694335,-30.7134197505154,10.4489096280657));
#19575=CARTESIAN_POINT('Ctrl Pts',(29.2324872694335,-30.7134197505154,10.4489096280657));
#19576=CARTESIAN_POINT('Ctrl Pts',(29.0572901908615,-30.7441313796429,10.547449245225));
#19577=CARTESIAN_POINT('Ctrl Pts',(28.8782237975451,-30.8034284655751,10.6271602259564));
#19578=CARTESIAN_POINT('Ctrl Pts',(28.503054529977,-30.9853913460156,10.7492445866574));
#19579=CARTESIAN_POINT('Ctrl Pts',(28.3114791415082,-31.1138893324332,10.7838550844415));
#19580=CARTESIAN_POINT('Ctrl Pts',(27.9650737062293,-31.4198934758751,10.7881210903218));
#19581=CARTESIAN_POINT('Ctrl Pts',(27.8134825546349,-31.5945262845251,10.7577447440201));
#19582=CARTESIAN_POINT('Ctrl Pts',(27.5849295832075,-31.9459440135453,10.6429386483201));
#19583=CARTESIAN_POINT('Ctrl Pts',(27.5028929046594,-32.1174607870144,10.5662273743849));
#19584=CARTESIAN_POINT('Ctrl Pts',(27.4496181106863,-32.288828370087,10.4701702229062));
#19585=CARTESIAN_POINT('',(30.1531295040175,-31.3534492698161,9.34999999998873));
#19586=CARTESIAN_POINT('Ctrl Pts',(30.1531295040175,-31.3534492698161,9.34999999998873));
#19587=CARTESIAN_POINT('Ctrl Pts',(29.972976337535,-31.2436844228417,9.55399283494789));
#19588=CARTESIAN_POINT('Ctrl Pts',(29.7974299499217,-31.1284362062249,9.75864949412254));
#19589=CARTESIAN_POINT('Ctrl Pts',(29.6264965064259,-31.0077399492937,9.96399986478578));
#19590=CARTESIAN_POINT('Ctrl Pts',(29.4923102887919,-30.9129909413234,10.1252040678106));
#19591=CARTESIAN_POINT('Ctrl Pts',(29.3609674112053,-30.8148836521694,10.286836024546));
#19592=CARTESIAN_POINT('Ctrl Pts',(29.2324872694335,-30.7134197505154,10.4489096280657));
#19593=CARTESIAN_POINT('',(32.4287989688052,-28.9934992272716,9.34999999998873));
#19594=CARTESIAN_POINT('Origin',(0.,0.,9.34999999999998));
#19595=CARTESIAN_POINT('',(31.7653999649232,-28.0536866918398,10.4701702229062));
#19596=CARTESIAN_POINT('Ctrl Pts',(31.7653999649232,-28.0536866918398,10.4701702229062));
#19597=CARTESIAN_POINT('Ctrl Pts',(31.8950230533648,-28.2152546247487,10.2660612053899));
#19598=CARTESIAN_POINT('Ctrl Pts',(32.0194461226553,-28.3814435471337,10.0627475751671));
#19599=CARTESIAN_POINT('Ctrl Pts',(32.1386630458013,-28.5522181289268,9.86020040449154));
#19600=CARTESIAN_POINT('Ctrl Pts',(32.2390779049944,-28.6960593314338,9.68959756483903));
#19601=CARTESIAN_POINT('Ctrl Pts',(32.3357987743735,-28.8431545396011,9.51953800447273));
#19602=CARTESIAN_POINT('Ctrl Pts',(32.4287989688052,-28.9934992272716,9.34999999998873));
#19603=CARTESIAN_POINT('',(33.3059180634108,-26.2405847244742,10.4489096280657));
#19604=CARTESIAN_POINT('Ctrl Pts',(33.3059180634108,-26.2405847244742,10.4489096280657));
#19605=CARTESIAN_POINT('Ctrl Pts',(33.1368749590177,-26.2959168974026,10.5474492452249));
#19606=CARTESIAN_POINT('Ctrl Pts',(32.9680700585873,-26.3800942293043,10.6271602259564));
#19607=CARTESIAN_POINT('Ctrl Pts',(32.6226154911153,-26.6135971436299,10.7492445866574));
#19608=CARTESIAN_POINT('Ctrl Pts',(32.4512772340277,-26.7680512262516,10.7838550844415));
#19609=CARTESIAN_POINT('Ctrl Pts',(32.1519466367895,-27.1202393222335,10.7881210903218));
#19610=CARTESIAN_POINT('Ctrl Pts',(32.0267513044621,-27.314668290914,10.7577447440201));
#19611=CARTESIAN_POINT('Ctrl Pts',(31.8505366300096,-27.6950355733208,10.6429386483201));
#19612=CARTESIAN_POINT('Ctrl Pts',(31.7937443484394,-27.8764815899828,10.5662273743849));
#19613=CARTESIAN_POINT('Ctrl Pts',(31.7653999649232,-28.0536866918397,10.4701702229062));
#19614=CARTESIAN_POINT('',(34.3082751850326,-26.7430786153924,9.34999999998873));
#19615=CARTESIAN_POINT('Ctrl Pts',(34.3082751850326,-26.7430786153924,9.34999999998873));
#19616=CARTESIAN_POINT('Ctrl Pts',(34.1143345515806,-26.6600694850449,9.55399283494758));
#19617=CARTESIAN_POINT('Ctrl Pts',(33.9241734417673,-26.5709771848618,9.75864949412193));
#19618=CARTESIAN_POINT('Ctrl Pts',(33.7378029859755,-26.4758358071633,9.96399986478487));
#19619=CARTESIAN_POINT('Ctrl Pts',(33.5914984008104,-26.4011478973383,10.12520406781));
#19620=CARTESIAN_POINT('Ctrl Pts',(33.4475302813471,-26.3227312393108,10.2868360245457));
#19621=CARTESIAN_POINT('Ctrl Pts',(33.3059180634108,-26.2405847244742,10.4489096280657));
#19622=CARTESIAN_POINT('',(36.2249257072755,-24.0832879296693,9.34999999998873));
#19623=CARTESIAN_POINT('Origin',(0.,0.,9.34999999999998));
#19624=CARTESIAN_POINT('',(35.4345298797235,-23.2474528526985,10.4701702229062));
#19625=CARTESIAN_POINT('Ctrl Pts',(35.4345298797235,-23.2474528526985,10.4701702229062));
#19626=CARTESIAN_POINT('Ctrl Pts',(35.5858271062678,-23.3889289681439,10.26606120539));
#19627=CARTESIAN_POINT('Ctrl Pts',(35.7326348777281,-23.53571907794,10.0627475751674));
#19628=CARTESIAN_POINT('Ctrl Pts',(35.874942101482,-23.68778908359,9.86020040449197));
#19629=CARTESIAN_POINT('Ctrl Pts',(35.9948056196667,-23.8158756656113,9.68959756483931));
#19630=CARTESIAN_POINT('Ctrl Pts',(36.1114758408168,-23.94770884177,9.51953800447287));
#19631=CARTESIAN_POINT('Ctrl Pts',(36.2249257072755,-24.0832879296692,9.34999999998873));
#19632=CARTESIAN_POINT('',(36.7013364119534,-21.2335670650402,10.4489096280657));
#19633=CARTESIAN_POINT('Ctrl Pts',(36.7013364119534,-21.2335670650402,10.4489096280657));
#19634=CARTESIAN_POINT('Ctrl Pts',(36.5418885288435,-21.3123933698997,10.547449234732));
#19635=CARTESIAN_POINT('Ctrl Pts',(36.3867815182114,-21.4197373256359,10.6271602090589));
#19636=CARTESIAN_POINT('Ctrl Pts',(36.0780741043059,-21.7000268175684,10.7492445801565));
#19637=CARTESIAN_POINT('Ctrl Pts',(35.9304609153722,-21.8772927714271,10.7838550842413));
#19638=CARTESIAN_POINT('Ctrl Pts',(35.6842986623995,-22.2684952883836,10.7881210901482));
#19639=CARTESIAN_POINT('Ctrl Pts',(35.5880477708337,-22.4787623858218,10.7577447489718));
#19640=CARTESIAN_POINT('Ctrl Pts',(35.4677586059889,-22.8803360402157,10.6429386624017));
#19641=CARTESIAN_POINT('Ctrl Pts',(35.4373668431343,-23.068017600367,10.5662273832428));
#19642=CARTESIAN_POINT('Ctrl Pts',(35.4345298797234,-23.2474528526985,10.4701702229062));
#19643=CARTESIAN_POINT('',(37.7650033201761,-21.5882960010295,9.34999999998873));
#19644=CARTESIAN_POINT('Ctrl Pts',(37.7650033201761,-21.5882960010295,9.34999999998873));
#19645=CARTESIAN_POINT('Ctrl Pts',(37.561223291772,-21.5337324138238,9.55399283494828));
#19646=CARTESIAN_POINT('Ctrl Pts',(37.3603185915744,-21.4726096923848,9.75864949412332));
#19647=CARTESIAN_POINT('Ctrl Pts',(37.1623050885176,-21.4049599980034,9.96399986478697));
#19648=CARTESIAN_POINT('Ctrl Pts',(37.0068604752686,-21.351853616786,10.1252040678114));
#19649=CARTESIAN_POINT('Ctrl Pts',(36.8531978896722,-21.2947239269079,10.2868360245464));
#19650=CARTESIAN_POINT('Ctrl Pts',(36.7013364119534,-21.2335670650402,10.4489096280657));
#19651=CARTESIAN_POINT('',(39.2836174224049,-18.6828103402862,9.34999999998873));
#19652=CARTESIAN_POINT('Origin',(0.,0.,9.34999999999998));
#19653=CARTESIAN_POINT('',(38.3823149509235,-17.967967913596,10.4701702229111));
#19654=CARTESIAN_POINT('Ctrl Pts',(38.3823149509235,-17.9679679135961,10.4701702229111));
#19655=CARTESIAN_POINT('Ctrl Pts',(38.5522063404067,-18.0864721658963,10.2660612053129));
#19656=CARTESIAN_POINT('Ctrl Pts',(38.7184102312306,-18.2108752398261,10.0627475750103));
#19657=CARTESIAN_POINT('Ctrl Pts',(38.8809107909569,-18.3411449626069,9.86020040425606));
#19658=CARTESIAN_POINT('Ctrl Pts',(39.0177828924946,-18.4508694506564,9.68959756468223));
#19659=CARTESIAN_POINT('Ctrl Pts',(39.1520273960987,-18.5647568514646,9.51953800439454));
#19660=CARTESIAN_POINT('Ctrl Pts',(39.2836174224049,-18.6828103402862,9.34999999998873));
#19661=CARTESIAN_POINT('',(39.3496213890631,-15.794295212713,10.4489096280657));
#19662=CARTESIAN_POINT('Ctrl Pts',(39.3496213890631,-15.794295212713,10.4489096280657));
#19663=CARTESIAN_POINT('Ctrl Pts',(39.2030145927147,-15.8950109898697,10.5474492452249));
#19664=CARTESIAN_POINT('Ctrl Pts',(39.0647629717849,-16.0233363845726,10.6271602259564));
#19665=CARTESIAN_POINT('Ctrl Pts',(38.7990871146753,-16.3447065887528,10.7492445866574));
#19666=CARTESIAN_POINT('Ctrl Pts',(38.6782040045,-16.5411757610285,10.7838550844415));
#19667=CARTESIAN_POINT('Ctrl Pts',(38.4902212524321,-16.9634289390146,10.7881210903218));
#19668=CARTESIAN_POINT('Ctrl Pts',(38.4248741812051,-17.1852537694119,10.7577447440202));
#19669=CARTESIAN_POINT('Ctrl Pts',(38.3629592862311,-17.5998589150624,10.6429386483196));
#19670=CARTESIAN_POINT('Ctrl Pts',(38.3595867413122,-17.7899553278346,10.5662273743845));
#19671=CARTESIAN_POINT('Ctrl Pts',(38.3823149509184,-17.9679679135941,10.4701702229063));
#19672=CARTESIAN_POINT('',(40.4529448929973,-15.9940379355905,9.34999999998873));
#19673=CARTESIAN_POINT('Ctrl Pts',(40.4529448929973,-15.9940379355905,9.34999999998873));
#19674=CARTESIAN_POINT('Ctrl Pts',(40.2434738433687,-15.9690306488142,9.5539928349466));
#19675=CARTESIAN_POINT('Ctrl Pts',(40.0359153931237,-15.937121788465,9.75864949411995));
#19676=CARTESIAN_POINT('Ctrl Pts',(39.8302898267027,-15.8983409300935,9.96399986478188));
#19677=CARTESIAN_POINT('Ctrl Pts',(39.668869589428,-15.8678971702586,10.125204067808));
#19678=CARTESIAN_POINT('Ctrl Pts',(39.5086406648125,-15.8332174442667,10.2868360245447));
#19679=CARTESIAN_POINT('Ctrl Pts',(39.3496213890631,-15.794295212713,10.4489096280657));
#19680=CARTESIAN_POINT('',(41.5426079714121,-12.9020046091509,9.34999999998873));
#19681=CARTESIAN_POINT('Origin',(0.,0.,9.34999999999998));
#19682=CARTESIAN_POINT('',(40.5487467751689,-12.3227069631099,10.4701702229062));
#19683=CARTESIAN_POINT('Ctrl Pts',(40.5487467751689,-12.3227069631099,10.4701702229062));
#19684=CARTESIAN_POINT('Ctrl Pts',(40.7337738287019,-12.4158269473367,10.2660612053901));
#19685=CARTESIAN_POINT('Ctrl Pts',(40.9159904068419,-12.5153104974644,10.0627475751677));
#19686=CARTESIAN_POINT('Ctrl Pts',(41.0953762596389,-12.6211280213779,9.86020040449231));
#19687=CARTESIAN_POINT('Ctrl Pts',(41.2464706233799,-12.7102567413914,9.68959756483955));
#19688=CARTESIAN_POINT('Ctrl Pts',(41.3955565785992,-12.8038799478931,9.51953800447299));
#19689=CARTESIAN_POINT('Ctrl Pts',(41.5426079714121,-12.9020046091509,9.34999999998874));
#19690=CARTESIAN_POINT('',(41.196861549629,-10.0334970568411,10.4489096280657));
#19691=CARTESIAN_POINT('Ctrl Pts',(41.196861549629,-10.0334970568411,10.4489096280657));
#19692=CARTESIAN_POINT('Ctrl Pts',(41.0660803486155,-10.1540520151186,10.5474492452249));
#19693=CARTESIAN_POINT('Ctrl Pts',(40.9474985376378,-10.3007464994071,10.6271602259564));
#19694=CARTESIAN_POINT('Ctrl Pts',(40.7302626263144,-10.6566552349241,10.7492445866574));
#19695=CARTESIAN_POINT('Ctrl Pts',(40.6385704103798,-10.8683280945857,10.7838550844415));
#19696=CARTESIAN_POINT('Ctrl Pts',(40.5125939444147,-11.3130360790174,10.7881210903218));
#19697=CARTESIAN_POINT('Ctrl Pts',(40.4794809770131,-11.5419029103595,10.7577447440201));
#19698=CARTESIAN_POINT('Ctrl Pts',(40.4772007506466,-11.9610993817016,10.6429386483201));
#19699=CARTESIAN_POINT('Ctrl Pts',(40.5009160736119,-12.1497408502739,10.5662273743849));
#19700=CARTESIAN_POINT('Ctrl Pts',(40.5487467751689,-12.3227069631099,10.4701702229062));
#19701=CARTESIAN_POINT('',(42.3173811644568,-10.0741873807795,9.34999999998873));
#19702=CARTESIAN_POINT('Ctrl Pts',(42.3173811644568,-10.0741873807795,9.34999999998873));
#19703=CARTESIAN_POINT('Ctrl Pts',(42.1064833201074,-10.0792454706758,9.55399283494713));
#19704=CARTESIAN_POINT('Ctrl Pts',(41.8964964113107,-10.0772000437951,9.75864949412103));
#19705=CARTESIAN_POINT('Ctrl Pts',(41.6874447250805,-10.0680774878744,9.96399986478351));
#19706=CARTESIAN_POINT('Ctrl Pts',(41.5233349143157,-10.0609160965801,10.1252040678091));
#19707=CARTESIAN_POINT('Ctrl Pts',(41.3598014495264,-10.0493923136882,10.2868360245452));
#19708=CARTESIAN_POINT('Ctrl Pts',(41.196861549629,-10.0334970568411,10.4489096280657));
#19709=CARTESIAN_POINT('',(42.9559108211099,-6.85855127048217,9.34999999998873));
#19710=CARTESIAN_POINT('Origin',(0.,0.,9.34999999999998));
#19711=CARTESIAN_POINT('',(41.8897230480066,-6.42659123460911,10.4701702229062));
#19712=CARTESIAN_POINT('Ctrl Pts',(41.8897230480066,-6.42659123460911,10.4701702229062));
#19713=CARTESIAN_POINT('Ctrl Pts',(42.0861191484164,-6.49243129646455,10.2660612053906));
#19714=CARTESIAN_POINT('Ctrl Pts',(42.2806390098723,-6.56497012464645,10.0627475751687));
#19715=CARTESIAN_POINT('Ctrl Pts',(42.4732583771426,-6.64418131011315,9.86020040449385));
#19716=CARTESIAN_POINT('Ctrl Pts',(42.6354991574955,-6.71089985833033,9.68959756484057));
#19717=CARTESIAN_POINT('Ctrl Pts',(42.7963916041473,-6.78235297197774,9.5195380044735));
#19718=CARTESIAN_POINT('Ctrl Pts',(42.9559108211099,-6.85855127048219,9.34999999998874));
#19719=CARTESIAN_POINT('',(42.2054524109828,-4.06844583510822,10.4489096280657));
#19720=CARTESIAN_POINT('Ctrl Pts',(42.2054524109828,-4.06844583510822,10.4489096280657));
#19721=CARTESIAN_POINT('Ctrl Pts',(42.0931591334149,-4.20638582320779,10.547449245225));
#19722=CARTESIAN_POINT('Ctrl Pts',(41.9966611160993,-4.36846312041362,10.6271602259564));
#19723=CARTESIAN_POINT('Ctrl Pts',(41.83228744726,-4.7516651117681,10.7492445866574));
#19724=CARTESIAN_POINT('Ctrl Pts',(41.7716527146639,-4.9742326098071,10.7838550844415));
#19725=CARTESIAN_POINT('Ctrl Pts',(41.7102470523625,-5.43234242855341,10.7881210903218));
#19726=CARTESIAN_POINT('Ctrl Pts',(41.7100422733126,-5.66359219215167,10.7577447440201));
#19727=CARTESIAN_POINT('Ctrl Pts',(41.7674431343865,-6.07884635789341,10.6429386483201));
#19728=CARTESIAN_POINT('Ctrl Pts',(41.8177635496502,-6.26219268596175,10.5662273743849));
#19729=CARTESIAN_POINT('Ctrl Pts',(41.8897230480066,-6.42659123460911,10.4701702229062));
#19730=CARTESIAN_POINT('',(43.3203575886581,-3.94925542245321,9.34999999998874));
#19731=CARTESIAN_POINT('Ctrl Pts',(43.3203575886581,-3.94925542245321,9.34999999998874));
#19732=CARTESIAN_POINT('Ctrl Pts',(43.1123262215187,-3.98427592089861,9.55399283494855));
#19733=CARTESIAN_POINT('Ctrl Pts',(42.9041855820802,-4.01213556647932,9.75864949412385));
#19734=CARTESIAN_POINT('Ctrl Pts',(42.6959634655163,-4.03285702194092,9.96399986478776));
#19735=CARTESIAN_POINT('Ctrl Pts',(42.5325048837559,-4.04912378446192,10.1252040678119));
#19736=CARTESIAN_POINT('Ctrl Pts',(42.3689959485452,-4.06099053565752,10.2868360245467));
#19737=CARTESIAN_POINT('Ctrl Pts',(42.2054524109828,-4.06844583510822,10.4489096280657));
#19738=CARTESIAN_POINT('',(43.4947552011075,-0.675477606375033,9.34999999998873));
#19739=CARTESIAN_POINT('Origin',(0.,0.,9.34999999999998));
#19740=CARTESIAN_POINT('',(42.3779453595727,-0.399648641330356,10.4701702229062));
#19741=CARTESIAN_POINT('Ctrl Pts',(42.3779453595728,-0.399648641330362,
10.4701702229062));
#19742=CARTESIAN_POINT('Ctrl Pts',(42.5817124486174,-0.436868467022762,
10.2660612053882));
#19743=CARTESIAN_POINT('Ctrl Pts',(42.7845757299618,-0.480985891902701,
10.0627475751638));
#19744=CARTESIAN_POINT('Ctrl Pts',(42.9865074368591,-0.531978227613834,
9.8602004044866));
#19745=CARTESIAN_POINT('Ctrl Pts',(43.1565918793968,-0.574928406792644,
9.68959756483575));
#19746=CARTESIAN_POINT('Ctrl Pts',(43.3260155112399,-0.622756848244752,
9.5195380044711));
#19747=CARTESIAN_POINT('Ctrl Pts',(43.4947552011075,-0.675477606375036,
9.34999999998873));
#19748=CARTESIAN_POINT('',(42.1897980655053,1.5002221180317E-9,10.6602019344947));
#19749=CARTESIAN_POINT('Ctrl Pts',(42.3779453595728,-0.399648641330344,
10.4701702229062));
#19750=CARTESIAN_POINT('Ctrl Pts',(42.3148062568321,-0.29790085588298,10.5342660162233));
#19751=CARTESIAN_POINT('Ctrl Pts',(42.2599040956416,-0.186267410922431,
10.5898537840787));
#19752=CARTESIAN_POINT('Ctrl Pts',(42.2057277134261,-0.0448313813822705,
10.6442542383995));
#19753=CARTESIAN_POINT('Ctrl Pts',(42.1975989914554,-0.0225266414925362,
10.6524010085462));
#19754=CARTESIAN_POINT('Ctrl Pts',(42.1897980655053,3.00045025180458E-9,
10.6602019344947));
#19755=CARTESIAN_POINT('',(41.5,-6.81700769243921E-15,11.35));
#19756=CARTESIAN_POINT('',(41.5,-6.81700769243921E-15,11.35));
#19757=CARTESIAN_POINT('Origin',(-1.73472347597681E-15,-1.73472347597681E-15,
11.35));
#19758=CARTESIAN_POINT('',(42.3548619717231,1.97942721139859,10.4489096280657));
#19759=CARTESIAN_POINT('Ctrl Pts',(42.1897980655053,3.00045276818706E-9,
10.6602019344947));
#19760=CARTESIAN_POINT('Ctrl Pts',(42.1528402486422,0.106722667340138,10.6971597513502));
#19761=CARTESIAN_POINT('Ctrl Pts',(42.1232380522063,0.21842602329369,10.7263532092198));
#19762=CARTESIAN_POINT('Ctrl Pts',(42.0584163598968,0.559888029352808,10.7884683253291));
#19763=CARTESIAN_POINT('Ctrl Pts',(42.0461300361259,0.795750669329838,10.796977768321));
#19764=CARTESIAN_POINT('Ctrl Pts',(42.0800217201965,1.20911028675496,10.7529995432141));
#19765=CARTESIAN_POINT('Ctrl Pts',(42.1138228892831,1.38567030932342,10.7137049327916));
#19766=CARTESIAN_POINT('Ctrl Pts',(42.2140016405932,1.70669242726629,10.6017906159603));
#19767=CARTESIAN_POINT('Ctrl Pts',(42.277687969919,1.8508168222083,10.5320034604965));
#19768=CARTESIAN_POINT('Ctrl Pts',(42.3548619717231,1.97942721139858,10.4489096280657));
#19769=CARTESIAN_POINT('',(43.4414564579495,2.25607198756208,9.34999999998873));
#19770=CARTESIAN_POINT('Ctrl Pts',(43.4414564579495,2.25607198756207,9.34999999998873));
#19771=CARTESIAN_POINT('Ctrl Pts',(43.2405264867429,2.19180199692502,9.55399283494924));
#19772=CARTESIAN_POINT('Ctrl Pts',(43.0384692598544,2.13460442092607,9.75864949412525));
#19773=CARTESIAN_POINT('Ctrl Pts',(42.8353155147877,2.08446078315935,9.96399986478986));
#19774=CARTESIAN_POINT('Ctrl Pts',(42.6758357073799,2.04509701119868,10.1252040678133));
#19775=CARTESIAN_POINT('Ctrl Pts',(42.5156798721472,2.01008129874923,10.2868360245474));
#19776=CARTESIAN_POINT('Ctrl Pts',(42.3548619717231,1.97942721139858,10.4489096280657));
#19777=CARTESIAN_POINT('',(43.1481717937269,5.52134683388133,9.34999999998873));
#19778=CARTESIAN_POINT('Origin',(0.,0.,9.34999999999998));
#19779=CARTESIAN_POINT('',(42.0034749115207,5.63542964579432,10.4701702229062));
#19780=CARTESIAN_POINT('Ctrl Pts',(42.0034749115207,5.63542964579433,10.4701702229062));
#19781=CARTESIAN_POINT('Ctrl Pts',(42.2104648788808,5.62758774458373,10.2660612053881));
#19782=CARTESIAN_POINT('Ctrl Pts',(42.4175418687127,5.6127898265531,10.0627475751637));
#19783=CARTESIAN_POINT('Ctrl Pts',(42.6246751680052,5.59105439750396,9.86020040448641));
#19784=CARTESIAN_POINT('Ctrl Pts',(42.799140843963,5.5727469291527,9.68959756483562));
#19785=CARTESIAN_POINT('Ctrl Pts',(42.9736466844327,5.54951680903709,9.51953800447104));
#19786=CARTESIAN_POINT('Ctrl Pts',(43.1481717937269,5.52134683388132,9.34999999998873));
#19787=CARTESIAN_POINT('',(41.6420486840549,7.98700482807798,10.4489096280657));
#19788=CARTESIAN_POINT('Ctrl Pts',(41.6420486840549,7.98700482807798,10.4489096280657));
#19789=CARTESIAN_POINT('Ctrl Pts',(41.5731662587824,7.82301570651073,10.547449245225));
#19790=CARTESIAN_POINT('Ctrl Pts',(41.526239540548,7.64031704551083,10.6271602259564));
#19791=CARTESIAN_POINT('Ctrl Pts',(41.4764846370605,7.22632801333153,10.7492445866574));
#19792=CARTESIAN_POINT('Ctrl Pts',(41.4810105474699,6.99569328456048,10.7838550844415));
#19793=CARTESIAN_POINT('Ctrl Pts',(41.5511566965011,6.53884015808498,10.7881210903218));
#19794=CARTESIAN_POINT('Ctrl Pts',(41.6161107996091,6.31689994183708,10.7577447440201));
#19795=CARTESIAN_POINT('Ctrl Pts',(41.7881771403425,5.93463817889894,10.6429386483201));
#19796=CARTESIAN_POINT('Ctrl Pts',(41.8881138550115,5.77289556463294,10.5662273743849));
#19797=CARTESIAN_POINT('Ctrl Pts',(42.0034749115207,5.63542964579435,10.4701702229062));
#19798=CARTESIAN_POINT('',(42.6782125485725,8.4154722778849,9.34999999998873));
#19799=CARTESIAN_POINT('Ctrl Pts',(42.6782125485725,8.41547227788491,9.34999999998874));
#19800=CARTESIAN_POINT('Ctrl Pts',(42.4884743280791,8.32326114672637,9.55399283494921));
#19801=CARTESIAN_POINT('Ctrl Pts',(42.2966138161958,8.23789001801242,9.75864949412517));
#19802=CARTESIAN_POINT('Ctrl Pts',(42.1026640670296,8.15934497780325,9.96399986478974));
#19803=CARTESIAN_POINT('Ctrl Pts',(41.9504095829507,8.09768552928415,10.1252040678132));
#19804=CARTESIAN_POINT('Ctrl Pts',(41.7968671586493,8.04023367450927,10.2868360245473));
#19805=CARTESIAN_POINT('Ctrl Pts',(41.6420486840549,7.98700482807799,10.4489096280657));
#19806=CARTESIAN_POINT('',(41.9232160376784,11.6057725748493,9.34999999998873));
#19807=CARTESIAN_POINT('Origin',(0.,0.,9.34999999999998));
#19808=CARTESIAN_POINT('',(40.7739348422944,11.5557868365697,10.4701702229111));
#19809=CARTESIAN_POINT('Ctrl Pts',(40.7739348422944,11.5557868365697,10.4701702229111));
#19810=CARTESIAN_POINT('Ctrl Pts',(40.9799339692217,11.5774824983428,10.2660612053109));
#19811=CARTESIAN_POINT('Ctrl Pts',(41.1870091772687,11.5923053301016,10.0627475750063));
#19812=CARTESIAN_POINT('Ctrl Pts',(41.3951274323872,11.6002692783676,9.86020040425015));
#19813=CARTESIAN_POINT('Ctrl Pts',(41.5704227236392,11.6069772080973,9.6895975646783));
#19814=CARTESIAN_POINT('Ctrl Pts',(41.7464583369758,11.6088183075705,9.51953800439259));
#19815=CARTESIAN_POINT('Ctrl Pts',(41.9232160376784,11.6057725748493,9.34999999998873));
#19816=CARTESIAN_POINT('',(40.0815233709314,13.8319900590777,10.4489096280657));
#19817=CARTESIAN_POINT('Ctrl Pts',(40.0815233709314,13.8319900590777,10.4489096280657));
#19818=CARTESIAN_POINT('Ctrl Pts',(40.0366801547423,13.6598671191027,10.5474492452249));
#19819=CARTESIAN_POINT('Ctrl Pts',(40.0162318132298,13.4723496987259,10.6271602259563));
#19820=CARTESIAN_POINT('Ctrl Pts',(40.0259001250806,13.0554936169282,10.7492445866574));
#19821=CARTESIAN_POINT('Ctrl Pts',(40.0632027123731,12.8278505213561,10.7838550844415));
#19822=CARTESIAN_POINT('Ctrl Pts',(40.1976518535586,12.3856303388352,10.7881210903218));
#19823=CARTESIAN_POINT('Ctrl Pts',(40.2935302035347,12.1751930866563,10.7577447440202));
#19824=CARTESIAN_POINT('Ctrl Pts',(40.5182466779901,11.8213097907411,10.6429386483196));
#19825=CARTESIAN_POINT('Ctrl Pts',(40.6401845549916,11.6754359604614,10.5662273743844));
#19826=CARTESIAN_POINT('Ctrl Pts',(40.7739348422892,11.5557868365679,10.4701702229063));
#19827=CARTESIAN_POINT('',(41.0461633055085,14.403557820848,9.34999999998873));
#19828=CARTESIAN_POINT('Ctrl Pts',(41.0461633055085,14.403557820848,9.34999999998873));
#19829=CARTESIAN_POINT('Ctrl Pts',(40.8714793587102,14.2852827018649,9.55399283498124));
#19830=CARTESIAN_POINT('Ctrl Pts',(40.6937212885455,14.1734759304099,9.75864949418953));
#19831=CARTESIAN_POINT('Ctrl Pts',(40.5129237928385,14.0681284382572,9.9639998648866));
#19832=CARTESIAN_POINT('Ctrl Pts',(40.3709940943463,13.9854285217585,10.125204067878));
#19833=CARTESIAN_POINT('Ctrl Pts',(40.2271907619836,13.9067100787605,10.2868360245799));
#19834=CARTESIAN_POINT('Ctrl Pts',(40.0815233709314,13.8319900590777,10.4489096280657));
#19835=CARTESIAN_POINT('',(39.8448244996745,17.4539382544778,9.34999999998873));
#19836=CARTESIAN_POINT('Origin',(0.,0.,9.34999999999998));
#19837=CARTESIAN_POINT('',(38.714355041992,17.2409015314888,10.4701702229111));
#19838=CARTESIAN_POINT('Ctrl Pts',(38.714355041992,17.2409015314888,10.4701702229111));
#19839=CARTESIAN_POINT('Ctrl Pts',(38.9151697802342,17.29169309514,10.2660612053137));
#19840=CARTESIAN_POINT('Ctrl Pts',(39.1180277523337,17.3358349265873,10.062747575012));
#19841=CARTESIAN_POINT('Ctrl Pts',(39.3228942756845,17.3733361291616,9.86020040425854));
#19842=CARTESIAN_POINT('Ctrl Pts',(39.4954506756946,17.404922902864,9.68959756468387));
#19843=CARTESIAN_POINT('Ctrl Pts',(39.6694324845389,17.431797742442,9.51953800439536));
#19844=CARTESIAN_POINT('Ctrl Pts',(39.8448244996745,17.4539382544777,9.34999999998873));
#19845=CARTESIAN_POINT('',(37.7050538275442,19.39539586064,10.4489096280657));
#19846=CARTESIAN_POINT('Ctrl Pts',(37.7050538275442,19.39539586064,10.4489096280657));
#19847=CARTESIAN_POINT('Ctrl Pts',(37.6851626990031,19.2186430289535,10.547449245225));
#19848=CARTESIAN_POINT('Ctrl Pts',(37.6916090034774,19.0301241631231,10.6271602259564));
#19849=CARTESIAN_POINT('Ctrl Pts',(37.7605037117184,18.6188870194187,10.7492445866574));
#19850=CARTESIAN_POINT('Ctrl Pts',(37.8298236027886,18.3988697140031,10.7838550844415));
#19851=CARTESIAN_POINT('Ctrl Pts',(38.0258387393331,17.9802848030951,10.7881210903218));
#19852=CARTESIAN_POINT('Ctrl Pts',(38.1506895294621,17.7856344105887,10.7577447440202));
#19853=CARTESIAN_POINT('Ctrl Pts',(38.4234815582478,17.4673336250877,10.6429386483196));
#19854=CARTESIAN_POINT('Ctrl Pts',(38.5649382940458,17.3402981493125,10.5662273743844));
#19855=CARTESIAN_POINT('Ctrl Pts',(38.7143550419872,17.2409015314862,10.4701702229063));
#19856=CARTESIAN_POINT('',(38.5785325449047,20.0984284630095,9.34999999998873));
#19857=CARTESIAN_POINT('Ctrl Pts',(38.5785325449047,20.0984284630095,9.34999999998873));
#19858=CARTESIAN_POINT('Ctrl Pts',(38.4224589332413,19.9564970965615,9.55399283498114));
#19859=CARTESIAN_POINT('Ctrl Pts',(38.2624219465224,19.8205307458207,9.75864949418933));
#19860=CARTESIAN_POINT('Ctrl Pts',(38.0984572199416,19.6905253728779,9.96399986488629));
#19861=CARTESIAN_POINT('Ctrl Pts',(37.969741586376,19.5884685201986,10.1252040678778));
#19862=CARTESIAN_POINT('Ctrl Pts',(37.8386047670737,19.4900859694592,10.2868360245798));
#19863=CARTESIAN_POINT('Ctrl Pts',(37.7050538275442,19.39539586064,10.4489096280657));
#19864=CARTESIAN_POINT('',(36.9553072378426,22.9467920842465,9.34999999998873));
#19865=CARTESIAN_POINT('Origin',(0.,0.,9.34999999999998));
#19866=CARTESIAN_POINT('',(35.8666626160154,22.575041189881,10.4701702229111));
#19867=CARTESIAN_POINT('Ctrl Pts',(35.8666626160154,22.575041189881,10.4701702229111));
#19868=CARTESIAN_POINT('Ctrl Pts',(36.0582049566091,22.6538946856465,10.266061205311));
#19869=CARTESIAN_POINT('Ctrl Pts',(36.2527160894488,22.7264569163896,10.0627475750066));
#19870=CARTESIAN_POINT('Ctrl Pts',(36.4501603894082,22.792731956933,9.86020040425056));
#19871=CARTESIAN_POINT('Ctrl Pts',(36.6164651474784,22.8485545589829,9.68959756467857));
#19872=CARTESIAN_POINT('Ctrl Pts',(36.784851383919,22.8999160444316,9.51953800439272));
#19873=CARTESIAN_POINT('Ctrl Pts',(36.9553072378426,22.9467920842465,9.34999999998873));
#19874=CARTESIAN_POINT('',(34.5610181206247,24.5639673341826,10.4489096280657));
#19875=CARTESIAN_POINT('Ctrl Pts',(34.5610181206247,24.5639673341826,10.4489096280657));
#19876=CARTESIAN_POINT('Ctrl Pts',(34.5664840057472,24.3861827887248,10.547449245225));
#19877=CARTESIAN_POINT('Ctrl Pts',(34.599693728039,24.2005001779054,10.6271602259563));
#19878=CARTESIAN_POINT('Ctrl Pts',(34.7264123350863,23.8032535746302,10.7492445866574));
#19879=CARTESIAN_POINT('Ctrl Pts',(34.8263383768539,23.5953409772317,10.7838550844415));
#19880=CARTESIAN_POINT('Ctrl Pts',(35.0799292058384,23.2089125196236,10.7881210903218));
#19881=CARTESIAN_POINT('Ctrl Pts',(35.2312108340732,23.0340115074558,10.7577447440202));
#19882=CARTESIAN_POINT('Ctrl Pts',(35.5465251581503,22.7577729184583,10.6429386483196));
#19883=CARTESIAN_POINT('Ctrl Pts',(35.7046211015316,22.6521618731341,10.5662273743845));
#19884=CARTESIAN_POINT('Ctrl Pts',(35.866662616011,22.5750411898778,10.4701702229063));
#19885=CARTESIAN_POINT('',(35.3255541129877,25.3841530607456,9.34999999998873));
#19886=CARTESIAN_POINT('Ctrl Pts',(35.3255541129877,25.3841530607456,9.34999999998873));
#19887=CARTESIAN_POINT('Ctrl Pts',(35.1912680451137,25.2214547601577,9.55399283498059));
#19888=CARTESIAN_POINT('Ctrl Pts',(35.0522100333821,25.064096712938,9.75864949418821));
#19889=CARTESIAN_POINT('Ctrl Pts',(34.9084159249257,24.912079993694,9.96399986488461));
#19890=CARTESIAN_POINT('Ctrl Pts',(34.7955346354005,24.7927437880465,10.1252040678767));
#19891=CARTESIAN_POINT('Ctrl Pts',(34.679733896632,24.6766999145867,10.2868360245792));
#19892=CARTESIAN_POINT('Ctrl Pts',(34.5610181206247,24.5639673341826,10.4489096280657));
#19893=CARTESIAN_POINT('',(33.313486490954,27.972515400264,9.34999999998873));
#19894=CARTESIAN_POINT('Origin',(0.,0.,9.34999999999998));
#19895=CARTESIAN_POINT('',(32.2888283700906,27.4496181106902,10.4701702229111));
#19896=CARTESIAN_POINT('Ctrl Pts',(32.2888283700906,27.4496181106902,10.4701702229111));
#19897=CARTESIAN_POINT('Ctrl Pts',(32.4671990633379,27.5549283087883,10.2660612053147));
#19898=CARTESIAN_POINT('Ctrl Pts',(32.6494036711709,27.6544337810593,10.062747575014));
#19899=CARTESIAN_POINT('Ctrl Pts',(32.835406351168,27.7481334908659,9.86020040426154));
#19900=CARTESIAN_POINT('Ctrl Pts',(32.9920739820132,27.8270555340672,9.68959756468587));
#19901=CARTESIAN_POINT('Ctrl Pts',(33.1514367878679,27.9018580936594,9.51953800439635));
#19902=CARTESIAN_POINT('Ctrl Pts',(33.313486490954,27.972515400264,9.34999999998873));
#19903=CARTESIAN_POINT('',(30.7134197505153,29.2324872694336,10.4489096280657));
#19904=CARTESIAN_POINT('Ctrl Pts',(30.7134197505153,29.2324872694336,10.4489096280657));
#19905=CARTESIAN_POINT('Ctrl Pts',(30.7441313796428,29.0572901908616,10.5474492452249));
#19906=CARTESIAN_POINT('Ctrl Pts',(30.803428465575,28.8782237975452,10.6271602259564));
#19907=CARTESIAN_POINT('Ctrl Pts',(30.9853913460155,28.5030545299772,10.7492445866574));
#19908=CARTESIAN_POINT('Ctrl Pts',(31.113889332433,28.3114791415084,10.7838550844415));
#19909=CARTESIAN_POINT('Ctrl Pts',(31.4198934758749,27.9650737062295,10.7881210903218));
#19910=CARTESIAN_POINT('Ctrl Pts',(31.5945262845249,27.813482554635,10.7577447440202));
#19911=CARTESIAN_POINT('Ctrl Pts',(31.9459440135467,27.5849295832066,10.6429386483196));
#19912=CARTESIAN_POINT('Ctrl Pts',(32.1174607870151,27.5028929046593,10.5662273743844));
#19913=CARTESIAN_POINT('Ctrl Pts',(32.2888283700867,27.4496181106864,10.4701702229063));
#19914=CARTESIAN_POINT('',(31.353449269816,30.1531295040176,9.34999999998873));
#19915=CARTESIAN_POINT('Ctrl Pts',(31.353449269816,30.1531295040176,9.34999999998873));
#19916=CARTESIAN_POINT('Ctrl Pts',(31.2436844228239,29.972976337506,9.55399283498083));
#19917=CARTESIAN_POINT('Ctrl Pts',(31.1284362061875,29.797429949865,9.75864949418871));
#19918=CARTESIAN_POINT('Ctrl Pts',(31.0077399492351,29.6264965063431,9.96399986488537));
#19919=CARTESIAN_POINT('Ctrl Pts',(30.9129909412829,29.4923102887379,10.1252040678772));
#19920=CARTESIAN_POINT('Ctrl Pts',(30.8148836521484,29.3609674111789,10.2868360245795));
#19921=CARTESIAN_POINT('Ctrl Pts',(30.7134197505153,29.2324872694336,10.4489096280657));
#19922=CARTESIAN_POINT('',(28.9934992272715,32.4287989688053,9.34999999998873));
#19923=CARTESIAN_POINT('Origin',(0.,0.,9.34999999999998));
#19924=CARTESIAN_POINT('',(28.0536866918396,31.7653999649234,10.4701702229062));
#19925=CARTESIAN_POINT('Ctrl Pts',(28.0536866918396,31.7653999649233,10.4701702229062));
#19926=CARTESIAN_POINT('Ctrl Pts',(28.2152546247496,31.8950230533658,10.2660612053885));
#19927=CARTESIAN_POINT('Ctrl Pts',(28.3814435471357,32.0194461226571,10.0627475751645));
#19928=CARTESIAN_POINT('Ctrl Pts',(28.55221812893,32.1386630458038,9.86020040448756));
#19929=CARTESIAN_POINT('Ctrl Pts',(28.696059331436,32.239077904996,9.68959756483639));
#19930=CARTESIAN_POINT('Ctrl Pts',(28.8431545396022,32.3357987743744,9.51953800447141));
#19931=CARTESIAN_POINT('Ctrl Pts',(28.9934992272715,32.4287989688053,9.34999999998873));
#19932=CARTESIAN_POINT('',(26.240584724474,33.3059180634109,10.4489096280657));
#19933=CARTESIAN_POINT('Ctrl Pts',(26.2405847244741,33.3059180634109,10.4489096280657));
#19934=CARTESIAN_POINT('Ctrl Pts',(26.2959168974024,33.1368749590178,10.547449245225));
#19935=CARTESIAN_POINT('Ctrl Pts',(26.3800942293042,32.9680700585874,10.6271602259564));
#19936=CARTESIAN_POINT('Ctrl Pts',(26.6135971436297,32.6226154911154,10.7492445866574));
#19937=CARTESIAN_POINT('Ctrl Pts',(26.7680512262515,32.4512772340278,10.7838550844415));
#19938=CARTESIAN_POINT('Ctrl Pts',(27.1202393222333,32.1519466367896,10.7881210903218));
#19939=CARTESIAN_POINT('Ctrl Pts',(27.3146682909138,32.0267513044622,10.7577447440201));
#19940=CARTESIAN_POINT('Ctrl Pts',(27.6950355733207,31.8505366300097,10.6429386483201));
#19941=CARTESIAN_POINT('Ctrl Pts',(27.8764815899826,31.7937443484395,10.5662273743849));
#19942=CARTESIAN_POINT('Ctrl Pts',(28.0536866918396,31.7653999649233,10.4701702229062));
#19943=CARTESIAN_POINT('',(26.7430786153922,34.3082751850327,9.34999999998873));
#19944=CARTESIAN_POINT('Ctrl Pts',(26.7430786153922,34.3082751850326,9.34999999998873));
#19945=CARTESIAN_POINT('Ctrl Pts',(26.6600694850447,34.1143345515807,9.55399283494745));
#19946=CARTESIAN_POINT('Ctrl Pts',(26.5709771848617,33.9241734417676,9.75864949412165));
#19947=CARTESIAN_POINT('Ctrl Pts',(26.4758358071633,33.737802985976,9.96399986478445));
#19948=CARTESIAN_POINT('Ctrl Pts',(26.4011478973383,33.5914984008107,10.1252040678097));
#19949=CARTESIAN_POINT('Ctrl Pts',(26.3227312393107,33.4475302813474,10.2868360245456));
#19950=CARTESIAN_POINT('Ctrl Pts',(26.2405847244741,33.3059180634109,10.4489096280657));
#19951=CARTESIAN_POINT('',(24.0832879296691,36.2249257072756,9.34999999998873));
#19952=CARTESIAN_POINT('Origin',(0.,0.,9.34999999999998));
#19953=CARTESIAN_POINT('',(23.2474528526983,35.4345298797235,10.4701702229062));
#19954=CARTESIAN_POINT('Ctrl Pts',(23.2474528526983,35.4345298797235,10.4701702229062));
#19955=CARTESIAN_POINT('Ctrl Pts',(23.3889289681428,35.5858271062667,10.2660612053916));
#19956=CARTESIAN_POINT('Ctrl Pts',(23.5357190779377,35.7326348777259,10.0627475751705));
#19957=CARTESIAN_POINT('Ctrl Pts',(23.6877890835865,35.8749421014788,9.86020040449658));
#19958=CARTESIAN_POINT('Ctrl Pts',(23.8158756656088,35.9948056196646,9.68959756484237));
#19959=CARTESIAN_POINT('Ctrl Pts',(23.9477088417686,36.1114758408158,9.51953800447439));
#19960=CARTESIAN_POINT('Ctrl Pts',(24.0832879296691,36.2249257072756,9.34999999998873));
#19961=CARTESIAN_POINT('',(21.2335670650401,36.7013364119535,10.4489096280657));
#19962=CARTESIAN_POINT('Ctrl Pts',(21.2335670650401,36.7013364119535,10.4489096280657));
#19963=CARTESIAN_POINT('Ctrl Pts',(21.3123933782934,36.5418885118648,10.547449245225));
#19964=CARTESIAN_POINT('Ctrl Pts',(21.4197373484345,36.3867814853001,10.6271602259564));
#19965=CARTESIAN_POINT('Ctrl Pts',(21.7000268506762,36.0780740767091,10.7492445866574));
#19966=CARTESIAN_POINT('Ctrl Pts',(21.8772927897887,35.9304609038183,10.7838550844415));
#19967=CARTESIAN_POINT('Ctrl Pts',(22.2684953043029,35.6842986523823,10.7881210903218));
#19968=CARTESIAN_POINT('Ctrl Pts',(22.4787624198984,35.5880477552547,10.7577447440202));
#19969=CARTESIAN_POINT('Ctrl Pts',(22.8803360747108,35.4677586003877,10.6429386483201));
#19970=CARTESIAN_POINT('Ctrl Pts',(23.0680176169135,35.4373668428728,10.5662273743849));
#19971=CARTESIAN_POINT('Ctrl Pts',(23.2474528526983,35.4345298797235,10.4701702229062));
#19972=CARTESIAN_POINT('',(21.5882960010294,37.7650033201762,9.34999999998873));
#19973=CARTESIAN_POINT('Ctrl Pts',(21.5882960010294,37.7650033201762,9.34999999998873));
#19974=CARTESIAN_POINT('Ctrl Pts',(21.533732413815,37.5612232917399,9.55399283498049));
#19975=CARTESIAN_POINT('Ctrl Pts',(21.4726096923653,37.3603185915109,9.75864949418803));
#19976=CARTESIAN_POINT('Ctrl Pts',(21.4049599979712,37.1623050884238,9.96399986488434));
#19977=CARTESIAN_POINT('Ctrl Pts',(21.3518536167628,37.0068604752068,10.1252040678765));
#19978=CARTESIAN_POINT('Ctrl Pts',(21.2947239268954,36.8531978896416,10.2868360245791));
#19979=CARTESIAN_POINT('Ctrl Pts',(21.2335670650401,36.7013364119535,10.4489096280657));
#19980=CARTESIAN_POINT('',(18.682810340286,39.283617422405,9.34999999998873));
#19981=CARTESIAN_POINT('Origin',(0.,0.,9.34999999999998));
#19982=CARTESIAN_POINT('',(17.9679679135941,38.3823149509186,10.4701702229062));
#19983=CARTESIAN_POINT('Ctrl Pts',(17.9679679135941,38.3823149509186,10.4701702229062));
#19984=CARTESIAN_POINT('Ctrl Pts',(18.0864721658495,38.5522063403388,10.2660612053895));
#19985=CARTESIAN_POINT('Ctrl Pts',(18.2108752397294,38.7184102311011,10.0627475751664));
#19986=CARTESIAN_POINT('Ctrl Pts',(18.3411449624555,38.880910790768,9.8602004044904));
#19987=CARTESIAN_POINT('Ctrl Pts',(18.4508694505517,39.0177828923714,9.68959756483827));
#19988=CARTESIAN_POINT('Ctrl Pts',(18.5647568514102,39.1520273960384,9.51953800447235));
#19989=CARTESIAN_POINT('Ctrl Pts',(18.6828103402861,39.283617422405,9.34999999998874));
#19990=CARTESIAN_POINT('',(15.7942952127128,39.3496213890631,10.4489096280657));
#19991=CARTESIAN_POINT('Ctrl Pts',(15.7942952127128,39.3496213890631,10.4489096280657));
#19992=CARTESIAN_POINT('Ctrl Pts',(15.8950109898695,39.2030145927147,10.547449245225));
#19993=CARTESIAN_POINT('Ctrl Pts',(16.0233363845725,39.0647629717849,10.6271602259564));
#19994=CARTESIAN_POINT('Ctrl Pts',(16.3447065887528,38.7990871146753,10.7492445866574));
#19995=CARTESIAN_POINT('Ctrl Pts',(16.5411757610284,38.6782040045,10.7838550844415));
#19996=CARTESIAN_POINT('Ctrl Pts',(16.9634289390145,38.4902212524321,10.7881210903218));
#19997=CARTESIAN_POINT('Ctrl Pts',(17.1852537694118,38.4248741812051,10.7577447440202));
#19998=CARTESIAN_POINT('Ctrl Pts',(17.5998589150605,38.3629592862315,10.6429386483201));
#19999=CARTESIAN_POINT('Ctrl Pts',(17.7899553278336,38.3595867413122,10.5662273743849));
#20000=CARTESIAN_POINT('Ctrl Pts',(17.9679679135941,38.3823149509185,10.4701702229062));
#20001=CARTESIAN_POINT('',(15.9940379355904,40.4529448929973,9.34999999998873));
#20002=CARTESIAN_POINT('Ctrl Pts',(15.9940379355903,40.4529448929973,9.34999999998873));
#20003=CARTESIAN_POINT('Ctrl Pts',(15.9690306488096,40.2434738433319,9.55399283498242));
#20004=CARTESIAN_POINT('Ctrl Pts',(15.9371217884536,40.0359153930508,9.7586494941919));
#20005=CARTESIAN_POINT('Ctrl Pts',(15.8983409300729,39.8302898265943,9.96399986489017));
#20006=CARTESIAN_POINT('Ctrl Pts',(15.8678971702429,39.6688695893563,10.1252040678804));
#20007=CARTESIAN_POINT('Ctrl Pts',(15.8332174442578,39.5086406647769,10.2868360245811));
#20008=CARTESIAN_POINT('Ctrl Pts',(15.7942952127128,39.3496213890631,10.4489096280657));
#20009=CARTESIAN_POINT('',(12.9020046091508,41.5426079714121,9.34999999998873));
#20010=CARTESIAN_POINT('Origin',(0.,0.,9.34999999999998));
#20011=CARTESIAN_POINT('',(12.3227069631098,40.548746775169,10.4701702229062));
#20012=CARTESIAN_POINT('Ctrl Pts',(12.3227069631098,40.548746775169,10.4701702229062));
#20013=CARTESIAN_POINT('Ctrl Pts',(12.4158269473365,40.7337738287018,10.2660612053903));
#20014=CARTESIAN_POINT('Ctrl Pts',(12.5153104974641,40.9159904068415,10.0627475751681));
#20015=CARTESIAN_POINT('Ctrl Pts',(12.6211280213774,41.0953762596384,9.86020040449293));
#20016=CARTESIAN_POINT('Ctrl Pts',(12.710256741391,41.2464706233796,9.68959756483996));
#20017=CARTESIAN_POINT('Ctrl Pts',(12.8038799478929,41.3955565785991,9.51953800447319));
#20018=CARTESIAN_POINT('Ctrl Pts',(12.9020046091508,41.5426079714121,9.34999999998873));
#20019=CARTESIAN_POINT('',(10.033497056841,41.196861549629,10.4489096280657));
#20020=CARTESIAN_POINT('Ctrl Pts',(10.033497056841,41.196861549629,10.4489096280657));
#20021=CARTESIAN_POINT('Ctrl Pts',(10.1540520151185,41.0660803486155,10.547449245225));
#20022=CARTESIAN_POINT('Ctrl Pts',(10.300746499407,40.9474985376379,10.6271602259564));
#20023=CARTESIAN_POINT('Ctrl Pts',(10.6566552349239,40.7302626263144,10.7492445866574));
#20024=CARTESIAN_POINT('Ctrl Pts',(10.8683280945855,40.6385704103798,10.7838550844415));
#20025=CARTESIAN_POINT('Ctrl Pts',(11.3130360790173,40.5125939444147,10.7881210903218));
#20026=CARTESIAN_POINT('Ctrl Pts',(11.5419029103594,40.4794809770131,10.7577447440201));
#20027=CARTESIAN_POINT('Ctrl Pts',(11.9610993817015,40.4772007506466,10.6429386483201));
#20028=CARTESIAN_POINT('Ctrl Pts',(12.1497408502737,40.500916073612,10.5662273743849));
#20029=CARTESIAN_POINT('Ctrl Pts',(12.3227069631098,40.548746775169,10.4701702229062));
#20030=CARTESIAN_POINT('',(10.0741873807793,42.3173811644569,9.34999999998873));
#20031=CARTESIAN_POINT('Ctrl Pts',(10.0741873807793,42.3173811644569,9.34999999998873));
#20032=CARTESIAN_POINT('Ctrl Pts',(10.0792454706757,42.1064833201057,9.55399283494883));
#20033=CARTESIAN_POINT('Ctrl Pts',(10.0772000437949,41.8964964113072,9.75864949412443));
#20034=CARTESIAN_POINT('Ctrl Pts',(10.068077487874,41.6874447250753,9.96399986478863));
#20035=CARTESIAN_POINT('Ctrl Pts',(10.0609160965797,41.5233349143123,10.1252040678125));
#20036=CARTESIAN_POINT('Ctrl Pts',(10.0493923136879,41.3598014495247,10.286836024547));
#20037=CARTESIAN_POINT('Ctrl Pts',(10.033497056841,41.196861549629,10.4489096280657));
#20038=CARTESIAN_POINT('',(6.85855127048205,42.9559108211099,9.34999999998873));
#20039=CARTESIAN_POINT('Origin',(0.,0.,9.34999999999998));
#20040=CARTESIAN_POINT('',(6.42659123460896,41.8897230480066,10.4701702229062));
#20041=CARTESIAN_POINT('Ctrl Pts',(6.42659123460897,41.8897230480066,10.4701702229062));
#20042=CARTESIAN_POINT('Ctrl Pts',(6.49243129646502,42.0861191484182,10.2660612053887));
#20043=CARTESIAN_POINT('Ctrl Pts',(6.56497012464767,42.2806390098759,10.0627475751649));
#20044=CARTESIAN_POINT('Ctrl Pts',(6.64418131011524,42.4732583771481,9.86020040448811));
#20045=CARTESIAN_POINT('Ctrl Pts',(6.71089985833178,42.6354991574991,9.68959756483675));
#20046=CARTESIAN_POINT('Ctrl Pts',(6.78235297197845,42.7963916041491,9.51953800447159));
#20047=CARTESIAN_POINT('Ctrl Pts',(6.85855127048204,42.95591082111,9.34999999998873));
#20048=CARTESIAN_POINT('',(4.06844583510807,42.2054524109828,10.4489096280657));
#20049=CARTESIAN_POINT('Ctrl Pts',(4.06844583510807,42.2054524109828,10.4489096280657));
#20050=CARTESIAN_POINT('Ctrl Pts',(4.2063858232076,42.0931591334149,10.547449245225));
#20051=CARTESIAN_POINT('Ctrl Pts',(4.36846312041344,41.9966611160993,10.6271602259564));
#20052=CARTESIAN_POINT('Ctrl Pts',(4.751665111768,41.83228744726,10.7492445866574));
#20053=CARTESIAN_POINT('Ctrl Pts',(4.97423260980699,41.7716527146639,10.7838550844415));
#20054=CARTESIAN_POINT('Ctrl Pts',(5.43234242855323,41.7102470523625,10.7881210903218));
#20055=CARTESIAN_POINT('Ctrl Pts',(5.66359219215152,41.7100422733126,10.7577447440201));
#20056=CARTESIAN_POINT('Ctrl Pts',(6.07884635789332,41.7674431343865,10.6429386483201));
#20057=CARTESIAN_POINT('Ctrl Pts',(6.26219268596163,41.8177635496503,10.5662273743849));
#20058=CARTESIAN_POINT('Ctrl Pts',(6.42659123460897,41.8897230480066,10.4701702229062));
#20059=CARTESIAN_POINT('',(3.94925542245304,43.3203575886581,9.34999999998873));
#20060=CARTESIAN_POINT('Ctrl Pts',(3.94925542245304,43.3203575886581,9.34999999998873));
#20061=CARTESIAN_POINT('Ctrl Pts',(3.98427592090395,43.112326221486,9.55399283498063));
#20062=CARTESIAN_POINT('Ctrl Pts',(4.01213556648794,42.9041855820147,9.75864949418831));
#20063=CARTESIAN_POINT('Ctrl Pts',(4.03285702195055,42.6959634654179,9.96399986488476));
#20064=CARTESIAN_POINT('Ctrl Pts',(4.04912378446653,42.5325048836902,10.1252040678768));
#20065=CARTESIAN_POINT('Ctrl Pts',(4.06099053565887,42.3689959485124,10.2868360245792));
#20066=CARTESIAN_POINT('Ctrl Pts',(4.06844583510807,42.2054524109828,10.4489096280657));
#20067=CARTESIAN_POINT('',(0.675477606374581,43.4947552011075,9.34999999998873));
#20068=CARTESIAN_POINT('Origin',(0.,0.,9.34999999999998));
#20069=CARTESIAN_POINT('',(0.399648641329917,42.3779453595728,10.4701702229062));
#20070=CARTESIAN_POINT('Ctrl Pts',(0.399648641329911,42.3779453595728,10.4701702229062));
#20071=CARTESIAN_POINT('Ctrl Pts',(0.436868467021998,42.5817124486157,10.2660612053899));
#20072=CARTESIAN_POINT('Ctrl Pts',(0.48098589190151,42.7845757299584,10.0627475751672));
#20073=CARTESIAN_POINT('Ctrl Pts',(0.531978227612102,42.9865074368541,9.86020040449165));
#20074=CARTESIAN_POINT('Ctrl Pts',(0.574928406791237,43.1565918793934,9.6895975648391));
#20075=CARTESIAN_POINT('Ctrl Pts',(0.622756848243766,43.3260155112382,9.51953800447277));
#20076=CARTESIAN_POINT('Ctrl Pts',(0.675477606374568,43.4947552011075,9.34999999998873));
#20077=CARTESIAN_POINT('',(-1.97942721139903,42.3548619717231,10.4489096280657));
#20078=CARTESIAN_POINT('Ctrl Pts',(-1.97942721139904,42.3548619717231,10.4489096280657));
#20079=CARTESIAN_POINT('Ctrl Pts',(-1.82691025384904,42.2633425849051,10.547449245225));
#20080=CARTESIAN_POINT('Ctrl Pts',(-1.65274957010463,42.1908927826067,10.6271602259564));
#20081=CARTESIAN_POINT('Ctrl Pts',(-1.25005521039323,42.0827275301346,10.7492445866574));
#20082=CARTESIAN_POINT('Ctrl Pts',(-1.02112390640528,42.0543846291766,10.7838550844415));
#20083=CARTESIAN_POINT('Ctrl Pts',(-0.558938048174559,42.058799812744,10.7881210903218));
#20084=CARTESIAN_POINT('Ctrl Pts',(-0.330012930637709,42.0915073907568,
10.7577447440201));
#20085=CARTESIAN_POINT('Ctrl Pts',(0.072845552183429,42.2074208232701,10.6429386483201));
#20086=CARTESIAN_POINT('Ctrl Pts',(0.247164337235477,42.2833219522895,10.5662273743849));
#20087=CARTESIAN_POINT('Ctrl Pts',(0.399648641329905,42.3779453595727,10.4701702229062));
#20088=CARTESIAN_POINT('',(-2.25607198756253,43.4414564579495,9.34999999998873));
#20089=CARTESIAN_POINT('Ctrl Pts',(-2.25607198756253,43.4414564579494,9.34999999998873));
#20090=CARTESIAN_POINT('Ctrl Pts',(-2.19180199691532,43.2405264867111,9.55399283498151));
#20091=CARTESIAN_POINT('Ctrl Pts',(-2.13460442090842,43.0384692597904,9.75864949419006));
#20092=CARTESIAN_POINT('Ctrl Pts',(-2.084460783136,42.8353155146912,9.9639998648874));
#20093=CARTESIAN_POINT('Ctrl Pts',(-2.04509701118501,42.6758357073152,10.1252040678786));
#20094=CARTESIAN_POINT('Ctrl Pts',(-2.0100812987435,42.5156798721146,10.2868360245801));
#20095=CARTESIAN_POINT('Ctrl Pts',(-1.97942721139904,42.3548619717231,10.4489096280657));
#20096=CARTESIAN_POINT('',(-5.52134683388147,43.1481717937269,9.34999999998873));
#20097=CARTESIAN_POINT('Origin',(0.,0.,9.34999999999998));
#20098=CARTESIAN_POINT('',(-5.63542964579448,42.0034749115207,10.4701702229062));
#20099=CARTESIAN_POINT('Ctrl Pts',(-5.63542964579449,42.0034749115207,10.4701702229062));
#20100=CARTESIAN_POINT('Ctrl Pts',(-5.62758774458395,42.2104648788792,10.2660612053897));
#20101=CARTESIAN_POINT('Ctrl Pts',(-5.61278982655349,42.4175418687094,10.0627475751669));
#20102=CARTESIAN_POINT('Ctrl Pts',(-5.59105439750463,42.6246751680003,9.86020040449119));
#20103=CARTESIAN_POINT('Ctrl Pts',(-5.57274692915329,42.7991408439597,9.6895975648388));
#20104=CARTESIAN_POINT('Ctrl Pts',(-5.54951680903751,42.9736466844311,9.51953800447262));
#20105=CARTESIAN_POINT('Ctrl Pts',(-5.52134683388148,43.1481717937269,9.34999999998873));
#20106=CARTESIAN_POINT('',(-7.98700482807813,41.6420486840549,10.4489096280657));
#20107=CARTESIAN_POINT('Ctrl Pts',(-7.98700482807813,41.6420486840549,10.4489096280657));
#20108=CARTESIAN_POINT('Ctrl Pts',(-7.82301570651087,41.5731662587824,10.547449245225));
#20109=CARTESIAN_POINT('Ctrl Pts',(-7.64031704551097,41.526239540548,10.6271602259564));
#20110=CARTESIAN_POINT('Ctrl Pts',(-7.22632801333171,41.4764846370605,10.7492445866574));
#20111=CARTESIAN_POINT('Ctrl Pts',(-6.99569328456065,41.4810105474699,10.7838550844415));
#20112=CARTESIAN_POINT('Ctrl Pts',(-6.53884015808512,41.5511566965011,10.7881210903218));
#20113=CARTESIAN_POINT('Ctrl Pts',(-6.31689994183723,41.6161107996091,10.7577447440201));
#20114=CARTESIAN_POINT('Ctrl Pts',(-5.93463817889906,41.7881771403424,10.6429386483201));
#20115=CARTESIAN_POINT('Ctrl Pts',(-5.77289556463307,41.8881138550115,10.5662273743849));
#20116=CARTESIAN_POINT('Ctrl Pts',(-5.6354296457945,42.0034749115207,10.4701702229062));
#20117=CARTESIAN_POINT('',(-8.41547227788506,42.6782125485725,9.34999999998873));
#20118=CARTESIAN_POINT('Ctrl Pts',(-8.41547227788505,42.6782125485725,9.34999999998873));
#20119=CARTESIAN_POINT('Ctrl Pts',(-8.32326114672774,42.4884743280816,9.55399283494648));
#20120=CARTESIAN_POINT('Ctrl Pts',(-8.23789001801484,42.2966138162009,9.75864949411971));
#20121=CARTESIAN_POINT('Ctrl Pts',(-8.15934497780653,42.1026640670373,9.96399986478153));
#20122=CARTESIAN_POINT('Ctrl Pts',(-8.09768552928625,41.9504095829559,10.1252040678078));
#20123=CARTESIAN_POINT('Ctrl Pts',(-8.04023367451032,41.7968671586518,10.2868360245446));
#20124=CARTESIAN_POINT('Ctrl Pts',(-7.98700482807813,41.6420486840549,10.4489096280657));
#20125=CARTESIAN_POINT('',(-11.6057725748495,41.9232160376784,9.34999999998873));
#20126=CARTESIAN_POINT('Origin',(0.,0.,9.34999999999998));
#20127=CARTESIAN_POINT('',(-11.5557868365679,40.7739348422893,10.4701702229062));
#20128=CARTESIAN_POINT('Ctrl Pts',(-11.5557868365679,40.7739348422893,10.4701702229062));
#20129=CARTESIAN_POINT('Ctrl Pts',(-11.5774824983335,40.9799339691383,10.266061205389));
#20130=CARTESIAN_POINT('Ctrl Pts',(-11.5923053300896,41.1870091771045,10.0627475751654));
#20131=CARTESIAN_POINT('Ctrl Pts',(-11.6002692783581,41.3951274321408,9.86020040448896));
#20132=CARTESIAN_POINT('Ctrl Pts',(-11.6069772080958,41.5704227234745,9.68959756483732));
#20133=CARTESIAN_POINT('Ctrl Pts',(-11.6088183075721,41.746458336893,9.51953800447188));
#20134=CARTESIAN_POINT('Ctrl Pts',(-11.6057725748495,41.9232160376784,9.34999999998873));
#20135=CARTESIAN_POINT('',(-13.8319900590778,40.0815233709313,10.4489096280657));
#20136=CARTESIAN_POINT('Ctrl Pts',(-13.8319900590778,40.0815233709313,10.4489096280657));
#20137=CARTESIAN_POINT('Ctrl Pts',(-13.6598671191028,40.0366801547422,10.5474492452249));
#20138=CARTESIAN_POINT('Ctrl Pts',(-13.4723496987259,40.0162318132297,10.6271602259564));
#20139=CARTESIAN_POINT('Ctrl Pts',(-13.0554936169282,40.0259001250806,10.7492445866574));
#20140=CARTESIAN_POINT('Ctrl Pts',(-12.8278505213562,40.0632027123731,10.7838550844415));
#20141=CARTESIAN_POINT('Ctrl Pts',(-12.3856303388352,40.1976518535586,10.7881210903218));
#20142=CARTESIAN_POINT('Ctrl Pts',(-12.1751930866564,40.2935302035347,10.7577447440201));
#20143=CARTESIAN_POINT('Ctrl Pts',(-11.8213097907427,40.5182466779891,10.6429386483201));
#20144=CARTESIAN_POINT('Ctrl Pts',(-11.6754359604621,40.6401845549909,10.5662273743849));
#20145=CARTESIAN_POINT('Ctrl Pts',(-11.5557868365679,40.7739348422893,10.4701702229062));
#20146=CARTESIAN_POINT('',(-14.4035578208482,41.0461633055084,9.34999999998873));
#20147=CARTESIAN_POINT('Ctrl Pts',(-14.4035578208482,41.0461633055084,9.34999999998873));
#20148=CARTESIAN_POINT('Ctrl Pts',(-14.2852827018843,40.8714793587385,9.55399283494804));
#20149=CARTESIAN_POINT('Ctrl Pts',(-14.1734759304465,40.6937212886033,9.75864949412283));
#20150=CARTESIAN_POINT('Ctrl Pts',(-14.0681284383089,40.5129237929268,9.96399986478622));
#20151=CARTESIAN_POINT('Ctrl Pts',(-13.9854285217914,40.370994094406,10.1252040678109));
#20152=CARTESIAN_POINT('Ctrl Pts',(-13.9067100787762,40.2271907620138,10.2868360245461));
#20153=CARTESIAN_POINT('Ctrl Pts',(-13.8319900590778,40.0815233709313,10.4489096280657));
#20154=CARTESIAN_POINT('',(-17.4539382544779,39.8448244996744,9.34999999998873));
#20155=CARTESIAN_POINT('Origin',(0.,0.,9.34999999999998));
#20156=CARTESIAN_POINT('',(-17.2409015314889,38.7143550419919,10.4701702229111));
#20157=CARTESIAN_POINT('Ctrl Pts',(-17.2409015314889,38.7143550419919,10.4701702229111));
#20158=CARTESIAN_POINT('Ctrl Pts',(-17.2916930951406,38.9151697802362,10.2660612053116));
#20159=CARTESIAN_POINT('Ctrl Pts',(-17.3358349265883,39.1180277523379,10.0627475750077));
#20160=CARTESIAN_POINT('Ctrl Pts',(-17.3733361291629,39.3228942756909,9.86020040425219));
#20161=CARTESIAN_POINT('Ctrl Pts',(-17.4049229028648,39.4954506756989,9.68959756467966));
#20162=CARTESIAN_POINT('Ctrl Pts',(-17.4317977424424,39.669432484541,9.51953800439327));
#20163=CARTESIAN_POINT('Ctrl Pts',(-17.4539382544779,39.8448244996744,9.34999999998873));
#20164=CARTESIAN_POINT('',(-19.3953958606401,37.7050538275442,10.4489096280657));
#20165=CARTESIAN_POINT('Ctrl Pts',(-19.3953958606401,37.7050538275442,10.4489096280657));
#20166=CARTESIAN_POINT('Ctrl Pts',(-19.2186430289537,37.685162699003,10.547449245225));
#20167=CARTESIAN_POINT('Ctrl Pts',(-19.0301241631232,37.6916090034774,10.6271602259564));
#20168=CARTESIAN_POINT('Ctrl Pts',(-18.6188870194189,37.7605037117184,10.7492445866574));
#20169=CARTESIAN_POINT('Ctrl Pts',(-18.3988697140032,37.8298236027885,10.7838550844415));
#20170=CARTESIAN_POINT('Ctrl Pts',(-17.9802848030952,38.025838739333,10.7881210903218));
#20171=CARTESIAN_POINT('Ctrl Pts',(-17.7856344105889,38.150689529462,10.7577447440202));
#20172=CARTESIAN_POINT('Ctrl Pts',(-17.4673336250879,38.4234815582477,10.6429386483196));
#20173=CARTESIAN_POINT('Ctrl Pts',(-17.3402981493126,38.5649382940457,10.5662273743844));
#20174=CARTESIAN_POINT('Ctrl Pts',(-17.2409015314864,38.7143550419871,10.4701702229063));
#20175=CARTESIAN_POINT('',(-20.0984284630096,38.5785325449046,9.34999999998873));
#20176=CARTESIAN_POINT('Ctrl Pts',(-20.0984284630096,38.5785325449046,9.34999999998873));
#20177=CARTESIAN_POINT('Ctrl Pts',(-19.9564970965613,38.4224589332409,9.55399283498155));
#20178=CARTESIAN_POINT('Ctrl Pts',(-19.8205307458203,38.2624219465217,9.75864949419015));
#20179=CARTESIAN_POINT('Ctrl Pts',(-19.6905253728772,38.0984572199405,9.96399986488752));
#20180=CARTESIAN_POINT('Ctrl Pts',(-19.5884685201982,37.9697415863752,10.1252040678787));
#20181=CARTESIAN_POINT('Ctrl Pts',(-19.4900859694591,37.8386047670733,10.2868360245802));
#20182=CARTESIAN_POINT('Ctrl Pts',(-19.3953958606401,37.7050538275442,10.4489096280657));
#20183=CARTESIAN_POINT('',(-22.9467920842467,36.9553072378425,9.34999999998873));
#20184=CARTESIAN_POINT('Origin',(0.,0.,9.34999999999998));
#20185=CARTESIAN_POINT('',(-22.5750411898779,35.8666626160111,10.4701702229062));
#20186=CARTESIAN_POINT('Ctrl Pts',(-22.5750411898779,35.8666626160111,10.4701702229062));
#20187=CARTESIAN_POINT('Ctrl Pts',(-22.6538946856141,36.0582049565317,10.2660612053891));
#20188=CARTESIAN_POINT('Ctrl Pts',(-22.7264569163319,36.2527160892947,10.0627475751656));
#20189=CARTESIAN_POINT('Ctrl Pts',(-22.7927319568545,36.4501603891746,9.8602004044892));
#20190=CARTESIAN_POINT('Ctrl Pts',(-22.848554558935,36.616465147321,9.68959756483748));
#20191=CARTESIAN_POINT('Ctrl Pts',(-22.8999160444098,36.7848513838393,9.51953800447196));
#20192=CARTESIAN_POINT('Ctrl Pts',(-22.9467920842467,36.9553072378425,9.34999999998873));
#20193=CARTESIAN_POINT('',(-24.5639673341827,34.5610181206246,10.4489096280657));
#20194=CARTESIAN_POINT('Ctrl Pts',(-24.5639673341828,34.5610181206246,10.4489096280657));
#20195=CARTESIAN_POINT('Ctrl Pts',(-24.3861827887249,34.5664840057471,10.547449245225));
#20196=CARTESIAN_POINT('Ctrl Pts',(-24.2005001779055,34.5996937280389,10.6271602259564));
#20197=CARTESIAN_POINT('Ctrl Pts',(-23.8032535746302,34.7264123350863,10.7492445866574));
#20198=CARTESIAN_POINT('Ctrl Pts',(-23.5953409772317,34.8263383768539,10.7838550844415));
#20199=CARTESIAN_POINT('Ctrl Pts',(-23.2089125196236,35.0799292058384,10.7881210903218));
#20200=CARTESIAN_POINT('Ctrl Pts',(-23.0340115074558,35.2312108340732,10.7577447440201));
#20201=CARTESIAN_POINT('Ctrl Pts',(-22.7577729184596,35.5465251581489,10.6429386483201));
#20202=CARTESIAN_POINT('Ctrl Pts',(-22.6521618731346,35.7046211015308,10.5662273743849));
#20203=CARTESIAN_POINT('Ctrl Pts',(-22.5750411898779,35.8666626160111,10.4701702229062));
#20204=CARTESIAN_POINT('',(-25.3841530607458,35.3255541129876,9.34999999998873));
#20205=CARTESIAN_POINT('Ctrl Pts',(-25.3841530607458,35.3255541129876,9.34999999998873));
#20206=CARTESIAN_POINT('Ctrl Pts',(-25.2214547601583,35.191268045114,9.55399283498005));
#20207=CARTESIAN_POINT('Ctrl Pts',(-25.064096712939,35.0522100333827,9.75864949418713));
#20208=CARTESIAN_POINT('Ctrl Pts',(-24.9120799936953,34.9084159249267,9.96399986488299));
#20209=CARTESIAN_POINT('Ctrl Pts',(-24.7927437880474,34.7955346354012,10.1252040678756));
#20210=CARTESIAN_POINT('Ctrl Pts',(-24.6766999145872,34.6797338966323,10.2868360245787));
#20211=CARTESIAN_POINT('Ctrl Pts',(-24.5639673341828,34.5610181206246,10.4489096280657));
#20212=CARTESIAN_POINT('',(-27.9725154002642,33.3134864909539,9.34999999998873));
#20213=CARTESIAN_POINT('Origin',(0.,0.,9.34999999999998));
#20214=CARTESIAN_POINT('',(-27.4496181106865,32.2888283700868,10.4701702229062));
#20215=CARTESIAN_POINT('Ctrl Pts',(-27.4496181106865,32.2888283700868,10.4701702229062));
#20216=CARTESIAN_POINT('Ctrl Pts',(-27.5549283087472,32.4671990632694,10.2660612053888));
#20217=CARTESIAN_POINT('Ctrl Pts',(-27.654433780984,32.6494036710336,10.0627475751651));
#20218=CARTESIAN_POINT('Ctrl Pts',(-27.7481334907604,32.8354063509586,9.86020040448855));
#20219=CARTESIAN_POINT('Ctrl Pts',(-27.8270555340008,32.9920739818714,9.68959756483705));
#20220=CARTESIAN_POINT('Ctrl Pts',(-27.9018580936281,33.1514367877958,9.51953800447174));
#20221=CARTESIAN_POINT('Ctrl Pts',(-27.9725154002642,33.3134864909539,9.34999999998874));
#20222=CARTESIAN_POINT('',(-29.2324872694337,30.7134197505152,10.4489096280657));
#20223=CARTESIAN_POINT('Ctrl Pts',(-29.2324872694337,30.7134197505152,10.4489096280657));
#20224=CARTESIAN_POINT('Ctrl Pts',(-29.0572901908617,30.7441313796427,10.547449245225));
#20225=CARTESIAN_POINT('Ctrl Pts',(-28.8782237975453,30.8034284655749,10.6271602259564));
#20226=CARTESIAN_POINT('Ctrl Pts',(-28.5030545299772,30.9853913460154,10.7492445866574));
#20227=CARTESIAN_POINT('Ctrl Pts',(-28.3114791415084,31.113889332433,10.7838550844415));
#20228=CARTESIAN_POINT('Ctrl Pts',(-27.9650737062295,31.4198934758749,10.7881210903218));
#20229=CARTESIAN_POINT('Ctrl Pts',(-27.8134825546351,31.5945262845249,10.7577447440201));
#20230=CARTESIAN_POINT('Ctrl Pts',(-27.5849295832077,31.9459440135451,10.6429386483201));
#20231=CARTESIAN_POINT('Ctrl Pts',(-27.5028929046597,32.1174607870142,10.5662273743849));
#20232=CARTESIAN_POINT('Ctrl Pts',(-27.4496181106865,32.2888283700868,10.4701702229062));
#20233=CARTESIAN_POINT('',(-30.1531295040177,31.3534492698159,9.34999999998873));
#20234=CARTESIAN_POINT('Ctrl Pts',(-30.1531295040177,31.3534492698159,9.34999999998873));
#20235=CARTESIAN_POINT('Ctrl Pts',(-29.9729763375347,31.2436844228412,9.5539928349485));
#20236=CARTESIAN_POINT('Ctrl Pts',(-29.7974299499209,31.128436206224,9.75864949412376));
#20237=CARTESIAN_POINT('Ctrl Pts',(-29.6264965064245,31.0077399492924,9.96399986478763));
#20238=CARTESIAN_POINT('Ctrl Pts',(-29.4923102887911,30.9129909413225,10.1252040678118));
#20239=CARTESIAN_POINT('Ctrl Pts',(-29.360967411205,30.8148836521688,10.2868360245466));
#20240=CARTESIAN_POINT('Ctrl Pts',(-29.2324872694337,30.7134197505152,10.4489096280657));
#20241=CARTESIAN_POINT('',(-32.4287989688054,28.9934992272714,9.34999999998873));
#20242=CARTESIAN_POINT('Origin',(0.,0.,9.34999999999998));
#20243=CARTESIAN_POINT('',(-31.7653999649278,28.0536866918426,10.4701702229111));
#20244=CARTESIAN_POINT('Ctrl Pts',(-31.7653999649278,28.0536866918426,10.4701702229111));
#20245=CARTESIAN_POINT('Ctrl Pts',(-31.8950230534163,28.2152546248113,10.2660612053145));
#20246=CARTESIAN_POINT('Ctrl Pts',(-32.0194461227511,28.3814435472605,10.0627475750136));
#20247=CARTESIAN_POINT('Ctrl Pts',(-32.138663045938,28.5522181291217,9.86020040426097));
#20248=CARTESIAN_POINT('Ctrl Pts',(-32.239077905082,28.6960593315664,9.68959756468549));
#20249=CARTESIAN_POINT('Ctrl Pts',(-32.3357987744158,28.8431545396688,9.51953800439617));
#20250=CARTESIAN_POINT('Ctrl Pts',(-32.4287989688055,28.9934992272714,9.34999999998873));
#20251=CARTESIAN_POINT('',(-33.305918063411,26.2405847244739,10.4489096280657));
#20252=CARTESIAN_POINT('Ctrl Pts',(-33.305918063411,26.2405847244739,10.4489096280657));
#20253=CARTESIAN_POINT('Ctrl Pts',(-33.1368749590179,26.2959168974023,10.5474492452249));
#20254=CARTESIAN_POINT('Ctrl Pts',(-32.9680700585876,26.380094229304,10.6271602259563));
#20255=CARTESIAN_POINT('Ctrl Pts',(-32.6226154911156,26.6135971436295,10.7492445866574));
#20256=CARTESIAN_POINT('Ctrl Pts',(-32.451277234028,26.7680512262512,10.7838550844415));
#20257=CARTESIAN_POINT('Ctrl Pts',(-32.1519466367897,27.1202393222332,10.7881210903218));
#20258=CARTESIAN_POINT('Ctrl Pts',(-32.0267513044624,27.3146682909137,10.7577447440202));
#20259=CARTESIAN_POINT('Ctrl Pts',(-31.850536630009,27.6950355733222,10.6429386483196));
#20260=CARTESIAN_POINT('Ctrl Pts',(-31.7937443484395,27.8764815899834,10.5662273743844));
#20261=CARTESIAN_POINT('Ctrl Pts',(-31.7653999649235,28.0536866918393,10.4701702229063));
#20262=CARTESIAN_POINT('',(-34.3082751850328,26.7430786153922,9.34999999998873));
#20263=CARTESIAN_POINT('Ctrl Pts',(-34.3082751850328,26.7430786153922,9.34999999998873));
#20264=CARTESIAN_POINT('Ctrl Pts',(-34.1143345515816,26.660069485045,9.55399283494663));
#20265=CARTESIAN_POINT('Ctrl Pts',(-33.9241734417693,26.5709771848624,9.75864949412001));
#20266=CARTESIAN_POINT('Ctrl Pts',(-33.7378029859783,26.4758358071644,9.96399986478199));
#20267=CARTESIAN_POINT('Ctrl Pts',(-33.5914984008123,26.401147897339,10.1252040678081));
#20268=CARTESIAN_POINT('Ctrl Pts',(-33.4475302813482,26.3227312393111,10.2868360245447));
#20269=CARTESIAN_POINT('Ctrl Pts',(-33.305918063411,26.2405847244739,10.4489096280657));
#20270=CARTESIAN_POINT('',(-36.2249257072757,24.083287929669,9.34999999998873));
#20271=CARTESIAN_POINT('Origin',(0.,0.,9.34999999999998));
#20272=CARTESIAN_POINT('',(-35.4345298797236,23.2474528526982,10.4701702229062));
#20273=CARTESIAN_POINT('Ctrl Pts',(-35.4345298797236,23.2474528526982,10.4701702229062));
#20274=CARTESIAN_POINT('Ctrl Pts',(-35.585827106268,23.3889289681438,10.2660612053899));
#20275=CARTESIAN_POINT('Ctrl Pts',(-35.7326348777284,23.5357190779399,10.0627475751672));
#20276=CARTESIAN_POINT('Ctrl Pts',(-35.8749421014824,23.68778908359,9.86020040449166));
#20277=CARTESIAN_POINT('Ctrl Pts',(-35.994805619667,23.8158756656112,9.68959756483911));
#20278=CARTESIAN_POINT('Ctrl Pts',(-36.111475840817,23.9477088417698,9.51953800447277));
#20279=CARTESIAN_POINT('Ctrl Pts',(-36.2249257072757,24.083287929669,9.34999999998873));
#20280=CARTESIAN_POINT('',(-36.7013364119536,21.2335670650399,10.4489096280657));
#20281=CARTESIAN_POINT('Ctrl Pts',(-36.7013364119536,21.2335670650399,10.4489096280657));
#20282=CARTESIAN_POINT('Ctrl Pts',(-36.5418885288437,21.3123933698994,10.547449234732));
#20283=CARTESIAN_POINT('Ctrl Pts',(-36.3867815182115,21.4197373256356,10.6271602090589));
#20284=CARTESIAN_POINT('Ctrl Pts',(-36.0780741043061,21.7000268175682,10.7492445801565));
#20285=CARTESIAN_POINT('Ctrl Pts',(-35.9304609153724,21.8772927714269,10.7838550842413));
#20286=CARTESIAN_POINT('Ctrl Pts',(-35.6842986623997,22.2684952883833,10.7881210901482));
#20287=CARTESIAN_POINT('Ctrl Pts',(-35.5880477708339,22.4787623858216,10.7577447489718));
#20288=CARTESIAN_POINT('Ctrl Pts',(-35.4677586059891,22.8803360402155,10.6429386624017));
#20289=CARTESIAN_POINT('Ctrl Pts',(-35.4373668431344,23.0680176003667,10.5662273832428));
#20290=CARTESIAN_POINT('Ctrl Pts',(-35.4345298797236,23.2474528526982,10.4701702229062));
#20291=CARTESIAN_POINT('',(-37.7650033201763,21.5882960010293,9.34999999998873));
#20292=CARTESIAN_POINT('Ctrl Pts',(-37.7650033201763,21.5882960010293,9.34999999998873));
#20293=CARTESIAN_POINT('Ctrl Pts',(-37.5612232917734,21.5337324138239,9.55399283494698));
#20294=CARTESIAN_POINT('Ctrl Pts',(-37.3603185915771,21.4726096923853,9.75864949412072));
#20295=CARTESIAN_POINT('Ctrl Pts',(-37.1623050885215,21.4049599980044,9.96399986478304));
#20296=CARTESIAN_POINT('Ctrl Pts',(-37.0068604752713,21.3518536167866,10.1252040678088));
#20297=CARTESIAN_POINT('Ctrl Pts',(-36.8531978896736,21.2947239269081,10.2868360245451));
#20298=CARTESIAN_POINT('Ctrl Pts',(-36.7013364119536,21.2335670650399,10.4489096280657));
#20299=CARTESIAN_POINT('',(-39.2836174224051,18.6828103402859,9.34999999998873));
#20300=CARTESIAN_POINT('Origin',(0.,0.,9.34999999999998));
#20301=CARTESIAN_POINT('',(-38.3823149509186,17.967967913594,10.4701702229062));
#20302=CARTESIAN_POINT('Ctrl Pts',(-38.3823149509186,17.967967913594,10.4701702229062));
#20303=CARTESIAN_POINT('Ctrl Pts',(-38.5522063403375,18.0864721658485,10.2660612053911));
#20304=CARTESIAN_POINT('Ctrl Pts',(-38.7184102310986,18.2108752397274,10.0627475751696));
#20305=CARTESIAN_POINT('Ctrl Pts',(-38.8809107907643,18.3411449624523,9.86020040449518));
#20306=CARTESIAN_POINT('Ctrl Pts',(-39.017782892369,18.4508694505494,9.68959756484145));
#20307=CARTESIAN_POINT('Ctrl Pts',(-39.1520273960372,18.564756851409,9.51953800447394));
#20308=CARTESIAN_POINT('Ctrl Pts',(-39.2836174224051,18.6828103402859,9.34999999998873));
#20309=CARTESIAN_POINT('',(-39.3496213890632,15.7942952127127,10.4489096280657));
#20310=CARTESIAN_POINT('Ctrl Pts',(-39.3496213890632,15.7942952127127,10.4489096280657));
#20311=CARTESIAN_POINT('Ctrl Pts',(-39.2030145927148,15.8950109898694,10.547449245225));
#20312=CARTESIAN_POINT('Ctrl Pts',(-39.0647629717849,16.0233363845724,10.6271602259564));
#20313=CARTESIAN_POINT('Ctrl Pts',(-38.7990871146753,16.3447065887526,10.7492445866574));
#20314=CARTESIAN_POINT('Ctrl Pts',(-38.6782040045001,16.5411757610283,10.7838550844415));
#20315=CARTESIAN_POINT('Ctrl Pts',(-38.4902212524322,16.9634289390144,10.7881210903218));
#20316=CARTESIAN_POINT('Ctrl Pts',(-38.4248741812052,17.1852537694117,10.7577447440201));
#20317=CARTESIAN_POINT('Ctrl Pts',(-38.3629592862315,17.5998589150603,10.6429386483201));
#20318=CARTESIAN_POINT('Ctrl Pts',(-38.3595867413123,17.7899553278335,10.5662273743849));
#20319=CARTESIAN_POINT('Ctrl Pts',(-38.3823149509186,17.967967913594,10.4701702229062));
#20320=CARTESIAN_POINT('',(-40.4529448929974,15.9940379355902,9.34999999998873));
#20321=CARTESIAN_POINT('Ctrl Pts',(-40.4529448929974,15.9940379355902,9.34999999998873));
#20322=CARTESIAN_POINT('Ctrl Pts',(-40.2434738433334,15.9690306488097,9.55399283498108));
#20323=CARTESIAN_POINT('Ctrl Pts',(-40.0359153930536,15.9371217884539,9.75864949418921));
#20324=CARTESIAN_POINT('Ctrl Pts',(-39.8302898265985,15.8983409300735,9.96399986488612));
#20325=CARTESIAN_POINT('Ctrl Pts',(-39.668869589359,15.8678971702433,10.1252040678777));
#20326=CARTESIAN_POINT('Ctrl Pts',(-39.5086406647783,15.833217444258,10.2868360245797));
#20327=CARTESIAN_POINT('Ctrl Pts',(-39.3496213890632,15.7942952127127,10.4489096280657));
#20328=CARTESIAN_POINT('',(-41.5426079714122,12.9020046091506,9.34999999998873));
#20329=CARTESIAN_POINT('Origin',(0.,0.,9.34999999999998));
#20330=CARTESIAN_POINT('',(-40.548746775169,12.3227069631096,10.4701702229062));
#20331=CARTESIAN_POINT('Ctrl Pts',(-40.548746775169,12.3227069631096,10.4701702229062));
#20332=CARTESIAN_POINT('Ctrl Pts',(-40.7337738287004,12.4158269473356,10.2660612053919));
#20333=CARTESIAN_POINT('Ctrl Pts',(-40.9159904068387,12.5153104974624,10.0627475751713));
#20334=CARTESIAN_POINT('Ctrl Pts',(-41.0953762596343,12.6211280213747,9.8602004044977));
#20335=CARTESIAN_POINT('Ctrl Pts',(-41.2464706233768,12.7102567413891,9.68959756484312));
#20336=CARTESIAN_POINT('Ctrl Pts',(-41.3955565785978,12.8038799478918,9.51953800447477));
#20337=CARTESIAN_POINT('Ctrl Pts',(-41.5426079714122,12.9020046091506,9.34999999998873));
#20338=CARTESIAN_POINT('',(-41.1968615496291,10.0334970568409,10.4489096280657));
#20339=CARTESIAN_POINT('Ctrl Pts',(-41.1968615496291,10.0334970568408,10.4489096280657));
#20340=CARTESIAN_POINT('Ctrl Pts',(-41.0660803486155,10.1540520151183,10.547449245225));
#20341=CARTESIAN_POINT('Ctrl Pts',(-40.9474985376379,10.3007464994068,10.6271602259564));
#20342=CARTESIAN_POINT('Ctrl Pts',(-40.7302626263145,10.6566552349238,10.7492445866574));
#20343=CARTESIAN_POINT('Ctrl Pts',(-40.6385704103799,10.8683280945854,10.7838550844415));
#20344=CARTESIAN_POINT('Ctrl Pts',(-40.5125939444148,11.3130360790171,10.7881210903218));
#20345=CARTESIAN_POINT('Ctrl Pts',(-40.4794809770131,11.5419029103592,10.7577447440201));
#20346=CARTESIAN_POINT('Ctrl Pts',(-40.4772007506467,11.9610993817013,10.6429386483201));
#20347=CARTESIAN_POINT('Ctrl Pts',(-40.500916073612,12.1497408502736,10.5662273743849));
#20348=CARTESIAN_POINT('Ctrl Pts',(-40.548746775169,12.3227069631096,10.4701702229062));
#20349=CARTESIAN_POINT('',(-42.3173811644569,10.0741873807792,9.34999999998873));
#20350=CARTESIAN_POINT('Ctrl Pts',(-42.3173811644569,10.0741873807792,9.34999999998873));
#20351=CARTESIAN_POINT('Ctrl Pts',(-42.1064833200743,10.0792454706763,9.55399283497921));
#20352=CARTESIAN_POINT('Ctrl Pts',(-41.8964964112446,10.0772000437942,9.75864949418546));
#20353=CARTESIAN_POINT('Ctrl Pts',(-41.6874447249818,10.0680774878698,9.96399986488047));
#20354=CARTESIAN_POINT('Ctrl Pts',(-41.5233349142502,10.0609160965752,10.125204067874));
#20355=CARTESIAN_POINT('Ctrl Pts',(-41.3598014494938,10.0493923136847,10.2868360245778));
#20356=CARTESIAN_POINT('Ctrl Pts',(-41.1968615496291,10.0334970568408,10.4489096280657));
#20357=CARTESIAN_POINT('',(-42.95591082111,6.85855127048189,9.34999999998873));
#20358=CARTESIAN_POINT('Origin',(0.,0.,9.34999999999998));
#20359=CARTESIAN_POINT('',(-41.8897230480067,6.4265912346088,10.4701702229062));
#20360=CARTESIAN_POINT('Ctrl Pts',(-41.8897230480067,6.4265912346088,10.4701702229062));
#20361=CARTESIAN_POINT('Ctrl Pts',(-42.0861191484169,6.49243129646439,10.2660612053901));
#20362=CARTESIAN_POINT('Ctrl Pts',(-42.2806390098733,6.56497012464649,10.0627475751677));
#20363=CARTESIAN_POINT('Ctrl Pts',(-42.4732583771441,6.64418131011342,9.86020040449235));
#20364=CARTESIAN_POINT('Ctrl Pts',(-42.6354991574965,6.71089985833043,9.68959756483957));
#20365=CARTESIAN_POINT('Ctrl Pts',(-42.7963916041478,6.78235297197764,9.519538004473));
#20366=CARTESIAN_POINT('Ctrl Pts',(-42.95591082111,6.85855127048187,9.34999999998873));
#20367=CARTESIAN_POINT('',(-42.2054524109828,4.06844583510791,10.4489096280657));
#20368=CARTESIAN_POINT('Ctrl Pts',(-42.2054524109828,4.06844583510792,10.4489096280657));
#20369=CARTESIAN_POINT('Ctrl Pts',(-42.093159133415,4.20638582320746,10.547449245225));
#20370=CARTESIAN_POINT('Ctrl Pts',(-41.9966611160993,4.3684631204133,10.6271602259564));
#20371=CARTESIAN_POINT('Ctrl Pts',(-41.83228744726,4.75166511176785,10.7492445866574));
#20372=CARTESIAN_POINT('Ctrl Pts',(-41.7716527146639,4.97423260980683,10.7838550844415));
#20373=CARTESIAN_POINT('Ctrl Pts',(-41.7102470523625,5.43234242855308,10.7881210903218));
#20374=CARTESIAN_POINT('Ctrl Pts',(-41.7100422733127,5.66359219215136,10.7577447440201));
#20375=CARTESIAN_POINT('Ctrl Pts',(-41.7674431343866,6.07884635789314,10.6429386483201));
#20376=CARTESIAN_POINT('Ctrl Pts',(-41.8177635496503,6.26219268596147,10.5662273743849));
#20377=CARTESIAN_POINT('Ctrl Pts',(-41.8897230480067,6.42659123460881,10.4701702229062));
#20378=CARTESIAN_POINT('',(-43.3203575886581,3.94925542245288,9.34999999998873));
#20379=CARTESIAN_POINT('Ctrl Pts',(-43.3203575886581,3.94925542245288,9.34999999998873));
#20380=CARTESIAN_POINT('Ctrl Pts',(-43.1123262214859,3.98427592090381,9.55399283498075));
#20381=CARTESIAN_POINT('Ctrl Pts',(-42.9041855820145,4.01213556648781,9.75864949418855));
#20382=CARTESIAN_POINT('Ctrl Pts',(-42.6959634654176,4.03285702195043,9.96399986488512));
#20383=CARTESIAN_POINT('Ctrl Pts',(-42.53250488369,4.04912378446638,10.1252040678771));
#20384=CARTESIAN_POINT('Ctrl Pts',(-42.3689959485123,4.06099053565872,10.2868360245794));
#20385=CARTESIAN_POINT('Ctrl Pts',(-42.2054524109828,4.06844583510791,10.4489096280657));
#20386=CARTESIAN_POINT('',(-43.4947552011066,0.675477606374448,9.34999999998968));
#20387=CARTESIAN_POINT('Origin',(0.,0.,9.34999999999998));
#20388=CARTESIAN_POINT('Ctrl Pts',(-42.3779453595728,0.399648641330075,
10.4701702229062));
#20389=CARTESIAN_POINT('Ctrl Pts',(-42.5817124486134,0.436868467021733,
10.2660612053923));
#20390=CARTESIAN_POINT('Ctrl Pts',(-42.7845757299537,0.480985891900656,
10.0627475751719));
#20391=CARTESIAN_POINT('Ctrl Pts',(-42.986507436847,0.531978227610498,9.86020040449869));
#20392=CARTESIAN_POINT('Ctrl Pts',(-43.1565918793884,0.574928406790011,
9.6895975648441));
#20393=CARTESIAN_POINT('Ctrl Pts',(-43.3260155112353,0.622756848243033,
9.51953800447573));
#20394=CARTESIAN_POINT('Ctrl Pts',(-43.4947552011066,0.675477606374445,
9.34999999998968));
#20395=CARTESIAN_POINT('Origin',(-1.73472347597681E-15,-1.73472347597681E-15,
11.35));
#20396=CARTESIAN_POINT('',(-5.00000000000001,14.142135623731,11.35));
#20397=CARTESIAN_POINT('',(5.,14.142135623731,11.35));
#20398=CARTESIAN_POINT('Origin',(-1.73472347597681E-15,-1.73472347597681E-15,
11.35));
#20399=CARTESIAN_POINT('',(5.,14.142135623731,-11.35));
#20400=CARTESIAN_POINT('',(5.,14.142135623731,11.35));
#20401=CARTESIAN_POINT('',(-5.00000000000001,14.142135623731,-11.35));
#20402=CARTESIAN_POINT('Origin',(-3.46944695195361E-15,1.73472347597681E-15,
-11.35));
#20403=CARTESIAN_POINT('',(-5.00000000000001,14.142135623731,11.35));
#20404=CARTESIAN_POINT('Origin',(-3.46944695195361E-15,3.46944695195361E-15,
-9.34999999999999));
#20405=CARTESIAN_POINT('',(42.3549304887758,1.97901608230145,-10.4488603766003));
#20406=CARTESIAN_POINT('',(42.3778559173176,-0.400053103664774,-10.4702558451011));
#20407=CARTESIAN_POINT('Ctrl Pts',(42.3778559173178,-0.400053103664613,
-10.470255845101));
#20408=CARTESIAN_POINT('Ctrl Pts',(42.3147058279902,-0.298272918361279,
-10.5343638976599));
#20409=CARTESIAN_POINT('Ctrl Pts',(42.2597977418668,-0.186602611546638,
-10.589958769092));
#20410=CARTESIAN_POINT('Ctrl Pts',(42.165574364121,0.0594627592708472,-10.6845737030941));
#20411=CARTESIAN_POINT('Ctrl Pts',(42.1277472101709,0.193934008724945,-10.7220376404442));
#20412=CARTESIAN_POINT('Ctrl Pts',(42.0583624188826,0.559734595935365,-10.788524357582));
#20413=CARTESIAN_POINT('Ctrl Pts',(42.046111502818,0.795598132314873,-10.7969991342825));
#20414=CARTESIAN_POINT('Ctrl Pts',(42.080062787682,1.20890695925822,-10.7529641474054));
#20415=CARTESIAN_POINT('Ctrl Pts',(42.1138804087149,1.38542074401615,-10.7136554733273));
#20416=CARTESIAN_POINT('Ctrl Pts',(42.2140750286918,1.70635615105641,-10.6017307219916));
#20417=CARTESIAN_POINT('Ctrl Pts',(42.2777622816001,1.85044081093512,-10.5319455628));
#20418=CARTESIAN_POINT('Ctrl Pts',(42.3549304887758,1.97901608230144,-10.4488603766003));
#20419=CARTESIAN_POINT('',(43.4947470521204,-0.676002124309743,-9.34999999999999));
#20420=CARTESIAN_POINT('Ctrl Pts',(42.3778559173176,-0.400053103664769,
-10.4702558451011));
#20421=CARTESIAN_POINT('Ctrl Pts',(42.581680861761,-0.437302204766713,-10.2660883608697));
#20422=CARTESIAN_POINT('Ctrl Pts',(42.7846012120674,-0.481452073895284,
-10.0627168613337));
#20423=CARTESIAN_POINT('Ctrl Pts',(42.9865892255721,-0.5324797140179,-9.86011239009894));
#20424=CARTESIAN_POINT('Ctrl Pts',(43.1566436205362,-0.575440057638944,
-9.68953899727716));
#20425=CARTESIAN_POINT('Ctrl Pts',(43.3260372643517,-0.623276250889277,
-9.51950878957767));
#20426=CARTESIAN_POINT('Ctrl Pts',(43.4947470521204,-0.676002124309744,
-9.35));
#20427=CARTESIAN_POINT('',(43.3203086503666,-3.94979220174698,-9.34999999999999));
#20428=CARTESIAN_POINT('Origin',(-3.46944695195361E-15,3.46944695195361E-15,
-9.34999999999999));
#20429=CARTESIAN_POINT('',(42.2054617208597,-4.06886253050386,-10.4488603765996));
#20430=CARTESIAN_POINT('Ctrl Pts',(43.3203086503666,-3.94979220174697,-9.34999999999999));
#20431=CARTESIAN_POINT('Ctrl Pts',(43.1122825236194,-3.98478982701022,-9.55398902691224));
#20432=CARTESIAN_POINT('Ctrl Pts',(42.9041475658189,-4.01262695712675,-9.75864153760776));
#20433=CARTESIAN_POINT('Ctrl Pts',(42.6959315890968,-4.03332628397407,-9.96398744092348));
#20434=CARTESIAN_POINT('Ctrl Pts',(42.5324864596819,-4.04957481690908,-10.1251796235343));
#20435=CARTESIAN_POINT('Ctrl Pts',(42.3689912631274,-4.06142404123509,-10.2867993162798));
#20436=CARTESIAN_POINT('Ctrl Pts',(42.2054617208598,-4.06886253050386,-10.4488603765996));
#20437=CARTESIAN_POINT('',(41.8895769551558,-6.42697885114752,-10.4702558450972));
#20438=CARTESIAN_POINT('Ctrl Pts',(42.2054617208598,-4.06886253050389,-10.4488603765996));
#20439=CARTESIAN_POINT('Ctrl Pts',(42.0931565705379,-4.20679248947824,-10.5474113287244));
#20440=CARTESIAN_POINT('Ctrl Pts',(41.996645286846,-4.36886244651051,-10.6271346454319));
#20441=CARTESIAN_POINT('Ctrl Pts',(41.8322466693354,-4.75204677305466,-10.7492419669034));
#20442=CARTESIAN_POINT('Ctrl Pts',(41.7715980988903,-4.97460297984299,-10.7838654920941));
#20443=CARTESIAN_POINT('Ctrl Pts',(41.7101624561659,-5.43269747180814,-10.788159089135));
#20444=CARTESIAN_POINT('Ctrl Pts',(41.7099416343871,-5.6639427088267,-10.7577973127672));
#20445=CARTESIAN_POINT('Ctrl Pts',(41.7673137310951,-6.07920795450595,-10.6430146790632));
#20446=CARTESIAN_POINT('Ctrl Pts',(41.8176243487664,-6.26256709540618,-10.5663096368479));
#20447=CARTESIAN_POINT('Ctrl Pts',(41.8895769551558,-6.42697885114752,-10.4702558450972));
#20448=CARTESIAN_POINT('',(42.9558281083822,-6.85906928986172,-9.34999999999999));
#20449=CARTESIAN_POINT('Ctrl Pts',(41.8895769551558,-6.42697885114752,-10.4702558450972));
#20450=CARTESIAN_POINT('Ctrl Pts',(42.0860261557596,-6.49285612411399,-10.266088360863));
#20451=CARTESIAN_POINT('Ctrl Pts',(42.2805978880048,-6.56543518807053,-10.0627168613241));
#20452=CARTESIAN_POINT('Ctrl Pts',(42.4732679644259,-6.64468933186833,-9.86011239008662));
#20453=CARTESIAN_POINT('Ctrl Pts',(42.635477556489,-6.7114136648501,-9.68953899726898));
#20454=CARTESIAN_POINT('Ctrl Pts',(42.796339217146,-6.78287018364921,-9.51950878957359));
#20455=CARTESIAN_POINT('Ctrl Pts',(42.9558281083822,-6.85906928986171,-9.34999999999999));
#20456=CARTESIAN_POINT('',(42.31725633263,-10.0747117317813,-9.34999999999999));
#20457=CARTESIAN_POINT('Origin',(-3.46944695195361E-15,3.46944695195361E-15,
-9.34999999999999));
#20458=CARTESIAN_POINT('',(41.1968114628114,-10.0339108357988,-10.4488603765985));
#20459=CARTESIAN_POINT('Ctrl Pts',(42.31725633263,-10.0747117317813,-9.34999999999999));
#20460=CARTESIAN_POINT('Ctrl Pts',(42.1063669305224,-10.079747927096,-9.55398902691493));
#20461=CARTESIAN_POINT('Ctrl Pts',(41.8963888498135,-10.0776810225061,-9.75864153761314));
#20462=CARTESIAN_POINT('Ctrl Pts',(41.6873463901567,-10.0685374369976,-9.96398744093155));
#20463=CARTESIAN_POINT('Ctrl Pts',(41.5232524891573,-10.0613599161357,-10.1251796235393));
#20464=CARTESIAN_POINT('Ctrl Pts',(41.3597351175228,-10.0498207399865,-10.2867993162818));
#20465=CARTESIAN_POINT('Ctrl Pts',(41.1968114628114,-10.0339108357988,-10.4488603765985));
#20466=CARTESIAN_POINT('',(40.548547005747,-12.3230698430749,-10.4702558451024));
#20467=CARTESIAN_POINT('Ctrl Pts',(41.1968114628111,-10.0339108357987,-10.4488603765988));
#20468=CARTESIAN_POINT('Ctrl Pts',(41.0660199366633,-10.1544541778436,-10.5474113291164));
#20469=CARTESIAN_POINT('Ctrl Pts',(40.9474260385374,-10.3011395093532,-10.6271346460638));
#20470=CARTESIAN_POINT('Ctrl Pts',(40.7301679463267,-10.6570272102986,-10.7492419673839));
#20471=CARTESIAN_POINT('Ctrl Pts',(40.6384636404816,-10.868686924454,-10.7838654923527));
#20472=CARTESIAN_POINT('Ctrl Pts',(40.5124596809018,-11.3133754715734,-10.7881590889262));
#20473=CARTESIAN_POINT('Ctrl Pts',(40.479331478489,-11.5422355392621,-10.7577973123347));
#20474=CARTESIAN_POINT('Ctrl Pts',(40.4770212041179,-11.9614388832522,-10.6430146784606));
#20475=CARTESIAN_POINT('Ctrl Pts',(40.5007250057626,-12.1500916390904,-10.566309636471));
#20476=CARTESIAN_POINT('Ctrl Pts',(40.5485470057468,-12.3230698430748,-10.4702558451027));
#20477=CARTESIAN_POINT('',(41.5424523787385,-12.9025055845851,-9.34999999999999));
#20478=CARTESIAN_POINT('Ctrl Pts',(40.548547005747,-12.3230698430749,-10.4702558451024));
#20479=CARTESIAN_POINT('Ctrl Pts',(40.7336213240881,-12.416234217002,-10.2660883599951));
#20480=CARTESIAN_POINT('Ctrl Pts',(40.9158835196664,-12.5157649757987,-10.0627168595901));
#20481=CARTESIAN_POINT('Ctrl Pts',(41.0953134525996,-12.6216322379599,-9.860112387496));
#20482=CARTESIAN_POINT('Ctrl Pts',(41.2463761214623,-12.7107622448981,-9.68953899554443));
#20483=CARTESIAN_POINT('Ctrl Pts',(41.395431118676,-12.8043844401388,-9.51950878871185));
#20484=CARTESIAN_POINT('Ctrl Pts',(41.5424523787385,-12.9025055845851,-9.34999999999999));
#20485=CARTESIAN_POINT('',(40.4527467088507,-15.9945391840333,-9.34999999999999));
#20486=CARTESIAN_POINT('Origin',(-3.46944695195361E-15,3.46944695195361E-15,
-9.34999999999999));
#20487=CARTESIAN_POINT('',(39.3495129251698,-15.7946976519001,-10.4488603766002));
#20488=CARTESIAN_POINT('Ctrl Pts',(40.4527467088507,-15.9945391840333,-9.34999999999999));
#20489=CARTESIAN_POINT('Ctrl Pts',(40.2432871314601,-15.9695114269873,-9.55398902691222));
#20490=CARTESIAN_POINT('Ctrl Pts',(40.0357404760446,-15.9375825639096,-9.7586415376077));
#20491=CARTESIAN_POINT('Ctrl Pts',(39.8301270351082,-15.8987822030802,-9.96398744092336));
#20492=CARTESIAN_POINT('Ctrl Pts',(39.6687248411344,-15.8683247420489,-10.1251796235344));
#20493=CARTESIAN_POINT('Ctrl Pts',(39.5085140365547,-15.8336320697752,-10.2867993162802));
#20494=CARTESIAN_POINT('Ctrl Pts',(39.3495129251698,-15.7946976519002,-10.4488603766002));
#20495=CARTESIAN_POINT('',(38.3820655716558,-17.9682986698111,-10.4702558451043));
#20496=CARTESIAN_POINT('Ctrl Pts',(39.3495129251697,-15.7946976518998,-10.4488603766004));
#20497=CARTESIAN_POINT('Ctrl Pts',(39.2028975619447,-15.8954004616404,-10.5474113291176));
#20498=CARTESIAN_POINT('Ctrl Pts',(39.064635279473,-16.0237150765457,-10.6271346460648));
#20499=CARTESIAN_POINT('Ctrl Pts',(38.7989404607774,-16.3450613035865,-10.7492419673849));
#20500=CARTESIAN_POINT('Ctrl Pts',(38.6780472545499,-16.5415157435849,-10.7838654923536));
#20501=CARTESIAN_POINT('Ctrl Pts',(38.4900400549303,-16.9637457693538,-10.7881590889271));
#20502=CARTESIAN_POINT('Ctrl Pts',(38.4246788663307,-17.185561736774,-10.7577973123357));
#20503=CARTESIAN_POINT('Ctrl Pts',(38.3627332511181,-17.60016940884,-10.6430146784615));
#20504=CARTESIAN_POINT('Ctrl Pts',(38.3593476958032,-17.7902753543356,-10.5663096364721));
#20505=CARTESIAN_POINT('Ctrl Pts',(38.3820655716563,-17.9682986698106,-10.470255845104));
#20506=CARTESIAN_POINT('',(39.2833921172024,-18.6832840733669,-9.34999999999999));
#20507=CARTESIAN_POINT('Ctrl Pts',(38.3820655716558,-17.9682986698111,-10.4702558451043));
#20508=CARTESIAN_POINT('Ctrl Pts',(38.5519974274795,-18.0868535864241,-10.2660883600012));
#20509=CARTESIAN_POINT('Ctrl Pts',(38.7182397528624,-18.211309880492,-10.0627168596004));
#20510=CARTESIAN_POINT('Ctrl Pts',(38.8807768654989,-18.341635108456,-9.86011238751062));
#20511=CARTESIAN_POINT('Ctrl Pts',(39.0176174116884,-18.4513563597297,-9.68953899555414));
#20512=CARTESIAN_POINT('Ctrl Pts',(39.1518314163795,-18.5652383538402,-9.51950878871669));
#20513=CARTESIAN_POINT('Ctrl Pts',(39.2833921172024,-18.6832840733669,-9.35));
#20514=CARTESIAN_POINT('',(37.7647358181625,-21.5887639429495,-9.34999999999999));
#20515=CARTESIAN_POINT('Origin',(-3.46944695195361E-15,3.46944695195361E-15,
-9.34999999999999));
#20516=CARTESIAN_POINT('',(36.7011717789887,-21.233949971968,-10.4488603766022));
#20517=CARTESIAN_POINT('Ctrl Pts',(37.7647358181625,-21.5887639429495,-9.34999999999999));
#20518=CARTESIAN_POINT('Ctrl Pts',(37.5609700584511,-21.5341817265036,-9.55398902691086));
#20519=CARTESIAN_POINT('Ctrl Pts',(37.3600798797159,-21.4730408845162,-9.75864153760501));
#20520=CARTESIAN_POINT('Ctrl Pts',(37.1620811542153,-21.4053736118224,-9.96398744091935));
#20521=CARTESIAN_POINT('Ctrl Pts',(37.0066563504919,-21.3522562366961,-10.1251796235324));
#20522=CARTESIAN_POINT('Ctrl Pts',(36.8530135429395,-21.2951163110601,-10.2867993162802));
#20523=CARTESIAN_POINT('Ctrl Pts',(36.7011717789887,-21.233949971968,-10.4488603766022));
#20524=CARTESIAN_POINT('',(35.4342359672589,-23.2477447519415,-10.4702558450997));
#20525=CARTESIAN_POINT('Ctrl Pts',(36.7011717789887,-21.233949971968,-10.4488603766022));
#20526=CARTESIAN_POINT('Ctrl Pts',(36.5417172446773,-21.3127622306018,-10.5474113291192));
#20527=CARTESIAN_POINT('Ctrl Pts',(36.386601199215,-21.4200940133731,-10.6271346460661));
#20528=CARTESIAN_POINT('Ctrl Pts',(36.0778784343425,-21.7003570840141,-10.7492419673852));
#20529=CARTESIAN_POINT('Ctrl Pts',(35.9302573647846,-21.8776070039851,-10.7838654923534));
#20530=CARTESIAN_POINT('Ctrl Pts',(35.6840742095426,-22.2687831226896,-10.7881590889257));
#20531=CARTESIAN_POINT('Ctrl Pts',(35.5878106000705,-22.479039456409,-10.7577973123336));
#20532=CARTESIAN_POINT('Ctrl Pts',(35.4674906781066,-22.8806112399779,-10.6430146784584));
#20533=CARTESIAN_POINT('Ctrl Pts',(35.4370846859756,-23.0683003663016,-10.5663096364684));
#20534=CARTESIAN_POINT('Ctrl Pts',(35.4342359672589,-23.2477447519415,-10.4702558450997));
#20535=CARTESIAN_POINT('',(36.2246352761032,-24.0837247765644,-9.34999999999999));
#20536=CARTESIAN_POINT('Ctrl Pts',(35.4342359672589,-23.2477447519415,-10.4702558450997));
#20537=CARTESIAN_POINT('Ctrl Pts',(35.585566038032,-23.3892767750272,-10.2660883599914));
#20538=CARTESIAN_POINT('Ctrl Pts',(35.7324042788861,-23.5361250331267,-10.0627168595854));
#20539=CARTESIAN_POINT('Ctrl Pts',(35.8747397843386,-23.6882551810849,-9.86011238749032));
#20540=CARTESIAN_POINT('Ctrl Pts',(35.9945725289411,-23.81633406842,-9.68953899554068));
#20541=CARTESIAN_POINT('Ctrl Pts',(36.1112133310069,-23.9481575524003,-9.51950878870999));
#20542=CARTESIAN_POINT('Ctrl Pts',(36.2246352761032,-24.0837247765644,-9.34999999999999));
#20543=CARTESIAN_POINT('',(34.3079438107283,-26.7435037248284,-9.34999999999999));
#20544=CARTESIAN_POINT('Origin',(-3.46944695195361E-15,3.46944695195361E-15,
-9.34999999999999));
#20545=CARTESIAN_POINT('',(33.3057006128401,-26.240940304242,-10.4488603766015));
#20546=CARTESIAN_POINT('Ctrl Pts',(34.3079438107283,-26.7435037248284,-9.34999999999999));
#20547=CARTESIAN_POINT('Ctrl Pts',(34.1140199519477,-26.6604781855038,-9.55398902691468));
#20548=CARTESIAN_POINT('Ctrl Pts',(33.9238757946085,-26.5713700158305,-9.75864153761266));
#20549=CARTESIAN_POINT('Ctrl Pts',(33.7375224676096,-26.4762133418042,-9.96398744093084));
#20550=CARTESIAN_POINT('Ctrl Pts',(33.5912390549387,-26.4015173691637,-10.1251796235398));
#20551=CARTESIAN_POINT('Ctrl Pts',(33.4472919689122,-26.3230933942746,-10.2867993162836));
#20552=CARTESIAN_POINT('Ctrl Pts',(33.3057006128402,-26.240940304242,-10.4488603766015));
#20553=CARTESIAN_POINT('',(31.7650675024754,-28.0539337918554,-10.4702558451018));
#20554=CARTESIAN_POINT('Ctrl Pts',(33.3057006128397,-26.2409403042424,-10.4488603766016));
#20555=CARTESIAN_POINT('Ctrl Pts',(33.1366529419318,-26.2962576214585,-10.5474113291188));
#20556=CARTESIAN_POINT('Ctrl Pts',(32.9678408488468,-26.380421606517,-10.6271346460658));
#20557=CARTESIAN_POINT('Ctrl Pts',(32.6223748430073,-26.6138961728501,-10.7492419673852));
#20558=CARTESIAN_POINT('Ctrl Pts',(32.4510310493911,-26.7683332755687,-10.7838654923535));
#20559=CARTESIAN_POINT('Ctrl Pts',(32.1516835176331,-27.1204922694895,-10.7881590889263));
#20560=CARTESIAN_POINT('Ctrl Pts',(32.0264771367756,-27.3149087568822,-10.7577973123345));
#20561=CARTESIAN_POINT('Ctrl Pts',(31.8502322746963,-27.6952698084771,-10.6430146784599));
#20562=CARTESIAN_POINT('Ctrl Pts',(31.7934248240649,-27.8767213062674,-10.5663096364702));
#20563=CARTESIAN_POINT('Ctrl Pts',(31.7650675024754,-28.0539337918554,-10.4702558451019));
#20564=CARTESIAN_POINT('',(32.428449324012,-28.9938902950258,-9.34999999999999));
#20565=CARTESIAN_POINT('Ctrl Pts',(31.7650675024754,-28.0539337918554,-10.4702558451018));
#20566=CARTESIAN_POINT('Ctrl Pts',(31.8947151443511,-28.2155617375662,-10.2660883599943));
#20567=CARTESIAN_POINT('Ctrl Pts',(32.0191600975335,-28.3818125526352,-10.0627168595892));
#20568=CARTESIAN_POINT('Ctrl Pts',(32.1383964553672,-28.5526506894797,-9.86011238749498));
#20569=CARTESIAN_POINT('Ctrl Pts',(32.2387819492775,-28.6964798960859,-9.68953899554376));
#20570=CARTESIAN_POINT('Ctrl Pts',(32.3354750783575,-28.843561323957,-9.51950878871151));
#20571=CARTESIAN_POINT('Ctrl Pts',(32.428449324012,-28.9938902950258,-9.35));
#20572=CARTESIAN_POINT('',(30.15274100324,-31.3538228927755,-9.34999999999999));
#20573=CARTESIAN_POINT('Origin',(-3.46944695195361E-15,3.46944695195361E-15,
-9.34999999999999));
#20574=CARTESIAN_POINT('',(29.2322214279089,-30.7137407645584,-10.4488603766032));
#20575=CARTESIAN_POINT('Ctrl Pts',(30.15274100324,-31.3538228927755,-9.34999999999999));
#20576=CARTESIAN_POINT('Ctrl Pts',(29.9726067759282,-31.2440441911298,-9.55398902691379));
#20577=CARTESIAN_POINT('Ctrl Pts',(29.7970794267014,-31.1287826791412,-9.75864153761091));
#20578=CARTESIAN_POINT('Ctrl Pts',(29.6261651145468,-31.0080737192595,-9.96398744092823));
#20579=CARTESIAN_POINT('Ctrl Pts',(29.4920010013578,-30.9133197437011,-10.1251796235386));
#20580=CARTESIAN_POINT('Ctrl Pts',(29.360679984414,-30.8152082055302,-10.2867993162838));
#20581=CARTESIAN_POINT('Ctrl Pts',(29.232221427909,-30.7137407645584,-10.4488603766032));
#20582=CARTESIAN_POINT('',(27.4492538662204,-32.2890256406531,-10.4702558450977));
#20583=CARTESIAN_POINT('Ctrl Pts',(29.232221427909,-30.7137407645579,-10.4488603766035));
#20584=CARTESIAN_POINT('Ctrl Pts',(29.0570219434909,-30.7444370393004,-10.5474113291203));
#20585=CARTESIAN_POINT('Ctrl Pts',(28.8779503301844,-30.8037198906201,-10.627134646067));
#20586=CARTESIAN_POINT('Ctrl Pts',(28.5027737750148,-30.9856530837616,-10.7492419673855));
#20587=CARTESIAN_POINT('Ctrl Pts',(28.3111953228635,-31.1141334751775,-10.7838654923533));
#20588=CARTESIAN_POINT('Ctrl Pts',(27.9647772670893,-31.4201064027429,-10.7881590889249));
#20589=CARTESIAN_POINT('Ctrl Pts',(27.8131769556956,-31.5947252847772,-10.7577973123325));
#20590=CARTESIAN_POINT('Ctrl Pts',(27.5845949906459,-31.9461325502595,-10.6430146784567));
#20591=CARTESIAN_POINT('Ctrl Pts',(27.5025425173903,-32.1176525902846,-10.5663096364665));
#20592=CARTESIAN_POINT('Ctrl Pts',(27.4492538662209,-32.2890256406529,-10.4702558450976));
#20593=CARTESIAN_POINT('',(27.9721136596011,-33.3138238185646,-9.34999999999999));
#20594=CARTESIAN_POINT('Ctrl Pts',(27.4492538662204,-32.2890256406531,-10.4702558450977));
#20595=CARTESIAN_POINT('Ctrl Pts',(27.5545798270844,-32.46745923011,-10.2660883599907));
#20596=CARTESIAN_POINT('Ctrl Pts',(27.6540981522194,-32.6497282149806,-10.062716859586));
#20597=CARTESIAN_POINT('Ctrl Pts',(27.7478080540396,-32.8357965689006,-9.86011238749213));
#20598=CARTESIAN_POINT('Ctrl Pts',(27.8267027380888,-32.9924481468975,-9.68953899554188));
#20599=CARTESIAN_POINT('Ctrl Pts',(27.9014798009146,-33.1517933649324,-9.51950878871058));
#20600=CARTESIAN_POINT('Ctrl Pts',(27.9721136596011,-33.3138238185646,-9.34999999999999));
#20601=CARTESIAN_POINT('',(25.3837153422573,-35.325868643577,-9.34999999999999));
#20602=CARTESIAN_POINT('Origin',(-3.46944695195361E-15,3.46944695195361E-15,
-9.34999999999999));
#20603=CARTESIAN_POINT('',(24.5636585134848,-34.5612980340113,-10.4488603766026));
#20604=CARTESIAN_POINT('Ctrl Pts',(25.3837153422573,-35.325868643577,-9.34999999999999));
#20605=CARTESIAN_POINT('Ctrl Pts',(25.2210377598187,-35.1915715573989,-9.55398902691333));
#20606=CARTESIAN_POINT('Ctrl Pts',(25.063700449356,-35.0525030950913,-9.75864153760996));
#20607=CARTESIAN_POINT('Ctrl Pts',(24.9117044745655,-34.9086991356805,-9.9639874409268));
#20608=CARTESIAN_POINT('Ctrl Pts',(24.7923908553075,-34.7958160748984,-10.1251796235375));
#20609=CARTESIAN_POINT('Ctrl Pts',(24.6763692246546,-34.6800142414323,-10.2867993162829));
#20610=CARTESIAN_POINT('Ctrl Pts',(24.5636585134848,-34.5612980340113,-10.4488603766026));
#20611=CARTESIAN_POINT('',(22.5746525783699,-35.8668060412517,-10.470255845099));
#20612=CARTESIAN_POINT('Ctrl Pts',(24.563658513485,-34.5612980340106,-10.448860376603));
#20613=CARTESIAN_POINT('Ctrl Pts',(24.3858737718256,-34.566748378646,-10.5474113291201));
#20614=CARTESIAN_POINT('Ctrl Pts',(24.2001880199446,-34.5999432683309,-10.6271346460669));
#20615=CARTESIAN_POINT('Ctrl Pts',(23.802938428188,-34.7266314531191,-10.7492419673858));
#20616=CARTESIAN_POINT('Ctrl Pts',(23.5950253023206,-34.8265396429691,-10.7838654923538));
#20617=CARTESIAN_POINT('Ctrl Pts',(23.2085887951579,-35.0800977777257,-10.7881590889258));
#20618=CARTESIAN_POINT('Ctrl Pts',(23.0336806983883,-35.2313643175223,-10.7577973123335));
#20619=CARTESIAN_POINT('Ctrl Pts',(22.7574148999991,-35.5466641583413,-10.643014678458));
#20620=CARTESIAN_POINT('Ctrl Pts',(22.6517877558542,-35.7047610872093,-10.5663096364679));
#20621=CARTESIAN_POINT('Ctrl Pts',(22.5746525783699,-35.8668060412516,-10.470255845099));
#20622=CARTESIAN_POINT('',(22.9463464260018,-36.9555839582859,-9.34999999999999));
#20623=CARTESIAN_POINT('Ctrl Pts',(22.5746525783699,-35.8668060412517,-10.4702558450989));
#20624=CARTESIAN_POINT('Ctrl Pts',(22.6535127253941,-36.0584128811362,-10.26608835999));
#20625=CARTESIAN_POINT('Ctrl Pts',(22.7260785163689,-36.2529895648998,-10.0627168595834));
#20626=CARTESIAN_POINT('Ctrl Pts',(22.7923542988114,-36.4505003207895,-9.86011238748777));
#20627=CARTESIAN_POINT('Ctrl Pts',(22.848152104745,-36.6167852957953,-9.68953899553898));
#20628=CARTESIAN_POINT('Ctrl Pts',(22.8994908559558,-36.7851504948688,-9.51950878870914));
#20629=CARTESIAN_POINT('Ctrl Pts',(22.9463464260018,-36.9555839582859,-9.34999999999999));
#20630=CARTESIAN_POINT('',(20.0979504375088,-38.5787815801827,-9.34999999999999));
#20631=CARTESIAN_POINT('Origin',(-3.46944695195361E-15,3.46944695195361E-15,
-9.34999999999999));
#20632=CARTESIAN_POINT('',(19.3950503474966,-37.7052869420423,-10.4488603765928));
#20633=CARTESIAN_POINT('Ctrl Pts',(20.0979504375088,-38.5787815801827,-9.34999999999999));
#20634=CARTESIAN_POINT('Ctrl Pts',(19.9560411463964,-38.4227000108602,-9.55398902691918));
#20635=CARTESIAN_POINT('Ctrl Pts',(19.8200968086136,-38.2626556310799,-9.75864153762166));
#20636=CARTESIAN_POINT('Ctrl Pts',(19.690113370912,-38.0986841060511,-9.96398744094433));
#20637=CARTESIAN_POINT('Ctrl Pts',(19.588079126809,-37.9699699336414,-10.125179623546));
#20638=CARTESIAN_POINT('Ctrl Pts',(19.4897187482756,-37.8388351962714,-10.2867993162823));
#20639=CARTESIAN_POINT('Ctrl Pts',(19.3950503474966,-37.7052869420423,-10.4488603765928));
#20640=CARTESIAN_POINT('',(17.2404964639731,-38.7144417021608,-10.470255845106));
#20641=CARTESIAN_POINT('Ctrl Pts',(19.3950503474966,-37.7052869420422,-10.4488603765929));
#20642=CARTESIAN_POINT('Ctrl Pts',(19.2182995332483,-37.6853804032696,-10.5474113291113));
#20643=CARTESIAN_POINT('Ctrl Pts',(19.029779669228,-37.6918115790903,-10.6271346460595));
#20644=CARTESIAN_POINT('Ctrl Pts',(18.6185438970004,-37.7606757494185,-10.7492419673812));
#20645=CARTESIAN_POINT('Ctrl Pts',(18.398528609088,-37.8299778950671,-10.7838654923508));
#20646=CARTESIAN_POINT('Ctrl Pts',(17.9799403834319,-38.0259595245895,-10.7881590889263));
#20647=CARTESIAN_POINT('Ctrl Pts',(17.7852851257429,-38.1507943716133,-10.7577973123358));
#20648=CARTESIAN_POINT('Ctrl Pts',(17.4669594689832,-38.4235681922572,-10.6430146784635));
#20649=CARTESIAN_POINT('Ctrl Pts',(17.3399079179993,-38.5650236124094,-10.5663096364746));
#20650=CARTESIAN_POINT('Ctrl Pts',(17.2404964639731,-38.7144417021598,-10.4702558451068));
#20651=CARTESIAN_POINT('',(17.4534577509835,-39.8450349797141,-9.34999999999999));
#20652=CARTESIAN_POINT('Ctrl Pts',(17.2404964639731,-38.7144417021608,-10.470255845106));
#20653=CARTESIAN_POINT('Ctrl Pts',(17.2912854319751,-38.9153212297603,-10.2660883599972));
#20654=CARTESIAN_POINT('Ctrl Pts',(17.3354214585452,-39.1182445922472,-10.0627168595908));
#20655=CARTESIAN_POINT('Ctrl Pts',(17.3729139378,-39.3231770006896,-9.86011238749544));
#20656=CARTESIAN_POINT('Ctrl Pts',(17.4044789831962,-39.4957102901439,-9.68953899554403));
#20657=CARTESIAN_POINT('Ctrl Pts',(17.4313343138652,-39.6696680403328,-9.51950878871163));
#20658=CARTESIAN_POINT('Ctrl Pts',(17.4534577509835,-39.8450349797141,-9.34999999999999));
#20659=CARTESIAN_POINT('',(14.4030492195297,-41.046341775849,-9.34999999999999));
#20660=CARTESIAN_POINT('Origin',(-3.46944695195361E-15,3.46944695195361E-15,
-9.34999999999999));
#20661=CARTESIAN_POINT('',(13.8316148870825,-40.0817049410147,-10.4488603765993));
#20662=CARTESIAN_POINT('Ctrl Pts',(14.4030492195297,-41.046341775849,-9.34999999999999));
#20663=CARTESIAN_POINT('Ctrl Pts',(14.2847970836793,-40.8716530940395,-9.55398902691715));
#20664=CARTESIAN_POINT('Ctrl Pts',(14.1730131532637,-40.6938908388371,-9.75864153761761));
#20665=CARTESIAN_POINT('Ctrl Pts',(14.0676883406023,-40.5130897355934,-9.96398744093829));
#20666=CARTESIAN_POINT('Ctrl Pts',(13.9850105946094,-40.3711647009173,-10.125179623544));
#20667=CARTESIAN_POINT('Ctrl Pts',(13.906313801843,-40.2273665847263,-10.2867993162846));
#20668=CARTESIAN_POINT('Ctrl Pts',(13.8316148870826,-40.0817049410147,-10.4488603765992));
#20669=CARTESIAN_POINT('',(11.5553735590042,-40.7739629732828,-10.4702558451002));
#20670=CARTESIAN_POINT('Ctrl Pts',(13.8316148870824,-40.0817049410149,-10.4488603765991));
#20671=CARTESIAN_POINT('Ctrl Pts',(13.6594961371153,-40.036846758561,-10.5474113291163));
#20672=CARTESIAN_POINT('Ctrl Pts',(13.4719798817408,-40.0163833003267,-10.6271346460633));
#20673=CARTESIAN_POINT('Ctrl Pts',(13.0551295034576,-40.0260215802802,-10.749241967383));
#20674=CARTESIAN_POINT('Ctrl Pts',(12.8274909302894,-40.0633068898959,-10.7838654923515));
#20675=CARTESIAN_POINT('Ctrl Pts',(12.385272235305,-40.1977223933772,-10.7881590889245));
#20676=CARTESIAN_POINT('Ctrl Pts',(12.1748324364042,-40.2935842701396,-10.7577973123327));
#20677=CARTESIAN_POINT('Ctrl Pts',(11.8209271136738,-40.5182791822383,-10.6430146784582));
#20678=CARTESIAN_POINT('Ctrl Pts',(11.6750375590451,-40.6402134692447,-10.5663096364687));
#20679=CARTESIAN_POINT('Ctrl Pts',(11.5553735590047,-40.7739629732822,-10.4702558451006));
#20680=CARTESIAN_POINT('',(11.6052670077404,-41.9233559925617,-9.34999999999999));
#20681=CARTESIAN_POINT('Ctrl Pts',(11.5553735590042,-40.7739629732828,-10.4702558451002));
#20682=CARTESIAN_POINT('Ctrl Pts',(11.5770574310621,-40.980025860697,-10.2660883599968));
#20683=CARTESIAN_POINT('Ctrl Pts',(11.5918652110079,-41.1871649674224,-10.0627168595958));
#20684=CARTESIAN_POINT('Ctrl Pts',(11.5998111483213,-41.3953471955505,-9.86011238750566));
#20685=CARTESIAN_POINT('Ctrl Pts',(11.6065008598849,-41.5706165192242,-9.68953899555085));
#20686=CARTESIAN_POINT('Ctrl Pts',(11.6083260729273,-41.7466255423864,-9.51950878871505));
#20687=CARTESIAN_POINT('Ctrl Pts',(11.6052670077404,-41.9233559925616,-9.34999999999999));
#20688=CARTESIAN_POINT('',(8.41494345441915,-42.6783168208275,-9.34999999999999));
#20689=CARTESIAN_POINT('Origin',(-3.46944695195361E-15,3.46944695195361E-15,
-9.34999999999999));
#20690=CARTESIAN_POINT('',(7.98660763467823,-41.642175013475,-10.4488603765986));
#20691=CARTESIAN_POINT('Ctrl Pts',(8.41494345441915,-42.6783168208275,-9.34999999999999));
#20692=CARTESIAN_POINT('Ctrl Pts',(8.3227557463064,-42.4885771843301,-9.55398902691651));
#20693=CARTESIAN_POINT('Ctrl Pts',(8.23740782172385,-42.2967157805956,-9.75864153761634));
#20694=CARTESIAN_POINT('Ctrl Pts',(8.15888574355747,-42.1027656882098,-9.96398744093637));
#20695=CARTESIAN_POINT('Ctrl Pts',(8.09724757616397,-41.9505189756976,-10.1251796235425));
#20696=CARTESIAN_POINT('Ctrl Pts',(8.03981640892606,-41.7969847956541,-10.2867993162835));
#20697=CARTESIAN_POINT('Ctrl Pts',(7.98660763467823,-41.642175013475,-10.4488603765986));
#20698=CARTESIAN_POINT('',(5.63501657134564,-42.0034439406514,-10.4702558450999));
#20699=CARTESIAN_POINT('Ctrl Pts',(7.98660763467821,-41.6421750134749,-10.4488603765987));
#20700=CARTESIAN_POINT('Ctrl Pts',(7.8226247910452,-41.5732783708473,-10.5474113287234));
#20701=CARTESIAN_POINT('Ctrl Pts',(7.63992943532065,-41.5263368556522,-10.6271346454309));
#20702=CARTESIAN_POINT('Ctrl Pts',(7.22595032355027,-41.4765530373371,-10.749241966903));
#20703=CARTESIAN_POINT('Ctrl Pts',(6.99532253008204,-41.4810624893143,-10.7838654920941));
#20704=CARTESIAN_POINT('Ctrl Pts',(6.53847566308335,-41.5511755542865,-10.7881590891358));
#20705=CARTESIAN_POINT('Ctrl Pts',(6.31653527029745,-41.6161129892238,-10.7577973127683));
#20706=CARTESIAN_POINT('Ctrl Pts',(5.93425477237866,-41.7881548523286,-10.643014679065));
#20707=CARTESIAN_POINT('Ctrl Pts',(5.7724971039899,-41.888085776068,-10.5663096368503));
#20708=CARTESIAN_POINT('Ctrl Pts',(5.6350165713459,-42.0034439406511,-10.4702558451003));
#20709=CARTESIAN_POINT('',(5.52082649506268,-43.1482383743695,-9.34999999999999));
#20710=CARTESIAN_POINT('Ctrl Pts',(5.63501657134564,-42.0034439406514,-10.4702558450999));
#20711=CARTESIAN_POINT('Ctrl Pts',(5.62715392638841,-42.2104953408534,-10.2660883608659));
#20712=CARTESIAN_POINT('Ctrl Pts',(5.61233201610448,-42.4176334360682,-10.0627168613273));
#20713=CARTESIAN_POINT('Ctrl Pts',(5.59056965525696,-42.6248274931923,-9.86011239009003));
#20714=CARTESIAN_POINT('Ctrl Pts',(5.57224784970726,-42.7992648739654,-9.68953899727123));
#20715=CARTESIAN_POINT('Ctrl Pts',(5.5490057889544,-42.9737421348353,-9.5195087895747));
#20716=CARTESIAN_POINT('Ctrl Pts',(5.52082649506267,-43.1482383743695,-9.34999999999999));
#20717=CARTESIAN_POINT('',(2.25553370726644,-43.4414844094374,-9.34999999999999));
#20718=CARTESIAN_POINT('Origin',(-3.46944695195361E-15,3.46944695195361E-15,
-9.34999999999999));
#20719=CARTESIAN_POINT('',(1.97901608230067,-42.3549304887752,-10.4488603766009));
#20720=CARTESIAN_POINT('Ctrl Pts',(2.25553370726645,-43.4414844094374,-9.34999999999999));
#20721=CARTESIAN_POINT('Ctrl Pts',(2.19128710278197,-43.2405563700915,-9.55398902691157));
#20722=CARTESIAN_POINT('Ctrl Pts',(2.13411262165437,-43.0385015627268,-9.75864153760641));
#20723=CARTESIAN_POINT('Ctrl Pts',(2.08399176105578,-42.8353507457784,-9.96398744092143));
#20724=CARTESIAN_POINT('Ctrl Pts',(2.04464794759835,-42.6758816594482,-10.1251796235333));
#20725=CARTESIAN_POINT('Ctrl Pts',(2.00965153883474,-42.5157369286965,-10.28679931628));
#20726=CARTESIAN_POINT('Ctrl Pts',(1.97901608230068,-42.3549304887753,-10.4488603766009));
#20727=CARTESIAN_POINT('',(-0.400053103665653,-42.3778559173192,-10.4702558450996));
#20728=CARTESIAN_POINT('Ctrl Pts',(1.97901608230066,-42.3549304887753,-10.4488603766009));
#20729=CARTESIAN_POINT('Ctrl Pts',(1.82650736151775,-42.2633979223932,-10.5474113291179));
#20730=CARTESIAN_POINT('Ctrl Pts',(1.65235205445741,-42.1909339439257,-10.6271346460647));
#20731=CARTESIAN_POINT('Ctrl Pts',(1.24967162819108,-42.0827414829252,-10.749241967384));
#20732=CARTESIAN_POINT('Ctrl Pts',(1.02074953110195,-42.0543832782663,-10.7838654923523));
#20733=CARTESIAN_POINT('Ctrl Pts',(0.558574576988531,-42.0587666057809,
-10.7881590889248));
#20734=CARTESIAN_POINT('Ctrl Pts',(0.329651656930575,-42.0914576603666,
-10.7577973123328));
#20735=CARTESIAN_POINT('Ctrl Pts',(-0.0732218856486514,-42.2073441982801,
-10.6430146784578));
#20736=CARTESIAN_POINT('Ctrl Pts',(-0.247554746683549,-42.2832374526635,
-10.5663096364682));
#20737=CARTESIAN_POINT('Ctrl Pts',(-0.400053103665666,-42.3778559173188,
-10.4702558451));
#20738=CARTESIAN_POINT('',(-0.676002124309578,-43.4947470521203,-9.34999999999999));
#20739=CARTESIAN_POINT('Ctrl Pts',(-0.400053103665649,-42.3778559173192,
-10.4702558450996));
#20740=CARTESIAN_POINT('Ctrl Pts',(-0.437302204927433,-42.5816808626376,
-10.2660883599915));
#20741=CARTESIAN_POINT('Ctrl Pts',(-0.481452074275132,-42.7846012138114,
-10.0627168595858));
#20742=CARTESIAN_POINT('Ctrl Pts',(-0.532479714674941,-42.9865892281722,
-9.86011238749097));
#20743=CARTESIAN_POINT('Ctrl Pts',(-0.575440058127383,-43.1566436222658,
-9.6895389955411));
#20744=CARTESIAN_POINT('Ctrl Pts',(-0.623276251159064,-43.326037265215,
-9.51950878871019));
#20745=CARTESIAN_POINT('Ctrl Pts',(-0.676002124309579,-43.4947470521204,
-9.34999999999999));
#20746=CARTESIAN_POINT('',(-3.9497922017429,-43.3203086503669,-9.34999999999999));
#20747=CARTESIAN_POINT('Origin',(-3.46944695195361E-15,3.46944695195361E-15,
-9.34999999999999));
#20748=CARTESIAN_POINT('',(-4.06886253049728,-42.2054617208604,-10.4488603765996));
#20749=CARTESIAN_POINT('Ctrl Pts',(-3.94979220174291,-43.3203086503669,
-9.34999999999999));
#20750=CARTESIAN_POINT('Ctrl Pts',(-3.98478982700535,-43.1122825236215,
-9.55398902691055));
#20751=CARTESIAN_POINT('Ctrl Pts',(-4.01262695712122,-42.9041475658228,
-9.75864153760437));
#20752=CARTESIAN_POINT('Ctrl Pts',(-4.03332628396802,-42.6959315891025,
-9.96398744091835));
#20753=CARTESIAN_POINT('Ctrl Pts',(-4.04957481690293,-42.5324864596859,
-10.1251796235308));
#20754=CARTESIAN_POINT('Ctrl Pts',(-4.06142404122876,-42.3689912631297,
-10.2867993162781));
#20755=CARTESIAN_POINT('Ctrl Pts',(-4.06886253049727,-42.2054617208604,
-10.4488603765996));
#20756=CARTESIAN_POINT('',(-6.42697885114042,-41.8895769551537,-10.4702558451003));
#20757=CARTESIAN_POINT('Ctrl Pts',(-4.06886253049729,-42.2054617208604,
-10.4488603765996));
#20758=CARTESIAN_POINT('Ctrl Pts',(-4.20679249002057,-42.0931565700915,
-10.5474113291167));
#20759=CARTESIAN_POINT('Ctrl Pts',(-4.36886244778991,-41.9966452860815,
-10.6271346460636));
#20760=CARTESIAN_POINT('Ctrl Pts',(-4.75204677534415,-41.8322466685932,
-10.7492419673832));
#20761=CARTESIAN_POINT('Ctrl Pts',(-4.97460298225344,-41.771598098344,-10.7838654923517));
#20762=CARTESIAN_POINT('Ctrl Pts',(-5.43269747428145,-41.7101624560557,
-10.7881590889246));
#20763=CARTESIAN_POINT('Ctrl Pts',(-5.66394271123907,-41.7099416344971,
-10.7577973123328));
#20764=CARTESIAN_POINT('Ctrl Pts',(-6.07920795595195,-41.7673137314921,
-10.6430146784582));
#20765=CARTESIAN_POINT('Ctrl Pts',(-6.2625670960526,-41.817624349051,-10.5663096364686));
#20766=CARTESIAN_POINT('Ctrl Pts',(-6.42697885114042,-41.8895769551538,
-10.4702558451003));
#20767=CARTESIAN_POINT('',(-6.85906928985839,-42.9558281083827,-9.34999999999999));
#20768=CARTESIAN_POINT('Ctrl Pts',(-6.42697885114041,-41.8895769551537,
-10.4702558451003));
#20769=CARTESIAN_POINT('Ctrl Pts',(-6.49285612438891,-42.0860261565974,
-10.2660883599931));
#20770=CARTESIAN_POINT('Ctrl Pts',(-6.56543518868484,-42.2805978896664,
-10.0627168595883));
#20771=CARTESIAN_POINT('Ctrl Pts',(-6.64468933287768,-42.4732679668919,
-9.86011238749433));
#20772=CARTESIAN_POINT('Ctrl Pts',(-6.71141366557098,-42.6354775581222,
-9.68953899554333));
#20773=CARTESIAN_POINT('Ctrl Pts',(-6.78287018403301,-42.7963392179579,
-9.51950878871131));
#20774=CARTESIAN_POINT('Ctrl Pts',(-6.85906928985838,-42.9558281083827,
-9.34999999999999));
#20775=CARTESIAN_POINT('',(-10.074711731795,-42.3172563326267,-9.34999999999999));
#20776=CARTESIAN_POINT('Origin',(-3.46944695195361E-15,3.46944695195361E-15,
-9.34999999999999));
#20777=CARTESIAN_POINT('',(-10.0339108358238,-41.1968114627984,-10.4488603766053));
#20778=CARTESIAN_POINT('Ctrl Pts',(-10.074711731795,-42.3172563326267,-9.34999999999999));
#20779=CARTESIAN_POINT('Ctrl Pts',(-10.0797479271121,-42.1063669305242,
-9.55398902690942));
#20780=CARTESIAN_POINT('Ctrl Pts',(-10.0776810225247,-41.8963888498204,
-9.75864153760213));
#20781=CARTESIAN_POINT('Ctrl Pts',(-10.0685374370191,-41.6873463901686,
-9.96398744091504));
#20782=CARTESIAN_POINT('Ctrl Pts',(-10.0613599161589,-41.5232524891608,
-10.1251796235305));
#20783=CARTESIAN_POINT('Ctrl Pts',(-10.0498207400108,-41.359735117518,-10.2867993162807));
#20784=CARTESIAN_POINT('Ctrl Pts',(-10.0339108358238,-41.1968114627984,
-10.4488603766053));
#20785=CARTESIAN_POINT('',(-12.3230698431045,-40.5485470057458,-10.470255845095));
#20786=CARTESIAN_POINT('Ctrl Pts',(-10.0339108358244,-41.1968114627986,
-10.4488603766049));
#20787=CARTESIAN_POINT('Ctrl Pts',(-10.1544541778703,-41.0660199366513,
-10.5474113291217));
#20788=CARTESIAN_POINT('Ctrl Pts',(-10.3011395093808,-40.947426038526,-10.6271346460681));
#20789=CARTESIAN_POINT('Ctrl Pts',(-10.657027210328,-40.7301679463169,-10.749241967386));
#20790=CARTESIAN_POINT('Ctrl Pts',(-10.8686869244842,-40.6384636404728,
-10.7838654923534));
#20791=CARTESIAN_POINT('Ctrl Pts',(-11.3133754716045,-40.5124596808953,
-10.7881590889241));
#20792=CARTESIAN_POINT('Ctrl Pts',(-11.5422355392933,-40.4793314784837,
-10.7577973123312));
#20793=CARTESIAN_POINT('Ctrl Pts',(-11.961438883283,-40.4770212041149,-10.6430146784548));
#20794=CARTESIAN_POINT('Ctrl Pts',(-12.1500916391208,-40.5007250057605,
-10.5663096364642));
#20795=CARTESIAN_POINT('Ctrl Pts',(-12.3230698431046,-40.5485470057456,
-10.4702558450952));
#20796=CARTESIAN_POINT('',(-12.9025055845987,-41.5424523787343,-9.34999999999999));
#20797=CARTESIAN_POINT('Ctrl Pts',(-12.3230698431044,-40.5485470057458,
-10.470255845095));
#20798=CARTESIAN_POINT('Ctrl Pts',(-12.4162342170306,-40.7336213240895,
-10.2660883599853));
#20799=CARTESIAN_POINT('Ctrl Pts',(-12.5157649758266,-40.9158835196705,
-10.062716859578));
#20800=CARTESIAN_POINT('Ctrl Pts',(-12.6216322379871,-41.0953134526064,
-9.86011238748152));
#20801=CARTESIAN_POINT('Ctrl Pts',(-12.7107622449211,-41.2463761214653,
-9.68953899553485));
#20802=CARTESIAN_POINT('Ctrl Pts',(-12.8043844401572,-41.3954311186753,
-9.51950878870709));
#20803=CARTESIAN_POINT('Ctrl Pts',(-12.9025055845986,-41.5424523787343,
-9.34999999999999));
#20804=CARTESIAN_POINT('',(-15.9945391840253,-40.4527467088538,-9.34999999999999));
#20805=CARTESIAN_POINT('Origin',(-3.46944695195361E-15,3.46944695195361E-15,
-9.34999999999999));
#20806=CARTESIAN_POINT('',(-15.7946976518867,-39.3495129251816,-10.4488603765943));
#20807=CARTESIAN_POINT('Ctrl Pts',(-15.9945391840253,-40.4527467088538,
-9.34999999999999));
#20808=CARTESIAN_POINT('Ctrl Pts',(-15.9695114269777,-40.2432871314623,
-9.55398902691376));
#20809=CARTESIAN_POINT('Ctrl Pts',(-15.9375825638984,-40.0357404760457,
-9.75864153761077));
#20810=CARTESIAN_POINT('Ctrl Pts',(-15.8987822030673,-39.8301270351085,
-9.96398744092793));
#20811=CARTESIAN_POINT('Ctrl Pts',(-15.8683247420356,-39.6687248411385,
-10.1251796235355));
#20812=CARTESIAN_POINT('Ctrl Pts',(-15.8336320697617,-39.5085140365627,
-10.2867993162778));
#20813=CARTESIAN_POINT('Ctrl Pts',(-15.7946976518867,-39.3495129251816,
-10.4488603765943));
#20814=CARTESIAN_POINT('',(-17.9682986697937,-38.3820655716606,-10.4702558451073));
#20815=CARTESIAN_POINT('Ctrl Pts',(-15.7946976518867,-39.3495129251816,
-10.4488603765943));
#20816=CARTESIAN_POINT('Ctrl Pts',(-15.8954004612252,-39.2028975625402,
-10.5474113287197));
#20817=CARTESIAN_POINT('Ctrl Pts',(-16.0237150755117,-39.0646352805812,
-10.6271346454281));
#20818=CARTESIAN_POINT('Ctrl Pts',(-16.345061301575,-38.7989404621477,-10.7492419669021));
#20819=CARTESIAN_POINT('Ctrl Pts',(-16.5415157414016,-38.6780472557653,
-10.7838654920944));
#20820=CARTESIAN_POINT('Ctrl Pts',(-16.9637457669869,-38.4900400557429,
-10.7881590891384));
#20821=CARTESIAN_POINT('Ctrl Pts',(-17.1855617344036,-38.4246788669136,
-10.7577973127721));
#20822=CARTESIAN_POINT('Ctrl Pts',(-17.600169407316,-38.3627332511513,-10.6430146790707));
#20823=CARTESIAN_POINT('Ctrl Pts',(-17.7902753536106,-38.3593476957178,
-10.5663096368568));
#20824=CARTESIAN_POINT('Ctrl Pts',(-17.9682986697938,-38.3820655716606,
-10.4702558451073));
#20825=CARTESIAN_POINT('',(-18.6832840733583,-39.2833921172065,-9.34999999999999));
#20826=CARTESIAN_POINT('Ctrl Pts',(-17.9682986697937,-38.3820655716606,
-10.4702558451073));
#20827=CARTESIAN_POINT('Ctrl Pts',(-18.0868535858997,-38.5519974267554,
-10.2660883608794));
#20828=CARTESIAN_POINT('Ctrl Pts',(-18.2113098794098,-38.718239751441,-10.062716861347));
#20829=CARTESIAN_POINT('Ctrl Pts',(-18.3416351067682,-38.8807768634145,
-9.8601123901159));
#20830=CARTESIAN_POINT('Ctrl Pts',(-18.4513563585572,-39.0176174103246,
-9.6895389972884));
#20831=CARTESIAN_POINT('Ctrl Pts',(-18.5652383532269,-39.1518314157116,
-9.51950878958326));
#20832=CARTESIAN_POINT('Ctrl Pts',(-18.6832840733583,-39.2833921172065,
-9.34999999999999));
#20833=CARTESIAN_POINT('',(-21.5887639429553,-37.7647358181592,-9.34999999999999));
#20834=CARTESIAN_POINT('Origin',(-3.46944695195361E-15,3.46944695195361E-15,
-9.34999999999999));
#20835=CARTESIAN_POINT('',(-21.2339499719768,-36.7011717789787,-10.4488603766065));
#20836=CARTESIAN_POINT('Ctrl Pts',(-21.5887639429553,-37.7647358181592,
-9.34999999999999));
#20837=CARTESIAN_POINT('Ctrl Pts',(-21.5341817265107,-37.5609700584485,
-9.55398902690961));
#20838=CARTESIAN_POINT('Ctrl Pts',(-21.4730408845247,-37.360079879714,-9.75864153760252));
#20839=CARTESIAN_POINT('Ctrl Pts',(-21.4053736118321,-37.162081154214,-9.96398744091563));
#20840=CARTESIAN_POINT('Ctrl Pts',(-21.3522562367057,-37.0066563504876,
-10.1251796235313));
#20841=CARTESIAN_POINT('Ctrl Pts',(-21.2951163110693,-36.8530135429323,
-10.2867993162817));
#20842=CARTESIAN_POINT('Ctrl Pts',(-21.2339499719768,-36.7011717789787,
-10.4488603766065));
#20843=CARTESIAN_POINT('',(-23.2477447519539,-35.434235967255,-10.4702558450962));
#20844=CARTESIAN_POINT('Ctrl Pts',(-21.2339499719768,-36.7011717789787,
-10.4488603766064));
#20845=CARTESIAN_POINT('Ctrl Pts',(-21.3127622306114,-36.5417172446673,
-10.547411329123));
#20846=CARTESIAN_POINT('Ctrl Pts',(-21.4200940133834,-36.3866011992051,
-10.6271346460693));
#20847=CARTESIAN_POINT('Ctrl Pts',(-21.7003570840256,-36.0778784343334,
-10.7492419673871));
#20848=CARTESIAN_POINT('Ctrl Pts',(-21.877607003997,-35.9302573647762,-10.7838654923545));
#20849=CARTESIAN_POINT('Ctrl Pts',(-22.2687831227019,-35.6840742095356,
-10.7881590889251));
#20850=CARTESIAN_POINT('Ctrl Pts',(-22.4790394564213,-35.5878106000643,
-10.7577973123323));
#20851=CARTESIAN_POINT('Ctrl Pts',(-22.8806112399902,-35.4674906781017,
-10.6430146784558));
#20852=CARTESIAN_POINT('Ctrl Pts',(-23.0683003663139,-35.4370846859713,
-10.5663096364652));
#20853=CARTESIAN_POINT('Ctrl Pts',(-23.2477447519539,-35.434235967255,-10.4702558450962));
#20854=CARTESIAN_POINT('',(-24.0837247765703,-36.2246352760993,-9.34999999999999));
#20855=CARTESIAN_POINT('Ctrl Pts',(-23.2477447519539,-35.434235967255,-10.4702558450962));
#20856=CARTESIAN_POINT('Ctrl Pts',(-23.3892767750413,-35.5855660380308,
-10.2660883599847));
#20857=CARTESIAN_POINT('Ctrl Pts',(-23.5361250331426,-35.7324042788876,
-10.0627168595755));
#20858=CARTESIAN_POINT('Ctrl Pts',(-23.6882551811027,-35.8747397843426,
-9.86011238747722));
#20859=CARTESIAN_POINT('Ctrl Pts',(-23.816334068434,-35.9945725289423,-9.68953899553199));
#20860=CARTESIAN_POINT('Ctrl Pts',(-23.9481575524104,-36.1112133310054,
-9.51950878870566));
#20861=CARTESIAN_POINT('Ctrl Pts',(-24.0837247765702,-36.2246352760993,
-9.34999999999999));
#20862=CARTESIAN_POINT('',(-26.7435037248304,-34.3079438107268,-9.34999999999999));
#20863=CARTESIAN_POINT('Origin',(-3.46944695195361E-15,3.46944695195361E-15,
-9.34999999999999));
#20864=CARTESIAN_POINT('',(-26.2409403042445,-33.3057006128373,-10.4488603766022));
#20865=CARTESIAN_POINT('Ctrl Pts',(-26.7435037248304,-34.3079438107268,
-9.34999999999999));
#20866=CARTESIAN_POINT('Ctrl Pts',(-26.6604781855069,-34.1140199519479,
-9.55398902691263));
#20867=CARTESIAN_POINT('Ctrl Pts',(-26.5713700158347,-33.9238757946104,
-9.75864153760855));
#20868=CARTESIAN_POINT('Ctrl Pts',(-26.4762133418097,-33.7375224676132,
-9.96398744092467));
#20869=CARTESIAN_POINT('Ctrl Pts',(-26.4015173691683,-33.59123905494,-10.1251796235359));
#20870=CARTESIAN_POINT('Ctrl Pts',(-26.3230933942782,-33.4472919689115,
-10.2867993162819));
#20871=CARTESIAN_POINT('Ctrl Pts',(-26.2409403042445,-33.3057006128373,
-10.4488603766022));
#20872=CARTESIAN_POINT('',(-28.053933791861,-31.7650675024729,-10.4702558451));
#20873=CARTESIAN_POINT('Ctrl Pts',(-26.2409403042452,-33.3057006128373,
-10.4488603766018));
#20874=CARTESIAN_POINT('Ctrl Pts',(-26.2962576214615,-33.1366529419292,
-10.547411329119));
#20875=CARTESIAN_POINT('Ctrl Pts',(-26.3804216065202,-32.9678408488439,
-10.627134646066));
#20876=CARTESIAN_POINT('Ctrl Pts',(-26.6138961728537,-32.6223748430043,
-10.7492419673853));
#20877=CARTESIAN_POINT('Ctrl Pts',(-26.7683332755725,-32.4510310493881,
-10.7838654923535));
#20878=CARTESIAN_POINT('Ctrl Pts',(-27.1204922694935,-32.1516835176302,
-10.7881590889259));
#20879=CARTESIAN_POINT('Ctrl Pts',(-27.3149087568863,-32.0264771367729,
-10.7577973123339));
#20880=CARTESIAN_POINT('Ctrl Pts',(-27.6952698084817,-31.8502322746937,
-10.6430146784589));
#20881=CARTESIAN_POINT('Ctrl Pts',(-27.8767213062725,-31.7934248240622,
-10.5663096364688));
#20882=CARTESIAN_POINT('Ctrl Pts',(-28.053933791861,-31.765067502473,-10.4702558451));
#20883=CARTESIAN_POINT('',(-28.9938902950281,-32.4284493240099,-9.34999999999999));
#20884=CARTESIAN_POINT('Ctrl Pts',(-28.053933791861,-31.7650675024729,-10.4702558451));
#20885=CARTESIAN_POINT('Ctrl Pts',(-28.2155617375712,-31.8947151443484,
-10.2660883599931));
#20886=CARTESIAN_POINT('Ctrl Pts',(-28.3818125526395,-32.0191600975308,
-10.0627168595884));
#20887=CARTESIAN_POINT('Ctrl Pts',(-28.5526506894832,-32.1383964553645,
-9.86011238749472));
#20888=CARTESIAN_POINT('Ctrl Pts',(-28.696479896089,-32.2387819492749,-9.68953899554359));
#20889=CARTESIAN_POINT('Ctrl Pts',(-28.8435613239597,-32.3354750783552,
-9.51950878871143));
#20890=CARTESIAN_POINT('Ctrl Pts',(-28.9938902950281,-32.4284493240099,
-9.34999999999999));
#20891=CARTESIAN_POINT('',(-31.3538228927626,-30.1527410032535,-9.34999999999999));
#20892=CARTESIAN_POINT('Origin',(-3.46944695195361E-15,3.46944695195361E-15,
-9.34999999999999));
#20893=CARTESIAN_POINT('',(-30.7137407645416,-29.2322214279374,-10.4488603765957));
#20894=CARTESIAN_POINT('Ctrl Pts',(-31.3538228927626,-30.1527410032535,
-9.34999999999999));
#20895=CARTESIAN_POINT('Ctrl Pts',(-31.2440441911153,-29.9726067759439,
-9.55398902691338));
#20896=CARTESIAN_POINT('Ctrl Pts',(-31.1287826791253,-29.7970794267192,
-9.75864153761002));
#20897=CARTESIAN_POINT('Ctrl Pts',(-31.0080737192424,-29.6261651145667,
-9.96398744092682));
#20898=CARTESIAN_POINT('Ctrl Pts',(-30.913319743684,-29.4920010013807,-10.1251796235352));
#20899=CARTESIAN_POINT('Ctrl Pts',(-30.8152082055132,-29.3606799844397,
-10.2867993162784));
#20900=CARTESIAN_POINT('Ctrl Pts',(-30.7137407645416,-29.2322214279374,
-10.4488603765957));
#20901=CARTESIAN_POINT('',(-32.2890256406275,-27.4492538662411,-10.4702558451039));
#20902=CARTESIAN_POINT('Ctrl Pts',(-30.7137407645416,-29.2322214279374,
-10.4488603765957));
#20903=CARTESIAN_POINT('Ctrl Pts',(-30.7444370392829,-29.0570219435195,
-10.5474113291135));
#20904=CARTESIAN_POINT('Ctrl Pts',(-30.8037198906013,-28.8779503302129,
-10.6271346460612));
#20905=CARTESIAN_POINT('Ctrl Pts',(-30.9856530837404,-28.5027737750429,
-10.7492419673821));
#20906=CARTESIAN_POINT('Ctrl Pts',(-31.114133475155,-28.3111953228912,-10.7838654923513));
#20907=CARTESIAN_POINT('Ctrl Pts',(-31.4201064027185,-27.9647772671156,
-10.7881590889256));
#20908=CARTESIAN_POINT('Ctrl Pts',(-31.5947252847521,-27.8131769557209,
-10.7577973123346));
#20909=CARTESIAN_POINT('Ctrl Pts',(-31.9461325502338,-27.5845949906688,
-10.6430146784613));
#20910=CARTESIAN_POINT('Ctrl Pts',(-32.1176525902589,-27.5025425174118,
-10.566309636472));
#20911=CARTESIAN_POINT('Ctrl Pts',(-32.2890256406275,-27.4492538662411,
-10.4702558451039));
#20912=CARTESIAN_POINT('',(-33.3138238185527,-27.9721136596152,-9.34999999999999));
#20913=CARTESIAN_POINT('Ctrl Pts',(-32.2890256406275,-27.4492538662411,
-10.4702558451039));
#20914=CARTESIAN_POINT('Ctrl Pts',(-32.4674592300822,-27.5545798271016,
-10.2660883600008));
#20915=CARTESIAN_POINT('Ctrl Pts',(-32.6497282149504,-27.6540981522332,
-10.0627168596001));
#20916=CARTESIAN_POINT('Ctrl Pts',(-32.8357965688679,-27.7478080540501,
-9.8601123875103));
#20917=CARTESIAN_POINT('Ctrl Pts',(-32.9924481468715,-27.826702738101,-9.68953899555392));
#20918=CARTESIAN_POINT('Ctrl Pts',(-33.1517933649134,-27.901479800928,-9.51950878871657));
#20919=CARTESIAN_POINT('Ctrl Pts',(-33.3138238185527,-27.9721136596152,
-9.34999999999999));
#20920=CARTESIAN_POINT('',(-35.3258686435787,-25.3837153422549,-9.34999999999999));
#20921=CARTESIAN_POINT('Origin',(-3.46944695195361E-15,3.46944695195361E-15,
-9.34999999999999));
#20922=CARTESIAN_POINT('',(-34.561298034014,-24.5636585134826,-10.4488603766016));
#20923=CARTESIAN_POINT('Ctrl Pts',(-35.3258686435787,-25.3837153422549,
-9.34999999999999));
#20924=CARTESIAN_POINT('Ctrl Pts',(-35.191571557402,-25.2210377598177,-9.5539890269114));
#20925=CARTESIAN_POINT('Ctrl Pts',(-35.0525030950958,-25.0637004493564,
-9.75864153760609));
#20926=CARTESIAN_POINT('Ctrl Pts',(-34.9086991356865,-24.9117044745671,
-9.96398744092097));
#20927=CARTESIAN_POINT('Ctrl Pts',(-34.7958160749033,-24.7923908553078,
-10.1251796235332));
#20928=CARTESIAN_POINT('Ctrl Pts',(-34.6800142414361,-24.6763692246536,
-10.2867993162803));
#20929=CARTESIAN_POINT('Ctrl Pts',(-34.561298034014,-24.5636585134826,-10.4488603766016));
#20930=CARTESIAN_POINT('',(-35.8668060412545,-22.5746525783676,-10.4702558450978));
#20931=CARTESIAN_POINT('Ctrl Pts',(-34.5612980340131,-24.5636585134822,
-10.4488603766026));
#20932=CARTESIAN_POINT('Ctrl Pts',(-34.5667483786485,-24.3858737718227,
-10.5474113291198));
#20933=CARTESIAN_POINT('Ctrl Pts',(-34.5999432683334,-24.2001880199414,
-10.6271346460667));
#20934=CARTESIAN_POINT('Ctrl Pts',(-34.7266314531219,-23.8029384281848,
-10.7492419673853));
#20935=CARTESIAN_POINT('Ctrl Pts',(-34.8265396429719,-23.5950253023176,
-10.7838654923531));
#20936=CARTESIAN_POINT('Ctrl Pts',(-35.0800977777285,-23.2085887951553,
-10.7881590889248));
#20937=CARTESIAN_POINT('Ctrl Pts',(-35.2313643175252,-23.0336806983859,
-10.7577973123324));
#20938=CARTESIAN_POINT('Ctrl Pts',(-35.546664158344,-22.7574148999972,-10.6430146784568));
#20939=CARTESIAN_POINT('Ctrl Pts',(-35.7047610872118,-22.6517877558527,
-10.5663096364666));
#20940=CARTESIAN_POINT('Ctrl Pts',(-35.8668060412538,-22.5746525783687,
-10.4702558450978));
#20941=CARTESIAN_POINT('',(-36.955583958287,-22.946346426,-9.34999999999999));
#20942=CARTESIAN_POINT('Ctrl Pts',(-35.8668060412545,-22.5746525783676,
-10.4702558450978));
#20943=CARTESIAN_POINT('Ctrl Pts',(-36.0584128811371,-22.6535127253913,
-10.2660883599907));
#20944=CARTESIAN_POINT('Ctrl Pts',(-36.2529895648988,-22.7260785163657,
-10.062716859586));
#20945=CARTESIAN_POINT('Ctrl Pts',(-36.4505003207866,-22.7923542988078,
-9.86011238749218));
#20946=CARTESIAN_POINT('Ctrl Pts',(-36.6167852957936,-22.8481521047421,
-9.68953899554191));
#20947=CARTESIAN_POINT('Ctrl Pts',(-36.7851504948685,-22.8994908559535,
-9.5195087887106));
#20948=CARTESIAN_POINT('Ctrl Pts',(-36.955583958287,-22.946346426,-9.34999999999999));
#20949=CARTESIAN_POINT('',(-38.5787815801808,-20.0979504375124,-9.34999999999999));
#20950=CARTESIAN_POINT('Origin',(-3.46944695195361E-15,3.46944695195361E-15,
-9.34999999999999));
#20951=CARTESIAN_POINT('',(-37.7052869420397,-19.3950503475036,-10.4488603765919));
#20952=CARTESIAN_POINT('Ctrl Pts',(-38.5787815801808,-20.0979504375124,
-9.34999999999999));
#20953=CARTESIAN_POINT('Ctrl Pts',(-38.4227000108615,-19.9560411464038,
-9.55398902691458));
#20954=CARTESIAN_POINT('Ctrl Pts',(-38.2626556310847,-19.8200968086245,
-9.75864153761241));
#20955=CARTESIAN_POINT('Ctrl Pts',(-38.0986841060596,-19.6901133709261,
-9.96398744093037));
#20956=CARTESIAN_POINT('Ctrl Pts',(-37.9699699336463,-19.5880791268205,
-10.1251796235364));
#20957=CARTESIAN_POINT('Ctrl Pts',(-37.8388351962726,-19.4897187482847,
-10.2867993162771));
#20958=CARTESIAN_POINT('Ctrl Pts',(-37.7052869420397,-19.3950503475036,
-10.4488603765919));
#20959=CARTESIAN_POINT('',(-38.7144417021568,-17.2404964639775,-10.4702558451079));
#20960=CARTESIAN_POINT('Ctrl Pts',(-37.70528694204,-19.3950503475025,-10.4488603765922));
#20961=CARTESIAN_POINT('Ctrl Pts',(-37.6853804032671,-19.2182995332542,
-10.5474113291108));
#20962=CARTESIAN_POINT('Ctrl Pts',(-37.6918115790876,-19.0297796692338,
-10.6271346460593));
#20963=CARTESIAN_POINT('Ctrl Pts',(-37.7606757494155,-18.6185438970059,
-10.7492419673815));
#20964=CARTESIAN_POINT('Ctrl Pts',(-37.829977895064,-18.3985286090935,-10.7838654923512));
#20965=CARTESIAN_POINT('Ctrl Pts',(-38.0259595245863,-17.9799403834372,
-10.7881590889269));
#20966=CARTESIAN_POINT('Ctrl Pts',(-38.1507943716101,-17.785285125748,-10.7577973123366));
#20967=CARTESIAN_POINT('Ctrl Pts',(-38.423568192254,-17.4669594689877,-10.6430146784646));
#20968=CARTESIAN_POINT('Ctrl Pts',(-38.5650236124062,-17.3399079180034,
-10.5663096364759));
#20969=CARTESIAN_POINT('Ctrl Pts',(-38.7144417021566,-17.2404964639768,
-10.4702558451083));
#20970=CARTESIAN_POINT('',(-39.845034979713,-17.4534577509859,-9.34999999999999));
#20971=CARTESIAN_POINT('Ctrl Pts',(-38.7144417021568,-17.2404964639775,
-10.4702558451079));
#20972=CARTESIAN_POINT('Ctrl Pts',(-38.9153212297535,-17.2912854319784,
-10.2660883600021));
#20973=CARTESIAN_POINT('Ctrl Pts',(-39.1182445922376,-17.3354214585475,
-10.0627168595987));
#20974=CARTESIAN_POINT('Ctrl Pts',(-39.323177000677,-17.3729139378015,-9.8601123875063));
#20975=CARTESIAN_POINT('Ctrl Pts',(-39.4957102901352,-17.4044789831982,
-9.68953899555125));
#20976=CARTESIAN_POINT('Ctrl Pts',(-39.6696680403279,-17.4313343138675,
-9.51950878871524));
#20977=CARTESIAN_POINT('Ctrl Pts',(-39.845034979713,-17.4534577509859,-9.34999999999999));
#20978=CARTESIAN_POINT('',(-41.0463417758467,-14.4030492195362,-9.34999999999999));
#20979=CARTESIAN_POINT('Origin',(-3.46944695195361E-15,3.46944695195361E-15,
-9.34999999999999));
#20980=CARTESIAN_POINT('',(-40.0817049410149,-13.8316148870952,-10.4488603765949));
#20981=CARTESIAN_POINT('Ctrl Pts',(-41.0463417758468,-14.4030492195362,
-9.34999999999999));
#20982=CARTESIAN_POINT('Ctrl Pts',(-40.871653094042,-14.2847970836902,-9.55398902691117));
#20983=CARTESIAN_POINT('Ctrl Pts',(-40.6938908388447,-14.1730131532785,
-9.75864153760559));
#20984=CARTESIAN_POINT('Ctrl Pts',(-40.5130897356062,-14.0676883406206,
-9.96398744092016));
#20985=CARTESIAN_POINT('Ctrl Pts',(-40.371164700926,-13.9850105946256,-10.1251796235305));
#20986=CARTESIAN_POINT('Ctrl Pts',(-40.2273665847308,-13.9063138018573,
-10.2867993162756));
#20987=CARTESIAN_POINT('Ctrl Pts',(-40.081704941015,-13.8316148870952,-10.4488603765949));
#20988=CARTESIAN_POINT('',(-40.7739629732767,-11.5553735590169,-10.4702558451026));
#20989=CARTESIAN_POINT('Ctrl Pts',(-40.0817049410152,-13.831614887095,-10.4488603765947));
#20990=CARTESIAN_POINT('Ctrl Pts',(-40.0368467585607,-13.6594961371281,
-10.5474113291124));
#20991=CARTESIAN_POINT('Ctrl Pts',(-40.0163833003259,-13.4719798817537,
-10.6271346460599));
#20992=CARTESIAN_POINT('Ctrl Pts',(-40.0260215802783,-13.0551295034711,
-10.7492419673806));
#20993=CARTESIAN_POINT('Ctrl Pts',(-40.0633068898933,-12.8274909303035,
-10.7838654923497));
#20994=CARTESIAN_POINT('Ctrl Pts',(-40.1977223933732,-12.3852722353198,
-10.7881590889239));
#20995=CARTESIAN_POINT('Ctrl Pts',(-40.2935842701349,-12.1748324364192,
-10.7577973123328));
#20996=CARTESIAN_POINT('Ctrl Pts',(-40.5182791822329,-11.8209271136879,
-10.6430146784594));
#20997=CARTESIAN_POINT('Ctrl Pts',(-40.6402134692392,-11.6750375590585,
-10.5663096364703));
#20998=CARTESIAN_POINT('Ctrl Pts',(-40.7739629732768,-11.5553735590173,
-10.4702558451023));
#20999=CARTESIAN_POINT('',(-41.9233559925594,-11.6052670077487,-9.34999999999999));
#21000=CARTESIAN_POINT('Ctrl Pts',(-40.7739629732767,-11.5553735590169,
-10.4702558451026));
#21001=CARTESIAN_POINT('Ctrl Pts',(-40.9800258606916,-11.5770574310741,
-10.2660883599987));
#21002=CARTESIAN_POINT('Ctrl Pts',(-41.1871649674178,-11.5918652110192,
-10.0627168595972));
#21003=CARTESIAN_POINT('Ctrl Pts',(-41.3953471955466,-11.5998111483317,
-9.86011238750657));
#21004=CARTESIAN_POINT('Ctrl Pts',(-41.5706165192209,-11.6065008598948,
-9.68953899555145));
#21005=CARTESIAN_POINT('Ctrl Pts',(-41.7466255423837,-11.6083260729364,
-9.51950878871534));
#21006=CARTESIAN_POINT('Ctrl Pts',(-41.9233559925594,-11.6052670077487,
-9.34999999999999));
#21007=CARTESIAN_POINT('',(-42.6783168208273,-8.4149434544203,-9.34999999999999));
#21008=CARTESIAN_POINT('Origin',(-3.46944695195361E-15,3.46944695195361E-15,
-9.34999999999999));
#21009=CARTESIAN_POINT('',(-41.6421750134749,-7.98660763468004,-10.4488603765984));
#21010=CARTESIAN_POINT('Ctrl Pts',(-42.6783168208273,-8.41494345442029,
-9.34999999999999));
#21011=CARTESIAN_POINT('Ctrl Pts',(-42.4885771843355,-8.32275574631041,
-9.5539890269104));
#21012=CARTESIAN_POINT('Ctrl Pts',(-42.2967157806069,-8.23740782173034,
-9.75864153760406));
#21013=CARTESIAN_POINT('Ctrl Pts',(-42.102765688227,-8.15888574356603,-9.96398744091788));
#21014=CARTESIAN_POINT('Ctrl Pts',(-41.9505189757091,-8.09724757616996,
-10.1251796235301));
#21015=CARTESIAN_POINT('Ctrl Pts',(-41.7969847956598,-8.0398164089298,-10.2867993162772));
#21016=CARTESIAN_POINT('Ctrl Pts',(-41.6421750134748,-7.98660763468004,
-10.4488603765984));
#21017=CARTESIAN_POINT('',(-42.0034439406495,-5.63501657134773,-10.4702558451016));
#21018=CARTESIAN_POINT('Ctrl Pts',(-41.6421750134749,-7.98660763468003,
-10.4488603765984));
#21019=CARTESIAN_POINT('Ctrl Pts',(-41.5732783705724,-7.82262479039399,
-10.5474113291159));
#21020=CARTESIAN_POINT('Ctrl Pts',(-41.5263368552795,-7.63992943387202,
-10.6271346460633));
#21021=CARTESIAN_POINT('Ctrl Pts',(-41.4765530372705,-7.22595032113848,
-10.7492419673834));
#21022=CARTESIAN_POINT('Ctrl Pts',(-41.4810624894699,-6.99532252761,-10.783865492352));
#21023=CARTESIAN_POINT('Ctrl Pts',(-41.5511755548784,-6.53847566067517,
-10.7881590889253));
#21024=CARTESIAN_POINT('Ctrl Pts',(-41.6161129900097,-6.31653526801044,
-10.7577973123337));
#21025=CARTESIAN_POINT('Ctrl Pts',(-41.788154853118,-5.93425477109959,-10.6430146784595));
#21026=CARTESIAN_POINT('Ctrl Pts',(-41.8880857765248,-5.77249710344573,
-10.5663096364699));
#21027=CARTESIAN_POINT('Ctrl Pts',(-42.0034439406495,-5.63501657134772,
-10.4702558451016));
#21028=CARTESIAN_POINT('',(-43.1482383743694,-5.52082649506381,-9.34999999999999));
#21029=CARTESIAN_POINT('Ctrl Pts',(-42.0034439406495,-5.63501657134772,
-10.4702558451016));
#21030=CARTESIAN_POINT('Ctrl Pts',(-42.2104953417357,-5.62715392635674,
-10.2660883599956));
#21031=CARTESIAN_POINT('Ctrl Pts',(-42.4176334378355,-5.61233201597962,
-10.0627168595919));
#21032=CARTESIAN_POINT('Ctrl Pts',(-42.6248274958417,-5.59056965498014,
-9.86011238749915));
#21033=CARTESIAN_POINT('Ctrl Pts',(-42.799264875735,-5.57224784947292,-9.68953899554653));
#21034=CARTESIAN_POINT('Ctrl Pts',(-42.9737421357223,-5.54900578881237,
-9.5195087887129));
#21035=CARTESIAN_POINT('Ctrl Pts',(-43.1482383743694,-5.5208264950638,-9.34999999999999));
#21036=CARTESIAN_POINT('',(-43.4414844094373,-2.25553370726721,-9.34999999999999));
#21037=CARTESIAN_POINT('Origin',(-3.46944695195361E-15,3.46944695195361E-15,
-9.34999999999999));
#21038=CARTESIAN_POINT('',(-42.3549304887756,-1.97901608230199,-10.4488603766005));
#21039=CARTESIAN_POINT('Ctrl Pts',(-43.4414844094373,-2.25553370726721,
-9.34999999999999));
#21040=CARTESIAN_POINT('Ctrl Pts',(-43.2405563700911,-2.19128710278271,
-9.55398902691193));
#21041=CARTESIAN_POINT('Ctrl Pts',(-43.038501562726,-2.13411262165511,-9.75864153760715));
#21042=CARTESIAN_POINT('Ctrl Pts',(-42.8353507457773,-2.08399176105654,
-9.96398744092254));
#21043=CARTESIAN_POINT('Ctrl Pts',(-42.6758816594476,-2.04464794759932,
-10.1251796235339));
#21044=CARTESIAN_POINT('Ctrl Pts',(-42.5157369286964,-2.00965153883589,
-10.2867993162801));
#21045=CARTESIAN_POINT('Ctrl Pts',(-42.3549304887756,-1.97901608230198,
-10.4488603766005));
#21046=CARTESIAN_POINT('',(-42.1895973099932,-1.50796436832281E-9,-10.6604026900068));
#21047=CARTESIAN_POINT('Ctrl Pts',(-42.3549304887756,-1.979016082302,-10.4488603766005));
#21048=CARTESIAN_POINT('Ctrl Pts',(-42.2777622816011,-1.8504408109375,-10.531945562799));
#21049=CARTESIAN_POINT('Ctrl Pts',(-42.2140750286935,-1.7063561510611,-10.6017307219897));
#21050=CARTESIAN_POINT('Ctrl Pts',(-42.1138804087173,-1.38542074402617,
-10.7136554733245));
#21051=CARTESIAN_POINT('Ctrl Pts',(-42.0800627876842,-1.20890695927121,
-10.7529641474029));
#21052=CARTESIAN_POINT('Ctrl Pts',(-42.046111502818,-0.795598132330741,
-10.7969991342822));
#21053=CARTESIAN_POINT('Ctrl Pts',(-42.0583624188812,-0.559734595950683,
-10.7885243575832));
#21054=CARTESIAN_POINT('Ctrl Pts',(-42.1231209760754,-0.218323779409197,
-10.7264706453147));
#21055=CARTESIAN_POINT('Ctrl Pts',(-42.1526851017604,-0.106675909104108,
-10.697314898232));
#21056=CARTESIAN_POINT('Ctrl Pts',(-42.1895973099932,-3.01592865264988E-9,
-10.6604026900068));
#21057=CARTESIAN_POINT('',(-41.5,-1.612837264507E-15,-11.35));
#21058=CARTESIAN_POINT('',(-43.5,-1.85776662433645E-15,-9.34999999999999));
#21059=CARTESIAN_POINT('Origin',(-3.46944695195361E-15,1.73472347597681E-15,
-11.35));
#21060=CARTESIAN_POINT('',(-42.3778559173175,0.400053103664136,-10.4702558451013));
#21061=CARTESIAN_POINT('Ctrl Pts',(-42.1895973099932,-3.0159285715309E-9,
-10.6604026900068));
#21062=CARTESIAN_POINT('Ctrl Pts',(-42.1974267713527,0.0226270606221863,
-10.652573228649));
#21063=CARTESIAN_POINT('Ctrl Pts',(-42.2055869083974,0.0450304331853256,
-10.6443948820145));
#21064=CARTESIAN_POINT('Ctrl Pts',(-42.2597977418648,0.186602611542281,
-10.589958769094));
#21065=CARTESIAN_POINT('Ctrl Pts',(-42.3147058279888,0.298272918359021,
-10.5343638976612));
#21066=CARTESIAN_POINT('Ctrl Pts',(-42.3778559173175,0.400053103664132,
-10.4702558451013));
#21067=CARTESIAN_POINT('',(-43.4947470521204,0.676002124309098,-9.34999999999999));
#21068=CARTESIAN_POINT('Ctrl Pts',(-42.3778559173175,0.400053103664149,
-10.4702558451013));
#21069=CARTESIAN_POINT('Ctrl Pts',(-42.5816808626342,0.437302204925704,
-10.2660883599949));
#21070=CARTESIAN_POINT('Ctrl Pts',(-42.7846012138064,0.481452074273063,
-10.0627168595909));
#21071=CARTESIAN_POINT('Ctrl Pts',(-42.9865892281655,0.532479714672422,
-9.86011238749772));
#21072=CARTESIAN_POINT('Ctrl Pts',(-43.1566436222613,0.57544005812541,-9.68953899554559));
#21073=CARTESIAN_POINT('Ctrl Pts',(-43.3260372652128,0.62327625115777,-9.51950878871243));
#21074=CARTESIAN_POINT('Ctrl Pts',(-43.4947470521204,0.676002124309097,
-9.34999999999999));
#21075=CARTESIAN_POINT('',(-43.3203086503669,3.94979220174326,-9.34999999999999));
#21076=CARTESIAN_POINT('Origin',(-3.46944695195361E-15,3.46944695195361E-15,
-9.34999999999999));
#21077=CARTESIAN_POINT('',(-42.2054617208597,4.06886253049829,-10.4488603766002));
#21078=CARTESIAN_POINT('Ctrl Pts',(-43.3203086503669,3.94979220174326,-9.34999999999999));
#21079=CARTESIAN_POINT('Ctrl Pts',(-43.1122825236194,3.98478982700619,-9.55398902691261));
#21080=CARTESIAN_POINT('Ctrl Pts',(-42.9041475658186,4.01262695712239,-9.75864153760851));
#21081=CARTESIAN_POINT('Ctrl Pts',(-42.6959315890961,4.03332628396938,-9.9639874409246));
#21082=CARTESIAN_POINT('Ctrl Pts',(-42.5324864596814,4.04957481690408,-10.1251796235352));
#21083=CARTESIAN_POINT('Ctrl Pts',(-42.3689912631271,4.0614240412298,-10.2867993162806));
#21084=CARTESIAN_POINT('Ctrl Pts',(-42.2054617208597,4.0688625304983,-10.4488603766002));
#21085=CARTESIAN_POINT('',(-41.8895769551539,6.42697885114126,-10.4702558451001));
#21086=CARTESIAN_POINT('Ctrl Pts',(-42.2054617208597,4.06886253049829,-10.4488603766002));
#21087=CARTESIAN_POINT('Ctrl Pts',(-42.0931565705377,4.20679248947244,-10.5474113287251));
#21088=CARTESIAN_POINT('Ctrl Pts',(-41.9966452868457,4.36886244650457,-10.6271346454328));
#21089=CARTESIAN_POINT('Ctrl Pts',(-41.8322466693347,4.75204677304844,-10.7492419669048));
#21090=CARTESIAN_POINT('Ctrl Pts',(-41.7715980988893,4.97460297983664,-10.7838654920958));
#21091=CARTESIAN_POINT('Ctrl Pts',(-41.7101624561644,5.43269747180171,-10.7881590891372));
#21092=CARTESIAN_POINT('Ctrl Pts',(-41.7099416343854,5.66394270882025,-10.7577973127697));
#21093=CARTESIAN_POINT('Ctrl Pts',(-41.7673137310929,6.07920795449955,-10.6430146790662));
#21094=CARTESIAN_POINT('Ctrl Pts',(-41.8176243487641,6.26256709539985,-10.5663096368512));
#21095=CARTESIAN_POINT('Ctrl Pts',(-41.8895769551532,6.42697885114131,-10.4702558451007));
#21096=CARTESIAN_POINT('',(-42.9558281083827,6.85906928985893,-9.34999999999999));
#21097=CARTESIAN_POINT('Ctrl Pts',(-41.8895769551539,6.42697885114127,-10.4702558451001));
#21098=CARTESIAN_POINT('Ctrl Pts',(-42.0860261557539,6.49285612410681,-10.2660883608697));
#21099=CARTESIAN_POINT('Ctrl Pts',(-42.2805978879953,6.56543518806218,-10.0627168613349));
#21100=CARTESIAN_POINT('Ctrl Pts',(-42.4732679644127,6.64468933185857,-9.86011239010124));
#21101=CARTESIAN_POINT('Ctrl Pts',(-42.6354775564803,6.71141366484236,-9.68953899727869));
#21102=CARTESIAN_POINT('Ctrl Pts',(-42.7963392171419,6.7828701836438,-9.51950878957843));
#21103=CARTESIAN_POINT('Ctrl Pts',(-42.9558281083827,6.85906928985893,-9.34999999999999));
#21104=CARTESIAN_POINT('',(-42.3172563326291,10.0747117317853,-9.34999999999999));
#21105=CARTESIAN_POINT('Origin',(-3.46944695195361E-15,3.46944695195361E-15,
-9.34999999999999));
#21106=CARTESIAN_POINT('',(-41.1968114628076,10.0339108358061,-10.4488603766004));
#21107=CARTESIAN_POINT('Ctrl Pts',(-42.3172563326291,10.0747117317853,-9.34999999999999));
#21108=CARTESIAN_POINT('Ctrl Pts',(-42.1063669305215,10.0797479271007,-9.55398902691476));
#21109=CARTESIAN_POINT('Ctrl Pts',(-41.8963888498126,10.0776810225116,-9.75864153761282));
#21110=CARTESIAN_POINT('Ctrl Pts',(-41.6873463901558,10.0685374370037,-9.96398744093108));
#21111=CARTESIAN_POINT('Ctrl Pts',(-41.5232524891554,10.0613599161423,-10.1251796235396));
#21112=CARTESIAN_POINT('Ctrl Pts',(-41.35973511752,10.0498207399935,-10.2867993162829));
#21113=CARTESIAN_POINT('Ctrl Pts',(-41.1968114628076,10.0339108358061,-10.4488603766004));
#21114=CARTESIAN_POINT('',(-40.5485470057466,12.3230698430839,-10.4702558451002));
#21115=CARTESIAN_POINT('Ctrl Pts',(-41.1968114628078,10.0339108358065,-10.4488603766002));
#21116=CARTESIAN_POINT('Ctrl Pts',(-41.0660199366602,10.1544541778516,-10.5474113291175));
#21117=CARTESIAN_POINT('Ctrl Pts',(-40.9474260385346,10.3011395093612,-10.6271346460645));
#21118=CARTESIAN_POINT('Ctrl Pts',(-40.7301679463243,10.6570272103071,-10.7492419673841));
#21119=CARTESIAN_POINT('Ctrl Pts',(-40.6384636404793,10.8686869244629,-10.7838654923525));
#21120=CARTESIAN_POINT('Ctrl Pts',(-40.5124596809,11.3133754715828,-10.7881590889254));
#21121=CARTESIAN_POINT('Ctrl Pts',(-40.4793314784874,11.5422355392716,-10.7577973123336));
#21122=CARTESIAN_POINT('Ctrl Pts',(-40.4770212041169,11.9614388832617,-10.6430146784589));
#21123=CARTESIAN_POINT('Ctrl Pts',(-40.5007250057618,12.1500916390997,-10.5663096364691));
#21124=CARTESIAN_POINT('Ctrl Pts',(-40.5485470057463,12.3230698430838,-10.4702558451005));
#21125=CARTESIAN_POINT('',(-41.5424523787372,12.9025055845893,-9.34999999999999));
#21126=CARTESIAN_POINT('Ctrl Pts',(-40.5485470057466,12.3230698430839,-10.4702558451002));
#21127=CARTESIAN_POINT('Ctrl Pts',(-40.7336213240878,12.4162342170104,-10.2660883599929));
#21128=CARTESIAN_POINT('Ctrl Pts',(-40.9158835196662,12.5157649758065,-10.0627168595879));
#21129=CARTESIAN_POINT('Ctrl Pts',(-41.0953134525995,12.621632237967,-9.86011238749391));
#21130=CARTESIAN_POINT('Ctrl Pts',(-41.2463761214618,12.7107622449043,-9.68953899554305));
#21131=CARTESIAN_POINT('Ctrl Pts',(-41.3954311186751,12.8043844401441,-9.51950878871116));
#21132=CARTESIAN_POINT('Ctrl Pts',(-41.5424523787372,12.9025055845893,-9.34999999999999));
#21133=CARTESIAN_POINT('',(-40.4527467088508,15.9945391840328,-9.34999999999999));
#21134=CARTESIAN_POINT('Origin',(-3.46944695195361E-15,3.46944695195361E-15,
-9.34999999999999));
#21135=CARTESIAN_POINT('',(-39.3495129251727,15.7946976518991,-10.4488603765979));
#21136=CARTESIAN_POINT('Ctrl Pts',(-40.4527467088508,15.9945391840329,-9.34999999999999));
#21137=CARTESIAN_POINT('Ctrl Pts',(-40.2432871314579,15.9695114269864,-9.55398902691462));
#21138=CARTESIAN_POINT('Ctrl Pts',(-40.03574047604,15.937582563908,-9.75864153761254));
#21139=CARTESIAN_POINT('Ctrl Pts',(-39.8301270351014,15.8987822030778,-9.96398744093064));
#21140=CARTESIAN_POINT('Ctrl Pts',(-39.6687248411308,15.8683247420467,-10.1251796235385));
#21141=CARTESIAN_POINT('Ctrl Pts',(-39.5085140365544,15.8336320697735,-10.2867993162811));
#21142=CARTESIAN_POINT('Ctrl Pts',(-39.3495129251727,15.7946976518991,-10.4488603765979));
#21143=CARTESIAN_POINT('',(-38.382065571658,17.9682986698097,-10.4702558451029));
#21144=CARTESIAN_POINT('Ctrl Pts',(-39.3495129251723,15.7946976518996,-10.4488603765981));
#21145=CARTESIAN_POINT('Ctrl Pts',(-39.2028975619468,15.8954004616402,-10.5474113291157));
#21146=CARTESIAN_POINT('Ctrl Pts',(-39.0646352794747,16.0237150765457,-10.6271346460632));
#21147=CARTESIAN_POINT('Ctrl Pts',(-38.7989404607791,16.3450613035865,-10.7492419673833));
#21148=CARTESIAN_POINT('Ctrl Pts',(-38.6780472545519,16.5415157435844,-10.783865492352));
#21149=CARTESIAN_POINT('Ctrl Pts',(-38.4900400549329,16.9637457693522,-10.7881590889255));
#21150=CARTESIAN_POINT('Ctrl Pts',(-38.4246788663334,17.1855617367719,-10.757797312334));
#21151=CARTESIAN_POINT('Ctrl Pts',(-38.3627332511209,17.6001694088377,-10.64301467846));
#21152=CARTESIAN_POINT('Ctrl Pts',(-38.3593476958059,17.7902753543337,-10.5663096364705));
#21153=CARTESIAN_POINT('Ctrl Pts',(-38.382065571659,17.9682986698092,-10.4702558451022));
#21154=CARTESIAN_POINT('',(-39.2833921172033,18.6832840733651,-9.34999999999999));
#21155=CARTESIAN_POINT('Ctrl Pts',(-38.382065571658,17.9682986698097,-10.4702558451029));
#21156=CARTESIAN_POINT('Ctrl Pts',(-38.5519974274827,18.0868535864236,-10.2660883599985));
#21157=CARTESIAN_POINT('Ctrl Pts',(-38.7182397528666,18.2113098804923,-10.0627168595965));
#21158=CARTESIAN_POINT('Ctrl Pts',(-38.880776865504,18.3416351084573,-9.86011238750546));
#21159=CARTESIAN_POINT('Ctrl Pts',(-39.017617411692,18.45135635973,-9.68953899555072));
#21160=CARTESIAN_POINT('Ctrl Pts',(-39.1518314163817,18.5652383538395,-9.51950878871498));
#21161=CARTESIAN_POINT('Ctrl Pts',(-39.2833921172033,18.6832840733651,-9.34999999999999));
#21162=CARTESIAN_POINT('',(-37.7647358181634,21.588763942948,-9.34999999999999));
#21163=CARTESIAN_POINT('Origin',(-3.46944695195361E-15,3.46944695195361E-15,
-9.34999999999999));
#21164=CARTESIAN_POINT('',(-36.7011717789913,21.2339499719654,-10.4488603766012));
#21165=CARTESIAN_POINT('Ctrl Pts',(-37.7647358181634,21.588763942948,-9.34999999999999));
#21166=CARTESIAN_POINT('Ctrl Pts',(-37.5609700584519,21.5341817265017,-9.55398902691111));
#21167=CARTESIAN_POINT('Ctrl Pts',(-37.3600798797167,21.473040884514,-9.7586415376055));
#21168=CARTESIAN_POINT('Ctrl Pts',(-37.162081154216,21.4053736118198,-9.96398744092007));
#21169=CARTESIAN_POINT('Ctrl Pts',(-37.0066563504932,21.3522562366935,-10.1251796235325));
#21170=CARTESIAN_POINT('Ctrl Pts',(-36.8530135429414,21.2951163110575,-10.2867993162797));
#21171=CARTESIAN_POINT('Ctrl Pts',(-36.7011717789913,21.2339499719654,-10.4488603766012));
#21172=CARTESIAN_POINT('',(-35.4342359672603,23.2477447519392,-10.4702558450998));
#21173=CARTESIAN_POINT('Ctrl Pts',(-36.7011717789913,21.2339499719654,-10.4488603766012));
#21174=CARTESIAN_POINT('Ctrl Pts',(-36.5417172446798,21.3127622305992,-10.5474113291184));
#21175=CARTESIAN_POINT('Ctrl Pts',(-36.3866011992174,21.4200940133705,-10.6271346460654));
#21176=CARTESIAN_POINT('Ctrl Pts',(-36.0778784343449,21.7003570840114,-10.7492419673846));
#21177=CARTESIAN_POINT('Ctrl Pts',(-35.9302573647871,21.8776070039822,-10.7838654923527));
#21178=CARTESIAN_POINT('Ctrl Pts',(-35.6840742095452,22.2687831226866,-10.7881590889251));
#21179=CARTESIAN_POINT('Ctrl Pts',(-35.5878106000732,22.4790394564059,-10.757797312333));
#21180=CARTESIAN_POINT('Ctrl Pts',(-35.4674906781093,22.8806112399746,-10.6430146784579));
#21181=CARTESIAN_POINT('Ctrl Pts',(-35.4370846859782,23.0683003662984,-10.566309636468));
#21182=CARTESIAN_POINT('Ctrl Pts',(-35.4342359672613,23.2477447519385,-10.4702558450994));
#21183=CARTESIAN_POINT('',(-36.224635276104,24.0837247765632,-9.34999999999999));
#21184=CARTESIAN_POINT('Ctrl Pts',(-35.4342359672603,23.2477447519392,-10.4702558450998));
#21185=CARTESIAN_POINT('Ctrl Pts',(-35.5855660380337,23.3892767750254,-10.2660883599909));
#21186=CARTESIAN_POINT('Ctrl Pts',(-35.7324042788881,23.5361250331255,-10.0627168595844));
#21187=CARTESIAN_POINT('Ctrl Pts',(-35.8747397843408,23.6882551810844,-9.86011238748882));
#21188=CARTESIAN_POINT('Ctrl Pts',(-35.9945725289429,23.8163340684192,-9.68953899553967));
#21189=CARTESIAN_POINT('Ctrl Pts',(-36.1112133310081,23.9481575523993,-9.51950878870948));
#21190=CARTESIAN_POINT('Ctrl Pts',(-36.224635276104,24.0837247765632,-9.34999999999999));
#21191=CARTESIAN_POINT('',(-34.3079438107289,26.7435037248277,-9.34999999999999));
#21192=CARTESIAN_POINT('Origin',(-3.46944695195361E-15,3.46944695195361E-15,
-9.34999999999999));
#21193=CARTESIAN_POINT('',(-33.3057006128448,26.2409403042404,-10.4488603765989));
#21194=CARTESIAN_POINT('Ctrl Pts',(-34.3079438107289,26.7435037248277,-9.34999999999999));
#21195=CARTESIAN_POINT('Ctrl Pts',(-34.1140199519504,26.6604781855035,-9.55398902691272));
#21196=CARTESIAN_POINT('Ctrl Pts',(-33.9238757946133,26.5713700158308,-9.75864153760872));
#21197=CARTESIAN_POINT('Ctrl Pts',(-33.7375224676165,26.4762133418051,-9.96398744092491));
#21198=CARTESIAN_POINT('Ctrl Pts',(-33.5912390549448,26.4015173691638,-10.125179623535));
#21199=CARTESIAN_POINT('Ctrl Pts',(-33.4472919689175,26.3230933942739,-10.2867993162798));
#21200=CARTESIAN_POINT('Ctrl Pts',(-33.3057006128448,26.2409403042404,-10.4488603765989));
#21201=CARTESIAN_POINT('',(-31.7650675024763,28.0539337918545,-10.4702558451018));
#21202=CARTESIAN_POINT('Ctrl Pts',(-33.3057006128448,26.2409403042404,-10.4488603765989));
#21203=CARTESIAN_POINT('Ctrl Pts',(-33.1366529419366,26.2962576214563,-10.5474113291164));
#21204=CARTESIAN_POINT('Ctrl Pts',(-32.9678408488513,26.3804216065147,-10.6271346460638));
#21205=CARTESIAN_POINT('Ctrl Pts',(-32.6223748430112,26.6138961728476,-10.7492419673837));
#21206=CARTESIAN_POINT('Ctrl Pts',(-32.4510310493948,26.7683332755662,-10.7838654923524));
#21207=CARTESIAN_POINT('Ctrl Pts',(-32.1516835176362,27.1204922694869,-10.7881590889256));
#21208=CARTESIAN_POINT('Ctrl Pts',(-32.0264771367785,27.3149087568795,-10.757797312334));
#21209=CARTESIAN_POINT('Ctrl Pts',(-31.8502322746985,27.6952698084749,-10.6430146784597));
#21210=CARTESIAN_POINT('Ctrl Pts',(-31.7934248240667,27.8767213062657,-10.5663096364699));
#21211=CARTESIAN_POINT('Ctrl Pts',(-31.7650675024771,28.0539337918543,-10.4702558451013));
#21212=CARTESIAN_POINT('',(-32.4284493240122,28.9938902950256,-9.34999999999999));
#21213=CARTESIAN_POINT('Ctrl Pts',(-31.7650675024763,28.0539337918545,-10.4702558451018));
#21214=CARTESIAN_POINT('Ctrl Pts',(-31.8947151443539,28.2155617375679,-10.2660883599912));
#21215=CARTESIAN_POINT('Ctrl Pts',(-32.019160097538,28.3818125526397,-10.0627168595829));
#21216=CARTESIAN_POINT('Ctrl Pts',(-32.1383964553732,28.552650689487,-9.86011238748564));
#21217=CARTESIAN_POINT('Ctrl Pts',(-32.2387819492814,28.6964798960908,-9.68953899553755));
#21218=CARTESIAN_POINT('Ctrl Pts',(-32.3354750783595,28.8435613239594,-9.51950878870842));
#21219=CARTESIAN_POINT('Ctrl Pts',(-32.4284493240122,28.9938902950256,-9.34999999999999));
#21220=CARTESIAN_POINT('',(-30.1527410032581,31.353822892758,-9.34999999999999));
#21221=CARTESIAN_POINT('Origin',(-3.46944695195361E-15,3.46944695195361E-15,
-9.34999999999999));
#21222=CARTESIAN_POINT('',(-29.2322214279503,30.7137407645344,-10.448860376592));
#21223=CARTESIAN_POINT('Ctrl Pts',(-30.1527410032581,31.353822892758,-9.34999999999999));
#21224=CARTESIAN_POINT('Ctrl Pts',(-29.9726067759491,31.2440441911095,-9.55398902691394));
#21225=CARTESIAN_POINT('Ctrl Pts',(-29.797079426725,31.1287826791183,-9.75864153761113));
#21226=CARTESIAN_POINT('Ctrl Pts',(-29.6261651145731,31.0080737192341,-9.96398744092845));
#21227=CARTESIAN_POINT('Ctrl Pts',(-29.4920010013893,30.9133197436759,-10.1251796235351));
#21228=CARTESIAN_POINT('Ctrl Pts',(-29.3606799844505,30.8152082055055,-10.2867993162765));
#21229=CARTESIAN_POINT('Ctrl Pts',(-29.2322214279503,30.7137407645344,-10.448860376592));
#21230=CARTESIAN_POINT('',(-27.4492538662502,32.2890256406138,-10.4702558451084));
#21231=CARTESIAN_POINT('Ctrl Pts',(-29.2322214279499,30.7137407645349,-10.4488603765919));
#21232=CARTESIAN_POINT('Ctrl Pts',(-29.0570219435323,30.7444370392754,-10.5474113291101));
#21233=CARTESIAN_POINT('Ctrl Pts',(-28.877950330226,30.803719890593,-10.6271346460583));
#21234=CARTESIAN_POINT('Ctrl Pts',(-28.502773775056,30.9856530837304,-10.7492419673805));
#21235=CARTESIAN_POINT('Ctrl Pts',(-28.311195322904,31.1141334751444,-10.7838654923505));
#21236=CARTESIAN_POINT('Ctrl Pts',(-27.9647772671275,31.4201064027068,-10.7881590889265));
#21237=CARTESIAN_POINT('Ctrl Pts',(-27.8131769557322,31.59472528474,-10.7577973123362));
#21238=CARTESIAN_POINT('Ctrl Pts',(-27.5845949906789,31.9461325502209,-10.6430146784644));
#21239=CARTESIAN_POINT('Ctrl Pts',(-27.5025425174213,32.1176525902456,-10.566309636476));
#21240=CARTESIAN_POINT('Ctrl Pts',(-27.4492538662497,32.2890256406138,-10.4702558451087));
#21241=CARTESIAN_POINT('',(-27.9721136596209,33.313823818548,-9.34999999999999));
#21242=CARTESIAN_POINT('Ctrl Pts',(-27.4492538662502,32.2890256406138,-10.4702558451084));
#21243=CARTESIAN_POINT('Ctrl Pts',(-27.5545798271122,32.4674592300734,-10.2660883600007));
#21244=CARTESIAN_POINT('Ctrl Pts',(-27.654098152245,32.6497282149467,-10.0627168595954));
#21245=CARTESIAN_POINT('Ctrl Pts',(-27.7478080540628,32.8357965688694,-9.86011238750101));
#21246=CARTESIAN_POINT('Ctrl Pts',(-27.8267027381112,32.9924481468711,-9.68953899554773));
#21247=CARTESIAN_POINT('Ctrl Pts',(-27.9014798009359,33.1517933649108,-9.51950878871348));
#21248=CARTESIAN_POINT('Ctrl Pts',(-27.9721136596209,33.313823818548,-9.34999999999999));
#21249=CARTESIAN_POINT('',(-25.3837153422505,35.3258686435819,-9.34999999999999));
#21250=CARTESIAN_POINT('Origin',(-3.46944695195361E-15,3.46944695195361E-15,
-9.34999999999999));
#21251=CARTESIAN_POINT('',(-24.5636585134689,34.561298034017,-10.4488603766072));
#21252=CARTESIAN_POINT('Ctrl Pts',(-25.3837153422505,35.3258686435819,-9.34999999999999));
#21253=CARTESIAN_POINT('Ctrl Pts',(-25.2210377598102,35.1915715574042,-9.55398902691391));
#21254=CARTESIAN_POINT('Ctrl Pts',(-25.0637004493459,35.052503095097,-9.75864153761116));
#21255=CARTESIAN_POINT('Ctrl Pts',(-24.9117044745538,34.9086991356865,-9.96398744092865));
#21256=CARTESIAN_POINT('Ctrl Pts',(-24.7923908552944,34.7958160749043,-10.1251796235402));
#21257=CARTESIAN_POINT('Ctrl Pts',(-24.67636922464,34.6800142414381,-10.2867993162866));
#21258=CARTESIAN_POINT('Ctrl Pts',(-24.5636585134689,34.561298034017,-10.4488603766072));
#21259=CARTESIAN_POINT('',(-22.5746525783567,35.8668060412644,-10.4702558450952));
#21260=CARTESIAN_POINT('Ctrl Pts',(-24.563658513468,34.5612980340179,-10.4488603766069));
#21261=CARTESIAN_POINT('Ctrl Pts',(-24.3858737718084,34.5667483786537,-10.5474113291238));
#21262=CARTESIAN_POINT('Ctrl Pts',(-24.200188019927,34.5999432683392,-10.6271346460702));
#21263=CARTESIAN_POINT('Ctrl Pts',(-23.8029384281704,34.7266314531289,-10.7492419673877));
#21264=CARTESIAN_POINT('Ctrl Pts',(-23.5950253023033,34.8265396429796,-10.7838654923547));
#21265=CARTESIAN_POINT('Ctrl Pts',(-23.2085887951417,35.0800977777375,-10.7881590889249));
#21266=CARTESIAN_POINT('Ctrl Pts',(-23.0336806983727,35.2313643175347,-10.7577973123318));
#21267=CARTESIAN_POINT('Ctrl Pts',(-22.757414899985,35.5466641583542,-10.6430146784548));
#21268=CARTESIAN_POINT('Ctrl Pts',(-22.6517877558409,35.7047610872222,-10.5663096364641));
#21269=CARTESIAN_POINT('Ctrl Pts',(-22.5746525783574,35.8668060412645,-10.4702558450948));
#21270=CARTESIAN_POINT('',(-22.9463464259947,36.9555839582903,-9.34999999999999));
#21271=CARTESIAN_POINT('Ctrl Pts',(-22.5746525783567,35.8668060412644,-10.4702558450952));
#21272=CARTESIAN_POINT('Ctrl Pts',(-22.6535127253813,36.0584128811461,-10.2660883599885));
#21273=CARTESIAN_POINT('Ctrl Pts',(-22.7260785163567,36.2529895649068,-10.062716859584));
#21274=CARTESIAN_POINT('Ctrl Pts',(-22.7923542987999,36.4505003207935,-9.86011238749044));
#21275=CARTESIAN_POINT('Ctrl Pts',(-22.848152104735,36.6167852957994,-9.68953899554077));
#21276=CARTESIAN_POINT('Ctrl Pts',(-22.8994908559473,36.785150494873,-9.51950878871004));
#21277=CARTESIAN_POINT('Ctrl Pts',(-22.9463464259947,36.9555839582903,-9.34999999999999));
#21278=CARTESIAN_POINT('',(-20.0979504374858,38.5787815801947,-9.34999999999999));
#21279=CARTESIAN_POINT('Origin',(-3.46944695195361E-15,3.46944695195361E-15,
-9.34999999999999));
#21280=CARTESIAN_POINT('',(-19.3950503474463,37.7052869420536,-10.4488603766057));
#21281=CARTESIAN_POINT('Ctrl Pts',(-20.0979504374858,38.5787815801947,-9.35));
#21282=CARTESIAN_POINT('Ctrl Pts',(-19.9560411463757,38.4227000108812,-9.55398902691007));
#21283=CARTESIAN_POINT('Ctrl Pts',(-19.8200968085948,38.2626556311101,-9.75864153760344));
#21284=CARTESIAN_POINT('Ctrl Pts',(-19.6901133708948,38.0986841060908,-9.96398744091703));
#21285=CARTESIAN_POINT('Ctrl Pts',(-19.5880791267801,37.9699699336721,-10.125179623532));
#21286=CARTESIAN_POINT('Ctrl Pts',(-19.4897187482356,37.8388351962927,-10.2867993162817));
#21287=CARTESIAN_POINT('Ctrl Pts',(-19.3950503474463,37.7052869420536,-10.4488603766058));
#21288=CARTESIAN_POINT('',(-17.2404964639284,38.7144417021942,-10.4702558450937));
#21289=CARTESIAN_POINT('Ctrl Pts',(-19.3950503474456,37.7052869420535,-10.4488603766062));
#21290=CARTESIAN_POINT('Ctrl Pts',(-19.2182995331962,37.6853804032832,-10.5474113291228));
#21291=CARTESIAN_POINT('Ctrl Pts',(-19.0297796691752,37.6918115791063,-10.6271346460691));
#21292=CARTESIAN_POINT('Ctrl Pts',(-18.6185438969465,37.7606757494393,-10.7492419673865));
#21293=CARTESIAN_POINT('Ctrl Pts',(-18.3985286090339,37.8299778950903,-10.7838654923536));
#21294=CARTESIAN_POINT('Ctrl Pts',(-17.9799403833786,38.0259595246174,-10.7881590889238));
#21295=CARTESIAN_POINT('Ctrl Pts',(-17.7852851256906,38.1507943716434,-10.7577973123307));
#21296=CARTESIAN_POINT('Ctrl Pts',(-17.4669594689343,38.4235681922903,-10.6430146784537));
#21297=CARTESIAN_POINT('Ctrl Pts',(-17.3399079179525,38.5650236124433,-10.566309636463));
#21298=CARTESIAN_POINT('Ctrl Pts',(-17.2404964639285,38.7144417021941,-10.4702558450937));
#21299=CARTESIAN_POINT('',(-17.4534577509583,39.8450349797251,-9.34999999999999));
#21300=CARTESIAN_POINT('Ctrl Pts',(-17.2404964639284,38.7144417021942,-10.4702558450937));
#21301=CARTESIAN_POINT('Ctrl Pts',(-17.2912854319336,38.9153212297907,-10.2660883599863));
#21302=CARTESIAN_POINT('Ctrl Pts',(-17.335421458507,39.1182445922746,-10.0627168595812));
#21303=CARTESIAN_POINT('Ctrl Pts',(-17.3729139377655,39.3231770007139,-9.86011238748706));
#21304=CARTESIAN_POINT('Ctrl Pts',(-17.4044789831645,39.4957102901639,-9.68953899553853));
#21305=CARTESIAN_POINT('Ctrl Pts',(-17.4313343138366,39.6696680403483,-9.51950878870892));
#21306=CARTESIAN_POINT('Ctrl Pts',(-17.4534577509583,39.8450349797251,-9.34999999999999));
#21307=CARTESIAN_POINT('',(-14.4030492195196,41.0463417758526,-9.34999999999999));
#21308=CARTESIAN_POINT('Origin',(-3.46944695195361E-15,3.46944695195361E-15,
-9.34999999999999));
#21309=CARTESIAN_POINT('',(-13.8316148870599,40.0817049410166,-10.4488603766049));
#21310=CARTESIAN_POINT('Ctrl Pts',(-14.4030492195196,41.0463417758526,-9.34999999999999));
#21311=CARTESIAN_POINT('Ctrl Pts',(-14.2847970836707,40.8716530940489,-9.55398902691104));
#21312=CARTESIAN_POINT('Ctrl Pts',(-14.1730131532563,40.6938908388526,-9.7586415376054));
#21313=CARTESIAN_POINT('Ctrl Pts',(-14.0676883405958,40.5130897356151,-9.96398744091997));
#21314=CARTESIAN_POINT('Ctrl Pts',(-13.9850105945971,40.3711647009326,-10.1251796235337));
#21315=CARTESIAN_POINT('Ctrl Pts',(-13.9063138018252,40.227366584735,-10.2867993162822));
#21316=CARTESIAN_POINT('Ctrl Pts',(-13.8316148870599,40.0817049410166,-10.4488603766049));
#21317=CARTESIAN_POINT('',(-11.5553735589841,40.7739629732932,-10.4702558450957));
#21318=CARTESIAN_POINT('Ctrl Pts',(-13.8316148870598,40.0817049410166,-10.4488603766049));
#21319=CARTESIAN_POINT('Ctrl Pts',(-13.6594961370917,40.0368467585633,-10.5474113291217));
#21320=CARTESIAN_POINT('Ctrl Pts',(-13.4719798817163,40.0163833003297,-10.6271346460682));
#21321=CARTESIAN_POINT('Ctrl Pts',(-13.0551295034324,40.0260215802851,-10.7492419673861));
#21322=CARTESIAN_POINT('Ctrl Pts',(-12.8274909302648,40.0633068899016,-10.7838654923536));
#21323=CARTESIAN_POINT('Ctrl Pts',(-12.3852722352818,40.1977223933844,-10.7881590889245));
#21324=CARTESIAN_POINT('Ctrl Pts',(-12.174832436382,40.2935842701473,-10.7577973123317));
#21325=CARTESIAN_POINT('Ctrl Pts',(-11.8209271136526,40.5182791822475,-10.6430146784553));
#21326=CARTESIAN_POINT('Ctrl Pts',(-11.6750375590242,40.6402134692549,-10.5663096364647));
#21327=CARTESIAN_POINT('Ctrl Pts',(-11.5553735589844,40.7739629732933,-10.4702558450954));
#21328=CARTESIAN_POINT('',(-11.6052670077299,41.9233559925646,-9.34999999999999));
#21329=CARTESIAN_POINT('Ctrl Pts',(-11.5553735589841,40.7739629732932,-10.4702558450957));
#21330=CARTESIAN_POINT('Ctrl Pts',(-11.5770574310437,40.9800258607092,-10.2660883599901));
#21331=CARTESIAN_POINT('Ctrl Pts',(-11.5918652109912,41.1871649674364,-10.0627168595868));
#21332=CARTESIAN_POINT('Ctrl Pts',(-11.5998111483063,41.3953471955663,-9.86011238749444));
#21333=CARTESIAN_POINT('Ctrl Pts',(-11.6065008598711,41.5706165192358,-9.68953899554343));
#21334=CARTESIAN_POINT('Ctrl Pts',(-11.608326072915,41.7466255423937,-9.51950878871137));
#21335=CARTESIAN_POINT('Ctrl Pts',(-11.6052670077299,41.9233559925646,-9.34999999999999));
#21336=CARTESIAN_POINT('',(-8.41494345442185,42.678316820827,-9.34999999999999));
#21337=CARTESIAN_POINT('Origin',(-3.46944695195361E-15,3.46944695195361E-15,
-9.34999999999999));
#21338=CARTESIAN_POINT('',(-7.98660763468405,41.6421750134759,-10.4488603765967));
#21339=CARTESIAN_POINT('Ctrl Pts',(-8.41494345442186,42.678316820827,-9.34999999999999));
#21340=CARTESIAN_POINT('Ctrl Pts',(-8.32275574631089,42.4885771843321,-9.55398902691367));
#21341=CARTESIAN_POINT('Ctrl Pts',(-8.23740782172991,42.2967157806002,-9.75864153761063));
#21342=CARTESIAN_POINT('Ctrl Pts',(-8.1588857435649,42.1027656882172,-9.96398744092778));
#21343=CARTESIAN_POINT('Ctrl Pts',(-8.09724757617075,41.9505189757028,-10.1251796235362));
#21344=CARTESIAN_POINT('Ctrl Pts',(-8.03981640893231,41.7969847956571,-10.2867993162793));
#21345=CARTESIAN_POINT('Ctrl Pts',(-7.98660763468405,41.6421750134759,-10.4488603765967));
#21346=CARTESIAN_POINT('',(-5.63501657135133,42.0034439406494,-10.4702558451012));
#21347=CARTESIAN_POINT('Ctrl Pts',(-7.98660763468398,41.6421750134755,-10.448860376597));
#21348=CARTESIAN_POINT('Ctrl Pts',(-7.82262479039767,41.5732783705729,-10.5474113291148));
#21349=CARTESIAN_POINT('Ctrl Pts',(-7.6399294338754,41.5263368552799,-10.6271346460624));
#21350=CARTESIAN_POINT('Ctrl Pts',(-7.22595032114179,41.4765530372707,-10.7492419673826));
#21351=CARTESIAN_POINT('Ctrl Pts',(-6.99532252761349,41.4810624894699,-10.7838654923514));
#21352=CARTESIAN_POINT('Ctrl Pts',(-6.53847566067895,41.551175554878,-10.7881590889251));
#21353=CARTESIAN_POINT('Ctrl Pts',(-6.31653526801434,41.6161129900091,-10.7577973123337));
#21354=CARTESIAN_POINT('Ctrl Pts',(-5.93425477110337,41.7881548531172,-10.6430146784598));
#21355=CARTESIAN_POINT('Ctrl Pts',(-5.77249710344944,41.888085776524,-10.5663096364702));
#21356=CARTESIAN_POINT('Ctrl Pts',(-5.63501657135134,42.0034439406487,-10.4702558451019));
#21357=CARTESIAN_POINT('',(-5.52082649506595,43.1482383743691,-9.34999999999999));
#21358=CARTESIAN_POINT('Ctrl Pts',(-5.63501657135133,42.0034439406494,-10.4702558451012));
#21359=CARTESIAN_POINT('Ctrl Pts',(-5.62715392636005,42.210495341738,-10.2660883599929));
#21360=CARTESIAN_POINT('Ctrl Pts',(-5.61233201598245,42.4176334378401,-10.062716859587));
#21361=CARTESIAN_POINT('Ctrl Pts',(-5.5905696549823,42.6248274958485,-9.86011238749209));
#21362=CARTESIAN_POINT('Ctrl Pts',(-5.57224784947496,42.7992648757395,-9.68953899554182));
#21363=CARTESIAN_POINT('Ctrl Pts',(-5.54900578881441,42.9737421357244,-9.51950878871054));
#21364=CARTESIAN_POINT('Ctrl Pts',(-5.52082649506595,43.1482383743691,-9.34999999999999));
#21365=CARTESIAN_POINT('',(-2.25553370726646,43.4414844094374,-9.34999999999999));
#21366=CARTESIAN_POINT('Origin',(-3.46944695195361E-15,3.46944695195361E-15,
-9.34999999999999));
#21367=CARTESIAN_POINT('',(-1.9790160823007,42.3549304887752,-10.4488603766009));
#21368=CARTESIAN_POINT('Ctrl Pts',(-2.25553370726647,43.4414844094374,-9.34999999999999));
#21369=CARTESIAN_POINT('Ctrl Pts',(-2.19128710278198,43.2405563700915,-9.55398902691156));
#21370=CARTESIAN_POINT('Ctrl Pts',(-2.13411262165439,43.0385015627268,-9.7586415376064));
#21371=CARTESIAN_POINT('Ctrl Pts',(-2.08399176105579,42.8353507457784,-9.96398744092142));
#21372=CARTESIAN_POINT('Ctrl Pts',(-2.04464794759835,42.6758816594482,-10.1251796235333));
#21373=CARTESIAN_POINT('Ctrl Pts',(-2.00965153883474,42.5157369286965,-10.28679931628));
#21374=CARTESIAN_POINT('Ctrl Pts',(-1.97901608230068,42.3549304887752,-10.4488603766009));
#21375=CARTESIAN_POINT('',(0.400053103665631,42.3778559173192,-10.4702558450996));
#21376=CARTESIAN_POINT('Ctrl Pts',(-1.97901608230066,42.3549304887752,-10.4488603766009));
#21377=CARTESIAN_POINT('Ctrl Pts',(-1.82650736151777,42.2633979223932,-10.5474113291179));
#21378=CARTESIAN_POINT('Ctrl Pts',(-1.65235205445744,42.1909339439257,-10.6271346460647));
#21379=CARTESIAN_POINT('Ctrl Pts',(-1.24967162819109,42.0827414829252,-10.7492419673841));
#21380=CARTESIAN_POINT('Ctrl Pts',(-1.02074953110196,42.0543832782663,-10.7838654923523));
#21381=CARTESIAN_POINT('Ctrl Pts',(-0.558574576988578,42.0587666057809,
-10.7881590889248));
#21382=CARTESIAN_POINT('Ctrl Pts',(-0.32965165693059,42.0914576603666,-10.7577973123328));
#21383=CARTESIAN_POINT('Ctrl Pts',(0.0732218856487259,42.2073441982801,
-10.6430146784578));
#21384=CARTESIAN_POINT('Ctrl Pts',(0.247554746683578,42.2832374526635,-10.5663096364682));
#21385=CARTESIAN_POINT('Ctrl Pts',(0.400053103665668,42.3778559173188,-10.4702558451));
#21386=CARTESIAN_POINT('',(0.67600212430957,43.4947470521204,-9.34999999999999));
#21387=CARTESIAN_POINT('Ctrl Pts',(0.400053103665649,42.3778559173192,-10.4702558450996));
#21388=CARTESIAN_POINT('Ctrl Pts',(0.437302204927781,42.5816808626396,-10.2660883599896));
#21389=CARTESIAN_POINT('Ctrl Pts',(0.48145207427596,42.7846012138153,-10.062716859582));
#21390=CARTESIAN_POINT('Ctrl Pts',(0.532479714676378,42.9865892281779,-9.86011238748525));
#21391=CARTESIAN_POINT('Ctrl Pts',(0.575440058128448,43.1566436222696,-9.68953899553729));
#21392=CARTESIAN_POINT('Ctrl Pts',(0.623276251159649,43.3260372652169,-9.51950878870829));
#21393=CARTESIAN_POINT('Ctrl Pts',(0.67600212430957,43.4947470521203,-9.34999999999999));
#21394=CARTESIAN_POINT('',(3.94979220174152,43.320308650367,-9.34999999999999));
#21395=CARTESIAN_POINT('Origin',(-3.46944695195361E-15,3.46944695195361E-15,
-9.34999999999999));
#21396=CARTESIAN_POINT('',(4.06886253049489,42.2054617208602,-10.4488603766));
#21397=CARTESIAN_POINT('Ctrl Pts',(3.94979220174152,43.320308650367,-9.34999999999999));
#21398=CARTESIAN_POINT('Ctrl Pts',(3.98478982700399,43.1122825236203,-9.55398902691186));
#21399=CARTESIAN_POINT('Ctrl Pts',(4.0126269571198,42.9041475658203,-9.758641537607));
#21400=CARTESIAN_POINT('Ctrl Pts',(4.03332628396646,42.6959315890987,-9.96398744092232));
#21401=CARTESIAN_POINT('Ctrl Pts',(4.04957481690103,42.5324864596833,-10.1251796235336));
#21402=CARTESIAN_POINT('Ctrl Pts',(4.06142404122659,42.3689912631283,-10.2867993162797));
#21403=CARTESIAN_POINT('Ctrl Pts',(4.06886253049491,42.2054617208602,-10.4488603766));
#21404=CARTESIAN_POINT('',(6.42697885113784,41.8895769551534,-10.4702558451011));
#21405=CARTESIAN_POINT('Ctrl Pts',(4.0688625304949,42.2054617208602,-10.4488603766));
#21406=CARTESIAN_POINT('Ctrl Pts',(4.20679249001818,42.0931565700911,-10.5474113291173));
#21407=CARTESIAN_POINT('Ctrl Pts',(4.36886244778761,41.996645286081,-10.6271346460644));
#21408=CARTESIAN_POINT('Ctrl Pts',(4.75204677534186,41.8322466685925,-10.7492419673842));
#21409=CARTESIAN_POINT('Ctrl Pts',(4.97460298225102,41.7715980983432,-10.7838654923527));
#21410=CARTESIAN_POINT('Ctrl Pts',(5.43269747427877,41.7101624560549,-10.7881590889257));
#21411=CARTESIAN_POINT('Ctrl Pts',(5.6639427112363,41.7099416344962,-10.757797312334));
#21412=CARTESIAN_POINT('Ctrl Pts',(6.07920795594927,41.7673137314911,-10.6430146784595));
#21413=CARTESIAN_POINT('Ctrl Pts',(6.26256709604998,41.81762434905,-10.56630963647));
#21414=CARTESIAN_POINT('Ctrl Pts',(6.42697885113787,41.8895769551527,-10.4702558451018));
#21415=CARTESIAN_POINT('',(6.8590692898575,42.9558281083829,-9.34999999999999));
#21416=CARTESIAN_POINT('Ctrl Pts',(6.42697885113785,41.8895769551534,-10.4702558451011));
#21417=CARTESIAN_POINT('Ctrl Pts',(6.49285612438642,42.0860261565966,-10.2660883599944));
#21418=CARTESIAN_POINT('Ctrl Pts',(6.5654351886824,42.2805978896651,-10.0627168595899));
#21419=CARTESIAN_POINT('Ctrl Pts',(6.64468933287527,42.4732679668901,-9.86011238749645));
#21420=CARTESIAN_POINT('Ctrl Pts',(6.71141366556903,42.6354775581211,-9.68953899554473));
#21421=CARTESIAN_POINT('Ctrl Pts',(6.78287018403159,42.7963392179574,-9.519508788712));
#21422=CARTESIAN_POINT('Ctrl Pts',(6.85906928985751,42.9558281083829,-9.34999999999999));
#21423=CARTESIAN_POINT('',(10.0747117317978,42.317256332626,-9.34999999999999));
#21424=CARTESIAN_POINT('Origin',(-3.46944695195361E-15,3.46944695195361E-15,
-9.34999999999999));
#21425=CARTESIAN_POINT('',(10.0339108358286,41.1968114627961,-10.4488603766063));
#21426=CARTESIAN_POINT('Ctrl Pts',(10.0747117317978,42.317256332626,-9.34999999999999));
#21427=CARTESIAN_POINT('Ctrl Pts',(10.0797479271153,42.1063669305229,-9.55398902690997));
#21428=CARTESIAN_POINT('Ctrl Pts',(10.0776810225284,41.8963888498183,-9.75864153760328));
#21429=CARTESIAN_POINT('Ctrl Pts',(10.0685374370231,41.6873463901658,-9.96398744091679));
#21430=CARTESIAN_POINT('Ctrl Pts',(10.0613599161632,41.5232524891582,-10.125179623532));
#21431=CARTESIAN_POINT('Ctrl Pts',(10.0498207400154,41.3597351175156,-10.286799316282));
#21432=CARTESIAN_POINT('Ctrl Pts',(10.0339108358287,41.1968114627961,-10.4488603766063));
#21433=CARTESIAN_POINT('',(12.3230698431103,40.5485470057438,-10.4702558450952));
#21434=CARTESIAN_POINT('Ctrl Pts',(10.0339108358291,41.1968114627954,-10.4488603766069));
#21435=CARTESIAN_POINT('Ctrl Pts',(10.1544541778752,41.0660199366484,-10.5474113291233));
#21436=CARTESIAN_POINT('Ctrl Pts',(10.3011395093857,40.9474260385234,-10.6271346460695));
#21437=CARTESIAN_POINT('Ctrl Pts',(10.6570272103333,40.7301679463145,-10.749241967387));
#21438=CARTESIAN_POINT('Ctrl Pts',(10.86868692449,40.6384636404703,-10.7838654923542));
#21439=CARTESIAN_POINT('Ctrl Pts',(11.3133754716112,40.5124596808929,-10.7881590889245));
#21440=CARTESIAN_POINT('Ctrl Pts',(11.5422355393004,40.4793314784814,-10.7577973123314));
#21441=CARTESIAN_POINT('Ctrl Pts',(11.9614388832899,40.4770212041131,-10.6430146784546));
#21442=CARTESIAN_POINT('Ctrl Pts',(12.1500916391271,40.5007250057588,-10.5663096364641));
#21443=CARTESIAN_POINT('Ctrl Pts',(12.3230698431103,40.5485470057438,-10.4702558450952));
#21444=CARTESIAN_POINT('',(12.9025055846018,41.5424523787333,-9.34999999999999));
#21445=CARTESIAN_POINT('Ctrl Pts',(12.3230698431103,40.5485470057438,-10.4702558450952));
#21446=CARTESIAN_POINT('Ctrl Pts',(12.4162342170355,40.7336213240864,-10.2660883599869));
#21447=CARTESIAN_POINT('Ctrl Pts',(12.5157649758303,40.9158835196663,-10.0627168595808));
#21448=CARTESIAN_POINT('Ctrl Pts',(12.6216322379894,41.0953134526012,-9.86011238748572));
#21449=CARTESIAN_POINT('Ctrl Pts',(12.7107622449237,41.2463761214615,-9.68953899553764));
#21450=CARTESIAN_POINT('Ctrl Pts',(12.8043844401601,41.3954311186729,-9.51950878870848));
#21451=CARTESIAN_POINT('Ctrl Pts',(12.9025055846018,41.5424523787333,-9.35));
#21452=CARTESIAN_POINT('',(15.9945391840345,40.4527467088502,-9.34999999999999));
#21453=CARTESIAN_POINT('Origin',(-3.46944695195361E-15,3.46944695195361E-15,
-9.34999999999999));
#21454=CARTESIAN_POINT('',(15.7946976519012,39.3495129251702,-10.4488603765994));
#21455=CARTESIAN_POINT('Ctrl Pts',(15.9945391840345,40.4527467088502,-9.34999999999999));
#21456=CARTESIAN_POINT('Ctrl Pts',(15.9695114269884,40.2432871314594,-9.55398902691247));
#21457=CARTESIAN_POINT('Ctrl Pts',(15.9375825639107,40.0357404760436,-9.75864153760821));
#21458=CARTESIAN_POINT('Ctrl Pts',(15.8987822030811,39.830127035107,-9.96398744092413));
#21459=CARTESIAN_POINT('Ctrl Pts',(15.8683247420498,39.6687248411337,-10.1251796235346));
#21460=CARTESIAN_POINT('Ctrl Pts',(15.8336320697762,39.5085140365546,-10.2867993162799));
#21461=CARTESIAN_POINT('Ctrl Pts',(15.7946976519012,39.3495129251702,-10.4488603765994));
#21462=CARTESIAN_POINT('',(17.9682986698117,38.3820655716568,-10.4702558451031));
#21463=CARTESIAN_POINT('Ctrl Pts',(15.7946976519015,39.3495129251703,-10.4488603765992));
#21464=CARTESIAN_POINT('Ctrl Pts',(15.895400461241,39.202897562529,-10.5474113287242));
#21465=CARTESIAN_POINT('Ctrl Pts',(16.0237150755281,39.0646352805704,-10.6271346454319));
#21466=CARTESIAN_POINT('Ctrl Pts',(16.3450613015928,38.7989404621379,-10.7492419669043));
#21467=CARTESIAN_POINT('Ctrl Pts',(16.5415157414198,38.6780472557562,-10.7838654920957));
#21468=CARTESIAN_POINT('Ctrl Pts',(16.9637457670055,38.4900400557353,-10.7881590891377));
#21469=CARTESIAN_POINT('Ctrl Pts',(17.1855617344222,38.424678866907,-10.7577973127706));
#21470=CARTESIAN_POINT('Ctrl Pts',(17.6001694073344,38.3627332511461,-10.6430146790677));
#21471=CARTESIAN_POINT('Ctrl Pts',(17.7902753536288,38.3593476957134,-10.5663096368531));
#21472=CARTESIAN_POINT('Ctrl Pts',(17.9682986698117,38.3820655716568,-10.4702558451031));
#21473=CARTESIAN_POINT('',(18.6832840733669,39.2833921172024,-9.34999999999999));
#21474=CARTESIAN_POINT('Ctrl Pts',(17.9682986698117,38.3820655716568,-10.4702558451031));
#21475=CARTESIAN_POINT('Ctrl Pts',(18.0868535859201,38.5519974267569,-10.2660883608694));
#21476=CARTESIAN_POINT('Ctrl Pts',(18.2113098794329,38.7182397514476,-10.0627168613312));
#21477=CARTESIAN_POINT('Ctrl Pts',(18.3416351067942,38.8807768634261,-9.86011239009425));
#21478=CARTESIAN_POINT('Ctrl Pts',(18.4513563585778,39.0176174103307,-9.68953899727404));
#21479=CARTESIAN_POINT('Ctrl Pts',(18.5652383532418,39.1518314157124,-9.5195087895761));
#21480=CARTESIAN_POINT('Ctrl Pts',(18.6832840733669,39.2833921172024,-9.34999999999999));
#21481=CARTESIAN_POINT('',(21.588763942955,37.7647358181594,-9.34999999999999));
#21482=CARTESIAN_POINT('Origin',(-3.46944695195361E-15,3.46944695195361E-15,
-9.34999999999999));
#21483=CARTESIAN_POINT('',(21.2339499719776,36.7011717789779,-10.4488603766068));
#21484=CARTESIAN_POINT('Ctrl Pts',(21.588763942955,37.7647358181594,-9.34999999999999));
#21485=CARTESIAN_POINT('Ctrl Pts',(21.5341817265093,37.5609700584441,-9.55398902691411));
#21486=CARTESIAN_POINT('Ctrl Pts',(21.473040884522,37.360079879705,-9.75864153761156));
#21487=CARTESIAN_POINT('Ctrl Pts',(21.4053736118279,37.1620811542006,-9.96398744092925));
#21488=CARTESIAN_POINT('Ctrl Pts',(21.3522562367029,37.0066563504785,-10.1251796235405));
#21489=CARTESIAN_POINT('Ctrl Pts',(21.2951163110683,36.8530135429274,-10.2867993162865));
#21490=CARTESIAN_POINT('Ctrl Pts',(21.2339499719776,36.7011717789779,-10.4488603766068));
#21491=CARTESIAN_POINT('',(23.2477447519555,35.4342359672547,-10.4702558450955));
#21492=CARTESIAN_POINT('Ctrl Pts',(21.2339499719779,36.7011717789774,-10.448860376607));
#21493=CARTESIAN_POINT('Ctrl Pts',(21.3127622302985,36.541717245301,-10.5474113287312));
#21494=CARTESIAN_POINT('Ctrl Pts',(21.4200940125319,36.3866012004346,-10.627134645438));
#21495=CARTESIAN_POINT('Ctrl Pts',(21.7003570822457,36.0778784359621,-10.749241966908));
#21496=CARTESIAN_POINT('Ctrl Pts',(21.8776070020259,35.9302573662764,-10.7838654920979));
#21497=CARTESIAN_POINT('Ctrl Pts',(22.2687831204933,35.6840742106644,-10.788159089137));
#21498=CARTESIAN_POINT('Ctrl Pts',(22.4790394541771,35.5878106009671,-10.7577973127683));
#21499=CARTESIAN_POINT('Ctrl Pts',(22.8806112385055,35.4674906783418,-10.6430146790628));
#21500=CARTESIAN_POINT('Ctrl Pts',(23.0683003656025,35.4370846859814,-10.5663096368471));
#21501=CARTESIAN_POINT('Ctrl Pts',(23.2477447519554,35.434235967254,-10.4702558450962));
#21502=CARTESIAN_POINT('',(24.0837247765699,36.2246352760995,-9.34999999999999));
#21503=CARTESIAN_POINT('Ctrl Pts',(23.2477447519555,35.4342359672547,-10.4702558450955));
#21504=CARTESIAN_POINT('Ctrl Pts',(23.3892767744334,35.5855660373794,-10.2660883608628));
#21505=CARTESIAN_POINT('Ctrl Pts',(23.5361250318794,35.7324042776236,-10.0627168613255));
#21506=CARTESIAN_POINT('Ctrl Pts',(23.6882551791415,35.8747397825072,-9.86011239008947));
#21507=CARTESIAN_POINT('Ctrl Pts',(23.816334067086,35.9945725277493,-9.68953899727089));
#21508=CARTESIAN_POINT('Ctrl Pts',(23.9481575517153,36.1112133304241,-9.51950878957455));
#21509=CARTESIAN_POINT('Ctrl Pts',(24.0837247765699,36.2246352760995,-9.34999999999999));
#21510=CARTESIAN_POINT('',(26.7435037248324,34.3079438107253,-9.34999999999999));
#21511=CARTESIAN_POINT('Origin',(-3.46944695195361E-15,3.46944695195361E-15,
-9.34999999999999));
#21512=CARTESIAN_POINT('',(26.2409403042474,33.3057006128359,-10.4488603766015));
#21513=CARTESIAN_POINT('Ctrl Pts',(26.7435037248324,34.3079438107253,-9.34999999999999));
#21514=CARTESIAN_POINT('Ctrl Pts',(26.6604781855094,34.1140199519472,-9.55398902691165));
#21515=CARTESIAN_POINT('Ctrl Pts',(26.5713700158378,33.9238757946105,-9.75864153760659));
#21516=CARTESIAN_POINT('Ctrl Pts',(26.4762133418134,33.7375224676141,-9.96398744092173));
#21517=CARTESIAN_POINT('Ctrl Pts',(26.4015173691717,33.5912390549401,-10.1251796235337));
#21518=CARTESIAN_POINT('Ctrl Pts',(26.3230933942815,33.4472919689108,-10.2867993162805));
#21519=CARTESIAN_POINT('Ctrl Pts',(26.2409403042474,33.3057006128359,-10.4488603766015));
#21520=CARTESIAN_POINT('',(28.0539337918648,31.7650675024716,-10.4702558450985));
#21521=CARTESIAN_POINT('Ctrl Pts',(26.2409403042471,33.3057006128354,-10.4488603766021));
#21522=CARTESIAN_POINT('Ctrl Pts',(26.2962576214637,33.1366529419271,-10.5474113291192));
#21523=CARTESIAN_POINT('Ctrl Pts',(26.3804216065228,32.9678408488418,-10.627134646066));
#21524=CARTESIAN_POINT('Ctrl Pts',(26.613896172857,32.6223748430022,-10.7492419673848));
#21525=CARTESIAN_POINT('Ctrl Pts',(26.768333275576,32.4510310493861,-10.7838654923528));
#21526=CARTESIAN_POINT('Ctrl Pts',(27.1204922694974,32.1516835176286,-10.7881590889247));
#21527=CARTESIAN_POINT('Ctrl Pts',(27.3149087568902,32.0264771367714,-10.7577973123325));
#21528=CARTESIAN_POINT('Ctrl Pts',(27.6952698084857,31.8502322746928,-10.6430146784569));
#21529=CARTESIAN_POINT('Ctrl Pts',(27.8767213062763,31.7934248240617,-10.5663096364667));
#21530=CARTESIAN_POINT('Ctrl Pts',(28.0539337918646,31.7650675024728,-10.4702558450978));
#21531=CARTESIAN_POINT('',(28.9938902950294,32.4284493240087,-9.34999999999999));
#21532=CARTESIAN_POINT('Ctrl Pts',(28.0539337918648,31.7650675024716,-10.4702558450985));
#21533=CARTESIAN_POINT('Ctrl Pts',(28.2155617375765,31.8947151443487,-10.2660883599894));
#21534=CARTESIAN_POINT('Ctrl Pts',(28.3818125526464,32.0191600975325,-10.0627168595826));
#21535=CARTESIAN_POINT('Ctrl Pts',(28.5526506894918,32.1383964553675,-9.86011238748669));
#21536=CARTESIAN_POINT('Ctrl Pts',(28.6964798960953,32.2387819492764,-9.68953899553826));
#21537=CARTESIAN_POINT('Ctrl Pts',(28.8435613239636,32.3354750783553,-9.51950878870877));
#21538=CARTESIAN_POINT('Ctrl Pts',(28.9938902950295,32.4284493240087,-9.34999999999999));
#21539=CARTESIAN_POINT('',(31.3538228927686,30.1527410032472,-9.34999999999999));
#21540=CARTESIAN_POINT('Origin',(-3.46944695195361E-15,3.46944695195361E-15,
-9.34999999999999));
#21541=CARTESIAN_POINT('',(30.7137407645493,29.2322214279229,-10.4488603766001));
#21542=CARTESIAN_POINT('Ctrl Pts',(31.3538228927686,30.1527410032472,-9.34999999999999));
#21543=CARTESIAN_POINT('Ctrl Pts',(31.2440441911241,29.9726067759396,-9.55398902690996));
#21544=CARTESIAN_POINT('Ctrl Pts',(31.128782679137,29.7970794267169,-9.7586415376032));
#21545=CARTESIAN_POINT('Ctrl Pts',(31.0080737192571,29.6261651145661,-9.9639874409166));
#21546=CARTESIAN_POINT('Ctrl Pts',(30.9133197436966,29.4920010013753,-10.1251796235298));
#21547=CARTESIAN_POINT('Ctrl Pts',(30.8152082055235,29.3606799844297,-10.2867993162779));
#21548=CARTESIAN_POINT('Ctrl Pts',(30.7137407645493,29.2322214279229,-10.4488603766001));
#21549=CARTESIAN_POINT('',(32.2890256406395,27.4492538662297,-10.4702558451021));
#21550=CARTESIAN_POINT('Ctrl Pts',(30.713740764549,29.232221427923,-10.4488603766003));
#21551=CARTESIAN_POINT('Ctrl Pts',(30.7444370392911,29.0570219435048,-10.5474113291176));
#21552=CARTESIAN_POINT('Ctrl Pts',(30.8037198906101,28.8779503301982,-10.6271346460648));
#21553=CARTESIAN_POINT('Ctrl Pts',(30.9856530837504,28.5027737750284,-10.7492419673845));
#21554=CARTESIAN_POINT('Ctrl Pts',(31.1141334751655,28.311195322877,-10.783865492353));
#21555=CARTESIAN_POINT('Ctrl Pts',(31.4201064027297,27.9647772671023,-10.7881590889261));
#21556=CARTESIAN_POINT('Ctrl Pts',(31.5947252847635,27.8131769557082,-10.7577973123345));
#21557=CARTESIAN_POINT('Ctrl Pts',(31.9461325502455,27.5845949906572,-10.64301467846));
#21558=CARTESIAN_POINT('Ctrl Pts',(32.1176525902707,27.5025425174008,-10.5663096364702));
#21559=CARTESIAN_POINT('Ctrl Pts',(32.2890256406393,27.4492538662306,-10.4702558451017));
#21560=CARTESIAN_POINT('',(33.313823818559,27.9721136596077,-9.34999999999999));
#21561=CARTESIAN_POINT('Ctrl Pts',(32.2890256406395,27.4492538662297,-10.4702558451021));
#21562=CARTESIAN_POINT('Ctrl Pts',(32.4674592300993,27.5545798270942,-10.2660883599925));
#21563=CARTESIAN_POINT('Ctrl Pts',(32.6497282149729,27.6540981522296,-10.0627168595853));
#21564=CARTESIAN_POINT('Ctrl Pts',(32.835796568896,27.74780805405,-9.86011238748894));
#21565=CARTESIAN_POINT('Ctrl Pts',(32.9924481468926,27.8267027380979,-9.68953899553974));
#21566=CARTESIAN_POINT('Ctrl Pts',(33.1517933649272,27.9014798009225,-9.51950878870952));
#21567=CARTESIAN_POINT('Ctrl Pts',(33.313823818559,27.9721136596077,-9.34999999999999));
#21568=CARTESIAN_POINT('',(35.3258686435729,25.383715342263,-9.34999999999999));
#21569=CARTESIAN_POINT('Origin',(-3.46944695195361E-15,3.46944695195361E-15,
-9.34999999999999));
#21570=CARTESIAN_POINT('',(34.5612980340057,24.5636585134986,-10.4488603765991));
#21571=CARTESIAN_POINT('Ctrl Pts',(35.3258686435729,25.383715342263,-9.34999999999999));
#21572=CARTESIAN_POINT('Ctrl Pts',(35.1915715573956,25.2210377598276,-9.55398902691078));
#21573=CARTESIAN_POINT('Ctrl Pts',(35.0525030950891,25.0637004493679,-9.75864153760484));
#21574=CARTESIAN_POINT('Ctrl Pts',(34.9086991356795,24.9117044745802,-9.96398744091905));
#21575=CARTESIAN_POINT('Ctrl Pts',(34.7958160748959,24.7923908553219,-10.1251796235311));
#21576=CARTESIAN_POINT('Ctrl Pts',(34.6800142414282,24.6763692246686,-10.286799316278));
#21577=CARTESIAN_POINT('Ctrl Pts',(34.5612980340057,24.5636585134986,-10.4488603765991));
#21578=CARTESIAN_POINT('',(35.8668060412405,22.5746525783803,-10.4702558451029));
#21579=CARTESIAN_POINT('Ctrl Pts',(34.561298034005,24.5636585134985,-10.4488603765997));
#21580=CARTESIAN_POINT('Ctrl Pts',(34.56674837864,24.3858737718396,-10.5474113291169));
#21581=CARTESIAN_POINT('Ctrl Pts',(34.5999432683243,24.2001880199589,-10.6271346460641));
#21582=CARTESIAN_POINT('Ctrl Pts',(34.7266314531113,23.8029384282025,-10.7492419673841));
#21583=CARTESIAN_POINT('Ctrl Pts',(34.8265396429607,23.5950253023348,-10.7838654923528));
#21584=CARTESIAN_POINT('Ctrl Pts',(35.0800977777163,23.2085887951713,-10.7881590889262));
#21585=CARTESIAN_POINT('Ctrl Pts',(35.2313643175126,23.0336806984012,-10.7577973123347));
#21586=CARTESIAN_POINT('Ctrl Pts',(35.5466641583307,22.7574149000112,-10.6430146784605));
#21587=CARTESIAN_POINT('Ctrl Pts',(35.7047610871982,22.6517877558659,-10.566309636471));
#21588=CARTESIAN_POINT('Ctrl Pts',(35.86680604124,22.5746525783811,-10.4702558451029));
#21589=CARTESIAN_POINT('',(36.9555839582819,22.9463464260082,-9.34999999999999));
#21590=CARTESIAN_POINT('Ctrl Pts',(35.8668060412405,22.5746525783803,-10.4702558451029));
#21591=CARTESIAN_POINT('Ctrl Pts',(36.0584128811214,22.653512725402,-10.2660883599983));
#21592=CARTESIAN_POINT('Ctrl Pts',(36.2529895648814,22.7260785163746,-10.062716859596));
#21593=CARTESIAN_POINT('Ctrl Pts',(36.4505003207673,22.792354298815,-9.86011238750467));
#21594=CARTESIAN_POINT('Ctrl Pts',(36.616785295779,22.8481521047499,-9.68953899555019));
#21595=CARTESIAN_POINT('Ctrl Pts',(36.7851504948585,22.8994908559617,-9.51950878871472));
#21596=CARTESIAN_POINT('Ctrl Pts',(36.9555839582819,22.9463464260082,-9.34999999999999));
#21597=CARTESIAN_POINT('',(38.5787815801853,20.0979504375039,-9.34999999999999));
#21598=CARTESIAN_POINT('Origin',(-3.46944695195361E-15,3.46944695195361E-15,
-9.34999999999999));
#21599=CARTESIAN_POINT('',(37.705286942044,19.3950503474818,-10.4488603765981));
#21600=CARTESIAN_POINT('Ctrl Pts',(38.5787815801853,20.0979504375039,-9.34999999999999));
#21601=CARTESIAN_POINT('Ctrl Pts',(38.4227000108675,19.9560411463938,-9.55398902691392));
#21602=CARTESIAN_POINT('Ctrl Pts',(38.2626556310921,19.820096808613,-9.75864153761112));
#21603=CARTESIAN_POINT('Ctrl Pts',(38.0986841060684,19.6901133709132,-9.9639874409285));
#21604=CARTESIAN_POINT('Ctrl Pts',(37.9699699336537,19.5880791268045,-10.1251796235371));
#21605=CARTESIAN_POINT('Ctrl Pts',(37.8388351962785,19.4897187482658,-10.2867993162805));
#21606=CARTESIAN_POINT('Ctrl Pts',(37.705286942044,19.3950503474818,-10.4488603765981));
#21607=CARTESIAN_POINT('',(38.7144417021698,17.2404964639591,-10.4702558451034));
#21608=CARTESIAN_POINT('Ctrl Pts',(37.7052869420443,19.3950503474814,-10.4488603765979));
#21609=CARTESIAN_POINT('Ctrl Pts',(37.6853804032726,19.2182995332333,-10.5474113291154));
#21610=CARTESIAN_POINT('Ctrl Pts',(37.6918115790941,19.0297796692134,-10.6271346460628));
#21611=CARTESIAN_POINT('Ctrl Pts',(37.7606757494237,18.6185438969855,-10.7492419673832));
#21612=CARTESIAN_POINT('Ctrl Pts',(37.8299778950733,18.3985286090725,-10.7838654923521));
#21613=CARTESIAN_POINT('Ctrl Pts',(38.0259595245977,17.9799403834156,-10.7881590889258));
#21614=CARTESIAN_POINT('Ctrl Pts',(38.1507943716225,17.7852851257265,-10.7577973123345));
#21615=CARTESIAN_POINT('Ctrl Pts',(38.4235681922673,17.4669594689679,-10.6430146784607));
#21616=CARTESIAN_POINT('Ctrl Pts',(38.5650236124193,17.3399079179848,-10.5663096364715));
#21617=CARTESIAN_POINT('Ctrl Pts',(38.7144417021694,17.2404964639595,-10.4702558451036));
#21618=CARTESIAN_POINT('',(39.8450349797172,17.4534577509763,-9.34999999999999));
#21619=CARTESIAN_POINT('Ctrl Pts',(38.7144417021698,17.2404964639591,-10.4702558451034));
#21620=CARTESIAN_POINT('Ctrl Pts',(38.9153212297648,17.2912854319613,-10.2660883599988));
#21621=CARTESIAN_POINT('Ctrl Pts',(39.118244592247,17.3354214585318,-10.0627168595964));
#21622=CARTESIAN_POINT('Ctrl Pts',(39.3231770006846,17.3729139377875,-9.86011238750502));
#21623=CARTESIAN_POINT('Ctrl Pts',(39.4957102901416,17.4044789831856,-9.68953899555042));
#21624=CARTESIAN_POINT('Ctrl Pts',(39.6696680403332,17.4313343138563,-9.51950878871483));
#21625=CARTESIAN_POINT('Ctrl Pts',(39.8450349797172,17.4534577509763,-9.34999999999999));
#21626=CARTESIAN_POINT('',(41.0463417758493,14.4030492195288,-9.34999999999999));
#21627=CARTESIAN_POINT('Origin',(-3.46944695195361E-15,3.46944695195361E-15,
-9.34999999999999));
#21628=CARTESIAN_POINT('',(40.081704941015,13.8316148870794,-10.4488603766));
#21629=CARTESIAN_POINT('Ctrl Pts',(41.0463417758493,14.4030492195288,-9.34999999999999));
#21630=CARTESIAN_POINT('Ctrl Pts',(40.8716530940425,14.2847970836798,-9.55398902691413));
#21631=CARTESIAN_POINT('Ctrl Pts',(40.6938908388429,14.1730131532654,-9.75864153761155));
#21632=CARTESIAN_POINT('Ctrl Pts',(40.5130897356021,14.067688340605,-9.96398744092918));
#21633=CARTESIAN_POINT('Ctrl Pts',(40.3711647009233,13.98501059461,-10.1251796235382));
#21634=CARTESIAN_POINT('Ctrl Pts',(40.2273665847295,13.9063138018416,-10.286799316282));
#21635=CARTESIAN_POINT('Ctrl Pts',(40.081704941015,13.8316148870794,-10.4488603766));
#21636=CARTESIAN_POINT('',(40.7739629732833,11.5553735590025,-10.4702558451001));
#21637=CARTESIAN_POINT('Ctrl Pts',(40.0817049410145,13.8316148870796,-10.4488603766004));
#21638=CARTESIAN_POINT('Ctrl Pts',(40.0368467585605,13.6594961371123,-10.5474113291177));
#21639=CARTESIAN_POINT('Ctrl Pts',(40.0163833003262,13.4719798817374,-10.6271346460648));
#21640=CARTESIAN_POINT('Ctrl Pts',(40.02602158028,13.0551295034541,-10.7492419673843));
#21641=CARTESIAN_POINT('Ctrl Pts',(40.0633068898957,12.8274909302863,-10.7838654923527));
#21642=CARTESIAN_POINT('Ctrl Pts',(40.197722393377,12.3852722353025,-10.7881590889254));
#21643=CARTESIAN_POINT('Ctrl Pts',(40.2935842701394,12.1748324364022,-10.7577973123335));
#21644=CARTESIAN_POINT('Ctrl Pts',(40.5182791822383,11.8209271136718,-10.6430146784588));
#21645=CARTESIAN_POINT('Ctrl Pts',(40.640213469245,11.6750375590429,-10.5663096364691));
#21646=CARTESIAN_POINT('Ctrl Pts',(40.7739629732828,11.5553735590024,-10.4702558451007));
#21647=CARTESIAN_POINT('',(41.9233559925618,11.6052670077401,-9.34999999999999));
#21648=CARTESIAN_POINT('Ctrl Pts',(40.7739629732833,11.5553735590025,-10.4702558451001));
#21649=CARTESIAN_POINT('Ctrl Pts',(40.9800258606994,11.5770574310607,-10.2660883599949));
#21650=CARTESIAN_POINT('Ctrl Pts',(41.1871649674267,11.5918652110069,-10.0627168595919));
#21651=CARTESIAN_POINT('Ctrl Pts',(41.3953471955567,11.5998111483204,-9.86011238749989));
#21652=CARTESIAN_POINT('Ctrl Pts',(41.5706165192284,11.6065008598841,-9.68953899554702));
#21653=CARTESIAN_POINT('Ctrl Pts',(41.7466255423886,11.6083260729267,-9.51950878871314));
#21654=CARTESIAN_POINT('Ctrl Pts',(41.9233559925618,11.6052670077401,-9.34999999999999));
#21655=CARTESIAN_POINT('',(42.6783168208273,8.41494345442032,-9.34999999999999));
#21656=CARTESIAN_POINT('Origin',(-3.46944695195361E-15,3.46944695195361E-15,
-9.34999999999999));
#21657=CARTESIAN_POINT('',(41.6421750134739,7.98660763468041,-10.4488603765993));
#21658=CARTESIAN_POINT('Ctrl Pts',(42.6783168208273,8.41494345442032,-9.34999999999999));
#21659=CARTESIAN_POINT('Ctrl Pts',(42.4885771843334,8.32275574630956,-9.55398902691263));
#21660=CARTESIAN_POINT('Ctrl Pts',(42.2967157806026,8.23740782172875,-9.75864153760853));
#21661=CARTESIAN_POINT('Ctrl Pts',(42.1027656882206,8.15888574356384,-9.96398744092461));
#21662=CARTESIAN_POINT('Ctrl Pts',(41.9505189757044,8.09724757616873,-10.1251796235349));
#21663=CARTESIAN_POINT('Ctrl Pts',(41.796984795657,8.03981640892943,-10.28679931628));
#21664=CARTESIAN_POINT('Ctrl Pts',(41.6421750134739,7.98660763468041,-10.4488603765993));
#21665=CARTESIAN_POINT('',(42.0034439406491,5.6350165713479,-10.4702558451019));
#21666=CARTESIAN_POINT('Ctrl Pts',(41.6421750134739,7.98660763468041,-10.4488603765993));
#21667=CARTESIAN_POINT('Ctrl Pts',(41.5732783705715,7.82262479039417,-10.5474113291168));
#21668=CARTESIAN_POINT('Ctrl Pts',(41.5263368552786,7.63992943387202,-10.6271346460642));
#21669=CARTESIAN_POINT('Ctrl Pts',(41.4765530372697,7.22595032113834,-10.7492419673841));
#21670=CARTESIAN_POINT('Ctrl Pts',(41.4810624894692,6.99532252760984,-10.7838654923528));
#21671=CARTESIAN_POINT('Ctrl Pts',(41.5511755548777,6.538475660675,-10.7881590889261));
#21672=CARTESIAN_POINT('Ctrl Pts',(41.616112990009,6.31653526801026,-10.7577973123345));
#21673=CARTESIAN_POINT('Ctrl Pts',(41.7881548531172,5.93425477109961,-10.6430146784602));
#21674=CARTESIAN_POINT('Ctrl Pts',(41.888085776524,5.77249710344601,-10.5663096364707));
#21675=CARTESIAN_POINT('Ctrl Pts',(42.0034439406485,5.6350165713482,-10.4702558451025));
#21676=CARTESIAN_POINT('',(43.1482383743694,5.52082649506359,-9.34999999999999));
#21677=CARTESIAN_POINT('Ctrl Pts',(42.0034439406491,5.6350165713479,-10.4702558451019));
#21678=CARTESIAN_POINT('Ctrl Pts',(42.2104953417366,5.62715392635685,-10.2660883599947));
#21679=CARTESIAN_POINT('Ctrl Pts',(42.4176334378376,5.61233201597956,-10.0627168595898));
#21680=CARTESIAN_POINT('Ctrl Pts',(42.624827495845,5.59056965497981,-9.86011238749592));
#21681=CARTESIAN_POINT('Ctrl Pts',(42.7992648757372,5.57224784947257,-9.68953899554438));
#21682=CARTESIAN_POINT('Ctrl Pts',(42.9737421357234,5.54900578881206,-9.51950878871182));
#21683=CARTESIAN_POINT('Ctrl Pts',(43.1482383743694,5.52082649506359,-9.34999999999999));
#21684=CARTESIAN_POINT('',(43.4414844094374,2.25553370726654,-9.34999999999999));
#21685=CARTESIAN_POINT('Origin',(-3.46944695195361E-15,3.46944695195361E-15,
-9.34999999999999));
#21686=CARTESIAN_POINT('Ctrl Pts',(43.4414844094374,2.25553370726654,-9.34999999999999));
#21687=CARTESIAN_POINT('Ctrl Pts',(43.2405563700923,2.19128710278242,-9.55398902691076));
#21688=CARTESIAN_POINT('Ctrl Pts',(43.0385015627283,2.13411262165513,-9.7586415376048));
#21689=CARTESIAN_POINT('Ctrl Pts',(42.8353507457808,2.08399176105678,-9.96398744091901));
#21690=CARTESIAN_POINT('Ctrl Pts',(42.67588165945,2.04464794759924,-10.1251796235315));
#21691=CARTESIAN_POINT('Ctrl Pts',(42.5157369286977,2.00965153883555,-10.2867993162788));
#21692=CARTESIAN_POINT('Ctrl Pts',(42.3549304887758,1.97901608230145,-10.4488603766003));
#21693=CARTESIAN_POINT('Origin',(-1.73472347597681E-15,-1.73472347597681E-15,
11.35));
#21694=CARTESIAN_POINT('Ctrl Pts',(8.41494345441915,-42.6783168208275,-9.34999999999999));
#21695=CARTESIAN_POINT('Ctrl Pts',(8.47350165196269,-42.6667708190677,-8.81583928864268));
#21696=CARTESIAN_POINT('Ctrl Pts',(8.53749789216075,-42.6540295511139,-8.29847152339217));
#21697=CARTESIAN_POINT('Ctrl Pts',(8.67708507802148,-42.6258516250367,-7.21668429187557));
#21698=CARTESIAN_POINT('Ctrl Pts',(8.74798535871021,-42.6113531950663,-6.68828131371252));
#21699=CARTESIAN_POINT('Ctrl Pts',(8.8148974458234,-42.5975067699932,-6.16441400296899));
#21700=CARTESIAN_POINT('Ctrl Pts',(10.821785190392,-42.1323980482125,-6.16441400296898));
#21701=CARTESIAN_POINT('Ctrl Pts',(10.9673906983499,-42.0949990013352,-6.69963387813806));
#21702=CARTESIAN_POINT('Ctrl Pts',(11.1049325306235,-42.0588790443691,-7.21760449588555));
#21703=CARTESIAN_POINT('Ctrl Pts',(11.369604888333,-41.988102864666,-8.28098049190398));
#21704=CARTESIAN_POINT('Ctrl Pts',(11.4933208311464,-41.9543450495947,-8.81289306231308));
#21705=CARTESIAN_POINT('Ctrl Pts',(11.6052670077404,-41.9233559925617,-9.34999999999999));
#21706=CARTESIAN_POINT('Origin',(-1.73472347597681E-15,-1.73472347597681E-15,
11.35));
#21707=CARTESIAN_POINT('Ctrl Pts',(4.71556960657991,-43.2436515951822,-6.16441400296899));
#21708=CARTESIAN_POINT('Ctrl Pts',(4.86501549971827,-43.2273550409941,-6.69963387813254));
#21709=CARTESIAN_POINT('Ctrl Pts',(5.00629776029487,-43.2111769767249,-7.21760449588749));
#21710=CARTESIAN_POINT('Ctrl Pts',(5.27834863560216,-43.1787880002625,-8.28098049191805));
#21711=CARTESIAN_POINT('Ctrl Pts',(5.405609566491,-43.1629804054675,-8.81289306231201));
#21712=CARTESIAN_POINT('Ctrl Pts',(5.52082649506267,-43.1482383743695,-9.34999999999999));
#21713=CARTESIAN_POINT('Ctrl Pts',(2.25553370726645,-43.4414844094374,-9.34999999999999));
#21714=CARTESIAN_POINT('Ctrl Pts',(2.31513903416692,-43.4383896297404,-8.81583928864891));
#21715=CARTESIAN_POINT('Ctrl Pts',(2.38029715641292,-43.4348856640963,-8.29847152332599));
#21716=CARTESIAN_POINT('Ctrl Pts',(2.52247368297688,-43.4268598764585,-7.21668429184531));
#21717=CARTESIAN_POINT('Ctrl Pts',(2.5947156427552,-43.4225991815798,-6.68828131367592));
#21718=CARTESIAN_POINT('Ctrl Pts',(2.66291721304302,-43.4184162760053,-6.16441400296897));
#21719=CARTESIAN_POINT('Origin',(-1.73472347597681E-15,-1.73472347597681E-15,
11.35));
#21720=CARTESIAN_POINT('Ctrl Pts',(14.4030492195297,-41.046341775849,-9.34999999999999));
#21721=CARTESIAN_POINT('Ctrl Pts',(14.4593682116851,-41.0265795953254,-8.81583928864243));
#21722=CARTESIAN_POINT('Ctrl Pts',(14.5208997909382,-41.0048604005364,-8.29847152344933));
#21723=CARTESIAN_POINT('Ctrl Pts',(14.6550564651938,-40.9571038072317,-7.21668089174327));
#21724=CARTESIAN_POINT('Ctrl Pts',(14.7231709221295,-40.9326630822678,-6.68828455624565));
#21725=CARTESIAN_POINT('Ctrl Pts',(14.787431786677,-40.9094348672085,-6.16441400296898));
#21726=CARTESIAN_POINT('Ctrl Pts',(16.7077004351884,-40.1634503767792,-6.16441400296897));
#21727=CARTESIAN_POINT('Ctrl Pts',(16.8465014496973,-40.105710173964,-6.69963387810965));
#21728=CARTESIAN_POINT('Ctrl Pts',(16.9775028986062,-40.0503836224622,-7.21760449589626));
#21729=CARTESIAN_POINT('Ctrl Pts',(17.2294087727606,-39.9426610384398,-8.28098049186901));
#21730=CARTESIAN_POINT('Ctrl Pts',(17.347061227683,-39.8916402148512,-8.81289306231304));
#21731=CARTESIAN_POINT('Ctrl Pts',(17.4534577509835,-39.8450349797141,-9.34999999999999));
#21732=CARTESIAN_POINT('Origin',(-1.73472347597681E-15,-1.73472347597681E-15,
11.35));
#21733=CARTESIAN_POINT('Ctrl Pts',(20.0979504375088,-38.5787815801827,-9.35));
#21734=CARTESIAN_POINT('Ctrl Pts',(20.1508837319947,-38.5512055219067,-8.81583928863476));
#21735=CARTESIAN_POINT('Ctrl Pts',(20.2086980447853,-38.520950540461,-8.29847152350441));
#21736=CARTESIAN_POINT('Ctrl Pts',(20.334692329685,-38.4545877635936,-7.21668429184472));
#21737=CARTESIAN_POINT('Ctrl Pts',(20.3986359710957,-38.4207017045448,-6.68828131367372));
#21738=CARTESIAN_POINT('Ctrl Pts',(20.4589366597946,-38.38856484359,-6.16441400296897));
#21739=CARTESIAN_POINT('Ctrl Pts',(22.2534950801302,-37.3768906775112,-6.16441400296898));
#21740=CARTESIAN_POINT('Ctrl Pts',(22.382666012821,-37.2999847427738,-6.69963387809245));
#21741=CARTESIAN_POINT('Ctrl Pts',(22.5044602666517,-37.2265778857695,-7.21760449589733));
#21742=CARTESIAN_POINT('Ctrl Pts',(22.7384715801301,-37.0841018185718,-8.28098049198328));
#21743=CARTESIAN_POINT('Ctrl Pts',(22.8476654824114,-37.0168566233269,-8.81289306231471));
#21744=CARTESIAN_POINT('Ctrl Pts',(22.9463464260018,-36.9555839582859,-9.34999999999999));
#21745=CARTESIAN_POINT('Origin',(-1.73472347597681E-15,-1.73472347597681E-15,
11.35));
#21746=CARTESIAN_POINT('Ctrl Pts',(25.3837153422573,-35.325868643577,-9.34999999999999));
#21747=CARTESIAN_POINT('Ctrl Pts',(25.4321853698649,-35.2910400765618,-8.81583928865113));
#21748=CARTESIAN_POINT('Ctrl Pts',(25.4851054835569,-35.2528652126025,-8.29847152324279));
#21749=CARTESIAN_POINT('Ctrl Pts',(25.6003732827136,-35.16924679404,-7.21668089167132));
#21750=CARTESIAN_POINT('Ctrl Pts',(25.6588428776096,-35.1266060300569,-6.68828455616324));
#21751=CARTESIAN_POINT('Ctrl Pts',(25.7139565811959,-35.0862143432485,-6.16441400296897));
#21752=CARTESIAN_POINT('Ctrl Pts',(27.3462727390257,-33.829445270102,-6.16441400296898));
#21753=CARTESIAN_POINT('Ctrl Pts',(27.4631840422152,-33.7349391864884,-6.69963387811431));
#21754=CARTESIAN_POINT('Ctrl Pts',(27.5732917211693,-33.6449463759102,-7.21760449589188));
#21755=CARTESIAN_POINT('Ctrl Pts',(27.7846446784427,-33.4706172274022,-8.28098049202515));
#21756=CARTESIAN_POINT('Ctrl Pts',(27.8831571551483,-33.3885165787492,-8.81289306232346));
#21757=CARTESIAN_POINT('Ctrl Pts',(27.9721136596011,-33.3138238185646,-9.34999999999998));
#21758=CARTESIAN_POINT('Origin',(-1.73472347597681E-15,-1.73472347597681E-15,
11.35));
#21759=CARTESIAN_POINT('Ctrl Pts',(30.15274100324,-31.3538228927755,-9.34999999999999));
#21760=CARTESIAN_POINT('Ctrl Pts',(30.195761053975,-31.3124508262114,-8.81583928863301));
#21761=CARTESIAN_POINT('Ctrl Pts',(30.2427096676391,-31.2671332098872,-8.29847152309517));
#21762=CARTESIAN_POINT('Ctrl Pts',(30.344904065072,-31.1679615880787,-7.21668089169457));
#21763=CARTESIAN_POINT('Ctrl Pts',(30.3967101103647,-31.1174337546518,-6.6882845561955));
#21764=CARTESIAN_POINT('Ctrl Pts',(30.44551449954,-31.0696096991627,-6.16441400296898));
#21765=CARTESIAN_POINT('Ctrl Pts',(31.8823591451049,-29.5933299130488,-6.16441400296898));
#21766=CARTESIAN_POINT('Ctrl Pts',(31.984630841798,-29.4831475518908,-6.69963387813157));
#21767=CARTESIAN_POINT('Ctrl Pts',(32.0808104710531,-29.378400781849,-7.21760449588776));
#21768=CARTESIAN_POINT('Ctrl Pts',(32.2652025353894,-29.1757673907798,-8.28098049202437));
#21769=CARTESIAN_POINT('Ctrl Pts',(32.3510281565927,-29.0804826211578,-8.81289306233601));
#21770=CARTESIAN_POINT('Ctrl Pts',(32.4284493240119,-28.9938902950258,-9.34999999999999));
#21771=CARTESIAN_POINT('Origin',(-1.73472347597681E-15,-1.73472347597681E-15,
11.35));
#21772=CARTESIAN_POINT('Ctrl Pts',(34.3079438107283,-26.7435037248284,-9.34999999999999));
#21773=CARTESIAN_POINT('Ctrl Pts',(34.3446381204109,-26.6964303746902,-8.81583928862145));
#21774=CARTESIAN_POINT('Ctrl Pts',(34.3846594956414,-26.6448925420002,-8.29847152310463));
#21775=CARTESIAN_POINT('Ctrl Pts',(34.4717001081413,-26.5321865651654,-7.21668089171778));
#21776=CARTESIAN_POINT('Ctrl Pts',(34.51578798215,-26.4748002632685,-6.68828455622075));
#21777=CARTESIAN_POINT('Ctrl Pts',(34.5572895402933,-26.4205173989522,-6.16441400296898));
#21778=CARTESIAN_POINT('Ctrl Pts',(35.7694126601179,-24.7547796990844,-6.16441400296898));
#21779=CARTESIAN_POINT('Ctrl Pts',(35.8549627934919,-24.6311640555206,-6.69963387812577));
#21780=CARTESIAN_POINT('Ctrl Pts',(35.9352564331632,-24.5137956681819,-7.21760449588857));
#21781=CARTESIAN_POINT('Ctrl Pts',(36.0889339138623,-24.2869830660677,-8.28098049192201));
#21782=CARTESIAN_POINT('Ctrl Pts',(36.1603255174261,-24.1804538985912,-8.81289306230615));
#21783=CARTESIAN_POINT('Ctrl Pts',(36.2246352761032,-24.0837247765644,-9.34999999999999));
#21784=CARTESIAN_POINT('Origin',(-1.73472347597681E-15,-1.73472347597681E-15,
11.35));
#21785=CARTESIAN_POINT('Ctrl Pts',(37.7647352670483,-21.588764907001,-9.35000993815262));
#21786=CARTESIAN_POINT('Ctrl Pts',(37.7943568453571,-21.5369485509418,-8.81584922680642));
#21787=CARTESIAN_POINT('Ctrl Pts',(37.8266368134661,-21.4802386995136,-8.29847152338959));
#21788=CARTESIAN_POINT('Ctrl Pts',(37.8967517451859,-21.3562927362902,-7.21668089172103));
#21789=CARTESIAN_POINT('Ctrl Pts',(37.9322239459333,-21.2932161855427,-6.68828455622328));
#21790=CARTESIAN_POINT('Ctrl Pts',(37.9655778209991,-21.23357955498,-6.16441400296897));
#21791=CARTESIAN_POINT('Ctrl Pts',(38.9283040838375,-19.4122935573384,-6.16441400296897));
#21792=CARTESIAN_POINT('Ctrl Pts',(38.9953910998897,-19.2777610893824,-6.69963387815563));
#21793=CARTESIAN_POINT('Ctrl Pts',(39.0581642030152,-19.150160366662,-7.21760449588037));
#21794=CARTESIAN_POINT('Ctrl Pts',(39.1779986697582,-18.9037858039865,-8.28098049192675));
#21795=CARTESIAN_POINT('Ctrl Pts',(39.2335029284966,-18.7881808653144,-8.8128930623207));
#21796=CARTESIAN_POINT('Ctrl Pts',(39.2833921172024,-18.6832840733669,-9.35));
#21797=CARTESIAN_POINT('Origin',(-1.73472347597681E-15,-1.73472347597681E-15,
11.35));
#21798=CARTESIAN_POINT('Ctrl Pts',(40.4527467088507,-15.9945391840333,-9.34999999999999));
#21799=CARTESIAN_POINT('Ctrl Pts',(40.4746925458677,-15.9390346536464,-8.81583928863806));
#21800=CARTESIAN_POINT('Ctrl Pts',(40.4985728888029,-15.8783091409716,-8.29847152339854));
#21801=CARTESIAN_POINT('Ctrl Pts',(40.5503346392115,-15.7456467907431,-7.21668429190581));
#21802=CARTESIAN_POINT('Ctrl Pts',(40.5764693694874,-15.6781632361046,-6.68828131374606));
#21803=CARTESIAN_POINT('Ctrl Pts',(40.6009964209531,-15.614387263859,-6.16441400296897));
#21804=CARTESIAN_POINT('Ctrl Pts',(41.2947274963708,-13.6746290991923,-6.16441400296898));
#21805=CARTESIAN_POINT('Ctrl Pts',(41.3419856969081,-13.5319184999507,-6.69963387813235));
#21806=CARTESIAN_POINT('Ctrl Pts',(41.3859603841398,-13.3966830245769,-7.21760449588791));
#21807=CARTESIAN_POINT('Ctrl Pts',(41.469512352753,-13.1357619769634,-8.28098049188705));
#21808=CARTESIAN_POINT('Ctrl Pts',(41.5079993600206,-13.0134346502621,-8.81289306230997));
#21809=CARTESIAN_POINT('Ctrl Pts',(41.5424523787385,-12.9025055845851,-9.34999999999999));
#21810=CARTESIAN_POINT('Origin',(-1.73472347597681E-15,-1.73472347597681E-15,
11.35));
#21811=CARTESIAN_POINT('Ctrl Pts',(42.31725633263,-10.0747117317813,-9.34999999999999));
#21812=CARTESIAN_POINT('Ctrl Pts',(42.3310796744042,-10.0166489392364,-8.81583928865039));
#21813=CARTESIAN_POINT('Ctrl Pts',(42.3460748083624,-9.95314299759242,-8.29847152349818));
#21814=CARTESIAN_POINT('Ctrl Pts',(42.3784298778726,-9.81446449364917,-7.21668429186938));
#21815=CARTESIAN_POINT('Ctrl Pts',(42.3946946831139,-9.74394846437754,-6.68828131370223));
#21816=CARTESIAN_POINT('Ctrl Pts',(42.4098958173845,-9.67733107621064,-6.16441400296897));
#21817=CARTESIAN_POINT('Ctrl Pts',(42.8205093412358,-7.65858862696908,-6.16441400296897));
#21818=CARTESIAN_POINT('Ctrl Pts',(42.8469766855802,-7.5106050726955,-6.69963387810951));
#21819=CARTESIAN_POINT('Ctrl Pts',(42.8712577590976,-7.37048784895445,-7.21760449589371));
#21820=CARTESIAN_POINT('Ctrl Pts',(42.9168263524529,-7.10033191646616,-8.28098049196745));
#21821=CARTESIAN_POINT('Ctrl Pts',(42.9375126237602,-6.97377243337836,-8.8128930623116));
#21822=CARTESIAN_POINT('Ctrl Pts',(42.9558281083822,-6.85906928986171,-9.34999999999999));
#21823=CARTESIAN_POINT('Origin',(-1.73472347597681E-15,-1.73472347597681E-15,
11.35));
#21824=CARTESIAN_POINT('Ctrl Pts',(43.3203086503665,-3.94979220174698,-9.34999999999999));
#21825=CARTESIAN_POINT('Ctrl Pts',(43.325728093523,-3.8903531380549,-8.81583928863827));
#21826=CARTESIAN_POINT('Ctrl Pts',(43.3315327608277,-3.82535956522521,-8.29847152323037));
#21827=CARTESIAN_POINT('Ctrl Pts',(43.3438225321466,-3.68348755612829,-7.21668089169733));
#21828=CARTESIAN_POINT('Ctrl Pts',(43.3498862347432,-3.61137542267607,-6.68828455619463));
#21829=CARTESIAN_POINT('Ctrl Pts',(43.3554520350114,-3.54327233497895,-6.16441400296897));
#21830=CARTESIAN_POINT('Ctrl Pts',(43.4745891000668,-1.48664137583803,-6.16441400296898));
#21831=CARTESIAN_POINT('Ctrl Pts',(43.4797267894152,-1.33639738493906,-6.69963387812117));
#21832=CARTESIAN_POINT('Ctrl Pts',(43.4838199565783,-1.19425079545893,-7.2176044958904));
#21833=CARTESIAN_POINT('Ctrl Pts',(43.4904775295168,-0.920359573847044,
-8.28098049193426));
#21834=CARTESIAN_POINT('Ctrl Pts',(43.492941952042,-0.792144320447485,-8.81289306231382));
#21835=CARTESIAN_POINT('Ctrl Pts',(43.4947470521204,-0.676002124309745,
-9.34999999999999));
#21836=CARTESIAN_POINT('Origin',(-1.73472347597681E-15,-1.73472347597681E-15,
11.35));
#21837=CARTESIAN_POINT('Ctrl Pts',(43.4414844094373,2.25553370726654,-9.34999999999999));
#21838=CARTESIAN_POINT('Ctrl Pts',(43.4383896297404,2.31513903416689,-8.81583928864678));
#21839=CARTESIAN_POINT('Ctrl Pts',(43.4348856640966,2.38029715640743,-8.29847152336333));
#21840=CARTESIAN_POINT('Ctrl Pts',(43.4268598764586,2.52247368297485,-7.21668429185844));
#21841=CARTESIAN_POINT('Ctrl Pts',(43.4225991815799,2.59471564275292,-6.6882813136911));
#21842=CARTESIAN_POINT('Ctrl Pts',(43.4184162760054,2.6629172130419,-6.16441400296898));
#21843=CARTESIAN_POINT('Ctrl Pts',(43.2436515951818,4.71556960658336,-6.16441400296898));
#21844=CARTESIAN_POINT('Ctrl Pts',(43.2273550409942,4.86501549971759,-6.6996338781248));
#21845=CARTESIAN_POINT('Ctrl Pts',(43.2111769767249,5.00629776029513,-7.21760449588901));
#21846=CARTESIAN_POINT('Ctrl Pts',(43.1787880002636,5.27834863559312,-8.28098049188509));
#21847=CARTESIAN_POINT('Ctrl Pts',(43.1629804054676,5.40560956649083,-8.81289306230564));
#21848=CARTESIAN_POINT('Ctrl Pts',(43.1482383743694,5.52082649506359,-9.34999999999999));
#21849=CARTESIAN_POINT('Origin',(-1.73472347597681E-15,-1.73472347597681E-15,
11.35));
#21850=CARTESIAN_POINT('Ctrl Pts',(42.6783168208273,8.41494345442032,-9.34999999999999));
#21851=CARTESIAN_POINT('Ctrl Pts',(42.6667708190677,8.47350165196264,-8.81583928865448));
#21852=CARTESIAN_POINT('Ctrl Pts',(42.654029551117,8.53749789214549,-8.29847152350322));
#21853=CARTESIAN_POINT('Ctrl Pts',(42.625851536471,8.67708551675633,-7.21668089172215));
#21854=CARTESIAN_POINT('Ctrl Pts',(42.6113532807691,8.74798494455602,-6.68828455622002));
#21855=CARTESIAN_POINT('Ctrl Pts',(42.5975067699923,8.81489744582799,-6.16441400296898));
#21856=CARTESIAN_POINT('Ctrl Pts',(42.1323980482129,10.8217851903902,-6.16441400296898));
#21857=CARTESIAN_POINT('Ctrl Pts',(42.0949990013376,10.9673906983404,-6.69963387811488));
#21858=CARTESIAN_POINT('Ctrl Pts',(42.0588790443691,11.1049325306234,-7.21760449589152));
#21859=CARTESIAN_POINT('Ctrl Pts',(41.9881028646612,11.3696048883509,-8.28098049197336));
#21860=CARTESIAN_POINT('Ctrl Pts',(41.9543450495945,11.4933208311469,-8.81289306231959));
#21861=CARTESIAN_POINT('Ctrl Pts',(41.9233559925618,11.60526700774,-9.34999999999999));
#21862=CARTESIAN_POINT('Origin',(-1.73472347597681E-15,-1.73472347597681E-15,
11.35));
#21863=CARTESIAN_POINT('Ctrl Pts',(41.0463417758493,14.4030492195288,-9.34999999999999));
#21864=CARTESIAN_POINT('Ctrl Pts',(41.0265795953255,14.4593682116847,-8.81583928863649));
#21865=CARTESIAN_POINT('Ctrl Pts',(41.0048604005271,14.5208997909645,-8.29847152324346));
#21866=CARTESIAN_POINT('Ctrl Pts',(40.9571039573323,14.6550560435348,-7.21668429184298));
#21867=CARTESIAN_POINT('Ctrl Pts',(40.9326629384941,14.7231713198794,-6.6882813136778));
#21868=CARTESIAN_POINT('Ctrl Pts',(40.9094348672085,14.7874317866772,-6.16441400296898));
#21869=CARTESIAN_POINT('Ctrl Pts',(40.1634514154035,16.7076979384513,-6.16440437552831));
#21870=CARTESIAN_POINT('Ctrl Pts',(40.105711212588,16.8464989529609,-6.69962425066112));
#21871=CARTESIAN_POINT('Ctrl Pts',(40.0503836224625,16.9775028986055,-7.21760449589682));
#21872=CARTESIAN_POINT('Ctrl Pts',(39.9426610384324,17.2294087727778,-8.28098049193118));
#21873=CARTESIAN_POINT('Ctrl Pts',(39.891640214852,17.3470612276812,-8.81289306231108));
#21874=CARTESIAN_POINT('Ctrl Pts',(39.8450349797172,17.4534577509763,-9.34999999999999));
#21875=CARTESIAN_POINT('Origin',(-1.73472347597681E-15,-1.73472347597681E-15,
11.35));
#21876=CARTESIAN_POINT('Ctrl Pts',(38.5787815801853,20.0979504375039,-9.34999999999999));
#21877=CARTESIAN_POINT('Ctrl Pts',(38.551205521908,20.1508837319923,-8.81583928865653));
#21878=CARTESIAN_POINT('Ctrl Pts',(38.5209505404534,20.2086980447997,-8.29847152339421));
#21879=CARTESIAN_POINT('Ctrl Pts',(38.4545875550103,20.3346927256946,-7.21668089168163));
#21880=CARTESIAN_POINT('Ctrl Pts',(38.420701903461,20.3986355978551,-6.68828455617096));
#21881=CARTESIAN_POINT('Ctrl Pts',(38.3885648435948,20.4589366597857,-6.16441400296898));
#21882=CARTESIAN_POINT('Ctrl Pts',(37.3768906775087,22.2534950801344,-6.16441400296899));
#21883=CARTESIAN_POINT('Ctrl Pts',(37.299984742768,22.3826660128308,-6.69963387811716));
#21884=CARTESIAN_POINT('Ctrl Pts',(37.2265778857701,22.5044602666508,-7.21760449589159));
#21885=CARTESIAN_POINT('Ctrl Pts',(37.0841018185842,22.7384715801098,-8.28098049189961));
#21886=CARTESIAN_POINT('Ctrl Pts',(37.0168566233263,22.8476654824123,-8.81289306230973));
#21887=CARTESIAN_POINT('Ctrl Pts',(36.9555839582819,22.9463464260082,-9.34999999999999));
#21888=CARTESIAN_POINT('Origin',(-1.73472347597681E-15,-1.73472347597681E-15,
11.35));
#21889=CARTESIAN_POINT('Ctrl Pts',(35.3258686435729,25.383715342263,-9.34999999999999));
#21890=CARTESIAN_POINT('Ctrl Pts',(35.2910400765608,25.4321853698662,-8.8158392886509));
#21891=CARTESIAN_POINT('Ctrl Pts',(35.2528652126222,25.4851054835298,-8.29847152347939));
#21892=CARTESIAN_POINT('Ctrl Pts',(35.1692467940428,25.6003732827099,-7.2166808917155));
#21893=CARTESIAN_POINT('Ctrl Pts',(35.1266060300575,25.6588428776089,-6.6882845562118));
#21894=CARTESIAN_POINT('Ctrl Pts',(35.0862143432449,25.7139565812008,-6.16441400296898));
#21895=CARTESIAN_POINT('Ctrl Pts',(33.8294452700945,27.346272739035,-6.16441400296899));
#21896=CARTESIAN_POINT('Ctrl Pts',(33.7349391864853,27.463184042219,-6.69963387811333));
#21897=CARTESIAN_POINT('Ctrl Pts',(33.6449463759122,27.5732917211668,-7.21760449589191));
#21898=CARTESIAN_POINT('Ctrl Pts',(33.4706172274441,27.7846446783919,-8.28098049178978));
#21899=CARTESIAN_POINT('Ctrl Pts',(33.388516578751,27.8831571551463,-8.81289306227819));
#21900=CARTESIAN_POINT('Ctrl Pts',(33.313823818559,27.9721136596077,-9.34999999999999));
#21901=CARTESIAN_POINT('Origin',(-1.73472347597681E-15,-1.73472347597681E-15,
11.35));
#21902=CARTESIAN_POINT('Ctrl Pts',(31.3538228927686,30.1527410032472,-9.34999999999999));
#21903=CARTESIAN_POINT('Ctrl Pts',(31.3124508262117,30.1957610539746,-8.81583928870648));
#21904=CARTESIAN_POINT('Ctrl Pts',(31.2671332099589,30.2427096675652,-8.29847152382584));
#21905=CARTESIAN_POINT('Ctrl Pts',(31.1679615880845,30.344904065066,-7.2166808917017));
#21906=CARTESIAN_POINT('Ctrl Pts',(31.1174337546515,30.396710110365,-6.68828455619383));
#21907=CARTESIAN_POINT('Ctrl Pts',(31.0696096991581,30.4455144995446,-6.16441400296898));
#21908=CARTESIAN_POINT('Ctrl Pts',(29.5933299130457,31.8823591451077,-6.16441400296898));
#21909=CARTESIAN_POINT('Ctrl Pts',(29.4831475518988,31.9846308417905,-6.69963387809554));
#21910=CARTESIAN_POINT('Ctrl Pts',(29.3784007818486,32.0808104710534,-7.2176044958975));
#21911=CARTESIAN_POINT('Ctrl Pts',(29.1757673907945,32.265202535376,-8.28098049194909));
#21912=CARTESIAN_POINT('Ctrl Pts',(29.0804826211604,32.3510281565903,-8.81289306230641));
#21913=CARTESIAN_POINT('Ctrl Pts',(28.9938902950294,32.4284493240087,-9.34999999999999));
#21914=CARTESIAN_POINT('Origin',(-1.73472347597681E-15,-1.73472347597681E-15,
11.35));
#21915=CARTESIAN_POINT('Ctrl Pts',(26.7435037248324,34.3079438107253,-9.34999999999999));
#21916=CARTESIAN_POINT('Ctrl Pts',(26.6964303746913,34.34463812041,-8.81583928865456));
#21917=CARTESIAN_POINT('Ctrl Pts',(26.6448925420221,34.3846594956245,-8.29847152331405));
#21918=CARTESIAN_POINT('Ctrl Pts',(26.5321865651601,34.4717001081453,-7.21668089167348));
#21919=CARTESIAN_POINT('Ctrl Pts',(26.4748002632605,34.5157879821561,-6.68828455616666));
#21920=CARTESIAN_POINT('Ctrl Pts',(26.4205173989462,34.5572895402979,-6.16441400296898));
#21921=CARTESIAN_POINT('Ctrl Pts',(24.7547796990912,35.7694126601132,-6.16441400296897));
#21922=CARTESIAN_POINT('Ctrl Pts',(24.631164055528,35.8549627934868,-6.69963387811261));
#21923=CARTESIAN_POINT('Ctrl Pts',(24.5137956681809,35.9352564331639,-7.21760449589143));
#21924=CARTESIAN_POINT('Ctrl Pts',(24.2869830660353,36.0889339138842,-8.28098049206058));
#21925=CARTESIAN_POINT('Ctrl Pts',(24.1804538985909,36.1603255174263,-8.8128930623247));
#21926=CARTESIAN_POINT('Ctrl Pts',(24.0837247765699,36.2246352760995,-9.34999999999999));
#21927=CARTESIAN_POINT('Origin',(-1.73472347597681E-15,-1.73472347597681E-15,
11.35));
#21928=CARTESIAN_POINT('Ctrl Pts',(21.588763942955,37.7647358181594,-9.34999999999999));
#21929=CARTESIAN_POINT('Ctrl Pts',(21.536947586891,37.7943573964709,-8.81583928863289));
#21930=CARTESIAN_POINT('Ctrl Pts',(21.4802386994667,37.8266368134926,-8.29847152300709));
#21931=CARTESIAN_POINT('Ctrl Pts',(21.3562931258567,37.8967515248122,-7.21668429183446));
#21932=CARTESIAN_POINT('Ctrl Pts',(21.2932158164189,37.9322241523787,-6.68828131367098));
#21933=CARTESIAN_POINT('Ctrl Pts',(21.2335795549855,37.965577820996,-6.16441400296897));
#21934=CARTESIAN_POINT('Ctrl Pts',(19.4122959772784,38.9283028770912,-6.1644043755283));
#21935=CARTESIAN_POINT('Ctrl Pts',(19.277763509337,38.995389893136,-6.699624250679));
#21936=CARTESIAN_POINT('Ctrl Pts',(19.1501603666614,39.0581642030155,-7.21760449589032));
#21937=CARTESIAN_POINT('Ctrl Pts',(18.9037858040018,39.1779986697508,-8.28098049186625));
#21938=CARTESIAN_POINT('Ctrl Pts',(18.7881808653155,39.233502928496,-8.81289306230204));
#21939=CARTESIAN_POINT('Ctrl Pts',(18.6832840733669,39.2833921172024,-9.34999999999999));
#21940=CARTESIAN_POINT('Origin',(-1.73472347597681E-15,-1.73472347597681E-15,
11.35));
#21941=CARTESIAN_POINT('Ctrl Pts',(15.9945391840345,40.4527467088502,-9.34999999999999));
#21942=CARTESIAN_POINT('Ctrl Pts',(15.9390346536467,40.4746925458676,-8.81583928865999));
#21943=CARTESIAN_POINT('Ctrl Pts',(15.8783091409914,40.4985728887952,-8.29847152355329));
#21944=CARTESIAN_POINT('Ctrl Pts',(15.7456467907371,40.5503346392138,-7.21668429185831));
#21945=CARTESIAN_POINT('Ctrl Pts',(15.6781632360945,40.5764693694913,-6.68828131368947));
#21946=CARTESIAN_POINT('Ctrl Pts',(15.6143872638506,40.6009964209563,-6.16441400296898));
#21947=CARTESIAN_POINT('Ctrl Pts',(13.6746290992085,41.2947274963655,-6.16441400296897));
#21948=CARTESIAN_POINT('Ctrl Pts',(13.531918499964,41.3419856969037,-6.69963387811841));
#21949=CARTESIAN_POINT('Ctrl Pts',(13.3966830245759,41.3859603841401,-7.21760449588863));
#21950=CARTESIAN_POINT('Ctrl Pts',(13.1357619769188,41.4695123527673,-8.28098049204476));
#21951=CARTESIAN_POINT('Ctrl Pts',(13.0134346502651,41.5079993600196,-8.81289306231732));
#21952=CARTESIAN_POINT('Ctrl Pts',(12.9025055846018,41.5424523787333,-9.35));
#21953=CARTESIAN_POINT('Origin',(-1.73472347597681E-15,-1.73472347597681E-15,
11.35));
#21954=CARTESIAN_POINT('Ctrl Pts',(10.0747117317978,42.317256332626,-9.34999999999999));
#21955=CARTESIAN_POINT('Ctrl Pts',(10.0166489392394,42.3310796744035,-8.81583928863872));
#21956=CARTESIAN_POINT('Ctrl Pts',(9.95314299752702,42.3460748083777,-8.29847152304224));
#21957=CARTESIAN_POINT('Ctrl Pts',(9.81446405776504,42.3784299795687,-7.21668089169946));
#21958=CARTESIAN_POINT('Ctrl Pts',(9.74394887671559,42.3946945890243,-6.68828455620137));
#21959=CARTESIAN_POINT('Ctrl Pts',(9.67733107622405,42.4098958173815,-6.16441400296897));
#21960=CARTESIAN_POINT('Ctrl Pts',(7.65858862696457,42.8205093412366,-6.16441400296897));
#21961=CARTESIAN_POINT('Ctrl Pts',(7.51060507268604,42.8469766855819,-6.69963387812706));
#21962=CARTESIAN_POINT('Ctrl Pts',(7.37048784895403,42.8712577590977,-7.21760449588847));
#21963=CARTESIAN_POINT('Ctrl Pts',(7.10033191648018,42.9168263524505,-8.28098049191645));
#21964=CARTESIAN_POINT('Ctrl Pts',(6.97377243337731,42.9375126237604,-8.81289306231198));
#21965=CARTESIAN_POINT('Ctrl Pts',(6.85906928985752,42.9558281083829,-9.35));
#21966=CARTESIAN_POINT('Origin',(-1.73472347597681E-15,-1.73472347597681E-15,
11.35));
#21967=CARTESIAN_POINT('Ctrl Pts',(3.94979220174152,43.320308650367,-9.34999999999999));
#21968=CARTESIAN_POINT('Ctrl Pts',(3.89035313805397,43.3257280935231,-8.81583928864517));
#21969=CARTESIAN_POINT('Ctrl Pts',(3.82535956525061,43.3315327608255,-8.29847152340904));
#21970=CARTESIAN_POINT('Ctrl Pts',(3.68348800204737,43.3438224935185,-7.21668429186925));
#21971=CARTESIAN_POINT('Ctrl Pts',(3.61137500115279,43.3498862691927,-6.68828131370428));
#21972=CARTESIAN_POINT('Ctrl Pts',(3.54327233497912,43.3554520350114,-6.16441400296898));
#21973=CARTESIAN_POINT('Ctrl Pts',(1.48664137583835,43.4745891000668,-6.16441400296897));
#21974=CARTESIAN_POINT('Ctrl Pts',(1.33639738494147,43.4797267894151,-6.69963387811528));
#21975=CARTESIAN_POINT('Ctrl Pts',(1.19425079545862,43.4838199565783,-7.21760449589258));
#21976=CARTESIAN_POINT('Ctrl Pts',(0.920359573842253,43.4904775295169,-8.2809804919506));
#21977=CARTESIAN_POINT('Ctrl Pts',(0.792144320446845,43.492941952042,-8.81289306231523));
#21978=CARTESIAN_POINT('Ctrl Pts',(0.676002124309571,43.4947470521204,-9.34999999999999));
#21979=CARTESIAN_POINT('Origin',(-1.73472347597681E-15,-1.73472347597681E-15,
11.35));
#21980=CARTESIAN_POINT('Ctrl Pts',(-2.25553370726646,43.4414844094374,-9.34999999999999));
#21981=CARTESIAN_POINT('Ctrl Pts',(-2.31513903416694,43.4383896297404,-8.81583928864895));
#21982=CARTESIAN_POINT('Ctrl Pts',(-2.38029715641292,43.4348856640963,-8.29847152332613));
#21983=CARTESIAN_POINT('Ctrl Pts',(-2.52247368297692,43.4268598764585,-7.21668429184511));
#21984=CARTESIAN_POINT('Ctrl Pts',(-2.59471564275521,43.4225991815798,-6.68828131367596));
#21985=CARTESIAN_POINT('Ctrl Pts',(-2.66291721304303,43.4184162760053,-6.16441400296898));
#21986=CARTESIAN_POINT('Ctrl Pts',(-4.71556960658337,43.2436515951818,-6.16441400296897));
#21987=CARTESIAN_POINT('Ctrl Pts',(-4.8650154997179,43.2273550409941,-6.69963387812718));
#21988=CARTESIAN_POINT('Ctrl Pts',(-5.00629776029438,43.2111769767249,-7.21760449588948));
#21989=CARTESIAN_POINT('Ctrl Pts',(-5.27834863559037,43.1787880002639,-8.28098049187636));
#21990=CARTESIAN_POINT('Ctrl Pts',(-5.40560956649133,43.1629804054675,-8.81289306230479));
#21991=CARTESIAN_POINT('Ctrl Pts',(-5.52082649506595,43.1482383743691,-9.34999999999999));
#21992=CARTESIAN_POINT('Origin',(-1.73472347597681E-15,-1.73472347597681E-15,
11.35));
#21993=CARTESIAN_POINT('Ctrl Pts',(-8.41494345442186,42.678316820827,-9.34999999999999));
#21994=CARTESIAN_POINT('Ctrl Pts',(-8.47350165196332,42.6667708190676,-8.81583928865055));
#21995=CARTESIAN_POINT('Ctrl Pts',(-8.53749789214447,42.6540295511172,-8.29847152350979));
#21996=CARTESIAN_POINT('Ctrl Pts',(-8.67708507802188,42.6258516250367,-7.21668429187095));
#21997=CARTESIAN_POINT('Ctrl Pts',(-8.74798535871346,42.6113531950656,-6.68828131370458));
#21998=CARTESIAN_POINT('Ctrl Pts',(-8.81489744582792,42.5975067699923,-6.16441400296897));
#21999=CARTESIAN_POINT('Ctrl Pts',(-10.8217851903811,42.1323980482153,-6.16441400296898));
#22000=CARTESIAN_POINT('Ctrl Pts',(-10.9673906983384,42.0949990013381,-6.69963387812129));
#22001=CARTESIAN_POINT('Ctrl Pts',(-11.1049325306246,42.0588790443689,-7.2176044958879));
#22002=CARTESIAN_POINT('Ctrl Pts',(-11.36960488837,41.9881028646561,-8.28098049203455));
#22003=CARTESIAN_POINT('Ctrl Pts',(-11.4933208311451,41.954345049595,-8.81289306232201));
#22004=CARTESIAN_POINT('Ctrl Pts',(-11.6052670077299,41.9233559925646,-9.34999999999999));
#22005=CARTESIAN_POINT('Origin',(-1.73472347597681E-15,-1.73472347597681E-15,
11.35));
#22006=CARTESIAN_POINT('Ctrl Pts',(-14.4030492195196,41.0463417758526,-9.34999999999999));
#22007=CARTESIAN_POINT('Ctrl Pts',(-14.4593682116834,41.026579595326,-8.81583928863168));
#22008=CARTESIAN_POINT('Ctrl Pts',(-14.5208997909904,41.0048604005178,-8.29847152306799));
#22009=CARTESIAN_POINT('Ctrl Pts',(-14.6550564651991,40.9571038072298,-7.21668089171361));
#22010=CARTESIAN_POINT('Ctrl Pts',(-14.7231709221274,40.9326630822685,-6.68828455621876));
#22011=CARTESIAN_POINT('Ctrl Pts',(-14.7874317866676,40.9094348672119,-6.16441400296897));
#22012=CARTESIAN_POINT('Ctrl Pts',(-16.7077004351661,40.1634503767885,-6.16441400296897));
#22013=CARTESIAN_POINT('Ctrl Pts',(-16.8465014496801,40.1057101739713,-6.69963387809185));
#22014=CARTESIAN_POINT('Ctrl Pts',(-16.9775028986086,40.0503836224612,-7.21760449589783));
#22015=CARTESIAN_POINT('Ctrl Pts',(-17.2294087728188,39.9426610384149,-8.2809804920777));
#22016=CARTESIAN_POINT('Ctrl Pts',(-17.3470612276791,39.8916402148528,-8.81289306232322));
#22017=CARTESIAN_POINT('Ctrl Pts',(-17.4534577509583,39.8450349797251,-9.34999999999999));
#22018=CARTESIAN_POINT('Origin',(-1.73472347597681E-15,-1.73472347597681E-15,
11.35));
#22019=CARTESIAN_POINT('Ctrl Pts',(-20.0979504374858,38.5787815801947,-9.34999999999999));
#22020=CARTESIAN_POINT('Ctrl Pts',(-20.1508837319902,38.5512055219091,-8.81583928863358));
#22021=CARTESIAN_POINT('Ctrl Pts',(-20.2086980448599,38.5209505404217,-8.29847152294191));
#22022=CARTESIAN_POINT('Ctrl Pts',(-20.3346927257031,38.4545875550058,-7.21668089166178));
#22023=CARTESIAN_POINT('Ctrl Pts',(-20.3986355978538,38.4207019034617,-6.68828455615817));
#22024=CARTESIAN_POINT('Ctrl Pts',(-20.4589366597763,38.3885648435998,-6.16441400296897));
#22025=CARTESIAN_POINT('Ctrl Pts',(-22.2534950801163,37.3768906775195,-6.16441400296897));
#22026=CARTESIAN_POINT('Ctrl Pts',(-22.3826660128241,37.299984742772,-6.6996338781274));
#22027=CARTESIAN_POINT('Ctrl Pts',(-22.5044602666512,37.2265778857698,-7.21760449588769));
#22028=CARTESIAN_POINT('Ctrl Pts',(-22.7384715801542,37.0841018185571,-8.28098049207543));
#22029=CARTESIAN_POINT('Ctrl Pts',(-22.8476674107164,37.0168554326535,-8.81290280339141));
#22030=CARTESIAN_POINT('Ctrl Pts',(-22.9463482217481,36.9555828432766,-9.35000977404799));
#22031=CARTESIAN_POINT('Origin',(-1.73472347597681E-15,-1.73472347597681E-15,
11.35));
#22032=CARTESIAN_POINT('Ctrl Pts',(-25.3837153422505,35.3258686435819,-9.35));
#22033=CARTESIAN_POINT('Ctrl Pts',(-25.4321853698649,35.2910400765618,-8.81583928862139));
#22034=CARTESIAN_POINT('Ctrl Pts',(-25.4851054835929,35.2528652125764,-8.29847152294655));
#22035=CARTESIAN_POINT('Ctrl Pts',(-25.6003732827113,35.1692467940417,-7.21668089172052));
#22036=CARTESIAN_POINT('Ctrl Pts',(-25.6588428775992,35.1266060300646,-6.68828455622536));
#22037=CARTESIAN_POINT('Ctrl Pts',(-25.7139565811841,35.0862143432572,-6.16441400296897));
#22038=CARTESIAN_POINT('Ctrl Pts',(-27.3462727390392,33.829445270091,-6.16441400296897));
#22039=CARTESIAN_POINT('Ctrl Pts',(-27.463184042233,33.7349391864739,-6.69963387815876));
#22040=CARTESIAN_POINT('Ctrl Pts',(-27.5732917211642,33.6449463759143,-7.21760449588191));
#22041=CARTESIAN_POINT('Ctrl Pts',(-27.7846446783725,33.4706172274601,-8.28098049170841));
#22042=CARTESIAN_POINT('Ctrl Pts',(-27.8831571551494,33.3885165787484,-8.81289306228552));
#22043=CARTESIAN_POINT('Ctrl Pts',(-27.9721136596209,33.313823818548,-9.34999999999999));
#22044=CARTESIAN_POINT('Origin',(-1.73472347597681E-15,-1.73472347597681E-15,
11.35));
#22045=CARTESIAN_POINT('Ctrl Pts',(-30.1527410032581,31.353822892758,-9.35));
#22046=CARTESIAN_POINT('Ctrl Pts',(-30.1957610539777,31.3124508262088,-8.81583928867595));
#22047=CARTESIAN_POINT('Ctrl Pts',(-30.2427096675459,31.2671332099776,-8.29847152400003));
#22048=CARTESIAN_POINT('Ctrl Pts',(-30.3449037438555,31.1679618997941,-7.2166842919219));
#22049=CARTESIAN_POINT('Ctrl Pts',(-30.3967104124394,31.1174334586449,-6.68828131375689));
#22050=CARTESIAN_POINT('Ctrl Pts',(-30.4455144995497,31.0696096991531,-6.16441400296897));
#22051=CARTESIAN_POINT('Ctrl Pts',(-31.8823591451153,29.5933299130376,-6.16441400296897));
#22052=CARTESIAN_POINT('Ctrl Pts',(-31.9846308417932,29.4831475518959,-6.69963387808623));
#22053=CARTESIAN_POINT('Ctrl Pts',(-32.080810471055,29.3784007818469,-7.21760449590099));
#22054=CARTESIAN_POINT('Ctrl Pts',(-32.2652025353664,29.175767390805,-8.28098049190116));
#22055=CARTESIAN_POINT('Ctrl Pts',(-32.351028156591,29.0804826211596,-8.81289306230433));
#22056=CARTESIAN_POINT('Ctrl Pts',(-32.4284493240122,28.9938902950255,-9.34999999999999));
#22057=CARTESIAN_POINT('Origin',(-1.73472347597681E-15,-1.73472347597681E-15,
11.35));
#22058=CARTESIAN_POINT('Ctrl Pts',(-34.3079438107289,26.7435037248276,-9.34999999999999));
#22059=CARTESIAN_POINT('Ctrl Pts',(-34.3446381204104,26.6964303746908,-8.81583928866682));
#22060=CARTESIAN_POINT('Ctrl Pts',(-34.3846594956096,26.6448925420414,-8.29847152347883));
#22061=CARTESIAN_POINT('Ctrl Pts',(-34.4717001081448,26.5321865651608,-7.21668089166674));
#22062=CARTESIAN_POINT('Ctrl Pts',(-34.5157879821584,26.4748002632575,-6.68828455615516));
#22063=CARTESIAN_POINT('Ctrl Pts',(-34.5572895403017,26.4205173989413,-6.16441400296897));
#22064=CARTESIAN_POINT('Ctrl Pts',(-35.7694126601179,24.7547796990843,-6.16441400296897));
#22065=CARTESIAN_POINT('Ctrl Pts',(-35.8549627934916,24.631164055521,-6.6996338781248));
#22066=CARTESIAN_POINT('Ctrl Pts',(-35.935256433163,24.5137956681822,-7.2176044958884));
#22067=CARTESIAN_POINT('Ctrl Pts',(-36.0889339138622,24.2869830660678,-8.2809804919214));
#22068=CARTESIAN_POINT('Ctrl Pts',(-36.1603255174268,24.1804538985902,-8.81289306230888));
#22069=CARTESIAN_POINT('Ctrl Pts',(-36.224635276104,24.0837247765632,-9.34999999999999));
#22070=CARTESIAN_POINT('Origin',(-1.73472347597681E-15,-1.73472347597681E-15,
11.35));
#22071=CARTESIAN_POINT('Ctrl Pts',(-37.7647358181634,21.5887639429479,-9.34999999999999));
#22072=CARTESIAN_POINT('Ctrl Pts',(-37.7943573964715,21.5369475868897,-8.81583928865539));
#22073=CARTESIAN_POINT('Ctrl Pts',(-37.8266368134634,21.4802386995183,-8.29847152342751));
#22074=CARTESIAN_POINT('Ctrl Pts',(-37.8967515248098,21.356293125861,-7.21668429186077));
#22075=CARTESIAN_POINT('Ctrl Pts',(-37.9322241523793,21.2932158164178,-6.68828131369573));
#22076=CARTESIAN_POINT('Ctrl Pts',(-37.9655778209998,21.2335795549787,-6.16441400296897));
#22077=CARTESIAN_POINT('Ctrl Pts',(-38.92830408384,19.4122935573335,-6.16441400296897));
#22078=CARTESIAN_POINT('Ctrl Pts',(-38.995391099886,19.2777610893897,-6.6996338781252));
#22079=CARTESIAN_POINT('Ctrl Pts',(-39.0581642030157,19.150160366661,-7.21760449589139));
#22080=CARTESIAN_POINT('Ctrl Pts',(-39.1779986697573,18.9037858039884,-8.28098049192254));
#22081=CARTESIAN_POINT('Ctrl Pts',(-39.2335029284966,18.7881808653144,-8.81289306231383));
#22082=CARTESIAN_POINT('Ctrl Pts',(-39.2833921172032,18.6832840733651,-9.34999999999999));
#22083=CARTESIAN_POINT('Origin',(-1.73472347597681E-15,-1.73472347597681E-15,
11.35));
#22084=CARTESIAN_POINT('Ctrl Pts',(-40.4527467088508,15.9945391840328,-9.34999999999999));
#22085=CARTESIAN_POINT('Ctrl Pts',(-40.4746925458678,15.9390346536462,-8.81583928863956));
#22086=CARTESIAN_POINT('Ctrl Pts',(-40.4985728888043,15.8783091409682,-8.29847152336921));
#22087=CARTESIAN_POINT('Ctrl Pts',(-40.5503348019053,15.7456463737683,-7.21668089171989));
#22088=CARTESIAN_POINT('Ctrl Pts',(-40.5764692176789,15.6781636308416,-6.68828455621838));
#22089=CARTESIAN_POINT('Ctrl Pts',(-40.6009964209562,15.6143872638508,-6.16441400296897));
#22090=CARTESIAN_POINT('Ctrl Pts',(-41.2947274963707,13.6746290991927,-6.16441400296901));
#22091=CARTESIAN_POINT('Ctrl Pts',(-41.3419856969067,13.5319184999549,-6.69963387811762));
#22092=CARTESIAN_POINT('Ctrl Pts',(-41.3859603841406,13.3966830245743,-7.21760449589209));
#22093=CARTESIAN_POINT('Ctrl Pts',(-41.4695123527587,13.1357619769457,-8.28098049195159));
#22094=CARTESIAN_POINT('Ctrl Pts',(-41.5079993600206,13.0134346502621,-8.81289306231735));
#22095=CARTESIAN_POINT('Ctrl Pts',(-41.5424523787372,12.9025055845893,-9.34999999999999));
#22096=CARTESIAN_POINT('Origin',(-1.73472347597681E-15,-1.73472347597681E-15,
11.35));
#22097=CARTESIAN_POINT('Ctrl Pts',(-42.3172560754436,10.0747128120527,-9.35000993815263));
#22098=CARTESIAN_POINT('Ctrl Pts',(-42.3310794172186,10.0166500195044,-8.81584922679741));
#22099=CARTESIAN_POINT('Ctrl Pts',(-42.3460748083683,9.95314299756727,-8.29847152331858));
#22100=CARTESIAN_POINT('Ctrl Pts',(-42.3784298778735,9.8144644936454,-7.21668429184823));
#22101=CARTESIAN_POINT('Ctrl Pts',(-42.3946946831143,9.74394846437601,-6.68828131367989));
#22102=CARTESIAN_POINT('Ctrl Pts',(-42.4098958173841,9.6773310762126,-6.16441400296897));
#22103=CARTESIAN_POINT('Ctrl Pts',(-42.8205093412364,7.65858862696564,-6.16441400296902));
#22104=CARTESIAN_POINT('Ctrl Pts',(-42.8469766855814,7.51060507268903,-6.69963387812033));
#22105=CARTESIAN_POINT('Ctrl Pts',(-42.8712577590977,7.37048784895363,-7.21760449589055));
#22106=CARTESIAN_POINT('Ctrl Pts',(-42.9168263524516,7.10033191647366,-8.28098049193938));
#22107=CARTESIAN_POINT('Ctrl Pts',(-42.9375126237604,6.97377243337723,-8.81289306231365));
#22108=CARTESIAN_POINT('Ctrl Pts',(-42.9558281083827,6.85906928985893,-9.34999999999999));
#22109=CARTESIAN_POINT('Origin',(-1.73472347597681E-15,-1.73472347597681E-15,
11.35));
#22110=CARTESIAN_POINT('Ctrl Pts',(-43.3203086503669,3.94979220174327,-9.34999999999999));
#22111=CARTESIAN_POINT('Ctrl Pts',(-43.325728093523,3.89035313805446,-8.81583928864667));
#22112=CARTESIAN_POINT('Ctrl Pts',(-43.3315327608263,3.82535956524115,-8.29847152334301));
#22113=CARTESIAN_POINT('Ctrl Pts',(-43.3438225321464,3.68348755613132,-7.21668089171067));
#22114=CARTESIAN_POINT('Ctrl Pts',(-43.3498862347431,3.61137542267791,-6.68828455620843));
#22115=CARTESIAN_POINT('Ctrl Pts',(-43.3554520350114,3.54327233497869,-6.16441400296897));
#22116=CARTESIAN_POINT('Ctrl Pts',(-43.4745891000669,1.48664137583783,-6.16441400296901));
#22117=CARTESIAN_POINT('Ctrl Pts',(-43.4797267894151,1.3363973849409,-6.69963387811629));
#22118=CARTESIAN_POINT('Ctrl Pts',(-43.4838199565783,1.19425079545889,-7.21760449589232));
#22119=CARTESIAN_POINT('Ctrl Pts',(-43.4904775295169,0.920359573845538,
-8.28098049193959));
#22120=CARTESIAN_POINT('Ctrl Pts',(-43.492941952042,0.792144320446992,-8.81289306231399));
#22121=CARTESIAN_POINT('Ctrl Pts',(-43.4947470521204,0.676002124309095,
-9.34999999999999));
#22122=CARTESIAN_POINT('Origin',(-1.73472347597681E-15,-1.73472347597681E-15,
11.35));
#22123=CARTESIAN_POINT('Ctrl Pts',(-43.4414844094373,-2.25553370726721,
-9.34999999999999));
#22124=CARTESIAN_POINT('Ctrl Pts',(-43.4383896297404,-2.31513903416679,
-8.81583928865233));
#22125=CARTESIAN_POINT('Ctrl Pts',(-43.4348856640966,-2.38029715640739,
-8.29847152336314));
#22126=CARTESIAN_POINT('Ctrl Pts',(-43.4268598764585,-2.52247368297661,
-7.21668429184337));
#22127=CARTESIAN_POINT('Ctrl Pts',(-43.4225991815797,-2.59471564275568,
-6.68828131367366));
#22128=CARTESIAN_POINT('Ctrl Pts',(-43.4184162760052,-2.66291721304384,
-6.16441400296897));
#22129=CARTESIAN_POINT('Ctrl Pts',(-43.2436515951816,-4.71556960658529,
-6.16441400296901));
#22130=CARTESIAN_POINT('Ctrl Pts',(-43.2273550409947,-4.86501549971271,
-6.699633878108));
#22131=CARTESIAN_POINT('Ctrl Pts',(-43.2111769767248,-5.0062977602958,-7.21760449589389));
#22132=CARTESIAN_POINT('Ctrl Pts',(-43.1787880002633,-5.27834863559578,
-8.2809804918952));
#22133=CARTESIAN_POINT('Ctrl Pts',(-43.1629804054676,-5.40560956649091,
-8.81289306230376));
#22134=CARTESIAN_POINT('Ctrl Pts',(-43.1482383743694,-5.5208264950638,-9.34999999999999));
#22135=CARTESIAN_POINT('Origin',(-1.73472347597681E-15,-1.73472347597681E-15,
11.35));
#22136=CARTESIAN_POINT('Ctrl Pts',(-42.6783168208273,-8.41494345442028,
-9.34999999999999));
#22137=CARTESIAN_POINT('Ctrl Pts',(-42.6667708190676,-8.47350165196288,
-8.8158392886554));
#22138=CARTESIAN_POINT('Ctrl Pts',(-42.6540295511159,-8.53749789215064,
-8.29847152346515));
#22139=CARTESIAN_POINT('Ctrl Pts',(-42.6258515364705,-8.67708551675907,
-7.21668089169991));
#22140=CARTESIAN_POINT('Ctrl Pts',(-42.6113532807684,-8.74798494455966,
-6.68828455619364));
#22141=CARTESIAN_POINT('Ctrl Pts',(-42.5975067699919,-8.81489744582999,
-6.16441400296896));
#22142=CARTESIAN_POINT('Ctrl Pts',(-42.1323980482118,-10.8217851903945,
-6.16441400296901));
#22143=CARTESIAN_POINT('Ctrl Pts',(-42.0949990013363,-10.9673906983452,
-6.69963387812546));
#22144=CARTESIAN_POINT('Ctrl Pts',(-42.0588790443698,-11.104932530621,-7.21760449589023));
#22145=CARTESIAN_POINT('Ctrl Pts',(-41.9881028646677,-11.3696048883265,
-8.28098049188592));
#22146=CARTESIAN_POINT('Ctrl Pts',(-41.9543450495943,-11.4933208311478,
-8.81289306230854));
#22147=CARTESIAN_POINT('Ctrl Pts',(-41.9233559925594,-11.6052670077487,
-9.34999999999999));
#22148=CARTESIAN_POINT('Origin',(-1.73472347597681E-15,-1.73472347597681E-15,
11.35));
#22149=CARTESIAN_POINT('Ctrl Pts',(-41.0463417758467,-14.4030492195362,
-9.34999999999999));
#22150=CARTESIAN_POINT('Ctrl Pts',(-41.0265795953249,-14.4593682116866,
-8.81583928863918));
#22151=CARTESIAN_POINT('Ctrl Pts',(-41.0048604005375,-14.5208997909351,
-8.29847152346152));
#22152=CARTESIAN_POINT('Ctrl Pts',(-40.9571039573334,-14.6550560435318,
-7.21668429186506));
#22153=CARTESIAN_POINT('Ctrl Pts',(-40.9326629384938,-14.7231713198805,
-6.68828131370069));
#22154=CARTESIAN_POINT('Ctrl Pts',(-40.9094348672063,-14.7874317866831,
-6.16441400296897));
#22155=CARTESIAN_POINT('Ctrl Pts',(-40.1634514153995,-16.7076979384609,
-6.16440437552835));
#22156=CARTESIAN_POINT('Ctrl Pts',(-40.1057112125809,-16.8464989529779,
-6.69962425069541));
#22157=CARTESIAN_POINT('Ctrl Pts',(-40.0503836224627,-16.977502898605,-7.21760449588796));
#22158=CARTESIAN_POINT('Ctrl Pts',(-39.9426610384488,-17.2294087727396,
-8.28098049178294));
#22159=CARTESIAN_POINT('Ctrl Pts',(-39.8916402148513,-17.3470612276828,
-8.81289306230247));
#22160=CARTESIAN_POINT('Ctrl Pts',(-39.845034979713,-17.4534577509859,-9.34999999999999));
#22161=CARTESIAN_POINT('Origin',(-1.73472347597681E-15,-1.73472347597681E-15,
11.35));
#22162=CARTESIAN_POINT('Ctrl Pts',(-38.5787815801808,-20.0979504375124,
-9.34999999999999));
#22163=CARTESIAN_POINT('Ctrl Pts',(-38.5512055219064,-20.1508837319952,
-8.81583928865245));
#22164=CARTESIAN_POINT('Ctrl Pts',(-38.5209505404797,-20.2086980447498,
-8.29847152379691));
#22165=CARTESIAN_POINT('Ctrl Pts',(-38.4545877635967,-20.334692329679,-7.21668429188963));
#22166=CARTESIAN_POINT('Ctrl Pts',(-38.4207017045473,-20.398635971091,-6.68828131372094));
#22167=CARTESIAN_POINT('Ctrl Pts',(-38.3885648435901,-20.4589366597944,
-6.16441400296898));
#22168=CARTESIAN_POINT('Ctrl Pts',(-37.3768920608804,-22.253492756628,-6.16440437552834));
#22169=CARTESIAN_POINT('Ctrl Pts',(-37.2999861261424,-22.3826636893199,
-6.69962425065386));
#22170=CARTESIAN_POINT('Ctrl Pts',(-37.2265778857679,-22.5044602666544,
-7.21760449589713));
#22171=CARTESIAN_POINT('Ctrl Pts',(-37.0841018185697,-22.7384715801335,
-8.28098049199277));
#22172=CARTESIAN_POINT('Ctrl Pts',(-37.0168566233265,-22.847665482412,-8.8128930623192));
#22173=CARTESIAN_POINT('Ctrl Pts',(-36.955583958287,-22.946346426,-9.34999999999999));
#22174=CARTESIAN_POINT('Origin',(-1.73472347597681E-15,-1.73472347597681E-15,
11.35));
#22175=CARTESIAN_POINT('Ctrl Pts',(-35.3258692915697,-25.3837144404623,
-9.35000993815263));
#22176=CARTESIAN_POINT('Ctrl Pts',(-35.2910407245523,-25.4321844680731,
-8.81584922678877));
#22177=CARTESIAN_POINT('Ctrl Pts',(-35.252865212596,-25.4851054835659,-8.29847152317624));
#22178=CARTESIAN_POINT('Ctrl Pts',(-35.1692467940378,-25.6003732827167,
-7.21668089167782));
#22179=CARTESIAN_POINT('Ctrl Pts',(-35.1266060300552,-25.658842877612,-6.6882845561739));
#22180=CARTESIAN_POINT('Ctrl Pts',(-35.0862143432467,-25.7139565811984,
-6.16441400296897));
#22181=CARTESIAN_POINT('Ctrl Pts',(-33.8294452700949,-27.3462727390344,
-6.16441400296902));
#22182=CARTESIAN_POINT('Ctrl Pts',(-33.7349391864802,-27.4631840422253,
-6.69963387813819));
#22183=CARTESIAN_POINT('Ctrl Pts',(-33.6449463759126,-27.5732917211663,
-7.21760449588766));
#22184=CARTESIAN_POINT('Ctrl Pts',(-33.4706172274317,-27.7846446784069,
-8.28098049186743));
#22185=CARTESIAN_POINT('Ctrl Pts',(-33.3885165787479,-27.88315715515,-8.8128930623081));
#22186=CARTESIAN_POINT('Ctrl Pts',(-33.3138238185527,-27.9721136596152,
-9.34999999999999));
#22187=CARTESIAN_POINT('Origin',(-1.73472347597681E-15,-1.73472347597681E-15,
11.35));
#22188=CARTESIAN_POINT('Ctrl Pts',(-31.3538228927626,-30.1527410032535,
-9.34999999999999));
#22189=CARTESIAN_POINT('Ctrl Pts',(-31.3124508262098,-30.1957610539767,
-8.81583928865918));
#22190=CARTESIAN_POINT('Ctrl Pts',(-31.2671332099354,-30.2427096675894,
-8.29847152356755));
#22191=CARTESIAN_POINT('Ctrl Pts',(-31.1679615880869,-30.3449040650636,
-7.21668089173702));
#22192=CARTESIAN_POINT('Ctrl Pts',(-31.1174337546538,-30.3967101103627,
-6.68828455623348));
#22193=CARTESIAN_POINT('Ctrl Pts',(-31.069609699158,-30.4455144995448,-6.16441400296898));
#22194=CARTESIAN_POINT('Ctrl Pts',(-29.5933299130507,-31.8823591451032,
-6.16441400296901));
#22195=CARTESIAN_POINT('Ctrl Pts',(-29.4831475518907,-31.9846308417981,
-6.69963387813632));
#22196=CARTESIAN_POINT('Ctrl Pts',(-29.3784007818493,-32.0808104710528,
-7.21760449588548));
#22197=CARTESIAN_POINT('Ctrl Pts',(-29.1757673907854,-32.2652025353842,
-8.280980491991));
#22198=CARTESIAN_POINT('Ctrl Pts',(-29.0804826211579,-32.3510281565926,
-8.81289306232937));
#22199=CARTESIAN_POINT('Ctrl Pts',(-28.9938902950281,-32.4284493240099,
-9.34999999999999));
#22200=CARTESIAN_POINT('Origin',(-1.73472347597681E-15,-1.73472347597681E-15,
11.35));
#22201=CARTESIAN_POINT('Ctrl Pts',(-26.7435037248304,-34.3079438107268,
-9.34999999999999));
#22202=CARTESIAN_POINT('Ctrl Pts',(-26.6964303746899,-34.344638120411,-8.8158392886314));
#22203=CARTESIAN_POINT('Ctrl Pts',(-26.6448925420125,-34.3846594956319,
-8.29847152322916));
#22204=CARTESIAN_POINT('Ctrl Pts',(-26.5321865651666,-34.4717001081404,
-7.2166808917316));
#22205=CARTESIAN_POINT('Ctrl Pts',(-26.4748002632703,-34.5157879821486,
-6.68828455623219));
#22206=CARTESIAN_POINT('Ctrl Pts',(-26.4205173989538,-34.5572895402921,
-6.16441400296898));
#22207=CARTESIAN_POINT('Ctrl Pts',(-24.7547796990836,-35.7694126601185,
-6.16441400296901));
#22208=CARTESIAN_POINT('Ctrl Pts',(-24.6311640555348,-35.854962793482,-6.69963387807314));
#22209=CARTESIAN_POINT('Ctrl Pts',(-24.5137956681789,-35.9352564331652,
-7.21760449590187));
#22210=CARTESIAN_POINT('Ctrl Pts',(-24.2869830660437,-36.0889339138785,
-8.28098049202429));
#22211=CARTESIAN_POINT('Ctrl Pts',(-24.1804538985908,-36.1603255174264,
-8.81289306231515));
#22212=CARTESIAN_POINT('Ctrl Pts',(-24.0837247765702,-36.2246352760993,
-9.34999999999999));
#22213=CARTESIAN_POINT('Origin',(-1.73472347597681E-15,-1.73472347597681E-15,
11.35));
#22214=CARTESIAN_POINT('Ctrl Pts',(-21.5887639429553,-37.7647358181592,
-9.34999999999999));
#22215=CARTESIAN_POINT('Ctrl Pts',(-21.5369475868915,-37.7943573964706,
-8.81583928865988));
#22216=CARTESIAN_POINT('Ctrl Pts',(-21.4802386994815,-37.8266368134842,
-8.29847152312796));
#22217=CARTESIAN_POINT('Ctrl Pts',(-21.3562931258516,-37.8967515248151,
-7.21668429177588));
#22218=CARTESIAN_POINT('Ctrl Pts',(-21.2932158164099,-37.9322241523837,
-6.68828131359938));
#22219=CARTESIAN_POINT('Ctrl Pts',(-21.2335795549793,-37.9655778209995,
-6.16441400296897));
#22220=CARTESIAN_POINT('Ctrl Pts',(-19.4122935573269,-38.9283040838433,
-6.16441400296902));
#22221=CARTESIAN_POINT('Ctrl Pts',(-19.2777610893895,-38.9953910998861,
-6.69963387811522));
#22222=CARTESIAN_POINT('Ctrl Pts',(-19.1501603666615,-39.0581642030155,
-7.21760449589381));
#22223=CARTESIAN_POINT('Ctrl Pts',(-18.9037858039981,-39.1779986697526,
-8.28098049188953));
#22224=CARTESIAN_POINT('Ctrl Pts',(-18.7881808653121,-39.2335029284977,
-8.81289306231679));
#22225=CARTESIAN_POINT('Ctrl Pts',(-18.6832840733583,-39.2833921172065,
-9.34999999999999));
#22226=CARTESIAN_POINT('Origin',(-1.73472347597681E-15,-1.73472347597681E-15,
11.35));
#22227=CARTESIAN_POINT('Ctrl Pts',(-15.9945391840253,-40.4527467088538,
-9.34999999999999));
#22228=CARTESIAN_POINT('Ctrl Pts',(-15.9390346536446,-40.4746925458684,
-8.81583928864358));
#22229=CARTESIAN_POINT('Ctrl Pts',(-15.8783091409867,-40.498572888797,-8.29847152349527));
#22230=CARTESIAN_POINT('Ctrl Pts',(-15.7456463737691,-40.550334801905,-7.21668089170353));
#22231=CARTESIAN_POINT('Ctrl Pts',(-15.6781636308371,-40.5764692176807,
-6.68828455619327));
#22232=CARTESIAN_POINT('Ctrl Pts',(-15.6143872638446,-40.6009964209586,
-6.16441400296898));
#22233=CARTESIAN_POINT('Ctrl Pts',(-13.6746290992012,-41.2947274963679,
-6.16441400296902));
#22234=CARTESIAN_POINT('Ctrl Pts',(-13.5319184999655,-41.3419856969032,
-6.69963387810014));
#22235=CARTESIAN_POINT('Ctrl Pts',(-13.3966830245737,-41.3859603841408,
-7.21760449589543));
#22236=CARTESIAN_POINT('Ctrl Pts',(-13.1357619769182,-41.4695123527675,
-8.28098049205013));
#22237=CARTESIAN_POINT('Ctrl Pts',(-13.0134346502636,-41.5079993600201,
-8.81289306232158));
#22238=CARTESIAN_POINT('Ctrl Pts',(-12.9025055845986,-41.5424523787343,
-9.34999999999999));
#22239=CARTESIAN_POINT('Origin',(-1.73472347597681E-15,-1.73472347597681E-15,
11.35));
#22240=CARTESIAN_POINT('Ctrl Pts',(-10.074711731795,-42.3172563326267,-9.35));
#22241=CARTESIAN_POINT('Ctrl Pts',(-10.0166489392386,-42.3310796744037,
-8.81583928863731));
#22242=CARTESIAN_POINT('Ctrl Pts',(-9.95314299752523,-42.3460748083781,
-8.29847152302227));
#22243=CARTESIAN_POINT('Ctrl Pts',(-9.81446405776189,-42.3784299795695,
-7.21668089167201));
#22244=CARTESIAN_POINT('Ctrl Pts',(-9.7439488767096,-42.3946945890256,-6.68828455616903));
#22245=CARTESIAN_POINT('Ctrl Pts',(-9.67733107621878,-42.4098958173827,
-6.16441400296897));
#22246=CARTESIAN_POINT('Ctrl Pts',(-7.65858862696401,-42.8205093412367,
-6.16441400296901));
#22247=CARTESIAN_POINT('Ctrl Pts',(-7.51060507269031,-42.8469766855811,
-6.69963387811412));
#22248=CARTESIAN_POINT('Ctrl Pts',(-7.3704878489533,-42.8712577590978,-7.21760449589294));
#22249=CARTESIAN_POINT('Ctrl Pts',(-7.10033191647729,-42.916826352451,-8.28098049192608));
#22250=CARTESIAN_POINT('Ctrl Pts',(-6.9737724333775,-42.9375126237603,-8.81289306230911));
#22251=CARTESIAN_POINT('Ctrl Pts',(-6.85906928985838,-42.9558281083827,
-9.34999999999999));
#22252=CARTESIAN_POINT('Origin',(-1.73472347597681E-15,-1.73472347597681E-15,
11.35));
#22253=CARTESIAN_POINT('Ctrl Pts',(-3.94979220174291,-43.3203086503669,
-9.34999999999999));
#22254=CARTESIAN_POINT('Ctrl Pts',(-3.8903531380541,-43.325728093523,-8.81583928864717));
#22255=CARTESIAN_POINT('Ctrl Pts',(-3.82535956524451,-43.331532760826,-8.29847152336844));
#22256=CARTESIAN_POINT('Ctrl Pts',(-3.683488002044,-43.3438224935188,-7.2166842918505));
#22257=CARTESIAN_POINT('Ctrl Pts',(-3.61137500114881,-43.349886269193,-6.68828131368176));
#22258=CARTESIAN_POINT('Ctrl Pts',(-3.5432723349768,-43.3554520350116,-6.16441400296897));
#22259=CARTESIAN_POINT('Ctrl Pts',(-1.48664137583836,-43.4745891000668,
-6.16441400296897));
#22260=CARTESIAN_POINT('Ctrl Pts',(-1.33639738494146,-43.4797267894151,
-6.69963387811538));
#22261=CARTESIAN_POINT('Ctrl Pts',(-1.19425079545864,-43.4838199565783,
-7.2176044958926));
#22262=CARTESIAN_POINT('Ctrl Pts',(-0.920359573842274,-43.4904775295169,
-8.28098049195057));
#22263=CARTESIAN_POINT('Ctrl Pts',(-0.792144320446858,-43.492941952042,
-8.81289306231522));
#22264=CARTESIAN_POINT('Ctrl Pts',(-0.676002124309579,-43.4947470521204,
-9.34999999999999));
#22265=CARTESIAN_POINT('Origin',(-1.73472347597681E-15,-1.73472347597681E-15,
11.35));
#22266=CARTESIAN_POINT('Ctrl Pts',(4.71518277776759,-43.2436937757663,6.16441400296896));
#22267=CARTESIAN_POINT('Ctrl Pts',(4.8650977532406,-43.2273474267669,6.70062138560741));
#22268=CARTESIAN_POINT('Ctrl Pts',(5.00655712290831,-43.2111479469791,7.21784327704619));
#22269=CARTESIAN_POINT('Ctrl Pts',(5.27969251824256,-43.178626142302,8.28373602794635));
#22270=CARTESIAN_POINT('Ctrl Pts',(5.40632229142204,-43.1628906187996,8.81321169230961));
#22271=CARTESIAN_POINT('Ctrl Pts',(5.52134683388059,-43.1481717937157,9.34999999998855));
#22272=CARTESIAN_POINT('Ctrl Pts',(2.25607198755898,-43.4414564579384,9.34999999999998));
#22273=CARTESIAN_POINT('Ctrl Pts',(2.31575404873037,-43.4383569525961,8.81613492203368));
#22274=CARTESIAN_POINT('Ctrl Pts',(2.38157881405563,-43.4348138690301,8.29345816615258));
#22275=CARTESIAN_POINT('Ctrl Pts',(2.52277267021435,-43.4268424365167,7.21621981188664));
#22276=CARTESIAN_POINT('Ctrl Pts',(2.59475150835134,-43.4225967225811,6.68773441334971));
#22277=CARTESIAN_POINT('Ctrl Pts',(2.66275246602647,-43.4184263798755,6.16441400296896));
#22278=CARTESIAN_POINT('Origin',(-1.73472347597681E-15,-1.73472347597681E-15,
11.35));
#22279=CARTESIAN_POINT('Ctrl Pts',(8.41547227788092,-42.6782125485618,9.34999999998854));
#22280=CARTESIAN_POINT('Ctrl Pts',(8.47410575612226,-42.6666509488314,8.81613492202544));
#22281=CARTESIAN_POINT('Ctrl Pts',(8.53875628688305,-42.6537760879159,8.29345816614668));
#22282=CARTESIAN_POINT('Ctrl Pts',(8.67737854004119,-42.6257918122874,7.21621981188599));
#22283=CARTESIAN_POINT('Ctrl Pts',(8.74802050929878,-42.6113456568892,6.68773441334886));
#22284=CARTESIAN_POINT('Ctrl Pts',(8.81473581362626,-42.5975402169653,6.16441400296897));
#22285=CARTESIAN_POINT('Ctrl Pts',(10.8214083018597,-42.1324948509395,6.16441400296896));
#22286=CARTESIAN_POINT('Ctrl Pts',(10.9674710310278,-42.0949797587143,6.70062138560767));
#22287=CARTESIAN_POINT('Ctrl Pts',(11.1051851219337,-42.0588133989565,7.2178432770462));
#22288=CARTESIAN_POINT('Ctrl Pts',(11.3709120573992,-41.9877513997447,8.28373602794641));
#22289=CARTESIAN_POINT('Ctrl Pts',(11.4940135235903,-41.9541547454922,8.81321169230964));
#22290=CARTESIAN_POINT('Ctrl Pts',(11.605772574847,-41.9232160376674,9.34999999998854));
#22291=CARTESIAN_POINT('Origin',(-1.73472347597681E-15,-1.73472347597681E-15,
11.35));
#22292=CARTESIAN_POINT('Ctrl Pts',(14.4035578208426,-41.0461633054985,9.34999999998854));
#22293=CARTESIAN_POINT('Ctrl Pts',(14.4599491076221,-41.0263749722096,8.8161349220257));
#22294=CARTESIAN_POINT('Ctrl Pts',(14.5221093054489,-41.0044304289847,8.29345816614813));
#22295=CARTESIAN_POINT('Ctrl Pts',(14.6553380062866,-40.9570029893927,7.21621981188605));
#22296=CARTESIAN_POINT('Ctrl Pts',(14.7232050398853,-40.9326504745967,6.68773441334895));
#22297=CARTESIAN_POINT('Ctrl Pts',(14.7872765596602,-40.9094909763997,6.16441400296897));
#22298=CARTESIAN_POINT('Ctrl Pts',(16.7073411592906,-40.1635998310296,6.16441400296896));
#22299=CARTESIAN_POINT('Ctrl Pts',(16.846578226198,-40.1056796946716,6.70062138560762));
#22300=CARTESIAN_POINT('Ctrl Pts',(16.9777435765859,-40.0502826977333,7.21784327704622));
#22301=CARTESIAN_POINT('Ctrl Pts',(17.2306526180698,-39.9421271213649,8.28373602794653));
#22302=CARTESIAN_POINT('Ctrl Pts',(17.3477197864163,-39.8913532673581,8.81321169230968));
#22303=CARTESIAN_POINT('Ctrl Pts',(17.4539382544739,-39.8448244996639,9.34999999998855));
#22304=CARTESIAN_POINT('Origin',(-1.73472347597681E-15,-1.73472347597681E-15,
11.35));
#22305=CARTESIAN_POINT('Ctrl Pts',(20.0984284630027,-38.5785325448956,9.34999999998854));
#22306=CARTESIAN_POINT('Ctrl Pts',(20.1514295943406,-38.5509203114491,8.81613492202573));
#22307=CARTESIAN_POINT('Ctrl Pts',(20.2098340568611,-38.5203528135321,8.2934581661483));
#22308=CARTESIAN_POINT('Ctrl Pts',(20.3349570532291,-38.4544476958773,7.21621981188512));
#22309=CARTESIAN_POINT('Ctrl Pts',(20.398667574077,-38.4206845686579,6.68773441334953));
#22310=CARTESIAN_POINT('Ctrl Pts',(20.4587909979238,-38.3886424727845,6.16441400296896));
#22311=CARTESIAN_POINT('Ctrl Pts',(22.2531607307116,-37.3770897408174,6.16441400296897));
#22312=CARTESIAN_POINT('Ctrl Pts',(22.3827376702025,-37.2999436472751,6.70062138560737));
#22313=CARTESIAN_POINT('Ctrl Pts',(22.5046841317882,-37.2264437362622,7.21784327704616));
#22314=CARTESIAN_POINT('Ctrl Pts',(22.7396267805353,-37.0833963183772,8.28373602794666));
#22315=CARTESIAN_POINT('Ctrl Pts',(22.8482765010835,-37.016478873864,8.81321169230972));
#22316=CARTESIAN_POINT('Ctrl Pts',(22.9467920842412,-36.9553072378327,9.34999999998855));
#22317=CARTESIAN_POINT('Origin',(-1.73472347597681E-15,-1.73472347597681E-15,
11.35));
#22318=CARTESIAN_POINT('Ctrl Pts',(25.3841530607376,-35.3255541129796,9.34999999998854));
#22319=CARTESIAN_POINT('Ctrl Pts',(25.4326850864425,-35.2906800848214,8.81613492202558));
#22320=CARTESIAN_POINT('Ctrl Pts',(25.4861448672244,-35.2521118983204,8.2934581661475));
#22321=CARTESIAN_POINT('Ctrl Pts',(25.6006150157412,-35.1690707407437,7.21621981188588));
#22322=CARTESIAN_POINT('Ctrl Pts',(25.6588720613602,-35.1265843210061,6.68773441334898));
#22323=CARTESIAN_POINT('Ctrl Pts',(25.7138234497508,-35.0863119121267,6.16441400296896));
#22324=CARTESIAN_POINT('Ctrl Pts',(27.3459701224716,-33.8296898901083,6.16441400296896));
#22325=CARTESIAN_POINT('Ctrl Pts',(27.4632491217272,-33.7348883113751,6.70062138560758));
#22326=CARTESIAN_POINT('Ctrl Pts',(27.5734942162173,-33.6447817325196,7.21784327704617));
#22327=CARTESIAN_POINT('Ctrl Pts',(27.7856877174178,-33.4697545060314,8.28373602794671));
#22328=CARTESIAN_POINT('Ctrl Pts',(27.8837081951772,-33.3880557172081,8.81321169230973));
#22329=CARTESIAN_POINT('Ctrl Pts',(27.9725154002573,-33.3134864909449,9.34999999998854));
#22330=CARTESIAN_POINT('Origin',(-1.73472347597681E-15,-1.73472347597681E-15,
11.35));
#22331=CARTESIAN_POINT('Ctrl Pts',(30.1531295040085,-31.3534492698092,9.34999999998854));
#22332=CARTESIAN_POINT('Ctrl Pts',(30.1962044519918,-31.3120233815841,8.81613492202547));
#22333=CARTESIAN_POINT('Ctrl Pts',(30.2436312640637,-31.2662396435548,8.29345816614697));
#22334=CARTESIAN_POINT('Ctrl Pts',(30.3451186039616,-31.1677526127026,7.21621640088951));
#22335=CARTESIAN_POINT('Ctrl Pts',(30.3967356067597,-31.11740840803,6.68773764820084));
#22336=CARTESIAN_POINT('Ctrl Pts',(30.4453966086845,-31.0697252215063,6.16441400296896));
#22337=CARTESIAN_POINT('Ctrl Pts',(31.8820944218039,-29.5936151100062,6.16441400296896));
#22338=CARTESIAN_POINT('Ctrl Pts',(31.9846880186039,-29.48308793284,6.70062138560735));
#22339=CARTESIAN_POINT('Ctrl Pts',(32.0809874737953,-29.3782089962415,7.21784327704616));
#22340=CARTESIAN_POINT('Ctrl Pts',(32.2661121796801,-29.1747650107446,8.28373602794627));
#22341=CARTESIAN_POINT('Ctrl Pts',(32.3515080003913,-29.0799480293518,8.81321169230959));
#22342=CARTESIAN_POINT('Ctrl Pts',(32.4287989687974,-28.9934992272635,9.34999999998855));
#22343=CARTESIAN_POINT('Origin',(-1.73472347597681E-15,-1.73472347597681E-15,
11.35));
#22344=CARTESIAN_POINT('Ctrl Pts',(37.7650033201655,-21.5882960010254,9.34999999998854));
#22345=CARTESIAN_POINT('Ctrl Pts',(37.7946624086853,-21.5364125371166,8.81613492202549));
#22346=CARTESIAN_POINT('Ctrl Pts',(37.8272693320525,-21.4791216851438,8.29345816614708));
#22347=CARTESIAN_POINT('Ctrl Pts',(37.8968987185776,-21.3560317832924,7.21621640088866));
#22348=CARTESIAN_POINT('Ctrl Pts',(37.9322412685768,-21.2931846824721,6.68773764820146));
#22349=CARTESIAN_POINT('Ctrl Pts',(37.9654972519551,-21.2337236115523,6.16441400296896));
#22350=CARTESIAN_POINT('Ctrl Pts',(38.928130432958,-19.412641782988,6.16441400296896));
#22351=CARTESIAN_POINT('Ctrl Pts',(38.995429164002,-19.2776877767616,6.70062138560751));
#22352=CARTESIAN_POINT('Ctrl Pts',(39.0582800036543,-19.1499264822817,7.2178432770462));
#22353=CARTESIAN_POINT('Ctrl Pts',(39.1785890639852,-18.9025677509498,8.28373602794626));
#22354=CARTESIAN_POINT('Ctrl Pts',(39.2338127233339,-18.7875327406115,8.81321169230958));
#22355=CARTESIAN_POINT('Ctrl Pts',(39.2836174223951,-18.6828103402806,9.34999999998855));
#22356=CARTESIAN_POINT('Origin',(-1.73472347597681E-15,-1.73472347597681E-15,
11.35));
#22357=CARTESIAN_POINT('Ctrl Pts',(34.3082751850227,-26.7430786153868,9.34999999998854));
#22358=CARTESIAN_POINT('Ctrl Pts',(34.3450161735614,-26.6959441787169,8.81613492202567));
#22359=CARTESIAN_POINT('Ctrl Pts',(34.385444543797,-26.6438769140362,8.29345816614794));
#22360=CARTESIAN_POINT('Ctrl Pts',(34.4718824493404,-26.5319495391969,7.21621981188585));
#22361=CARTESIAN_POINT('Ctrl Pts',(34.5158098676116,-26.4747712115684,6.68773441334903));
#22362=CARTESIAN_POINT('Ctrl Pts',(34.557189289939,-26.4206485230648,6.16441400296897));
#22363=CARTESIAN_POINT('Ctrl Pts',(35.7691912190764,-24.755099667203,6.16441400296895));
#22364=CARTESIAN_POINT('Ctrl Pts',(35.8550109036455,-24.631096906197,6.70062138560717));
#22365=CARTESIAN_POINT('Ctrl Pts',(35.9354043403351,-24.5135806445587,7.21784327704611));
#22366=CARTESIAN_POINT('Ctrl Pts',(36.0896916457482,-24.2858614329137,8.28373602794642));
#22367=CARTESIAN_POINT('Ctrl Pts',(36.1607243967626,-24.1798564592629,8.81321169230963));
#22368=CARTESIAN_POINT('Ctrl Pts',(36.2249257072666,-24.0832879296623,9.34999999998854));
#22369=CARTESIAN_POINT('Origin',(-1.73472347597681E-15,-1.73472347597681E-15,
11.35));
#22370=CARTESIAN_POINT('Ctrl Pts',(40.4529448929862,-15.9940379355879,9.34999999998854));
#22371=CARTESIAN_POINT('Ctrl Pts',(40.4749183079745,-15.9384616421459,8.81613492202553));
#22372=CARTESIAN_POINT('Ctrl Pts',(40.499040001544,-15.877113479414,8.29345816614729));
#22373=CARTESIAN_POINT('Ctrl Pts',(40.5504429790727,-15.7453675775639,7.21621981188599));
#22374=CARTESIAN_POINT('Ctrl Pts',(40.5764820318144,-15.6781295900963,6.68773441334888));
#22375=CARTESIAN_POINT('Ctrl Pts',(40.6009371733745,-15.6145413203111,6.16441400296896));
#22376=CARTESIAN_POINT('Ctrl Pts',(41.2946051706827,-13.6749984935074,6.16441400296896));
#22377=CARTESIAN_POINT('Ctrl Pts',(41.3420129401109,-13.5318405164523,6.70062138560745));
#22378=CARTESIAN_POINT('Ctrl Pts',(41.3860417208775,-13.3964350406532,7.2178432770462));
#22379=CARTESIAN_POINT('Ctrl Pts',(41.4699233906006,-13.1344723000805,8.28373602794641));
#22380=CARTESIAN_POINT('Ctrl Pts',(41.508213763831,-13.0127490341317,8.81321169230963));
#22381=CARTESIAN_POINT('Ctrl Pts',(41.5426079714016,-12.9020046091468,9.34999999998855));
#22382=CARTESIAN_POINT('Origin',(-1.73472347597681E-15,-1.73472347597681E-15,
11.35));
#22383=CARTESIAN_POINT('Ctrl Pts',(42.3173811644455,-10.0741873807785,9.34999999998854));
#22384=CARTESIAN_POINT('Ctrl Pts',(42.3312215905392,-10.016049630869,8.81613492202556));
#22385=CARTESIAN_POINT('Ctrl Pts',(42.3463670061913,-9.95189302905774,8.29345816614737));
#22386=CARTESIAN_POINT('Ctrl Pts',(42.3784973788108,-9.81417270409282,7.21621981188622));
#22387=CARTESIAN_POINT('Ctrl Pts',(42.3947024282284,-9.74391335880868,6.68773441334868));
#22388=CARTESIAN_POINT('Ctrl Pts',(42.4098590973783,-9.67749199640711,6.16441400296896));
#22389=CARTESIAN_POINT('Ctrl Pts',(42.8204408309399,-7.65897167013824,6.16441400296896));
#22390=CARTESIAN_POINT('Ctrl Pts',(42.8469925532796,-7.51052400583368,6.70062138560742));
#22391=CARTESIAN_POINT('Ctrl Pts',(42.8713029761526,-7.37023081372545,7.21784327704618));
#22392=CARTESIAN_POINT('Ctrl Pts',(42.917049666367,-7.09899686987205,8.2837360279463));
#22393=CARTESIAN_POINT('Ctrl Pts',(42.9376272719005,-6.97306328298636,8.8132116923096));
#22394=CARTESIAN_POINT('Ctrl Pts',(42.955910821099,-6.85855127047957,9.34999999998855));
#22395=CARTESIAN_POINT('Origin',(-1.73472347597681E-15,-1.73472347597681E-15,
11.35));
#22396=CARTESIAN_POINT('Ctrl Pts',(43.3203575886467,-3.94925542245386,9.34999999998855));
#22397=CARTESIAN_POINT('Ctrl Pts',(43.3257832746831,-3.88973973300951,8.81613492202556));
#22398=CARTESIAN_POINT('Ctrl Pts',(43.3316440954308,-3.82408073551946,8.29345816614743));
#22399=CARTESIAN_POINT('Ctrl Pts',(43.3438477814109,-3.68318957610333,7.21621981188594));
#22400=CARTESIAN_POINT('Ctrl Pts',(43.3498889394299,-3.61133915066155,6.6877344133489));
#22401=CARTESIAN_POINT('Ctrl Pts',(43.3554385900939,-3.54343684303868,6.16441400296896));
#22402=CARTESIAN_POINT('Ctrl Pts',(43.4745757998335,-1.48703027021543,6.16441400296896));
#22403=CARTESIAN_POINT('Ctrl Pts',(43.4797309585866,-1.33631488501896,6.70062138560747));
#22404=CARTESIAN_POINT('Ctrl Pts',(43.4838281334618,-1.19398994142081,7.21784327704619));
#22405=CARTESIAN_POINT('Ctrl Pts',(43.4905085734774,-0.919006335209355,
8.28373602794638));
#22406=CARTESIAN_POINT('Ctrl Pts',(43.4929545106062,-0.791426072053404,
8.81321169230962));
#22407=CARTESIAN_POINT('Ctrl Pts',(43.4947552010963,-0.675477606374008,
9.34999999998855));
#22408=CARTESIAN_POINT('Origin',(-1.73472347597681E-15,-1.73472347597681E-15,
11.35));
#22409=CARTESIAN_POINT('Ctrl Pts',(43.4414565156357,2.25607087657594,9.35000993791518));
#22410=CARTESIAN_POINT('Ctrl Pts',(43.4383570102934,2.31575293774707,8.81614485995222));
#22411=CARTESIAN_POINT('Ctrl Pts',(43.4348138690301,2.38157881405584,8.29345816614752));
#22412=CARTESIAN_POINT('Ctrl Pts',(43.4268424365168,2.52277267021401,7.21621981188581));
#22413=CARTESIAN_POINT('Ctrl Pts',(43.4225967225812,2.59475150835097,6.6877344133491));
#22414=CARTESIAN_POINT('Ctrl Pts',(43.4184263798756,2.66275246602603,6.16441400296896));
#22415=CARTESIAN_POINT('Ctrl Pts',(43.2436937757663,4.71518277776774,6.16441400296896));
#22416=CARTESIAN_POINT('Ctrl Pts',(43.2273474267669,4.86509775324073,6.70062138560733));
#22417=CARTESIAN_POINT('Ctrl Pts',(43.211147946979,5.00655712290845,7.21784327704615));
#22418=CARTESIAN_POINT('Ctrl Pts',(43.1786261423019,5.2796925182427,8.28373602794632));
#22419=CARTESIAN_POINT('Ctrl Pts',(43.1628906187996,5.40632229142219,8.8132116923096));
#22420=CARTESIAN_POINT('Ctrl Pts',(43.1481717937157,5.52134683388074,9.34999999998855));
#22421=CARTESIAN_POINT('Origin',(-1.73472347597681E-15,-1.73472347597681E-15,
11.35));
#22422=CARTESIAN_POINT('Ctrl Pts',(42.6782125485618,8.41547227788107,9.34999999998855));
#22423=CARTESIAN_POINT('Ctrl Pts',(42.6666509488314,8.47410575612239,8.81613492202559));
#22424=CARTESIAN_POINT('Ctrl Pts',(42.6537760879159,8.53875628688309,8.29345816614751));
#22425=CARTESIAN_POINT('Ctrl Pts',(42.6257917236771,8.67737897897861,7.21621640088911));
#22426=CARTESIAN_POINT('Ctrl Pts',(42.6113457422261,8.74802009690499,6.68773764820129));
#22427=CARTESIAN_POINT('Ctrl Pts',(42.5975402169653,8.81473581362641,6.16441400296896));
#22428=CARTESIAN_POINT('Ctrl Pts',(42.1324948509395,10.8214083018598,6.16441400296896));
#22429=CARTESIAN_POINT('Ctrl Pts',(42.0949797587143,10.9674710310278,6.7006213856072));
#22430=CARTESIAN_POINT('Ctrl Pts',(42.0588133989564,11.1051851219338,7.2178432770461));
#22431=CARTESIAN_POINT('Ctrl Pts',(41.9877513997447,11.3709120573994,8.2837360279465));
#22432=CARTESIAN_POINT('Ctrl Pts',(41.9541547454921,11.4940135235905,8.81321169230966));
#22433=CARTESIAN_POINT('Ctrl Pts',(41.9232160376674,11.6057725748471,9.34999999998855));
#22434=CARTESIAN_POINT('Origin',(-1.73472347597681E-15,-1.73472347597681E-15,
11.35));
#22435=CARTESIAN_POINT('Ctrl Pts',(41.0461633054984,14.4035578208427,9.34999999998854));
#22436=CARTESIAN_POINT('Ctrl Pts',(41.0263749722095,14.4599491076222,8.8161349220256));
#22437=CARTESIAN_POINT('Ctrl Pts',(41.0044304289846,14.5221093054492,8.29345816614753));
#22438=CARTESIAN_POINT('Ctrl Pts',(40.9570029893926,14.6553380062868,7.2162198118858));
#22439=CARTESIAN_POINT('Ctrl Pts',(40.9326504745967,14.7232050398854,6.6877344133491));
#22440=CARTESIAN_POINT('Ctrl Pts',(40.9094909763996,14.7872765596604,6.16441400296896));
#22441=CARTESIAN_POINT('Ctrl Pts',(40.1635998310295,16.7073411592907,6.16441400296896));
#22442=CARTESIAN_POINT('Ctrl Pts',(40.1056796946715,16.8465782261981,6.70062138560777));
#22443=CARTESIAN_POINT('Ctrl Pts',(40.0502826977332,16.977743576586,7.2178432770462));
#22444=CARTESIAN_POINT('Ctrl Pts',(39.9421271213649,17.2306526180698,8.2837360279462));
#22445=CARTESIAN_POINT('Ctrl Pts',(39.8913532673581,17.3477197864164,8.81321169230956));
#22446=CARTESIAN_POINT('Ctrl Pts',(39.8448244996638,17.453938254474,9.34999999998855));
#22447=CARTESIAN_POINT('Origin',(-1.73472347597681E-15,-1.73472347597681E-15,
11.35));
#22448=CARTESIAN_POINT('Ctrl Pts',(38.5785325448955,20.0984284630028,9.34999999998854));
#22449=CARTESIAN_POINT('Ctrl Pts',(38.550920311449,20.1514295943407,8.81613492202552));
#22450=CARTESIAN_POINT('Ctrl Pts',(38.5203528135319,20.2098340568614,8.29345816614715));
#22451=CARTESIAN_POINT('Ctrl Pts',(38.4544476958772,20.3349570532291,7.21621981188606));
#22452=CARTESIAN_POINT('Ctrl Pts',(38.4206845686578,20.3986675740772,6.68773441334892));
#22453=CARTESIAN_POINT('Ctrl Pts',(38.3886424727845,20.4587909979239,6.16441400296896));
#22454=CARTESIAN_POINT('Ctrl Pts',(37.3770911258214,22.2531584044164,6.16440437643718));
#22455=CARTESIAN_POINT('Ctrl Pts',(37.2999450322789,22.3827353439075,6.70061175907635));
#22456=CARTESIAN_POINT('Ctrl Pts',(37.2264437362621,22.5046841317884,7.21784327704632));
#22457=CARTESIAN_POINT('Ctrl Pts',(37.0833963183771,22.7396267805354,8.28373602794611));
#22458=CARTESIAN_POINT('Ctrl Pts',(37.0164788738639,22.8482765010836,8.81321169230953));
#22459=CARTESIAN_POINT('Ctrl Pts',(36.9553072378326,22.9467920842413,9.34999999998855));
#22460=CARTESIAN_POINT('Origin',(-1.73472347597681E-15,-1.73472347597681E-15,
11.35));
#22461=CARTESIAN_POINT('Ctrl Pts',(35.3255541129795,25.3841530607377,9.34999999998854));
#22462=CARTESIAN_POINT('Ctrl Pts',(35.2906800848213,25.4326850864426,8.8161349220256));
#22463=CARTESIAN_POINT('Ctrl Pts',(35.2521118983203,25.4861448672246,8.29345816614758));
#22464=CARTESIAN_POINT('Ctrl Pts',(35.1690707407436,25.6006150157413,7.21621981188613));
#22465=CARTESIAN_POINT('Ctrl Pts',(35.126584321006,25.6588720613604,6.6877344133489));
#22466=CARTESIAN_POINT('Ctrl Pts',(35.0863119121266,25.713823449751,6.16441400296896));
#22467=CARTESIAN_POINT('Ctrl Pts',(33.8296898901082,27.3459701224717,6.16441400296896));
#22468=CARTESIAN_POINT('Ctrl Pts',(33.7348883113749,27.4632491217274,6.70062138560785));
#22469=CARTESIAN_POINT('Ctrl Pts',(33.6447817325195,27.5734942162174,7.21784327704626));
#22470=CARTESIAN_POINT('Ctrl Pts',(33.4697545060313,27.7856877174178,8.28373602794632));
#22471=CARTESIAN_POINT('Ctrl Pts',(33.388055717208,27.8837081951773,8.81321169230959));
#22472=CARTESIAN_POINT('Ctrl Pts',(33.3134864909448,27.9725154002575,9.34999999998854));
#22473=CARTESIAN_POINT('Origin',(-1.73472347597681E-15,-1.73472347597681E-15,
11.35));
#22474=CARTESIAN_POINT('Ctrl Pts',(31.3534492698091,30.1531295040086,9.34999999998854));
#22475=CARTESIAN_POINT('Ctrl Pts',(31.312023381584,30.1962044519919,8.81613492202545));
#22476=CARTESIAN_POINT('Ctrl Pts',(31.2662396435547,30.2436312640639,8.29345816614677));
#22477=CARTESIAN_POINT('Ctrl Pts',(31.1677529245535,30.3451182826104,7.21621981188611));
#22478=CARTESIAN_POINT('Ctrl Pts',(31.1174081132829,30.396735907551,6.68773441334884));
#22479=CARTESIAN_POINT('Ctrl Pts',(31.0697252215062,30.4453966086846,6.16441400296896));
#22480=CARTESIAN_POINT('Ctrl Pts',(29.593615110006,31.882094421804,6.16441400296896));
#22481=CARTESIAN_POINT('Ctrl Pts',(29.4830879328398,31.9846880186041,6.70062138560775));
#22482=CARTESIAN_POINT('Ctrl Pts',(29.3782089962414,32.0809874737954,7.21784327704626));
#22483=CARTESIAN_POINT('Ctrl Pts',(29.1747650107445,32.2661121796802,8.28373602794619));
#22484=CARTESIAN_POINT('Ctrl Pts',(29.0799480293516,32.3515080003914,8.81321169230955));
#22485=CARTESIAN_POINT('Ctrl Pts',(28.9934992272633,32.4287989687975,9.34999999998855));
#22486=CARTESIAN_POINT('Origin',(-1.73472347597681E-15,-1.73472347597681E-15,
11.35));
#22487=CARTESIAN_POINT('Ctrl Pts',(26.7430786153867,34.3082751850228,9.34999999998854));
#22488=CARTESIAN_POINT('Ctrl Pts',(26.6959441787167,34.3450161735616,8.81613492202541));
#22489=CARTESIAN_POINT('Ctrl Pts',(26.6438769140359,34.3854445437972,8.29345816614648));
#22490=CARTESIAN_POINT('Ctrl Pts',(26.5319495391968,34.4718824493405,7.21621981188615));
#22491=CARTESIAN_POINT('Ctrl Pts',(26.4747712115682,34.5158098676118,6.68773441334885));
#22492=CARTESIAN_POINT('Ctrl Pts',(26.4206485230647,34.5571892899391,6.16441400296896));
#22493=CARTESIAN_POINT('Ctrl Pts',(24.7550996672029,35.7691912190764,6.16441400296896));
#22494=CARTESIAN_POINT('Ctrl Pts',(24.6310969061966,35.8550109036457,6.70062138560821));
#22495=CARTESIAN_POINT('Ctrl Pts',(24.5135806445585,35.9354043403352,7.21784327704631));
#22496=CARTESIAN_POINT('Ctrl Pts',(24.2858614329136,36.0896916457482,8.28373602794605));
#22497=CARTESIAN_POINT('Ctrl Pts',(24.1798564592628,36.1607243967627,8.81321169230951));
#22498=CARTESIAN_POINT('Ctrl Pts',(24.0832879296622,36.2249257072667,9.34999999998855));
#22499=CARTESIAN_POINT('Origin',(-1.73472347597681E-15,-1.73472347597681E-15,
11.35));
#22500=CARTESIAN_POINT('Ctrl Pts',(21.5882960010253,37.7650033201656,9.34999999998854));
#22501=CARTESIAN_POINT('Ctrl Pts',(21.5364125371165,37.7946624086854,8.81613492202566));
#22502=CARTESIAN_POINT('Ctrl Pts',(21.4791216851438,37.8272693320525,8.29345816614794));
#22503=CARTESIAN_POINT('Ctrl Pts',(21.3560321730463,37.896898498102,7.21621981188577));
#22504=CARTESIAN_POINT('Ctrl Pts',(21.2931843149217,37.9322414741441,6.6877344133491));
#22505=CARTESIAN_POINT('Ctrl Pts',(21.2337236115522,37.9654972519551,6.16441400296897));
#22506=CARTESIAN_POINT('Ctrl Pts',(19.4126417829879,38.9281304329581,6.16441400296896));
#22507=CARTESIAN_POINT('Ctrl Pts',(19.2776877767614,38.9954291640021,6.70062138560747));
#22508=CARTESIAN_POINT('Ctrl Pts',(19.1499264822816,39.0582800036544,7.21784327704618));
#22509=CARTESIAN_POINT('Ctrl Pts',(18.9025677509496,39.1785890639853,8.28373602794654));
#22510=CARTESIAN_POINT('Ctrl Pts',(18.7875327406113,39.2338127233339,8.81321169230967));
#22511=CARTESIAN_POINT('Ctrl Pts',(18.6828103402805,39.2836174223952,9.34999999998855));
#22512=CARTESIAN_POINT('Origin',(-1.73472347597681E-15,-1.73472347597681E-15,
11.35));
#22513=CARTESIAN_POINT('Ctrl Pts',(15.9940379355878,40.4529448929863,9.34999999998854));
#22514=CARTESIAN_POINT('Ctrl Pts',(15.9384616421457,40.4749183079745,8.81613492202557));
#22515=CARTESIAN_POINT('Ctrl Pts',(15.8771134794139,40.4990400015441,8.29345816614744));
#22516=CARTESIAN_POINT('Ctrl Pts',(15.7453671603999,40.5504431418366,7.2162164008887));
#22517=CARTESIAN_POINT('Ctrl Pts',(15.6781299831607,40.5764818806474,6.68773764820152));
#22518=CARTESIAN_POINT('Ctrl Pts',(15.6145413203109,40.6009371733745,6.16441400296895));
#22519=CARTESIAN_POINT('Ctrl Pts',(13.6749984935073,41.2946051706827,6.16441400296896));
#22520=CARTESIAN_POINT('Ctrl Pts',(13.5318405164522,41.342012940111,6.70062138560718));
#22521=CARTESIAN_POINT('Ctrl Pts',(13.396435040653,41.3860417208776,7.21784327704614));
#22522=CARTESIAN_POINT('Ctrl Pts',(13.1344723000804,41.4699233906007,8.28373602794635));
#22523=CARTESIAN_POINT('Ctrl Pts',(13.0127490341315,41.508213763831,8.81321169230961));
#22524=CARTESIAN_POINT('Ctrl Pts',(12.9020046091466,41.5426079714016,9.34999999998854));
#22525=CARTESIAN_POINT('Origin',(-1.73472347597681E-15,-1.73472347597681E-15,
11.35));
#22526=CARTESIAN_POINT('Ctrl Pts',(10.0741873807783,42.3173811644455,9.34999999998854));
#22527=CARTESIAN_POINT('Ctrl Pts',(10.0160496308688,42.3312215905392,8.81613492202556));
#22528=CARTESIAN_POINT('Ctrl Pts',(9.95189302905758,42.3463670061913,8.2934581661474));
#22529=CARTESIAN_POINT('Ctrl Pts',(9.81417270409262,42.3784973788108,7.21621981188586));
#22530=CARTESIAN_POINT('Ctrl Pts',(9.74391335880857,42.3947024282284,6.68773441334904));
#22531=CARTESIAN_POINT('Ctrl Pts',(9.67749199640696,42.4098590973783,6.16441400296896));
#22532=CARTESIAN_POINT('Ctrl Pts',(7.65897167013808,42.8204408309399,6.16441400296896));
#22533=CARTESIAN_POINT('Ctrl Pts',(7.51052400583346,42.8469925532796,6.70062138560763));
#22534=CARTESIAN_POINT('Ctrl Pts',(7.37023081372529,42.8713029761526,7.2178432770462));
#22535=CARTESIAN_POINT('Ctrl Pts',(7.09899686987191,42.9170496663671,8.28373602794623));
#22536=CARTESIAN_POINT('Ctrl Pts',(6.97306328298622,42.9376272719005,8.81321169230957));
#22537=CARTESIAN_POINT('Ctrl Pts',(6.85855127047942,42.955910821099,9.34999999998854));
#22538=CARTESIAN_POINT('Origin',(-1.73472347597681E-15,-1.73472347597681E-15,
11.35));
#22539=CARTESIAN_POINT('Ctrl Pts',(3.9492554224537,43.3203575886467,9.34999999998854));
#22540=CARTESIAN_POINT('Ctrl Pts',(3.88973973300936,43.3257832746831,8.81613492202564));
#22541=CARTESIAN_POINT('Ctrl Pts',(3.82408073551934,43.3316440954308,8.29345816614775));
#22542=CARTESIAN_POINT('Ctrl Pts',(3.68318912998151,43.343847820053,7.21621640088861));
#22543=CARTESIAN_POINT('Ctrl Pts',(3.6113395703927,43.3498889051253,6.68773764820155));
#22544=CARTESIAN_POINT('Ctrl Pts',(3.54343684303852,43.3554385900939,6.16441400296896));
#22545=CARTESIAN_POINT('Ctrl Pts',(1.48703027021497,43.4745757998335,6.16441400296896));
#22546=CARTESIAN_POINT('Ctrl Pts',(1.33631488501848,43.4797309585866,6.70062138560754));
#22547=CARTESIAN_POINT('Ctrl Pts',(1.19398994142034,43.4838281334618,7.21784327704621));
#22548=CARTESIAN_POINT('Ctrl Pts',(0.9190063352089,43.4905085734774,8.28373602794634));
#22549=CARTESIAN_POINT('Ctrl Pts',(0.791426072052943,43.4929545106062,8.8132116923096));
#22550=CARTESIAN_POINT('Ctrl Pts',(0.675477606373541,43.4947552010963,9.34999999998854));
#22551=CARTESIAN_POINT('Origin',(-1.73472347597681E-15,-1.73472347597681E-15,
11.35));
#22552=CARTESIAN_POINT('Ctrl Pts',(-2.25607087657641,43.4414565156357,9.35000993791518));
#22553=CARTESIAN_POINT('Ctrl Pts',(-2.31575293774753,43.4383570102934,8.81614485995224));
#22554=CARTESIAN_POINT('Ctrl Pts',(-2.38157881405629,43.4348138690301,8.29345816614757));
#22555=CARTESIAN_POINT('Ctrl Pts',(-2.52277267021449,43.4268424365167,7.21621981188565));
#22556=CARTESIAN_POINT('Ctrl Pts',(-2.59475150835141,43.4225967225811,6.68773441334928));
#22557=CARTESIAN_POINT('Ctrl Pts',(-2.66275246602649,43.4184263798755,6.16441400296896));
#22558=CARTESIAN_POINT('Ctrl Pts',(-4.7151827777679,43.2436937757662,6.16441400296896));
#22559=CARTESIAN_POINT('Ctrl Pts',(-4.86509775324099,43.2273474267669,6.70062138560767));
#22560=CARTESIAN_POINT('Ctrl Pts',(-5.00655712290862,43.211147946979,7.21784327704619));
#22561=CARTESIAN_POINT('Ctrl Pts',(-5.27969251824286,43.1786261423019,8.28373602794632));
#22562=CARTESIAN_POINT('Ctrl Pts',(-5.40632229142235,43.1628906187995,8.8132116923096));
#22563=CARTESIAN_POINT('Ctrl Pts',(-5.5213468338809,43.1481717937156,9.34999999998855));
#22564=CARTESIAN_POINT('Origin',(-1.73472347597681E-15,-1.73472347597681E-15,
11.35));
#22565=CARTESIAN_POINT('Ctrl Pts',(-8.41547227788122,42.6782125485618,9.34999999998854));
#22566=CARTESIAN_POINT('Ctrl Pts',(-8.47410575612254,42.6666509488314,8.8161349220256));
#22567=CARTESIAN_POINT('Ctrl Pts',(-8.53875628688322,42.6537760879159,8.29345816614766));
#22568=CARTESIAN_POINT('Ctrl Pts',(-8.67737854004153,42.6257918122873,7.21621981188561));
#22569=CARTESIAN_POINT('Ctrl Pts',(-8.74802050929902,42.6113456568892,6.68773441334929));
#22570=CARTESIAN_POINT('Ctrl Pts',(-8.81473581362657,42.5975402169653,6.16441400296896));
#22571=CARTESIAN_POINT('Ctrl Pts',(-10.82140830186,42.1324948509394,6.16441400296896));
#22572=CARTESIAN_POINT('Ctrl Pts',(-10.9674710310281,42.0949797587142,6.70062138560754));
#22573=CARTESIAN_POINT('Ctrl Pts',(-11.105185121934,42.0588133989564,7.21784327704616));
#22574=CARTESIAN_POINT('Ctrl Pts',(-11.3709120573995,41.9877513997446,8.28373602794637));
#22575=CARTESIAN_POINT('Ctrl Pts',(-11.4940135235907,41.9541547454921,8.81321169230963));
#22576=CARTESIAN_POINT('Ctrl Pts',(-11.6057725748473,41.9232160376673,9.34999999998855));
#22577=CARTESIAN_POINT('Origin',(-1.73472347597681E-15,-1.73472347597681E-15,
11.35));
#22578=CARTESIAN_POINT('Ctrl Pts',(-14.4035578208429,41.0461633054983,9.34999999998854));
#22579=CARTESIAN_POINT('Ctrl Pts',(-14.4599491076224,41.0263749722094,8.81613492202563));
#22580=CARTESIAN_POINT('Ctrl Pts',(-14.5221093054493,41.0044304289846,8.29345816614773));
#22581=CARTESIAN_POINT('Ctrl Pts',(-14.655338006287,40.9570029893926,7.2162198118857));
#22582=CARTESIAN_POINT('Ctrl Pts',(-14.7232050398856,40.9326504745966,6.68773441334913));
#22583=CARTESIAN_POINT('Ctrl Pts',(-14.7872765596605,40.9094909763996,6.16441400296896));
#22584=CARTESIAN_POINT('Ctrl Pts',(-16.7073411592909,40.1635998310295,6.16441400296896));
#22585=CARTESIAN_POINT('Ctrl Pts',(-16.8465782261982,40.1056796946715,6.70062138560753));
#22586=CARTESIAN_POINT('Ctrl Pts',(-16.9777435765862,40.0502826977332,7.21784327704622));
#22587=CARTESIAN_POINT('Ctrl Pts',(-17.23065261807,39.9421271213648,8.28373602794643));
#22588=CARTESIAN_POINT('Ctrl Pts',(-17.3477197864166,39.891353267358,8.81321169230964));
#22589=CARTESIAN_POINT('Ctrl Pts',(-17.4539382544742,39.8448244996638,9.34999999998855));
#22590=CARTESIAN_POINT('Origin',(-1.73472347597681E-15,-1.73472347597681E-15,
11.35));
#22591=CARTESIAN_POINT('Ctrl Pts',(-20.0984284630029,38.5785325448954,9.34999999998854));
#22592=CARTESIAN_POINT('Ctrl Pts',(-20.1514295943409,38.5509203114489,8.8161349220255));
#22593=CARTESIAN_POINT('Ctrl Pts',(-20.2098340568615,38.5203528135319,8.29345816614704));
#22594=CARTESIAN_POINT('Ctrl Pts',(-20.3349570532293,38.4544476958771,7.21621981188546));
#22595=CARTESIAN_POINT('Ctrl Pts',(-20.3986675740773,38.4206845686577,6.68773441334931));
#22596=CARTESIAN_POINT('Ctrl Pts',(-20.458790997924,38.3886424727844,6.16441400296896));
#22597=CARTESIAN_POINT('Ctrl Pts',(-22.2531607307118,37.3770897408173,6.16441400296896));
#22598=CARTESIAN_POINT('Ctrl Pts',(-22.3827376702031,37.2999436472748,6.70062138560852));
#22599=CARTESIAN_POINT('Ctrl Pts',(-22.5046841317886,37.226443736262,7.21784327704636));
#22600=CARTESIAN_POINT('Ctrl Pts',(-22.7396267805356,37.083396318377,8.28373602794636));
#22601=CARTESIAN_POINT('Ctrl Pts',(-22.8482765010838,37.0164788738638,8.81321169230961));
#22602=CARTESIAN_POINT('Ctrl Pts',(-22.9467920842415,36.9553072378325,9.34999999998855));
#22603=CARTESIAN_POINT('Origin',(-1.73472347597681E-15,-1.73472347597681E-15,
11.35));
#22604=CARTESIAN_POINT('Ctrl Pts',(-25.3841530607378,35.3255541129794,9.34999999998854));
#22605=CARTESIAN_POINT('Ctrl Pts',(-25.4326850864427,35.2906800848212,8.8161349220256));
#22606=CARTESIAN_POINT('Ctrl Pts',(-25.4861448672247,35.2521118983202,8.29345816614765));
#22607=CARTESIAN_POINT('Ctrl Pts',(-25.6006150157415,35.1690707407435,7.21621981188596));
#22608=CARTESIAN_POINT('Ctrl Pts',(-25.6588720613605,35.1265843210059,6.68773441334894));
#22609=CARTESIAN_POINT('Ctrl Pts',(-25.7138234497511,35.0863119121265,6.16441400296896));
#22610=CARTESIAN_POINT('Ctrl Pts',(-27.3459701224718,33.8296898901081,6.16441400296896));
#22611=CARTESIAN_POINT('Ctrl Pts',(-27.4632491217274,33.7348883113749,6.70062138560753));
#22612=CARTESIAN_POINT('Ctrl Pts',(-27.5734942162175,33.6447817325194,7.2178432770462));
#22613=CARTESIAN_POINT('Ctrl Pts',(-27.785687717418,33.4697545060312,8.28373602794646));
#22614=CARTESIAN_POINT('Ctrl Pts',(-27.8837081951774,33.3880557172079,8.81321169230965));
#22615=CARTESIAN_POINT('Ctrl Pts',(-27.9725154002576,33.3134864909447,9.34999999998855));
#22616=CARTESIAN_POINT('Origin',(-1.73472347597681E-15,-1.73472347597681E-15,
11.35));
#22617=CARTESIAN_POINT('Ctrl Pts',(-30.1531295040087,31.353449269809,9.34999999998854));
#22618=CARTESIAN_POINT('Ctrl Pts',(-30.196204451992,31.3120233815839,8.81613492202546));
#22619=CARTESIAN_POINT('Ctrl Pts',(-30.243631264064,31.2662396435546,8.29345816614692));
#22620=CARTESIAN_POINT('Ctrl Pts',(-30.3451182826105,31.1677529245534,7.21621981188656));
#22621=CARTESIAN_POINT('Ctrl Pts',(-30.3967359075512,31.1174081132828,6.68773441334847));
#22622=CARTESIAN_POINT('Ctrl Pts',(-30.4453966086847,31.0697252215061,6.16441400296896));
#22623=CARTESIAN_POINT('Ctrl Pts',(-31.8820944218041,29.5936151100059,6.16441400296896));
#22624=CARTESIAN_POINT('Ctrl Pts',(-31.9846880186042,29.4830879328396,6.70062138560796));
#22625=CARTESIAN_POINT('Ctrl Pts',(-32.0809874737955,29.3782089962413,7.21784327704624));
#22626=CARTESIAN_POINT('Ctrl Pts',(-32.2661121796803,29.1747650107444,8.2837360279461));
#22627=CARTESIAN_POINT('Ctrl Pts',(-32.3515080003915,29.0799480293515,8.81321169230952));
#22628=CARTESIAN_POINT('Ctrl Pts',(-32.4287989687976,28.9934992272632,9.34999999998854));
#22629=CARTESIAN_POINT('Origin',(-1.73472347597681E-15,-1.73472347597681E-15,
11.35));
#22630=CARTESIAN_POINT('Ctrl Pts',(-37.7650033201657,21.5882960010252,9.34999999998855));
#22631=CARTESIAN_POINT('Ctrl Pts',(-37.7946624086854,21.5364125371163,8.81613492202542));
#22632=CARTESIAN_POINT('Ctrl Pts',(-37.8272693320526,21.4791216851435,8.29345816614661));
#22633=CARTESIAN_POINT('Ctrl Pts',(-37.896898498102,21.3560321730462,7.21621981188615));
#22634=CARTESIAN_POINT('Ctrl Pts',(-37.9322414741442,21.2931843149215,6.68773441334878));
#22635=CARTESIAN_POINT('Ctrl Pts',(-37.9654972519552,21.2337236115521,6.16441400296896));
#22636=CARTESIAN_POINT('Ctrl Pts',(-38.9281304329582,19.4126417829877,6.16441400296896));
#22637=CARTESIAN_POINT('Ctrl Pts',(-38.9954291640021,19.2776877767614,6.70062138560718));
#22638=CARTESIAN_POINT('Ctrl Pts',(-39.0582800036545,19.1499264822814,7.21784327704614));
#22639=CARTESIAN_POINT('Ctrl Pts',(-39.1785890639854,18.9025677509495,8.28373602794646));
#22640=CARTESIAN_POINT('Ctrl Pts',(-39.233812723334,18.7875327406112,8.81321169230965));
#22641=CARTESIAN_POINT('Ctrl Pts',(-39.2836174223953,18.6828103402803,9.34999999998855));
#22642=CARTESIAN_POINT('Origin',(-1.73472347597681E-15,-1.73472347597681E-15,
11.35));
#22643=CARTESIAN_POINT('Ctrl Pts',(-34.3082751850229,26.7430786153866,9.34999999998854));
#22644=CARTESIAN_POINT('Ctrl Pts',(-34.3450161735616,26.6959441787166,8.81613492202578));
#22645=CARTESIAN_POINT('Ctrl Pts',(-34.3854445437971,26.643876914036,8.29345816614856));
#22646=CARTESIAN_POINT('Ctrl Pts',(-34.4718824493406,26.5319495391966,7.21621981188526));
#22647=CARTESIAN_POINT('Ctrl Pts',(-34.5158098676118,26.4747712115682,6.68773441334945));
#22648=CARTESIAN_POINT('Ctrl Pts',(-34.5571892899392,26.4206485230645,6.16441400296896));
#22649=CARTESIAN_POINT('Ctrl Pts',(-35.7691912190765,24.7550996672027,6.16441400296896));
#22650=CARTESIAN_POINT('Ctrl Pts',(-35.8550109036458,24.6310969061965,6.7006213856079));
#22651=CARTESIAN_POINT('Ctrl Pts',(-35.9354043403353,24.5135806445584,7.21784327704629));
#22652=CARTESIAN_POINT('Ctrl Pts',(-36.0896916457483,24.2858614329134,8.28373602794633));
#22653=CARTESIAN_POINT('Ctrl Pts',(-36.1607243967628,24.1798564592627,8.8132116923096));
#22654=CARTESIAN_POINT('Ctrl Pts',(-36.2249257072668,24.0832879296621,9.34999999998854));
#22655=CARTESIAN_POINT('Origin',(-1.73472347597681E-15,-1.73472347597681E-15,
11.35));
#22656=CARTESIAN_POINT('Ctrl Pts',(-40.4529448929863,15.9940379355876,9.34999999998855));
#22657=CARTESIAN_POINT('Ctrl Pts',(-40.4749183079746,15.9384616421456,8.8161349220257));
#22658=CARTESIAN_POINT('Ctrl Pts',(-40.4990400015441,15.8771134794139,8.29345816614812));
#22659=CARTESIAN_POINT('Ctrl Pts',(-40.5504429790729,15.7453675775636,7.2162198118858));
#22660=CARTESIAN_POINT('Ctrl Pts',(-40.5764820318145,15.678129590096,6.68773441334901));
#22661=CARTESIAN_POINT('Ctrl Pts',(-40.6009371733746,15.6145413203108,6.16441400296896));
#22662=CARTESIAN_POINT('Ctrl Pts',(-41.2946051706828,13.6749984935071,6.16441400296895));
#22663=CARTESIAN_POINT('Ctrl Pts',(-41.3420129401111,13.5318405164519,6.70062138560768));
#22664=CARTESIAN_POINT('Ctrl Pts',(-41.3860417208777,13.3964350406529,7.21784327704624));
#22665=CARTESIAN_POINT('Ctrl Pts',(-41.4699233906007,13.1344723000802,8.28373602794634));
#22666=CARTESIAN_POINT('Ctrl Pts',(-41.5082137638311,13.0127490341314,8.81321169230959));
#22667=CARTESIAN_POINT('Ctrl Pts',(-41.5426079714017,12.9020046091465,9.34999999998854));
#22668=CARTESIAN_POINT('Origin',(-1.73472347597681E-15,-1.73472347597681E-15,
11.35));
#22669=CARTESIAN_POINT('Ctrl Pts',(-42.3173809068055,10.0741884630147,9.35000993791518));
#22670=CARTESIAN_POINT('Ctrl Pts',(-42.3312213328992,10.0160507131051,8.81614485995214));
#22671=CARTESIAN_POINT('Ctrl Pts',(-42.3463670061913,9.95189302905741,8.29345816614713));
#22672=CARTESIAN_POINT('Ctrl Pts',(-42.3784973788108,9.81417270409247,7.2162198118858));
#22673=CARTESIAN_POINT('Ctrl Pts',(-42.3947024282285,9.74391335880843,6.68773441334909));
#22674=CARTESIAN_POINT('Ctrl Pts',(-42.4098590973783,9.67749199640681,6.16441400296896));
#22675=CARTESIAN_POINT('Ctrl Pts',(-42.8204408309399,7.65897167013792,6.16441400296896));
#22676=CARTESIAN_POINT('Ctrl Pts',(-42.8469925532797,7.51052400583325,6.7006213856078));
#22677=CARTESIAN_POINT('Ctrl Pts',(-42.8713029761526,7.37023081372511,7.21784327704623));
#22678=CARTESIAN_POINT('Ctrl Pts',(-42.9170496663671,7.09899686987174,8.28373602794625));
#22679=CARTESIAN_POINT('Ctrl Pts',(-42.9376272719005,6.97306328298604,8.81321169230957));
#22680=CARTESIAN_POINT('Ctrl Pts',(-42.955910821099,6.85855127047925,9.34999999998854));
#22681=CARTESIAN_POINT('Origin',(-1.73472347597681E-15,-1.73472347597681E-15,
11.35));
#22682=CARTESIAN_POINT('Ctrl Pts',(-43.3203574876474,3.94925653034038,9.35000993791518));
#22683=CARTESIAN_POINT('Ctrl Pts',(-43.3257831736837,3.88974084089603,8.81614485995219));
#22684=CARTESIAN_POINT('Ctrl Pts',(-43.3316440954308,3.82408073551913,8.29345816614738));
#22685=CARTESIAN_POINT('Ctrl Pts',(-43.343847820053,3.68318912998135,7.21621640088867));
#22686=CARTESIAN_POINT('Ctrl Pts',(-43.3498889051253,3.61133957039253,6.68773764820154));
#22687=CARTESIAN_POINT('Ctrl Pts',(-43.3554385900939,3.54343684303836,6.16441400296897));
#22688=CARTESIAN_POINT('Ctrl Pts',(-43.4745757998335,1.48703027021514,6.16441400296896));
#22689=CARTESIAN_POINT('Ctrl Pts',(-43.4797309585866,1.33631488501862,6.70062138560764));
#22690=CARTESIAN_POINT('Ctrl Pts',(-43.4838281334618,1.19398994142049,7.21784327704629));
#22691=CARTESIAN_POINT('Ctrl Pts',(-43.4905085734774,0.919006335208971,
8.28373602794674));
#22692=CARTESIAN_POINT('Ctrl Pts',(-43.4929545106062,0.79142607205295,8.81321169231029));
#22693=CARTESIAN_POINT('Ctrl Pts',(-43.4947552010963,0.675477606373505,
9.34999999998951));
#22694=CARTESIAN_POINT('Origin',(-1.73472347597681E-15,-1.73472347597681E-15,
11.35));
#22695=CARTESIAN_POINT('Ctrl Pts',(-43.4414564579383,-2.25607198755999,
9.3499999999895));
#22696=CARTESIAN_POINT('Ctrl Pts',(-43.438356952596,-2.31575404873114,8.81613492202627));
#22697=CARTESIAN_POINT('Ctrl Pts',(-43.4348138690301,-2.38157881405607,
8.29345816614802));
#22698=CARTESIAN_POINT('Ctrl Pts',(-43.4268424112758,-2.52277311729442,
7.21621640088862));
#22699=CARTESIAN_POINT('Ctrl Pts',(-43.4225967483597,-2.59475108801018,
6.68773764820165));
#22700=CARTESIAN_POINT('Ctrl Pts',(-43.4184263798756,-2.66275246602632,
6.16441400296896));
#22701=CARTESIAN_POINT('Ctrl Pts',(-43.2436937757662,-4.71518277776806,
6.16441400296896));
#22702=CARTESIAN_POINT('Ctrl Pts',(-43.2273474267669,-4.86509775324113,
6.70062138560761));
#22703=CARTESIAN_POINT('Ctrl Pts',(-43.211147946979,-5.00655712290883,7.21784327704638));
#22704=CARTESIAN_POINT('Ctrl Pts',(-43.1786261423019,-5.27969251824321,
8.2837360279471));
#22705=CARTESIAN_POINT('Ctrl Pts',(-43.1628906187995,-5.40632229142282,
8.81321169231093));
#22706=CARTESIAN_POINT('Ctrl Pts',(-43.1481717937156,-5.52134683388146,
9.34999999999046));
#22707=CARTESIAN_POINT('Origin',(-1.73472347597681E-15,-1.73472347597681E-15,
11.35));
#22708=CARTESIAN_POINT('Ctrl Pts',(-42.6782127637814,-8.41547118641672,
9.3500099379171));
#22709=CARTESIAN_POINT('Ctrl Pts',(-42.666651164051,-8.47410466465809,8.81614485995349));
#22710=CARTESIAN_POINT('Ctrl Pts',(-42.6537760879159,-8.53875628688335,
8.29345816614791));
#22711=CARTESIAN_POINT('Ctrl Pts',(-42.6257917236771,-8.6773789789789,7.2162164008893));
#22712=CARTESIAN_POINT('Ctrl Pts',(-42.6113457422261,-8.74802009690531,
6.68773764820119));
#22713=CARTESIAN_POINT('Ctrl Pts',(-42.5975402169652,-8.81473581362672,
6.16441400296896));
#22714=CARTESIAN_POINT('Ctrl Pts',(-42.1324948509394,-10.8214083018602,
6.16441400296896));
#22715=CARTESIAN_POINT('Ctrl Pts',(-42.0949797587142,-10.9674710310282,
6.70062138560751));
#22716=CARTESIAN_POINT('Ctrl Pts',(-42.0588133989563,-11.1051851219342,
7.21784327704638));
#22717=CARTESIAN_POINT('Ctrl Pts',(-41.9877513997445,-11.3709120573999,
8.28373602794749));
#22718=CARTESIAN_POINT('Ctrl Pts',(-41.9541547454919,-11.4940135235913,
8.81321169231162));
#22719=CARTESIAN_POINT('Ctrl Pts',(-41.9232160376671,-11.605772574848,9.34999999999142));
#22720=CARTESIAN_POINT('Origin',(-1.73472347597681E-15,-1.73472347597681E-15,
11.35));
#22721=CARTESIAN_POINT('Ctrl Pts',(-41.0461633054984,-14.4035578208427,
9.34999999999141));
#22722=CARTESIAN_POINT('Ctrl Pts',(-41.0263749722095,-14.4599491076223,
8.81613492202769));
#22723=CARTESIAN_POINT('Ctrl Pts',(-41.0044304289846,-14.5221093054493,
8.29345816614916));
#22724=CARTESIAN_POINT('Ctrl Pts',(-40.9570029893925,-14.6553380062871,
7.21621981188594));
#22725=CARTESIAN_POINT('Ctrl Pts',(-40.9326504745966,-14.7232050398857,
6.68773441334922));
#22726=CARTESIAN_POINT('Ctrl Pts',(-40.9094909763995,-14.7872765596607,
6.16441400296896));
#22727=CARTESIAN_POINT('Ctrl Pts',(-40.1636008708697,-16.7073386595674,
6.16440437643718));
#22728=CARTESIAN_POINT('Ctrl Pts',(-40.1056807345117,-16.8465757264749,
6.70061175907592));
#22729=CARTESIAN_POINT('Ctrl Pts',(-40.0502826977331,-16.9777435765864,
7.21784327704649));
#22730=CARTESIAN_POINT('Ctrl Pts',(-39.9421271213646,-17.2306526180706,
8.28373602794814));
#22731=CARTESIAN_POINT('Ctrl Pts',(-39.8913532673577,-17.3477197864173,
8.81321169231236));
#22732=CARTESIAN_POINT('Ctrl Pts',(-39.8448244996634,-17.4539382544751,
9.34999999999236));
#22733=CARTESIAN_POINT('Origin',(-1.73472347597681E-15,-1.73472347597681E-15,
11.35));
#22734=CARTESIAN_POINT('Ctrl Pts',(-38.5785325448956,-20.0984284630027,
9.34999999999236));
#22735=CARTESIAN_POINT('Ctrl Pts',(-38.550920311449,-20.1514295943407,8.81613492202805));
#22736=CARTESIAN_POINT('Ctrl Pts',(-38.5203528135318,-20.2098340568616,
8.29345816614786));
#22737=CARTESIAN_POINT('Ctrl Pts',(-38.4544476958771,-20.3349570532293,
7.21621981188626));
#22738=CARTESIAN_POINT('Ctrl Pts',(-38.4206845686576,-20.3986675740774,
6.68773441334922));
#22739=CARTESIAN_POINT('Ctrl Pts',(-38.3886424727843,-20.4587909979242,
6.16441400296896));
#22740=CARTESIAN_POINT('Ctrl Pts',(-37.3770897408172,-22.253160730712,6.16441400296896));
#22741=CARTESIAN_POINT('Ctrl Pts',(-37.2999436472748,-22.382737670203,6.7006213856076));
#22742=CARTESIAN_POINT('Ctrl Pts',(-37.2264437362619,-22.5046841317887,
7.21784327704656));
#22743=CARTESIAN_POINT('Ctrl Pts',(-37.0833963183767,-22.7396267805362,
8.28373602794849));
#22744=CARTESIAN_POINT('Ctrl Pts',(-37.0164788738633,-22.8482765010846,
8.81321169231301));
#22745=CARTESIAN_POINT('Ctrl Pts',(-36.9553072378319,-22.9467920842425,
9.34999999999332));
#22746=CARTESIAN_POINT('Origin',(-1.73472347597681E-15,-1.73472347597681E-15,
11.35));
#22747=CARTESIAN_POINT('Ctrl Pts',(-35.3255541129796,-25.3841530607375,
9.34999999999331));
#22748=CARTESIAN_POINT('Ctrl Pts',(-35.2906800848214,-25.4326850864425,
8.81613492202895));
#22749=CARTESIAN_POINT('Ctrl Pts',(-35.2521118983203,-25.4861448672246,
8.29345816614959));
#22750=CARTESIAN_POINT('Ctrl Pts',(-35.1690707407434,-25.6006150157417,
7.21621981188549));
#22751=CARTESIAN_POINT('Ctrl Pts',(-35.1265843210059,-25.6588720613605,
6.68773441334979));
#22752=CARTESIAN_POINT('Ctrl Pts',(-35.0863119121265,-25.7138234497512,
6.16441400296896));
#22753=CARTESIAN_POINT('Ctrl Pts',(-33.829691592081,-27.3459680169616,6.16440437643717));
#22754=CARTESIAN_POINT('Ctrl Pts',(-33.7348900133477,-27.4632470162174,
6.70061175907647));
#22755=CARTESIAN_POINT('Ctrl Pts',(-33.6447817325192,-27.5734942162178,
7.21784327704671));
#22756=CARTESIAN_POINT('Ctrl Pts',(-33.4697545060307,-27.7856877174186,
8.283736027949));
#22757=CARTESIAN_POINT('Ctrl Pts',(-33.3880557172072,-27.8837081951783,
8.81321169231373));
#22758=CARTESIAN_POINT('Ctrl Pts',(-33.3134864909438,-27.9725154002586,
9.34999999999427));
#22759=CARTESIAN_POINT('Origin',(-1.73472347597681E-15,-1.73472347597681E-15,
11.35));
#22760=CARTESIAN_POINT('Ctrl Pts',(-31.3534492698093,-30.1531295040083,
9.34999999999427));
#22761=CARTESIAN_POINT('Ctrl Pts',(-31.3120233815842,-30.1962044519918,
8.81613492202955));
#22762=CARTESIAN_POINT('Ctrl Pts',(-31.2662396435547,-30.2436312640638,
8.29345816614953));
#22763=CARTESIAN_POINT('Ctrl Pts',(-31.1677526127023,-30.3451186039619,
7.21621640088924));
#22764=CARTESIAN_POINT('Ctrl Pts',(-31.1174084080297,-30.39673560676,6.68773764820165));
#22765=CARTESIAN_POINT('Ctrl Pts',(-31.069725221506,-30.4453966086848,6.16441400296896));
#22766=CARTESIAN_POINT('Ctrl Pts',(-29.5936151100058,-31.8820944218042,
6.16441400296896));
#22767=CARTESIAN_POINT('Ctrl Pts',(-29.4830879328395,-31.9846880186044,
6.70062138560807));
#22768=CARTESIAN_POINT('Ctrl Pts',(-29.3782089962411,-32.0809874737957,
7.21784327704683));
#22769=CARTESIAN_POINT('Ctrl Pts',(-29.1747650107437,-32.266112179681,8.28373602794916));
#22770=CARTESIAN_POINT('Ctrl Pts',(-29.0799480293506,-32.3515080003924,
8.81321169231431));
#22771=CARTESIAN_POINT('Ctrl Pts',(-28.993499227262,-32.4287989687987,9.34999999999522));
#22772=CARTESIAN_POINT('Origin',(-1.73472347597681E-15,-1.73472347597681E-15,
11.35));
#22773=CARTESIAN_POINT('Ctrl Pts',(-26.7430794927964,-34.3082745010876,
9.35000993792185));
#22774=CARTESIAN_POINT('Ctrl Pts',(-26.6959450561263,-34.3450154896264,
8.81614485995699));
#22775=CARTESIAN_POINT('Ctrl Pts',(-26.6438769140361,-34.3854445437971,
8.29345816615072));
#22776=CARTESIAN_POINT('Ctrl Pts',(-26.5319495391965,-34.4718824493407,
7.21621981188563));
#22777=CARTESIAN_POINT('Ctrl Pts',(-26.4747712115681,-34.5158098676118,
6.68773441334982));
#22778=CARTESIAN_POINT('Ctrl Pts',(-26.4206485230644,-34.5571892899393,
6.16441400296896));
#22779=CARTESIAN_POINT('Ctrl Pts',(-24.7550996672026,-35.7691912190766,
6.16441400296896));
#22780=CARTESIAN_POINT('Ctrl Pts',(-24.6310969061966,-35.8550109036457,
6.7006213856071));
#22781=CARTESIAN_POINT('Ctrl Pts',(-24.5135806445582,-35.9354043403354,
7.21784327704669));
#22782=CARTESIAN_POINT('Ctrl Pts',(-24.2858614329126,-36.0896916457489,
8.28373602794951));
#22783=CARTESIAN_POINT('Ctrl Pts',(-24.1798564592615,-36.1607243967636,
8.81321169231496));
#22784=CARTESIAN_POINT('Ctrl Pts',(-24.0832879296606,-36.2249257072678,
9.34999999999617));
#22785=CARTESIAN_POINT('Origin',(-1.73472347597681E-15,-1.73472347597681E-15,
11.35));
#22786=CARTESIAN_POINT('Ctrl Pts',(-21.5882960010258,-37.7650033201653,
9.34999999999617));
#22787=CARTESIAN_POINT('Ctrl Pts',(-21.5364125371168,-37.7946624086852,
8.81613492203093));
#22788=CARTESIAN_POINT('Ctrl Pts',(-21.4791216851438,-37.8272693320525,
8.29345816615057));
#22789=CARTESIAN_POINT('Ctrl Pts',(-21.3560317832921,-37.8968987185778,
7.21621640088953));
#22790=CARTESIAN_POINT('Ctrl Pts',(-21.2931846824718,-37.932241268577,6.6877376482016));
#22791=CARTESIAN_POINT('Ctrl Pts',(-21.2337236115519,-37.9654972519553,
6.16441400296896));
#22792=CARTESIAN_POINT('Ctrl Pts',(-19.4126417829876,-38.9281304329582,
6.16441400296896));
#22793=CARTESIAN_POINT('Ctrl Pts',(-19.277687776761,-38.9954291640023,6.70062138560802));
#22794=CARTESIAN_POINT('Ctrl Pts',(-19.1499264822811,-39.0582800036546,
7.21784327704692));
#22795=CARTESIAN_POINT('Ctrl Pts',(-18.9025677509485,-39.1785890639858,
8.28373602794993));
#22796=CARTESIAN_POINT('Ctrl Pts',(-18.7875327406098,-39.2338127233347,
8.81321169231564));
#22797=CARTESIAN_POINT('Ctrl Pts',(-18.6828103402785,-39.2836174223961,
9.34999999999711));
#22798=CARTESIAN_POINT('Origin',(-1.73472347597681E-15,-1.73472347597681E-15,
11.35));
#22799=CARTESIAN_POINT('Ctrl Pts',(-15.9940379355884,-40.452944892986,9.34999999999712));
#22800=CARTESIAN_POINT('Ctrl Pts',(-15.9384616421462,-40.4749183079744,
8.81613492203165));
#22801=CARTESIAN_POINT('Ctrl Pts',(-15.8771134794141,-40.499040001544,8.29345816615128));
#22802=CARTESIAN_POINT('Ctrl Pts',(-15.7453675775635,-40.5504429790729,
7.21621981188616));
#22803=CARTESIAN_POINT('Ctrl Pts',(-15.678129590096,-40.5764820318145,6.68773441334964));
#22804=CARTESIAN_POINT('Ctrl Pts',(-15.6145413203107,-40.6009371733746,
6.16441400296896));
#22805=CARTESIAN_POINT('Ctrl Pts',(-13.674998493507,-41.2946051706828,6.16441400296896));
#22806=CARTESIAN_POINT('Ctrl Pts',(-13.5318405164519,-41.3420129401111,
6.70062138560741));
#22807=CARTESIAN_POINT('Ctrl Pts',(-13.3964350406525,-41.3860417208777,
7.21784327704686));
#22808=CARTESIAN_POINT('Ctrl Pts',(-13.1344723000791,-41.4699233906011,
8.28373602795046));
#22809=CARTESIAN_POINT('Ctrl Pts',(-13.0127490341297,-41.5082137638316,
8.81321169231636));
#22810=CARTESIAN_POINT('Ctrl Pts',(-12.9020046091443,-41.5426079714023,
9.34999999999807));
#22811=CARTESIAN_POINT('Origin',(-1.73472347597681E-15,-1.73472347597681E-15,
11.35));
#22812=CARTESIAN_POINT('Ctrl Pts',(-10.0741873807791,-42.3173811644454,
9.34999999999807));
#22813=CARTESIAN_POINT('Ctrl Pts',(-10.0160496308693,-42.3312215905391,
8.81613492203228));
#22814=CARTESIAN_POINT('Ctrl Pts',(-9.95189302905782,-42.3463670061912,
8.29345816615143));
#22815=CARTESIAN_POINT('Ctrl Pts',(-9.81417226801106,-42.3784974805493,
7.21621640088982));
#22816=CARTESIAN_POINT('Ctrl Pts',(-9.74391376938527,-42.3947023345391,
6.68773764820157));
#22817=CARTESIAN_POINT('Ctrl Pts',(-9.67749199640667,-42.4098590973784,
6.16441400296896));
#22818=CARTESIAN_POINT('Ctrl Pts',(-7.65897167013777,-42.82044083094,6.16441400296896));
#22819=CARTESIAN_POINT('Ctrl Pts',(-7.51052400583302,-42.8469925532797,
6.70062138560811));
#22820=CARTESIAN_POINT('Ctrl Pts',(-7.37023081372475,-42.8713029761527,
7.21784327704703));
#22821=CARTESIAN_POINT('Ctrl Pts',(-7.09899686987048,-42.9170496663673,
8.28373602795068));
#22822=CARTESIAN_POINT('Ctrl Pts',(-6.97306328298415,-42.9376272719008,
8.81321169231697));
#22823=CARTESIAN_POINT('Ctrl Pts',(-6.85855127047687,-42.9559108210994,
9.34999999999902));
#22824=CARTESIAN_POINT('Origin',(-1.73472347597681E-15,-1.73472347597681E-15,
11.35));
#22825=CARTESIAN_POINT('Ctrl Pts',(-3.94925542245455,-43.3203575886467,
9.34999999999902));
#22826=CARTESIAN_POINT('Ctrl Pts',(-3.88973973300997,-43.3257832746831,
8.81613492203305));
#22827=CARTESIAN_POINT('Ctrl Pts',(-3.82408073551961,-43.3316440954307,
8.29345816615224));
#22828=CARTESIAN_POINT('Ctrl Pts',(-3.68318957610294,-43.3438477814109,
7.21621981188656));
#22829=CARTESIAN_POINT('Ctrl Pts',(-3.61133915066117,-43.3498889394299,
6.68773441334963));
#22830=CARTESIAN_POINT('Ctrl Pts',(-3.54343684303821,-43.3554385900939,
6.16441400296896));
#22831=CARTESIAN_POINT('Ctrl Pts',(-1.48703027021498,-43.4745757998335,
6.16441400296896));
#22832=CARTESIAN_POINT('Ctrl Pts',(-1.33631488501835,-43.4797309585866,
6.70062138560807));
#22833=CARTESIAN_POINT('Ctrl Pts',(-1.19398994142009,-43.4838281334618,
7.21784327704716));
#22834=CARTESIAN_POINT('Ctrl Pts',(-0.919006335207703,-43.4905085734775,
8.2837360279511));
#22835=CARTESIAN_POINT('Ctrl Pts',(-0.791426072051028,-43.4929545106062,
8.81321169231764));
#22836=CARTESIAN_POINT('Ctrl Pts',(-0.675477606371082,-43.4947552010963,
9.34999999999997));
#22837=CARTESIAN_POINT('Origin',(-1.73472347597681E-15,-1.73472347597681E-15,
11.35));
#22838=CARTESIAN_POINT('',(-5.00000000000001,19.,11.35));
#22839=CARTESIAN_POINT('',(-5.00000000000001,19.,11.35));
#22840=CARTESIAN_POINT('',(5.00000000000001,19.,11.35));
#22841=CARTESIAN_POINT('',(-5.00000000000001,19.,11.35));
#22842=CARTESIAN_POINT('',(5.00000000000001,19.,11.35));
#22843=CARTESIAN_POINT('Origin',(-3.46944695195361E-15,1.73472347597681E-15,
-11.35));
#22844=CARTESIAN_POINT('',(-5.00000000000001,19.,-11.35));
#22845=CARTESIAN_POINT('',(-5.00000000000001,19.,-11.35));
#22846=CARTESIAN_POINT('',(5.,19.,-11.35));
#22847=CARTESIAN_POINT('',(5.,19.,-11.35));
#22848=CARTESIAN_POINT('',(-5.00000000000001,19.,-11.35));
#22849=CARTESIAN_POINT('Origin',(-5.00000000000001,19.,11.35));
#22850=CARTESIAN_POINT('',(-5.00000000000001,19.,11.35));
#22851=CARTESIAN_POINT('Origin',(5.00000000000001,19.,11.35));
#22852=CARTESIAN_POINT('',(5.00000000000001,19.,11.35));
#22853=CARTESIAN_POINT('Origin',(-5.00000000000001,19.,11.35));
#22854=CARTESIAN_POINT('Ctrl Pts',(1.19058808997907,-37.7800000000001,0.));
#22855=CARTESIAN_POINT('Ctrl Pts',(1.40487380426479,-37.7800000000001,3.24562220582793));
#22856=CARTESIAN_POINT('Ctrl Pts',(1.6191595185505,-39.1882226984277,6.16982677025167));
#22857=CARTESIAN_POINT('Ctrl Pts',(1.83344523283622,-40.5964453968553,9.09403133467541));
#22858=CARTESIAN_POINT('Ctrl Pts',(2.04773094712193,-43.1339750175689,11.1176436806954));
#22859=CARTESIAN_POINT('Ctrl Pts',(2.26201666140765,-45.6715046382825,13.1412560267153));
#22860=CARTESIAN_POINT('Ctrl Pts',(2.47630237569335,-48.8357523191413,13.8634749112255));
#22861=CARTESIAN_POINT('Ctrl Pts',(2.69058808997906,-52.0000000000001,14.5856937957357));
#22862=CARTESIAN_POINT('Ctrl Pts',(2.90487380426478,-55.1642476808588,13.8634749112255));
#22863=CARTESIAN_POINT('Ctrl Pts',(0.476235235991632,-37.1500000000001,
0.));
#22864=CARTESIAN_POINT('Ctrl Pts',(0.690520950277344,-37.1500000000001,
3.38941559469372));
#22865=CARTESIAN_POINT('Ctrl Pts',(0.904806664563056,-38.6206123116491,
6.44317352589573));
#22866=CARTESIAN_POINT('Ctrl Pts',(1.11909237884877,-40.0912246232982,9.49693145709774));
#22867=CARTESIAN_POINT('Ctrl Pts',(1.33337809313448,-42.7411764423979,11.6101975146502));
#22868=CARTESIAN_POINT('Ctrl Pts',(1.5476638074202,-45.3911282614975,13.7234635722027));
#22869=CARTESIAN_POINT('Ctrl Pts',(1.76194952170592,-48.6955641307488,14.4776794959001));
#22870=CARTESIAN_POINT('Ctrl Pts',(1.97623523599162,-52.,15.2318954195974));
#22871=CARTESIAN_POINT('Ctrl Pts',(2.19052095027735,-55.3044358692514,14.4776794959001));
#22872=CARTESIAN_POINT('Ctrl Pts',(-0.476235235991626,-37.1500000000001,
0.));
#22873=CARTESIAN_POINT('Ctrl Pts',(-0.261949521705911,-37.1500000000001,
3.38941559469374));
#22874=CARTESIAN_POINT('Ctrl Pts',(-0.0476638074202001,-38.6206123116491,
6.44317352589574));
#22875=CARTESIAN_POINT('Ctrl Pts',(0.166621906865511,-40.0912246232982,
9.49693145709774));
#22876=CARTESIAN_POINT('Ctrl Pts',(0.380907621151232,-42.7411764423979,
11.6101975146502));
#22877=CARTESIAN_POINT('Ctrl Pts',(0.595193335436941,-45.3911282614975,
13.7234635722027));
#22878=CARTESIAN_POINT('Ctrl Pts',(0.809479049722664,-48.6955641307488,
14.4776794959001));
#22879=CARTESIAN_POINT('Ctrl Pts',(1.02376476400836,-52.,15.2318954195974));
#22880=CARTESIAN_POINT('Ctrl Pts',(1.23805047829409,-55.3044358692514,14.4776794959001));
#22881=CARTESIAN_POINT('Ctrl Pts',(-1.19058808997907,-37.7800000000001,
0.));
#22882=CARTESIAN_POINT('Ctrl Pts',(-0.976302375693358,-37.7800000000001,
3.24562220582793));
#22883=CARTESIAN_POINT('Ctrl Pts',(-0.762016661407643,-39.1882226984277,
6.16982677025167));
#22884=CARTESIAN_POINT('Ctrl Pts',(-0.547730947121919,-40.5964453968553,
9.09403133467541));
#22885=CARTESIAN_POINT('Ctrl Pts',(-0.333445232836209,-43.1339750175689,
11.1176436806954));
#22886=CARTESIAN_POINT('Ctrl Pts',(-0.119159518550487,-45.6715046382825,
13.1412560267153));
#22887=CARTESIAN_POINT('Ctrl Pts',(0.0951261957352154,-48.8357523191413,
13.8634749112255));
#22888=CARTESIAN_POINT('Ctrl Pts',(0.309411910020934,-52.0000000000001,
14.5856937957357));
#22889=CARTESIAN_POINT('Ctrl Pts',(0.523697624306638,-55.1642476808588,
13.8634749112255));
#22890=CARTESIAN_POINT('',(-1.19058808997887,-37.7800000000033,1.58522090049187E-9));
#22891=CARTESIAN_POINT('Ctrl Pts',(-1.19058808977083,-37.7800000000001,
3.15398724759345E-9));
#22892=CARTESIAN_POINT('Ctrl Pts',(-1.17440993602501,-37.7800000000544,
0.245038153359724));
#22893=CARTESIAN_POINT('Ctrl Pts',(-1.15808907769182,-37.7863378834492,
0.49079116054718));
#22894=CARTESIAN_POINT('Ctrl Pts',(-1.1416567390423,-37.7990994960401,0.736766500751943));
#22895=CARTESIAN_POINT('Ctrl Pts',(-1.12527834683773,-37.8118192129736,
0.981934317728601));
#22896=CARTESIAN_POINT('Ctrl Pts',(-1.10878923236178,-37.8309206530838,
1.22732257379415));
#22897=CARTESIAN_POINT('Ctrl Pts',(-1.09222177854598,-37.8564381709177,
1.47243294819272));
#22898=CARTESIAN_POINT('Ctrl Pts',(-1.07567927587712,-37.8819172585049,
1.71717417806026));
#22899=CARTESIAN_POINT('Ctrl Pts',(-1.05905869844395,-37.9137931614489,
1.96163791544663));
#22900=CARTESIAN_POINT('Ctrl Pts',(-1.04239332675412,-37.9520483461932,
2.20532408781658));
#22901=CARTESIAN_POINT('Ctrl Pts',(-1.02574224814004,-37.990270721333,2.44880126245258));
#22902=CARTESIAN_POINT('Ctrl Pts',(-1.00904648207997,-38.0348614248357,
2.69150175434289));
#22903=CARTESIAN_POINT('Ctrl Pts',(-0.992339825173114,-38.0857510285919,
2.93292951870084));
#22904=CARTESIAN_POINT('Ctrl Pts',(-0.975636663332195,-38.1366299861415,
3.17430677588902));
#22905=CARTESIAN_POINT('Ctrl Pts',(-0.958922645775983,-38.1938051285017,
3.41441139321683));
#22906=CARTESIAN_POINT('Ctrl Pts',(-0.942231694696393,-38.2571558430123,
3.65275710617991));
#22907=CARTESIAN_POINT('Ctrl Pts',(-0.925519549713774,-38.3205869992482,
3.89140546672155));
#22908=CARTESIAN_POINT('Ctrl Pts',(-0.908830560429391,-38.3902092841862,
4.12829002084532));
#22909=CARTESIAN_POINT('Ctrl Pts',(-0.892198465543069,-38.4658518732155,
4.36293874381168));
#22910=CARTESIAN_POINT('Ctrl Pts',(-0.875549399287467,-38.5415716478501,
4.59782690204795));
#22911=CARTESIAN_POINT('Ctrl Pts',(-0.858957373411739,-38.6233238148463,
4.83047425898284));
#22912=CARTESIAN_POINT('Ctrl Pts',(-0.842455462103365,-38.7108897721526,
5.06042975962723));
#22913=CARTESIAN_POINT('Ctrl Pts',(-0.825905305674876,-38.7987117379933,
5.29105756001572));
#22914=CARTESIAN_POINT('Ctrl Pts',(-0.809445820257816,-38.8923812869644,
5.51897736308919));
#22915=CARTESIAN_POINT('Ctrl Pts',(-0.79310915730404,-38.9916337971041,
5.74376259357518));
#22916=CARTESIAN_POINT('Ctrl Pts',(-0.782692415217241,-39.0549201489446,
5.887092340753));
#22917=CARTESIAN_POINT('Ctrl Pts',(-0.772325583322888,-39.1204754951866,
6.02914825316372));
#22918=CARTESIAN_POINT('Ctrl Pts',(-0.762016661407643,-39.1882226984277,
6.16982677025167));
#22919=CARTESIAN_POINT('Ctrl Pts',(-0.74585196858537,-39.2944523060397,
6.39041482340753));
#22920=CARTESIAN_POINT('Ctrl Pts',(-0.729544808776673,-39.406692292665,
6.60890054013437));
#22921=CARTESIAN_POINT('Ctrl Pts',(-0.713126327696533,-39.5248066659344,
6.82480412009635));
#22922=CARTESIAN_POINT('Ctrl Pts',(-0.696744912258959,-39.6426543893767,
7.04022028560845));
#22923=CARTESIAN_POINT('Ctrl Pts',(-0.680252704622003,-39.7663499173029,
7.25306552031141));
#22924=CARTESIAN_POINT('Ctrl Pts',(-0.663682105814804,-39.8957079164889,
7.46287566270863));
#22925=CARTESIAN_POINT('Ctrl Pts',(-0.647138159319839,-40.0248578550113,
7.67234834443288));
#22926=CARTESIAN_POINT('Ctrl Pts',(-0.630516102446333,-40.1596519133109,
7.87879526534386));
#22927=CARTESIAN_POINT('Ctrl Pts',(-0.613849224526778,-40.2998572837037,
8.08177334613496));
#22928=CARTESIAN_POINT('Ctrl Pts',(-0.597198339076355,-40.4399281219983,
8.28455666215324));
#22929=CARTESIAN_POINT('Ctrl Pts',(-0.580502748574263,-40.5853996820896,
8.48387739273973));
#22930=CARTESIAN_POINT('Ctrl Pts',(-0.563796248533928,-40.7359942171173,
8.67931873612112));
#22931=CARTESIAN_POINT('Ctrl Pts',(-0.547088944955135,-40.8865959953438,
8.87476947971412));
#22932=CARTESIAN_POINT('Ctrl Pts',(-0.53037076138362,-41.0423209776528,
9.06634009533642));
#22933=CARTESIAN_POINT('Ctrl Pts',(-0.513675645355332,-41.2028492923188,
9.25364450341684));
#22934=CARTESIAN_POINT('Ctrl Pts',(-0.496974404888472,-41.363436495213,
9.44101762227112));
#22935=CARTESIAN_POINT('Ctrl Pts',(-0.480296279392564,-41.5288302394218,
9.62412107875557));
#22936=CARTESIAN_POINT('Ctrl Pts',(-0.463674941839292,-41.6986725382703,
9.80260437466549));
#22937=CARTESIAN_POINT('Ctrl Pts',(-0.447026491441732,-41.8687918850872,
9.98137881379988));
#22938=CARTESIAN_POINT('Ctrl Pts',(-0.43043504426164,-42.0433739554922,
10.1555177270943));
#22939=CARTESIAN_POINT('Ctrl Pts',(-0.413933671136304,-42.2220261712039,
10.3247095747714));
#22940=CARTESIAN_POINT('Ctrl Pts',(-0.409164215743291,-42.2736627087955,
10.3736117457742));
#22941=CARTESIAN_POINT('Ctrl Pts',(-0.404402278730915,-42.3256390786474,
10.4221009095726));
#22942=CARTESIAN_POINT('Ctrl Pts',(-0.399648641329912,-42.3779453595728,
10.4701702229062));
#22943=CARTESIAN_POINT('',(-4.97404252170606E-6,-37.3300000000069,1.04083408558609E-14));
#22944=CARTESIAN_POINT('Origin',(-1.73472347597681E-15,-39.13,1.04083408558608E-14));
#22945=CARTESIAN_POINT('',(1.19058808997907,-37.78,0.));
#22946=CARTESIAN_POINT('Origin',(-1.73472347597681E-15,-39.13,1.04083408558608E-14));
#22947=CARTESIAN_POINT('Ctrl Pts',(1.19058808997907,-37.78,0.));
#22948=CARTESIAN_POINT('Ctrl Pts',(1.40487380426478,-37.7800000000001,3.24562220582793));
#22949=CARTESIAN_POINT('Ctrl Pts',(1.6191595185505,-39.1882226984277,6.16982677025167));
#22950=CARTESIAN_POINT('Ctrl Pts',(1.79805338220529,-40.3638605623321,8.61106394926976));
#22951=CARTESIAN_POINT('Ctrl Pts',(1.97942721139903,-42.3548619717231,10.4489096280657));
#22952=CARTESIAN_POINT('Ctrl Pts',(3.45,-44.43,0.));
#22953=CARTESIAN_POINT('Ctrl Pts',(3.66428571428572,-44.4300000000001,1.72780310113343));
#22954=CARTESIAN_POINT('Ctrl Pts',(3.87857142857143,-45.1796656699787,3.28449990511991));
#22955=CARTESIAN_POINT('Ctrl Pts',(4.09285714285715,-45.9293313399574,4.84119670910639));
#22956=CARTESIAN_POINT('Ctrl Pts',(4.30714285714286,-47.2801821999294,5.91846432228298));
#22957=CARTESIAN_POINT('Ctrl Pts',(4.52142857142857,-48.6310330599015,6.99573193545956));
#22958=CARTESIAN_POINT('Ctrl Pts',(4.73571428571428,-50.3155165299508,7.38020429521639));
#22959=CARTESIAN_POINT('Ctrl Pts',(4.95,-52.0000000000001,7.76467665497322));
#22960=CARTESIAN_POINT('Ctrl Pts',(5.16428571428571,-53.6844834700494,7.38020429521639));
#22961=CARTESIAN_POINT('Ctrl Pts',(2.26368121662725,-42.3765540157191,0.));
#22962=CARTESIAN_POINT('Ctrl Pts',(2.47796693091296,-42.3765540157191,2.19648874705823));
#22963=CARTESIAN_POINT('Ctrl Pts',(2.69225264519868,-43.3295747662224,4.17545672685567));
#22964=CARTESIAN_POINT('Ctrl Pts',(2.90653835948438,-44.2825955167256,6.15442470665314));
#22965=CARTESIAN_POINT('Ctrl Pts',(3.12082407377011,-45.9998795700625,7.5239130403414));
#22966=CARTESIAN_POINT('Ctrl Pts',(3.33510978805582,-47.7171636233994,8.89340137402968));
#22967=CARTESIAN_POINT('Ctrl Pts',(3.54939550234153,-49.8585818116997,9.38216610144961));
#22968=CARTESIAN_POINT('Ctrl Pts',(3.76368121662725,-52.0000000000001,9.87093082886953));
#22969=CARTESIAN_POINT('Ctrl Pts',(3.97796693091296,-54.1414181883004,9.3821661014496));
#22970=CARTESIAN_POINT('Ctrl Pts',(1.50077089879006,-40.1311229851416,0.));
#22971=CARTESIAN_POINT('Ctrl Pts',(1.71505661307578,-40.1311229851416,2.70899372698069));
#22972=CARTESIAN_POINT('Ctrl Pts',(1.92934232736149,-41.30651131265,5.14971273833323));
#22973=CARTESIAN_POINT('Ctrl Pts',(2.1436280416472,-42.4818996401584,7.59043174968577));
#22974=CARTESIAN_POINT('Ctrl Pts',(2.35791375593292,-44.5998762217203,9.27946171175751));
#22975=CARTESIAN_POINT('Ctrl Pts',(2.57219947021862,-46.7178528032822,10.9684916738293));
#22976=CARTESIAN_POINT('Ctrl Pts',(2.78648518450434,-49.3589264016411,11.5712994880388));
#22977=CARTESIAN_POINT('Ctrl Pts',(3.00077089879007,-52.0000000000001,12.1741073022483));
#22978=CARTESIAN_POINT('Ctrl Pts',(3.21505661307576,-54.641073598359,11.5712994880388));
#22979=CARTESIAN_POINT('Ctrl Pts',(1.19058808997907,-37.78,0.));
#22980=CARTESIAN_POINT('Ctrl Pts',(1.40487380426479,-37.7800000000001,3.24562220582793));
#22981=CARTESIAN_POINT('Ctrl Pts',(1.6191595185505,-39.1882226984276,6.16982677025167));
#22982=CARTESIAN_POINT('Ctrl Pts',(1.83344523283622,-40.5964453968553,9.09403133467541));
#22983=CARTESIAN_POINT('Ctrl Pts',(2.04773094712193,-43.1339750175689,11.1176436806954));
#22984=CARTESIAN_POINT('Ctrl Pts',(2.26201666140765,-45.6715046382825,13.1412560267153));
#22985=CARTESIAN_POINT('Ctrl Pts',(2.47630237569336,-48.8357523191413,13.8634749112255));
#22986=CARTESIAN_POINT('Ctrl Pts',(2.69058808997906,-52.0000000000001,14.5856937957357));
#22987=CARTESIAN_POINT('Ctrl Pts',(2.90487380426478,-55.1642476808588,13.8634749112255));
#22988=CARTESIAN_POINT('Origin',(19.0359549110502,-35.425667181256,0.));
#22989=CARTESIAN_POINT('Ctrl Pts',(-1.19058808997907,-37.7800000000001,
0.));
#22990=CARTESIAN_POINT('Ctrl Pts',(-0.976302375693358,-37.7800000000001,
3.24562220582793));
#22991=CARTESIAN_POINT('Ctrl Pts',(-0.762016661407643,-39.1882226984276,
6.16982677025168));
#22992=CARTESIAN_POINT('Ctrl Pts',(-0.547730947121923,-40.5964453968553,
9.09403133467541));
#22993=CARTESIAN_POINT('Ctrl Pts',(-0.333445232836209,-43.1339750175689,
11.1176436806954));
#22994=CARTESIAN_POINT('Ctrl Pts',(-0.119159518550493,-45.6715046382825,
13.1412560267153));
#22995=CARTESIAN_POINT('Ctrl Pts',(0.0951261957352102,-48.8357523191413,
13.8634749112255));
#22996=CARTESIAN_POINT('Ctrl Pts',(0.309411910020934,-52.0000000000001,
14.5856937957357));
#22997=CARTESIAN_POINT('Ctrl Pts',(0.523697624306634,-55.1642476808588,
13.8634749112255));
#22998=CARTESIAN_POINT('Ctrl Pts',(-1.50077089879006,-40.1311229851416,
0.));
#22999=CARTESIAN_POINT('Ctrl Pts',(-1.28648518450434,-40.1311229851416,
2.70899372698069));
#23000=CARTESIAN_POINT('Ctrl Pts',(-1.07219947021864,-41.3065113126499,
5.14971273833323));
#23001=CARTESIAN_POINT('Ctrl Pts',(-0.857913755932923,-42.4818996401584,
7.59043174968577));
#23002=CARTESIAN_POINT('Ctrl Pts',(-0.643628041647201,-44.5998762217203,
9.27946171175751));
#23003=CARTESIAN_POINT('Ctrl Pts',(-0.429342327361493,-46.7178528032822,
10.9684916738293));
#23004=CARTESIAN_POINT('Ctrl Pts',(-0.215056613075784,-49.3589264016411,
11.5712994880388));
#23005=CARTESIAN_POINT('Ctrl Pts',(-0.000770898790054586,-52.0000000000001,
12.1741073022483));
#23006=CARTESIAN_POINT('Ctrl Pts',(0.213514815495646,-54.641073598359,11.5712994880388));
#23007=CARTESIAN_POINT('Ctrl Pts',(-2.26368121662725,-42.3765540157191,
0.));
#23008=CARTESIAN_POINT('Ctrl Pts',(-2.04939550234155,-42.3765540157191,
2.19648874705823));
#23009=CARTESIAN_POINT('Ctrl Pts',(-1.83510978805583,-43.3295747662223,
4.17545672685568));
#23010=CARTESIAN_POINT('Ctrl Pts',(-1.62082407377013,-44.2825955167256,
6.15442470665313));
#23011=CARTESIAN_POINT('Ctrl Pts',(-1.4065383594844,-45.9998795700625,7.5239130403414));
#23012=CARTESIAN_POINT('Ctrl Pts',(-1.19225264519869,-47.7171636233994,
8.89340137402967));
#23013=CARTESIAN_POINT('Ctrl Pts',(-0.977966930912963,-49.8585818116997,
9.3821661014496));
#23014=CARTESIAN_POINT('Ctrl Pts',(-0.763681216627249,-52.0000000000001,
9.87093082886953));
#23015=CARTESIAN_POINT('Ctrl Pts',(-0.549395502341532,-54.1414181883004,
9.3821661014496));
#23016=CARTESIAN_POINT('Ctrl Pts',(-3.45,-44.4300000000001,0.));
#23017=CARTESIAN_POINT('Ctrl Pts',(-3.23571428571428,-44.4300000000001,
1.72780310113343));
#23018=CARTESIAN_POINT('Ctrl Pts',(-3.02142857142857,-45.1796656699788,
3.28449990511991));
#23019=CARTESIAN_POINT('Ctrl Pts',(-2.80714285714286,-45.9293313399574,
4.84119670910638));
#23020=CARTESIAN_POINT('Ctrl Pts',(-2.59285714285715,-47.2801821999294,
5.91846432228297));
#23021=CARTESIAN_POINT('Ctrl Pts',(-2.37857142857143,-48.6310330599014,
6.99573193545956));
#23022=CARTESIAN_POINT('Ctrl Pts',(-2.16428571428571,-50.3155165299508,
7.38020429521639));
#23023=CARTESIAN_POINT('Ctrl Pts',(-1.95000000000001,-52.0000000000001,
7.76467665497322));
#23024=CARTESIAN_POINT('Ctrl Pts',(-1.73571428571428,-53.6844834700494,
7.38020429521639));
#23025=CARTESIAN_POINT('Origin',(-19.0359549110502,-35.425667181256,0.));
#23026=CARTESIAN_POINT('Ctrl Pts',(1.06226042837001,-37.8397258902528,1.59647049649061));
#23027=CARTESIAN_POINT('Ctrl Pts',(1.10262802813221,-37.8163671782172,1.15259151032668));
#23028=CARTESIAN_POINT('Ctrl Pts',(1.14747953738505,-37.7797757625757,0.635572917996464));
#23029=CARTESIAN_POINT('Ctrl Pts',(1.31732736909556,-37.7806592587273,-1.86858636177033));
#23030=CARTESIAN_POINT('Ctrl Pts',(1.43803115336731,-38.1455252315354,-3.71029995869598));
#23031=CARTESIAN_POINT('Ctrl Pts',(1.69365713820689,-39.5779229780087,-7.16936247493924));
#23032=CARTESIAN_POINT('Ctrl Pts',(1.81514228728894,-40.6266263701707,-8.73699595770183));
#23033=CARTESIAN_POINT('Ctrl Pts',(2.0664373721633,-43.2633442117449,-11.373025698218));
#23034=CARTESIAN_POINT('Ctrl Pts',(2.18792249430893,-44.8298904725309,-12.4235805192224));
#23035=CARTESIAN_POINT('Ctrl Pts',(2.44354852690307,-48.2902066278842,-13.85294708216));
#23036=CARTESIAN_POINT('Ctrl Pts',(2.56492073910889,-50.1387215498278,-14.2204718556691));
#23037=CARTESIAN_POINT('Ctrl Pts',(2.69099156569462,-51.9999633056261,-14.2198708430667));
#23038=CARTESIAN_POINT('Ctrl Pts',(0.347755560296868,-37.2107726459064,
1.62964593809825));
#23039=CARTESIAN_POINT('Ctrl Pts',(0.387786383581994,-37.1876088095763,
1.18947011987008));
#23040=CARTESIAN_POINT('Ctrl Pts',(0.433007907800631,-37.1499104513489,
0.664243870396088));
#23041=CARTESIAN_POINT('Ctrl Pts',(0.603323715733815,-37.150263273314,-1.95287905127288));
#23042=CARTESIAN_POINT('Ctrl Pts',(0.72328369871309,-37.5316956084199,-3.87337387078179));
#23043=CARTESIAN_POINT('Ctrl Pts',(0.979785618814997,-39.027330971542,-7.48792130214399));
#23044=CARTESIAN_POINT('Ctrl Pts',(1.10069469072639,-40.1224384633822,-9.12360836231754));
#23045=CARTESIAN_POINT('Ctrl Pts',(1.35224759480683,-42.8765051571252,-11.8774049927137));
#23046=CARTESIAN_POINT('Ctrl Pts',(1.47315665468806,-44.5117551326448,-12.9732563608769));
#23047=CARTESIAN_POINT('Ctrl Pts',(1.72965859378933,-48.126801308994,-14.4676858045579));
#23048=CARTESIAN_POINT('Ctrl Pts',(1.85032539219322,-50.0548871962143,-14.8501851005342));
#23049=CARTESIAN_POINT('Ctrl Pts',(1.97670704765982,-51.9999570907663,-14.8499483202528));
#23050=CARTESIAN_POINT('Ctrl Pts',(-0.604714876209436,-37.2110085708708,
1.62975512103804));
#23051=CARTESIAN_POINT('Ctrl Pts',(-0.564689496472769,-37.1878478844499,
1.18963915964465));
#23052=CARTESIAN_POINT('Ctrl Pts',(-0.519462564176609,-37.1500900231906,
0.664246312466032));
#23053=CARTESIAN_POINT('Ctrl Pts',(-0.34914675626714,-37.1497353315388,
-1.95288623096613));
#23054=CARTESIAN_POINT('Ctrl Pts',(-0.229186815972883,-37.5322524147635,
-3.87317034518711));
#23055=CARTESIAN_POINT('Ctrl Pts',(0.0273151950961837,-39.0266771563425,
-7.48823335804281));
#23056=CARTESIAN_POINT('Ctrl Pts',(0.148224209656984,-40.1225272605589,
-9.12349227713643));
#23057=CARTESIAN_POINT('Ctrl Pts',(0.399777134874542,-42.8763256602578,
-11.8775764776329));
#23058=CARTESIAN_POINT('Ctrl Pts',(0.520686157648162,-44.5120149889529,
-12.9726927515284));
#23059=CARTESIAN_POINT('Ctrl Pts',(0.777188149407483,-48.1265710168792,
-14.4683433355078));
#23060=CARTESIAN_POINT('Ctrl Pts',(0.897861662853934,-50.0549848089201,
-14.8498038985528));
#23061=CARTESIAN_POINT('Ctrl Pts',(1.02423658127911,-51.9999570902567,-14.8500516281495));
#23062=CARTESIAN_POINT('Ctrl Pts',(-1.31891566289573,-37.8403157026637,
1.59674345384007));
#23063=CARTESIAN_POINT('Ctrl Pts',(-1.27856167200511,-37.816964865386,1.15301410976404));
#23064=CARTESIAN_POINT('Ctrl Pts',(-1.23369664255802,-37.7802246921786,
0.635579023171327));
#23065=CARTESIAN_POINT('Ctrl Pts',(-1.06384881090689,-37.7793394042942,
-1.86860431100347));
#23066=CARTESIAN_POINT('Ctrl Pts',(-0.943145133347884,-38.1469172473993,
-3.70979114470452));
#23067=CARTESIAN_POINT('Ctrl Pts',(-0.687518921089859,-39.5762884400051,
-7.17014261469109));
#23068=CARTESIAN_POINT('Ctrl Pts',(-0.566033915384881,-40.6268483631173,
-8.73670574474909));
#23069=CARTESIAN_POINT('Ctrl Pts',(-0.314738777667137,-43.2628954695717,
-11.373454410516));
#23070=CARTESIAN_POINT('Ctrl Pts',(-0.193253748290483,-44.8305401132962,
-12.4221714958367));
#23071=CARTESIAN_POINT('Ctrl Pts',(0.0623724159481351,-48.2896308976019,
-13.8545909095489));
#23072=CARTESIAN_POINT('Ctrl Pts',(0.183762141934924,-50.1389656602283,
-14.2195188100007));
#23073=CARTESIAN_POINT('Ctrl Pts',(0.309815399742843,-51.9999633043522,
-14.2201291128083));
#23074=CARTESIAN_POINT('Ctrl Pts',(1.19058808997907,-37.78,0.));
#23075=CARTESIAN_POINT('Ctrl Pts',(1.31732736909556,-37.7806592587273,-1.86858636177033));
#23076=CARTESIAN_POINT('Ctrl Pts',(1.43803115336731,-38.1455252315354,-3.71029995869598));
#23077=CARTESIAN_POINT('Ctrl Pts',(1.69365713820689,-39.5779229780087,-7.16936247493924));
#23078=CARTESIAN_POINT('Ctrl Pts',(1.81514228728894,-40.6266263701707,-8.73699595770183));
#23079=CARTESIAN_POINT('Ctrl Pts',(1.95357130555244,-42.0790951378326,-10.1890856763505));
#23080=CARTESIAN_POINT('Ctrl Pts',(1.96630970889272,-42.2157732130427,-10.3203928635177));
#23081=CARTESIAN_POINT('Ctrl Pts',(1.97901608230067,-42.3549304887752,-10.4488603766009));
#23082=CARTESIAN_POINT('Ctrl Pts',(-1.19058808997907,-37.7800000000001,
2.1094237467878E-15));
#23083=CARTESIAN_POINT('Ctrl Pts',(-1.06384881090689,-37.7793394042942,
-1.86860431100347));
#23084=CARTESIAN_POINT('Ctrl Pts',(-0.943145133347884,-38.1469172473993,
-3.70979114470452));
#23085=CARTESIAN_POINT('Ctrl Pts',(-0.687518921089859,-39.5762884400051,
-7.17014261469109));
#23086=CARTESIAN_POINT('Ctrl Pts',(-0.566033915384881,-40.6268483631173,
-8.73670574474909));
#23087=CARTESIAN_POINT('Ctrl Pts',(-0.42689829031798,-42.0863595386748,
-10.1966053555719));
#23088=CARTESIAN_POINT('Ctrl Pts',(-0.41345820181274,-42.2307237103642,
-10.3350231942276));
#23089=CARTESIAN_POINT('Ctrl Pts',(-0.400053103665672,-42.3778559173188,
-10.4702558451));
#23090=CARTESIAN_POINT('Ctrl Pts',(3.32327712822012,-44.4799848904464,1.24689064510955));
#23091=CARTESIAN_POINT('Ctrl Pts',(3.36716940899972,-44.4545866217131,0.764254540719014));
#23092=CARTESIAN_POINT('Ctrl Pts',(3.40814518985255,-44.429349685102,0.332948627185772));
#23093=CARTESIAN_POINT('Ctrl Pts',(3.57305327241219,-44.4319119278293,-0.978870002659466));
#23094=CARTESIAN_POINT('Ctrl Pts',(3.70160805588082,-44.6279251367563,-1.98783577088437));
#23095=CARTESIAN_POINT('Ctrl Pts',(3.94798856176874,-45.3861024076399,-3.80852727284065));
#23096=CARTESIAN_POINT('Ctrl Pts',(4.07555420744412,-45.9491021672716,-4.65544360722303));
#23097=CARTESIAN_POINT('Ctrl Pts',(4.32412798456521,-47.3456501222045,-6.04997283343043));
#23098=CARTESIAN_POINT('Ctrl Pts',(4.45169355820317,-48.1894265020396,-6.618321698991));
#23099=CARTESIAN_POINT('Ctrl Pts',(4.69807420295718,-50.013763693226,-7.36768403082578));
#23100=CARTESIAN_POINT('Ctrl Pts',(4.82686758916904,-51.0241709100527,-7.57138648682318));
#23101=CARTESIAN_POINT('Ctrl Pts',(4.94968218283415,-52.0000289040989,-7.56962581969448));
#23102=CARTESIAN_POINT('Ctrl Pts',(2.13646282181016,-42.4296678529921,1.35489302548968));
#23103=CARTESIAN_POINT('Ctrl Pts',(2.17926392766628,-42.4049009926309,0.884255395658553));
#23104=CARTESIAN_POINT('Ctrl Pts',(2.22143926476967,-42.3761273929605,0.426396892757904));
#23105=CARTESIAN_POINT('Ctrl Pts',(2.38787268687497,-42.3778082879602,-1.25360819498149));
#23106=CARTESIAN_POINT('Ctrl Pts',(2.5140031472761,-42.6265178497758,-2.51960912779656));
#23107=CARTESIAN_POINT('Ctrl Pts',(2.76323860082846,-43.5922658248206,-4.8464758678243));
#23108=CARTESIAN_POINT('Ctrl Pts',(2.8889266274111,-44.3056264360906,-5.91572199046689));
#23109=CARTESIAN_POINT('Ctrl Pts',(3.13834072492096,-46.0849874081721,-7.69376028692028));
#23110=CARTESIAN_POINT('Ctrl Pts',(3.26402870377777,-47.1521724801729,-8.41063186554706));
#23111=CARTESIAN_POINT('Ctrl Pts',(3.51326424840899,-49.4814303102184,-9.37059840621927));
#23112=CARTESIAN_POINT('Ctrl Pts',(3.63979023544684,-50.7508064960244,-9.62435378625662));
#23113=CARTESIAN_POINT('Ctrl Pts',(3.76358612954926,-52.0000086477592,-9.62320046360554));
#23114=CARTESIAN_POINT('Ctrl Pts',(1.37301063256244,-40.1875259567355,1.47293173916723));
#23115=CARTESIAN_POINT('Ctrl Pts',(1.41462159884989,-40.1634477706497,1.01538079142922));
#23116=CARTESIAN_POINT('Ctrl Pts',(1.45810560976048,-40.1308402311943,0.52858064812525));
#23117=CARTESIAN_POINT('Ctrl Pts',(1.62620698164419,-40.1319542826288,-1.55402875455442));
#23118=CARTESIAN_POINT('Ctrl Pts',(1.74968648306502,-40.4376784663506,-3.10121432123458));
#23119=CARTESIAN_POINT('Ctrl Pts',(2.00204375396077,-41.6310829191854,-5.98129145450958));
#23120=CARTESIAN_POINT('Ctrl Pts',(2.12567864735027,-42.5084456369459,-7.29389406576053));
#23121=CARTESIAN_POINT('Ctrl Pts',(2.3760116183751,-44.7065608867208,-9.49113593804617));
#23122=CARTESIAN_POINT('Ctrl Pts',(2.49964647926793,-46.0177955705498,-10.3708286017073));
#23123=CARTESIAN_POINT('Ctrl Pts',(2.75200381047715,-48.8994560970608,-11.5604045561349));
#23124=CARTESIAN_POINT('Ctrl Pts',(2.87602039417755,-50.4518266808844,-11.8694761541618));
#23125=CARTESIAN_POINT('Ctrl Pts',(3.000919362602,-51.9999864978575,-11.8687142284813));
#23126=CARTESIAN_POINT('Ctrl Pts',(1.06226042837001,-37.8397258902528,1.59647049649061));
#23127=CARTESIAN_POINT('Ctrl Pts',(1.10262802813221,-37.8163671782172,1.15259151032668));
#23128=CARTESIAN_POINT('Ctrl Pts',(1.14747953738505,-37.7797757625757,0.635572917996464));
#23129=CARTESIAN_POINT('Ctrl Pts',(1.31732736909556,-37.7806592587273,-1.86858636177033));
#23130=CARTESIAN_POINT('Ctrl Pts',(1.43803115336731,-38.1455252315354,-3.71029995869598));
#23131=CARTESIAN_POINT('Ctrl Pts',(1.69365713820689,-39.5779229780087,-7.16936247493924));
#23132=CARTESIAN_POINT('Ctrl Pts',(1.81514228728894,-40.6266263701707,-8.73699595770183));
#23133=CARTESIAN_POINT('Ctrl Pts',(2.0664373721633,-43.2633442117449,-11.373025698218));
#23134=CARTESIAN_POINT('Ctrl Pts',(2.18792249430953,-44.8298904725309,-12.4235805192224));
#23135=CARTESIAN_POINT('Ctrl Pts',(2.44354852690246,-48.2902066278842,-13.85294708216));
#23136=CARTESIAN_POINT('Ctrl Pts',(2.56492073910889,-50.1387215498278,-14.2204718556691));
#23137=CARTESIAN_POINT('Ctrl Pts',(2.69099156569462,-51.9999633056261,-14.2198708430667));
#23138=CARTESIAN_POINT('Ctrl Pts',(-1.31891566289574,-37.8403157026637,
1.59674345384007));
#23139=CARTESIAN_POINT('Ctrl Pts',(-1.27856167200496,-37.816964865386,1.15301410976406));
#23140=CARTESIAN_POINT('Ctrl Pts',(-1.23369664255802,-37.7802246921786,
0.635579023171327));
#23141=CARTESIAN_POINT('Ctrl Pts',(-1.06384881090689,-37.7793394042942,
-1.86860431100347));
#23142=CARTESIAN_POINT('Ctrl Pts',(-0.943145133347888,-38.1469172473993,
-3.70979114470452));
#23143=CARTESIAN_POINT('Ctrl Pts',(-0.687518921089859,-39.5762884400051,
-7.17014261469109));
#23144=CARTESIAN_POINT('Ctrl Pts',(-0.566033915384886,-40.6268483631173,
-8.73670574475149));
#23145=CARTESIAN_POINT('Ctrl Pts',(-0.314738777667137,-43.2628954695717,
-11.3734544105136));
#23146=CARTESIAN_POINT('Ctrl Pts',(-0.193253748290479,-44.830540113301,
-12.4221714958367));
#23147=CARTESIAN_POINT('Ctrl Pts',(0.0623724159481334,-48.2896308975971,
-13.8545909095489));
#23148=CARTESIAN_POINT('Ctrl Pts',(0.183762141935159,-50.1389656602319,
-14.2195188100007));
#23149=CARTESIAN_POINT('Ctrl Pts',(0.309815399742839,-51.9999633043522,
-14.2201291128083));
#23150=CARTESIAN_POINT('Ctrl Pts',(-1.62853105321834,-40.1882694324258,
1.47327580984132));
#23151=CARTESIAN_POINT('Ctrl Pts',(-1.58693724130863,-40.1642011727047,
1.01591349030511));
#23152=CARTESIAN_POINT('Ctrl Pts',(-1.54343618780062,-40.1314061200099,
0.528588343875644));
#23153=CARTESIAN_POINT('Ctrl Pts',(-1.37533481599184,-40.1302905677455,
-1.55405138008459));
#23154=CARTESIAN_POINT('Ctrl Pts',(-1.25185544908537,-40.4394331428107,
-3.10057294640679));
#23155=CARTESIAN_POINT('Ctrl Pts',(-0.99949789152226,-41.6290225365179,
-5.982274843346));
#23156=CARTESIAN_POINT('Ctrl Pts',(-0.875863178863688,-42.5087254655101,
-7.29352824389351));
#23157=CARTESIAN_POINT('Ctrl Pts',(-0.625530141228115,-44.7059952341645,
-9.49167634236414));
#23158=CARTESIAN_POINT('Ctrl Pts',(-0.501895397273558,-46.0186144616128,
-10.369052486768));
#23159=CARTESIAN_POINT('Ctrl Pts',(-0.249537900122174,-48.8987303723102,
-11.5624766483463));
#23160=CARTESIAN_POINT('Ctrl Pts',(-0.125494944833563,-50.4521347865941,
-11.8682745705925));
#23161=CARTESIAN_POINT('Ctrl Pts',(-0.000622417322686238,-51.9999864962518,
-11.8690397849987));
#23162=CARTESIAN_POINT('Ctrl Pts',(-2.39089944281231,-42.4307892712954,
1.35541200298501));
#23163=CARTESIAN_POINT('Ctrl Pts',(-2.34812421168709,-42.4060373833274,
0.885058889676134));
#23164=CARTESIAN_POINT('Ctrl Pts',(-2.30592316845611,-42.3769809488797,
0.426408500609331));
#23165=CARTESIAN_POINT('Ctrl Pts',(-2.13948974646398,-42.3752988308948,
-1.2536423221009));
#23166=CARTESIAN_POINT('Ctrl Pts',(-2.01335948895663,-42.6291645083452,
-2.51864171288184));
#23167=CARTESIAN_POINT('Ctrl Pts',(-1.76412360301132,-43.5891580556313,
-4.84795915807201));
#23168=CARTESIAN_POINT('Ctrl Pts',(-1.63843584903307,-44.306048514286,-5.915170204659));
#23169=CARTESIAN_POINT('Ctrl Pts',(-1.38902165105132,-46.0841342086093,
-7.69457540340395));
#23170=CARTESIAN_POINT('Ctrl Pts',(-1.26333384857794,-47.1534076509294,
-8.40795287035375));
#23171=CARTESIAN_POINT('Ctrl Pts',(-1.01409805364826,-49.4803356664615,
-9.37372383743554));
#23172=CARTESIAN_POINT('Ctrl Pts',(-0.887523067773768,-50.7512717901712,
-9.62254086006318));
#23173=CARTESIAN_POINT('Ctrl Pts',(-0.763776277074748,-52.0000086453373,
-9.62369151535372));
#23174=CARTESIAN_POINT('Ctrl Pts',(-3.5767226147735,-44.4816940061638,1.2476816011619));
#23175=CARTESIAN_POINT('Ctrl Pts',(-3.53286976879601,-44.4563185563517,
0.765479118782407));
#23176=CARTESIAN_POINT('Ctrl Pts',(-3.49185481010397,-44.4306505608144,
0.332966318319628));
#23177=CARTESIAN_POINT('Ctrl Pts',(-3.32694672771567,-44.4280873491762,
-0.978922014648203));
#23178=CARTESIAN_POINT('Ctrl Pts',(-3.19839225347182,-44.6319588195941,
-1.98636136652616));
#23179=CARTESIAN_POINT('Ctrl Pts',(-2.95201108858767,-45.381365961698,-3.81078790535049));
#23180=CARTESIAN_POINT('Ctrl Pts',(-2.82444585837899,-45.9497454423789,
-4.65460264912874));
#23181=CARTESIAN_POINT('Ctrl Pts',(-2.5758719281337,-47.3443497895988,-6.05121512490362));
#23182=CARTESIAN_POINT('Ctrl Pts',(-2.44830662331528,-48.1913089840266,
-6.61423873300174));
#23183=CARTESIAN_POINT('Ctrl Pts',(-2.20192559708918,-50.0120953836876,
-7.37244739486218));
#23184=CARTESIAN_POINT('Ctrl Pts',(-2.07303718495312,-51.024880382195,-7.56862230180471));
#23185=CARTESIAN_POINT('Ctrl Pts',(-1.95031777657922,-52.0000289004077,
-7.57037421505985));
#23186=CARTESIAN_POINT('Ctrl Pts',(-6.55512420987408,-37.2260157227862,
0.));
#23187=CARTESIAN_POINT('Ctrl Pts',(-6.34301961518532,-37.2565117595591,
3.24562220582792));
#23188=CARTESIAN_POINT('Ctrl Pts',(-6.33132600607604,-38.680896818179,6.16982677025167));
#23189=CARTESIAN_POINT('Ctrl Pts',(-6.31963239696676,-40.1052818767989,
9.09403133467541));
#23190=CARTESIAN_POINT('Ctrl Pts',(-6.46865591986352,-42.6474791415621,
11.1176436806954));
#23191=CARTESIAN_POINT('Ctrl Pts',(-6.61767944276027,-45.1896764063252,
13.1412560267153));
#23192=CARTESIAN_POINT('Ctrl Pts',(-6.85589424502954,-48.3522126450341,
13.8634749112255));
#23193=CARTESIAN_POINT('Ctrl Pts',(-7.09410904729881,-51.514748883743,14.5856937957357));
#23194=CARTESIAN_POINT('Ctrl Pts',(-7.33232384956808,-54.6772851224519,
13.8634749112255));
#23195=CARTESIAN_POINT('Ctrl Pts',(-7.19674949232908,-39.5090640497073,
0.));
#23196=CARTESIAN_POINT('Ctrl Pts',(-6.9846448976403,-39.5395600864802,2.70899372698068));
#23197=CARTESIAN_POINT('Ctrl Pts',(-6.93981550268921,-40.7334806923574,
5.14971273833322));
#23198=CARTESIAN_POINT('Ctrl Pts',(-6.89498610773809,-41.9274012982346,
7.59043174968578));
#23199=CARTESIAN_POINT('Ctrl Pts',(-6.9843010077209,-44.0543159688391,9.2794617117575));
#23200=CARTESIAN_POINT('Ctrl Pts',(-7.07361590770374,-46.1812306394436,
10.9684916738292));
#23201=CARTESIAN_POINT('Ctrl Pts',(-7.23737527503327,-48.8259179534578,
11.5712994880388));
#23202=CARTESIAN_POINT('Ctrl Pts',(-7.40113464236278,-51.4706052674719,
12.1741073022483));
#23203=CARTESIAN_POINT('Ctrl Pts',(-7.56489400969232,-54.1152925814861,
11.5712994880388));
#23204=CARTESIAN_POINT('Ctrl Pts',(-8.27145263712698,-41.6230663715377,
0.));
#23205=CARTESIAN_POINT('Ctrl Pts',(-8.05934804243821,-41.6535624083105,
2.19648874705823));
#23206=CARTESIAN_POINT('Ctrl Pts',(-7.98287244172838,-42.627378818489,4.17545672685568));
#23207=CARTESIAN_POINT('Ctrl Pts',(-7.90639684101858,-43.6011952286675,
6.15442470665313));
#23208=CARTESIAN_POINT('Ctrl Pts',(-7.93868724864975,-45.3314958432333,
7.5239130403414));
#23209=CARTESIAN_POINT('Ctrl Pts',(-7.9709776562809,-47.0617964577992,8.89340137402966));
#23210=CARTESIAN_POINT('Ctrl Pts',(-8.06362864473556,-49.2119141333855,
9.3821661014496));
#23211=CARTESIAN_POINT('Ctrl Pts',(-8.15627963319022,-51.3620318089719,
9.87093082886953));
#23212=CARTESIAN_POINT('Ctrl Pts',(-8.24893062164489,-53.5121494845583,
9.3821661014496));
#23213=CARTESIAN_POINT('Ctrl Pts',(-9.7379322389713,-43.4867804707271,0.));
#23214=CARTESIAN_POINT('Ctrl Pts',(-9.52582764428252,-43.5172765074999,
1.72780310113342));
#23215=CARTESIAN_POINT('Ctrl Pts',(-9.42041159817581,-44.2898076986597,
3.28449990511991));
#23216=CARTESIAN_POINT('Ctrl Pts',(-9.31499555206908,-45.0623388898195,
4.84119670910639));
#23217=CARTESIAN_POINT('Ctrl Pts',(-9.29513707904857,-46.4299360725759,
5.91846432228297));
#23218=CARTESIAN_POINT('Ctrl Pts',(-9.27527860602804,-47.7975332553324,
6.99573193545956));
#23219=CARTESIAN_POINT('Ctrl Pts',(-9.30290100395336,-49.495367149254,7.38020429521638));
#23220=CARTESIAN_POINT('Ctrl Pts',(-9.33052340187867,-51.1932010431757,
7.76467665497321));
#23221=CARTESIAN_POINT('Ctrl Pts',(-9.35814579980399,-52.8910349370973,
7.38020429521638));
#23222=CARTESIAN_POINT('',(-6.55512420988052,-37.22601572281,1.57948858047412E-9));
#23223=CARTESIAN_POINT('Origin',(-23.8837944332598,-32.3559861244012,0.));
#23224=CARTESIAN_POINT('Ctrl Pts',(-6.55512420969261,-37.226015722898,3.13104709159877E-9));
#23225=CARTESIAN_POINT('Ctrl Pts',(-6.53911072623215,-37.2283181142836,
0.245038153335359));
#23226=CARTESIAN_POINT('Ctrl Pts',(-6.52385796555383,-37.2369141874759,
0.490791160521495));
#23227=CARTESIAN_POINT('Ctrl Pts',(-6.50940905124972,-37.2518844708665,
0.736766500725045));
#23228=CARTESIAN_POINT('Ctrl Pts',(-6.49500757191982,-37.2668056076575,
0.981934317700707));
#23229=CARTESIAN_POINT('Ctrl Pts',(-6.48140471121339,-37.2880592683071,
1.22732257376537));
#23230=CARTESIAN_POINT('Ctrl Pts',(-6.46863741161224,-37.3156748491109,
1.47243294816315));
#23231=CARTESIAN_POINT('Ctrl Pts',(-6.45588933999698,-37.343248839914,1.71717417802991));
#23232=CARTESIAN_POINT('Ctrl Pts',(-6.44397435004891,-37.3771656469145,
1.96163791541559));
#23233=CARTESIAN_POINT('Ctrl Pts',(-6.43292288824284,-37.4174031787122,
2.20532408778497));
#23234=CARTESIAN_POINT('Ctrl Pts',(-6.42188090473605,-37.457606200743,2.44880126242042));
#23235=CARTESIAN_POINT('Ctrl Pts',(-6.41170099625808,-37.5041190904231,
2.69150175431029));
#23236=CARTESIAN_POINT('Ctrl Pts',(-6.4024067347573,-37.5568683165634,2.93292951866791));
#23237=CARTESIAN_POINT('Ctrl Pts',(-6.39311441763456,-37.6096065074603,
3.17430677585578));
#23238=CARTESIAN_POINT('Ctrl Pts',(-6.38470739581513,-37.6685783420143,
3.41441139318338));
#23239=CARTESIAN_POINT('Ctrl Pts',(-6.37720208124067,-37.7336596075968,
3.65275710614636));
#23240=CARTESIAN_POINT('Ctrl Pts',(-6.36968723653768,-37.7988235123306,
3.89140546668784));
#23241=CARTESIAN_POINT('Ctrl Pts',(-6.36307640132128,-37.8701122336038,
4.12829002081156));
#23242=CARTESIAN_POINT('Ctrl Pts',(-6.35737866000311,-37.9473518840361,
4.36293874377797));
#23243=CARTESIAN_POINT('Ctrl Pts',(-6.35167510471667,-38.0246703497133,
4.59782690201429));
#23244=CARTESIAN_POINT('Ctrl Pts',(-6.34688650816463,-38.1079516890034,
4.83047425894932));
#23245=CARTESIAN_POINT('Ctrl Pts',(-6.34301449757132,-38.196974817961,5.06042975959396));
#23246=CARTESIAN_POINT('Ctrl Pts',(-6.33913116673682,-38.2862582156518,
5.29105755998276));
#23247=CARTESIAN_POINT('Ctrl Pts',(-6.33616978186108,-38.3813167726778,
5.51897736305666));
#23248=CARTESIAN_POINT('Ctrl Pts',(-6.33412450750884,-38.4818839849188,
5.74376259354316));
#23249=CARTESIAN_POINT('Ctrl Pts',(-6.33282037976348,-38.5460086299152,
5.88709234072609));
#23250=CARTESIAN_POINT('Ctrl Pts',(-6.33188856576809,-38.612372071261,6.02914825314187));
#23251=CARTESIAN_POINT('Ctrl Pts',(-6.33132600608609,-38.6808968182129,
6.16982677023484));
#23252=CARTESIAN_POINT('Ctrl Pts',(-6.33044389595582,-38.7883456372328,
6.39041482339097));
#23253=CARTESIAN_POINT('Ctrl Pts',(-6.33027613506487,-38.9017639334401,
6.60890054011818));
#23254=CARTESIAN_POINT('Ctrl Pts',(-6.33083419837773,-39.0210126661744,
6.82480412008061));
#23255=CARTESIAN_POINT('Ctrl Pts',(-6.33139100183133,-39.1399921882013,
7.04022028559308));
#23256=CARTESIAN_POINT('Ctrl Pts',(-6.33267037013978,-39.2647757598683,
7.25306552029648));
#23257=CARTESIAN_POINT('Ctrl Pts',(-6.33467799886863,-39.3951753232291,
7.46287566269424));
#23258=CARTESIAN_POINT('Ctrl Pts',(-6.33668239850791,-39.5253651506641,
7.67234834441885));
#23259=CARTESIAN_POINT('Ctrl Pts',(-6.33941272481299,-39.6611527651412,
7.87879526533028));
#23260=CARTESIAN_POINT('Ctrl Pts',(-6.34286879629103,-39.8023029910568,
8.08177334612192));
#23261=CARTESIAN_POINT('Ctrl Pts',(-6.34632155154412,-39.9433177782516,
8.28455666214124));
#23262=CARTESIAN_POINT('Ctrl Pts',(-6.35049865962759,-40.0896846778747,
8.48387739272885));
#23263=CARTESIAN_POINT('Ctrl Pts',(-6.35539404456574,-40.2411239605253,
8.67931873611141));
#23264=CARTESIAN_POINT('Ctrl Pts',(-6.36028966495896,-40.3925705270046,
8.87476947970524));
#23265=CARTESIAN_POINT('Ctrl Pts',(-6.36590362406253,-40.5490896991202,
9.06634009532846));
#23266=CARTESIAN_POINT('Ctrl Pts',(-6.37222400138258,-40.7103600297418,
9.25364450340987));
#23267=CARTESIAN_POINT('Ctrl Pts',(-6.37854669727067,-40.8716895207925,
9.44101762226479));
#23268=CARTESIAN_POINT('Ctrl Pts',(-6.38557631500248,-41.0377733398943,
9.62412107874998));
#23269=CARTESIAN_POINT('Ctrl Pts',(-6.39329523799166,-41.208252351997,9.80260437466072));
#23270=CARTESIAN_POINT('Ctrl Pts',(-6.40102675214305,-41.3790094506799,
9.98137881379636));
#23271=CARTESIAN_POINT('Ctrl Pts',(-6.40944980108705,-41.5541757364557,
10.1555177270921));
#23272=CARTESIAN_POINT('Ctrl Pts',(-6.41854124933288,-41.7333579204532,
10.3247095747706));
#23273=CARTESIAN_POINT('Ctrl Pts',(-6.421168985615,-41.7851476368183,10.3736117457737));
#23274=CARTESIAN_POINT('Ctrl Pts',(-6.42385252692466,-41.8372726564643,
10.4221009095723));
#23275=CARTESIAN_POINT('Ctrl Pts',(-6.42659123460866,-41.8897230480067,
10.4701702229062));
#23276=CARTESIAN_POINT('Ctrl Pts',(-2.90816428999286,-44.4687528548127,
0.));
#23277=CARTESIAN_POINT('Ctrl Pts',(-2.69605969530409,-44.4992488915856,
1.72780310113342));
#23278=CARTESIAN_POINT('Ctrl Pts',(-2.59064364919737,-45.2717800827454,
3.28449990511991));
#23279=CARTESIAN_POINT('Ctrl Pts',(-2.48522760309065,-46.0443112739052,
4.84119670910638));
#23280=CARTESIAN_POINT('Ctrl Pts',(-2.46536913007014,-47.4119084566616,
5.91846432228298));
#23281=CARTESIAN_POINT('Ctrl Pts',(-2.4455106570496,-48.779505639418,6.99573193545957));
#23282=CARTESIAN_POINT('Ctrl Pts',(-2.47313305497492,-50.4773395333397,
7.38020429521639));
#23283=CARTESIAN_POINT('Ctrl Pts',(-2.50075545290024,-52.1751734272613,
7.76467665497322));
#23284=CARTESIAN_POINT('Ctrl Pts',(-2.52837785082555,-53.873007321183,7.38020429521639));
#23285=CARTESIAN_POINT('Ctrl Pts',(-3.79017222552544,-42.2673772240308,
0.));
#23286=CARTESIAN_POINT('Ctrl Pts',(-3.57806763083667,-42.2978732608037,
2.19648874705823));
#23287=CARTESIAN_POINT('Ctrl Pts',(-3.50159203012685,-43.2716896709822,
4.17545672685568));
#23288=CARTESIAN_POINT('Ctrl Pts',(-3.42511642941705,-44.2455060811606,
6.15442470665314));
#23289=CARTESIAN_POINT('Ctrl Pts',(-3.4574068370482,-45.9758066957265,7.5239130403414));
#23290=CARTESIAN_POINT('Ctrl Pts',(-3.48969724467936,-47.7061073102924,
8.89340137402967));
#23291=CARTESIAN_POINT('Ctrl Pts',(-3.58234823313402,-49.8562249858787,
9.3821661014496));
#23292=CARTESIAN_POINT('Ctrl Pts',(-3.67499922158868,-52.006342661465,9.87093082886954));
#23293=CARTESIAN_POINT('Ctrl Pts',(-3.76765021004335,-54.1564603370514,
9.3821661014496));
#23294=CARTESIAN_POINT('Ctrl Pts',(-4.22575906238243,-39.9362279852004,
0.));
#23295=CARTESIAN_POINT('Ctrl Pts',(-4.01365446769365,-39.9667240219733,
2.70899372698068));
#23296=CARTESIAN_POINT('Ctrl Pts',(-3.96882507274256,-41.1606446278505,
5.14971273833322));
#23297=CARTESIAN_POINT('Ctrl Pts',(-3.92399567779144,-42.3545652337278,
7.59043174968577));
#23298=CARTESIAN_POINT('Ctrl Pts',(-4.01331057777426,-44.4814799043322,
9.2794617117575));
#23299=CARTESIAN_POINT('Ctrl Pts',(-4.10262547775709,-46.6083945749367,
10.9684916738292));
#23300=CARTESIAN_POINT('Ctrl Pts',(-4.26638484508662,-49.2530818889509,
11.5712994880388));
#23301=CARTESIAN_POINT('Ctrl Pts',(-4.43014421241612,-51.897769202965,12.1741073022483));
#23302=CARTESIAN_POINT('Ctrl Pts',(-4.59390357974567,-54.5424565169792,
11.5712994880388));
#23303=CARTESIAN_POINT('Ctrl Pts',(-4.19818497005538,-37.5648924257372,
0.));
#23304=CARTESIAN_POINT('Ctrl Pts',(-3.98608037536661,-37.59538846251,3.24562220582793));
#23305=CARTESIAN_POINT('Ctrl Pts',(-3.97438676625733,-39.0197735211299,
6.16982677025167));
#23306=CARTESIAN_POINT('Ctrl Pts',(-3.96269315714806,-40.4441585797499,
9.09403133467541));
#23307=CARTESIAN_POINT('Ctrl Pts',(-4.11171668004481,-42.986355844513,11.1176436806954));
#23308=CARTESIAN_POINT('Ctrl Pts',(-4.26074020294156,-45.5285531092762,
13.1412560267153));
#23309=CARTESIAN_POINT('Ctrl Pts',(-4.49895500521084,-48.6910893479851,
13.8634749112255));
#23310=CARTESIAN_POINT('Ctrl Pts',(-4.7371698074801,-51.853625586694,14.5856937957357));
#23311=CARTESIAN_POINT('Ctrl Pts',(-4.97538460974937,-55.0161618254029,
13.8634749112255));
#23312=CARTESIAN_POINT('',(-4.19818497005538,-37.5648924257372,0.));
#23313=CARTESIAN_POINT('Ctrl Pts',(-4.19818497005538,-37.5648924257372,
0.));
#23314=CARTESIAN_POINT('Ctrl Pts',(-3.98608037536661,-37.59538846251,3.24562220582793));
#23315=CARTESIAN_POINT('Ctrl Pts',(-3.97438676625733,-39.0197735211299,
6.16982677025167));
#23316=CARTESIAN_POINT('Ctrl Pts',(-3.96462449666041,-40.2089043379837,
8.61106394926975));
#23317=CARTESIAN_POINT('Ctrl Pts',(-4.06844583510776,-42.2054524109828,
10.4489096280657));
#23318=CARTESIAN_POINT('Origin',(13.8005982420124,-37.7741838134885,0.));
#23319=CARTESIAN_POINT('Ctrl Pts',(-4.19818497005538,-37.5648924257372,
0.));
#23320=CARTESIAN_POINT('Ctrl Pts',(-3.98608037536661,-37.59538846251,3.24562220582793));
#23321=CARTESIAN_POINT('Ctrl Pts',(-3.97438676625733,-39.0197735211299,
6.16982677025167));
#23322=CARTESIAN_POINT('Ctrl Pts',(-3.96269315714806,-40.4441585797499,
9.09403133467541));
#23323=CARTESIAN_POINT('Ctrl Pts',(-4.11171668004481,-42.986355844513,11.1176436806954));
#23324=CARTESIAN_POINT('Ctrl Pts',(-4.26074020294156,-45.5285531092762,
13.1412560267153));
#23325=CARTESIAN_POINT('Ctrl Pts',(-4.49895500521085,-48.6910893479851,
13.8634749112255));
#23326=CARTESIAN_POINT('Ctrl Pts',(-4.7371698074801,-51.853625586694,14.5856937957357));
#23327=CARTESIAN_POINT('Ctrl Pts',(-4.97538460974937,-55.0161618254029,
13.8634749112255));
#23328=CARTESIAN_POINT('Ctrl Pts',(-4.81560839388882,-36.8396419064669,
0.));
#23329=CARTESIAN_POINT('Ctrl Pts',(-4.60350379920004,-36.8701379432397,
3.38941559469373));
#23330=CARTESIAN_POINT('Ctrl Pts',(-4.60068915780633,-38.3562775787769,
6.44317352589573));
#23331=CARTESIAN_POINT('Ctrl Pts',(-4.59787451641258,-39.8424172143141,
9.49693145709774));
#23332=CARTESIAN_POINT('Ctrl Pts',(-4.76289738629099,-42.4958923815832,
11.6101975146502));
#23333=CARTESIAN_POINT('Ctrl Pts',(-4.92792025616937,-45.1493675488523,
13.7234635722027));
#23334=CARTESIAN_POINT('Ctrl Pts',(-5.18608591779754,-48.4506650623305,
14.4776794959001));
#23335=CARTESIAN_POINT('Ctrl Pts',(-5.44425157942571,-51.7519625758087,
15.2318954195974));
#23336=CARTESIAN_POINT('Ctrl Pts',(-5.70241724105386,-55.0532600892869,
14.4776794959001));
#23337=CARTESIAN_POINT('Ctrl Pts',(-5.7583840898163,-36.7040912252865,0.));
#23338=CARTESIAN_POINT('Ctrl Pts',(-5.54627949512753,-36.7345872620594,
3.38941559469373));
#23339=CARTESIAN_POINT('Ctrl Pts',(-5.54346485373381,-38.2207268975965,
6.44317352589573));
#23340=CARTESIAN_POINT('Ctrl Pts',(-5.54065021234007,-39.7068665331337,
9.49693145709774));
#23341=CARTESIAN_POINT('Ctrl Pts',(-5.70567308221847,-42.3603417004028,
11.6101975146502));
#23342=CARTESIAN_POINT('Ctrl Pts',(-5.87069595209686,-45.0138168676719,
13.7234635722027));
#23343=CARTESIAN_POINT('Ctrl Pts',(-6.12886161372502,-48.3151143811501,
14.4776794959001));
#23344=CARTESIAN_POINT('Ctrl Pts',(-6.3870272753532,-51.6164118946283,15.2318954195974));
#23345=CARTESIAN_POINT('Ctrl Pts',(-6.64519293698135,-54.9177094081065,
14.4776794959001));
#23346=CARTESIAN_POINT('Ctrl Pts',(-6.55512420987408,-37.2260157227862,
0.));
#23347=CARTESIAN_POINT('Ctrl Pts',(-6.34301961518532,-37.2565117595591,
3.24562220582792));
#23348=CARTESIAN_POINT('Ctrl Pts',(-6.33132600607604,-38.680896818179,6.16982677025167));
#23349=CARTESIAN_POINT('Ctrl Pts',(-6.31963239696676,-40.1052818767989,
9.09403133467541));
#23350=CARTESIAN_POINT('Ctrl Pts',(-6.46865591986352,-42.6474791415621,
11.1176436806954));
#23351=CARTESIAN_POINT('Ctrl Pts',(-6.61767944276027,-45.1896764063252,
13.1412560267153));
#23352=CARTESIAN_POINT('Ctrl Pts',(-6.85589424502954,-48.3522126450341,
13.8634749112255));
#23353=CARTESIAN_POINT('Ctrl Pts',(-7.0941090472988,-51.514748883743,14.5856937957357));
#23354=CARTESIAN_POINT('Ctrl Pts',(-7.33232384956808,-54.6772851224519,
13.8634749112255));
#23355=CARTESIAN_POINT('',(-5.31261783616131,-36.9500337175413,1.04083408558609E-14));
#23356=CARTESIAN_POINT('Origin',(-5.56877962163367,-38.7317130208009,1.04083408558608E-14));
#23357=CARTESIAN_POINT('Origin',(-5.56877962163367,-38.7317130208009,1.04083408558608E-14));
#23358=CARTESIAN_POINT('Ctrl Pts',(-11.7862169042733,-35.914217116421,0.));
#23359=CARTESIAN_POINT('Ctrl Pts',(-11.5806112670702,-35.9745883786013,
3.24562220582792));
#23360=CARTESIAN_POINT('Ctrl Pts',(-11.7717478112972,-37.3861394252073,
6.16982677025168));
#23361=CARTESIAN_POINT('Ctrl Pts',(-11.9628843555243,-38.7976904718134,
9.09403133467542));
#23362=CARTESIAN_POINT('Ctrl Pts',(-12.4721834264256,-41.2928035754071,
11.1176436806954));
#23363=CARTESIAN_POINT('Ctrl Pts',(-12.9814824973271,-43.7879166790007,
13.1412560267153));
#23364=CARTESIAN_POINT('Ctrl Pts',(-13.6673484497319,-46.884361357741,13.8634749112255));
#23365=CARTESIAN_POINT('Ctrl Pts',(-14.3532144021367,-49.9808060364813,
14.5856937957357));
#23366=CARTESIAN_POINT('Ctrl Pts',(-15.0390803545415,-53.0772507152216,
13.8634749112255));
#23367=CARTESIAN_POINT('Ctrl Pts',(-12.746223019916,-38.0827145049533,0.));
#23368=CARTESIAN_POINT('Ctrl Pts',(-12.5406173827129,-38.1430857671336,
2.70899372698069));
#23369=CARTESIAN_POINT('Ctrl Pts',(-12.6661569043003,-39.3312338708267,
5.14971273833323));
#23370=CARTESIAN_POINT('Ctrl Pts',(-12.7916964258877,-40.5193819745198,
7.59043174968578));
#23371=CARTESIAN_POINT('Ctrl Pts',(-13.1827937463383,-42.6119368849888,
9.27946171175752));
#23372=CARTESIAN_POINT('Ctrl Pts',(-13.5738910667889,-44.7044917954578,
10.9684916738293));
#23373=CARTESIAN_POINT('Ctrl Pts',(-14.1123618472579,-47.2989546180623,
11.5712994880388));
#23374=CARTESIAN_POINT('Ctrl Pts',(-14.6508326277268,-49.8934174406667,
12.1741073022483));
#23375=CARTESIAN_POINT('Ctrl Pts',(-15.1893034081958,-52.4878802632712,
11.5712994880388));
#23376=CARTESIAN_POINT('Ctrl Pts',(-14.1108411348345,-40.0222531270433,
0.));
#23377=CARTESIAN_POINT('Ctrl Pts',(-13.9052354976314,-40.0826243892237,
2.19648874705824));
#23378=CARTESIAN_POINT('Ctrl Pts',(-13.9681268331905,-41.0574123652206,
4.17545672685568));
#23379=CARTESIAN_POINT('Ctrl Pts',(-14.0310181687496,-42.0322003412177,
6.15442470665314));
#23380=CARTESIAN_POINT('Ctrl Pts',(-14.3092273587161,-43.7402935862749,
7.5239130403414));
#23381=CARTESIAN_POINT('Ctrl Pts',(-14.5874365486826,-45.4483868313322,
8.89340137402967));
#23382=CARTESIAN_POINT('Ctrl Pts',(-14.9851381329361,-47.563433798757,9.38216610144961));
#23383=CARTESIAN_POINT('Ctrl Pts',(-15.3828397171896,-49.6784807661818,
9.87093082886954));
#23384=CARTESIAN_POINT('Ctrl Pts',(-15.7805413014431,-51.7935277336065,
9.38216610144961));
#23385=CARTESIAN_POINT('Ctrl Pts',(-15.8276282594348,-41.6582954965892,
0.));
#23386=CARTESIAN_POINT('Ctrl Pts',(-15.6220226222317,-41.7186667587696,
1.72780310113343));
#23387=CARTESIAN_POINT('Ctrl Pts',(-15.6276222110079,-42.4983369638544,
3.28449990511991));
#23388=CARTESIAN_POINT('Ctrl Pts',(-15.6332217997841,-43.2780071689393,
4.84119670910638));
#23389=CARTESIAN_POINT('Ctrl Pts',(-15.8081948292724,-44.6345103396638,
5.91846432228298));
#23390=CARTESIAN_POINT('Ctrl Pts',(-15.9831678587607,-45.9910135103884,
6.99573193545956));
#23391=CARTESIAN_POINT('Ctrl Pts',(-16.2521360565317,-47.6676348262508,
7.38020429521639));
#23392=CARTESIAN_POINT('Ctrl Pts',(-16.5211042543027,-49.3442561421131,
7.76467665497322));
#23393=CARTESIAN_POINT('Ctrl Pts',(-16.7900724520737,-51.0208774579755,
7.38020429521639));
#23394=CARTESIAN_POINT('',(-11.7862169043636,-35.9142171164879,1.5794896091565E-9));
#23395=CARTESIAN_POINT('Origin',(-28.2454287759838,-28.6276304970125,0.));
#23396=CARTESIAN_POINT('Ctrl Pts',(-11.7862169041096,-35.9142171165575,
3.13105415629025E-9));
#23397=CARTESIAN_POINT('Ctrl Pts',(-11.7706940792789,-35.9187750292274,
0.245038153335357));
#23398=CARTESIAN_POINT('Ctrl Pts',(-11.7568199184777,-35.9294543009582,
0.490791160521484));
#23399=CARTESIAN_POINT('Ctrl Pts',(-11.7446485667473,-35.9463285033518,
0.736766500725023));
#23400=CARTESIAN_POINT('Ctrl Pts',(-11.732517172881,-35.9631473086865,0.981934317700669));
#23401=CARTESIAN_POINT('Ctrl Pts',(-11.7220774809609,-35.9861205266374,
1.22732257376532));
#23402=CARTESIAN_POINT('Ctrl Pts',(-11.7133702409767,-36.0152719968249,
1.47243294816308));
#23403=CARTESIAN_POINT('Ctrl Pts',(-11.704676114391,-36.0443795639103,1.71717417802986));
#23404=CARTESIAN_POINT('Ctrl Pts',(-11.6977092667636,-36.079646826587,1.96163791541557));
#23405=CARTESIAN_POINT('Ctrl Pts',(-11.6924966907341,-36.1210475853283,
2.20532408778498));
#23406=CARTESIAN_POINT('Ctrl Pts',(-11.6872885852766,-36.1624128366599,
2.44880126242047));
#23407=CARTESIAN_POINT('Ctrl Pts',(-11.6838317679612,-36.2099010442177,
2.69150175431038));
#23408=CARTESIAN_POINT('Ctrl Pts',(-11.6821391062285,-36.2634360706163,
2.93292951866803));
#23409=CARTESIAN_POINT('Ctrl Pts',(-11.6804467986039,-36.3169598973807,
3.17430677585587));
#23410=CARTESIAN_POINT('Ctrl Pts',(-11.6805179152419,-36.3765279276398,
3.41441139318343));
#23411=CARTESIAN_POINT('Ctrl Pts',(-11.6823510237341,-36.442014877408,3.65275710614637));
#23412=CARTESIAN_POINT('Ctrl Pts',(-11.6841864598781,-36.5075849814587,
3.89140546668792));
#23413=CARTESIAN_POINT('Ctrl Pts',(-11.6877883562709,-36.5790889062839,
4.12829002081172));
#23414=CARTESIAN_POINT('Ctrl Pts',(-11.6931409581034,-36.6563532415795,
4.3629387437782));
#23415=CARTESIAN_POINT('Ctrl Pts',(-11.6984990217243,-36.7336964173083,
4.59782690201463));
#23416=CARTESIAN_POINT('Ctrl Pts',(-11.7056113365129,-36.8168115609901,
4.83047425894977));
#23417=CARTESIAN_POINT('Ctrl Pts',(-11.7144480496046,-36.9054796074171,
5.06042975959451));
#23418=CARTESIAN_POINT('Ctrl Pts',(-11.7233105977815,-36.994406884455,5.29105755998321));
#23419=CARTESIAN_POINT('Ctrl Pts',(-11.7339075987035,-37.0889193314433,
5.51897736305701));
#23420=CARTESIAN_POINT('Ctrl Pts',(-11.7461953488408,-37.1887539873582,
5.7437625935434));
#23421=CARTESIAN_POINT('Ctrl Pts',(-11.7540303837175,-37.2524115326579,
5.88709234072625));
#23422=CARTESIAN_POINT('Ctrl Pts',(-11.7625525566674,-37.318232100817,6.02914825314195));
#23423=CARTESIAN_POINT('Ctrl Pts',(-11.771747811312,-37.3861394252394,6.16982677023483));
#23424=CARTESIAN_POINT('Ctrl Pts',(-11.7861662410924,-37.4926201075707,
6.39041482339093));
#23425=CARTESIAN_POINT('Ctrl Pts',(-11.8021412942474,-37.6049078439223,
6.60890054011811));
#23426=CARTESIAN_POINT('Ctrl Pts',(-11.8196645413938,-37.7228633758097,
6.82480412008051));
#23427=CARTESIAN_POINT('Ctrl Pts',(-11.8371482288262,-37.8405526164633,
7.04022028559307));
#23428=CARTESIAN_POINT('Ctrl Pts',(-11.8561731288309,-37.9638839982,7.25306552029657));
#23429=CARTESIAN_POINT('Ctrl Pts',(-11.8767181155647,-38.0926705666685,
7.46287566269442));
#23430=CARTESIAN_POINT('Ctrl Pts',(-11.897230057542,-38.2212499935681,7.67234834441907));
#23431=CARTESIAN_POINT('Ctrl Pts',(-11.9192571854559,-38.3552669199728,
7.87879526533054));
#23432=CARTESIAN_POINT('Ctrl Pts',(-11.9427658506829,-38.494488589857,8.08177334612222));
#23433=CARTESIAN_POINT('Ctrl Pts',(-11.9662519584997,-38.6335766715389,
8.28455666214102));
#23434=CARTESIAN_POINT('Ctrl Pts',(-11.9912167312942,-38.7778593027057,
8.48387739272812));
#23435=CARTESIAN_POINT('Ctrl Pts',(-12.0176143452908,-38.9270604659002,
8.6793187361102));
#23436=CARTESIAN_POINT('Ctrl Pts',(-12.0440132289428,-39.076268805276,8.87476947970396));
#23437=CARTESIAN_POINT('Ctrl Pts',(-12.0718450467037,-39.2303958882196,
9.06634009532711));
#23438=CARTESIAN_POINT('Ctrl Pts',(-12.1010522527165,-39.3891252359318,
9.25364450340846));
#23439=CARTESIAN_POINT('Ctrl Pts',(-12.1302701731047,-39.547912811939,9.44101762226378));
#23440=CARTESIAN_POINT('Ctrl Pts',(-12.1608644313192,-39.7113057183252,
9.62412107874935));
#23441=CARTESIAN_POINT('Ctrl Pts',(-12.1927664798385,-39.8789509826187,
9.80260437466046));
#23442=CARTESIAN_POINT('Ctrl Pts',(-12.2247205672069,-40.0468697110623,
9.98137881379621));
#23443=CARTESIAN_POINT('Ctrl Pts',(-12.2579866432888,-40.2190543317698,
10.1555177270921));
#23444=CARTESIAN_POINT('Ctrl Pts',(-12.2924858372373,-40.3951188515068,
10.3247095747706));
#23445=CARTESIAN_POINT('Ctrl Pts',(-12.3024572720617,-40.4460074573699,
10.3736117457737));
#23446=CARTESIAN_POINT('Ctrl Pts',(-12.3125316625311,-40.4972200117265,
10.4221009095723));
#23447=CARTESIAN_POINT('Ctrl Pts',(-12.3227069631095,-40.5487467751691,
10.4701702229062));
#23448=CARTESIAN_POINT('Ctrl Pts',(-9.20712674149475,-43.6022501387951,
0.));
#23449=CARTESIAN_POINT('Ctrl Pts',(-9.00152110429164,-43.6626214009754,
1.72780310113343));
#23450=CARTESIAN_POINT('Ctrl Pts',(-9.00712069306788,-44.4422916060603,
3.28449990511991));
#23451=CARTESIAN_POINT('Ctrl Pts',(-9.01272028184411,-45.2219618111451,
4.84119670910639));
#23452=CARTESIAN_POINT('Ctrl Pts',(-9.18769331133237,-46.5784649818697,
5.91846432228298));
#23453=CARTESIAN_POINT('Ctrl Pts',(-9.36266634082062,-47.9349681525942,
6.99573193545956));
#23454=CARTESIAN_POINT('Ctrl Pts',(-9.63163453859162,-49.6115894684566,
7.38020429521639));
#23455=CARTESIAN_POINT('Ctrl Pts',(-9.90060273636263,-51.288210784319,7.76467665497322));
#23456=CARTESIAN_POINT('Ctrl Pts',(-10.1695709341336,-52.9648321001814,
7.38020429521639));
#23457=CARTESIAN_POINT('Ctrl Pts',(-9.76686869112056,-41.297758521112,0.));
#23458=CARTESIAN_POINT('Ctrl Pts',(-9.56126305391744,-41.3581297832923,
2.19648874705824));
#23459=CARTESIAN_POINT('Ctrl Pts',(-9.62415438947656,-42.3329177592893,
4.17545672685568));
#23460=CARTESIAN_POINT('Ctrl Pts',(-9.68704572503569,-43.3077057352863,
6.15442470665314));
#23461=CARTESIAN_POINT('Ctrl Pts',(-9.96525491500219,-45.0157989803436,
7.5239130403414));
#23462=CARTESIAN_POINT('Ctrl Pts',(-10.2434641049687,-46.7238922254008,
8.89340137402967));
#23463=CARTESIAN_POINT('Ctrl Pts',(-10.6411656892222,-48.8389391928256,
9.38216610144961));
#23464=CARTESIAN_POINT('Ctrl Pts',(-11.0388672734757,-50.9539861602504,
9.87093082886954));
#23465=CARTESIAN_POINT('Ctrl Pts',(-11.4365688577292,-53.0690331276752,
9.38216610144961));
#23466=CARTESIAN_POINT('Ctrl Pts',(-9.86626475512766,-38.9283465500519,
0.));
#23467=CARTESIAN_POINT('Ctrl Pts',(-9.66065911792456,-38.9887178122322,
2.70899372698069));
#23468=CARTESIAN_POINT('Ctrl Pts',(-9.78619863951197,-40.1768659159253,
5.14971273833323));
#23469=CARTESIAN_POINT('Ctrl Pts',(-9.91173816109936,-41.3650140196185,
7.59043174968578));
#23470=CARTESIAN_POINT('Ctrl Pts',(-10.30283548155,-43.4575689300875,9.27946171175752));
#23471=CARTESIAN_POINT('Ctrl Pts',(-10.6939328020006,-45.5501238405564,
10.9684916738293));
#23472=CARTESIAN_POINT('Ctrl Pts',(-11.2324035824695,-48.1445866631609,
11.5712994880388));
#23473=CARTESIAN_POINT('Ctrl Pts',(-11.7708743629385,-50.7390494857654,
12.1741073022483));
#23474=CARTESIAN_POINT('Ctrl Pts',(-12.3093451434074,-53.3335123083699,
11.5712994880388));
#23475=CARTESIAN_POINT('Ctrl Pts',(-9.50149509066523,-36.5850719698905,
0.));
#23476=CARTESIAN_POINT('Ctrl Pts',(-9.29588945346213,-36.6454432320708,
3.24562220582793));
#23477=CARTESIAN_POINT('Ctrl Pts',(-9.48702599768917,-38.0569942786768,
6.16982677025168));
#23478=CARTESIAN_POINT('Ctrl Pts',(-9.67816254191622,-39.4685453252829,
9.09403133467541));
#23479=CARTESIAN_POINT('Ctrl Pts',(-10.1874616128176,-41.9636584288766,
11.1176436806954));
#23480=CARTESIAN_POINT('Ctrl Pts',(-10.696760683719,-44.4587715324702,13.1412560267153));
#23481=CARTESIAN_POINT('Ctrl Pts',(-11.3826266361238,-47.5552162112105,
13.8634749112255));
#23482=CARTESIAN_POINT('Ctrl Pts',(-12.0684925885286,-50.6516608899508,
14.5856937957357));
#23483=CARTESIAN_POINT('Ctrl Pts',(-12.7543585409334,-53.7481055686911,
13.8634749112255));
#23484=CARTESIAN_POINT('',(-9.50149509066523,-36.5850719698905,3.46944695195361E-15));
#23485=CARTESIAN_POINT('Ctrl Pts',(-9.50149509066523,-36.5850719698905,
3.46944695195361E-15));
#23486=CARTESIAN_POINT('Ctrl Pts',(-9.29588945346213,-36.6454432320708,
3.24562220582793));
#23487=CARTESIAN_POINT('Ctrl Pts',(-9.48702599768917,-38.0569942786769,
6.16982677025168));
#23488=CARTESIAN_POINT('Ctrl Pts',(-9.64659405380704,-39.235410774219,8.61106394926974));
#23489=CARTESIAN_POINT('Ctrl Pts',(-10.0334970568407,-41.1968615496291,
10.4489096280657));
#23490=CARTESIAN_POINT('Origin',(8.28430119040622,-39.3537269950291,0.));
#23491=CARTESIAN_POINT('Ctrl Pts',(-9.50149509066523,-36.5850719698905,
0.));
#23492=CARTESIAN_POINT('Ctrl Pts',(-9.29588945346213,-36.6454432320708,
3.24562220582793));
#23493=CARTESIAN_POINT('Ctrl Pts',(-9.48702599768917,-38.0569942786769,
6.16982677025168));
#23494=CARTESIAN_POINT('Ctrl Pts',(-9.67816254191622,-39.4685453252829,
9.0940313346754));
#23495=CARTESIAN_POINT('Ctrl Pts',(-10.1874616128176,-41.9636584288766,
11.1176436806954));
#23496=CARTESIAN_POINT('Ctrl Pts',(-10.696760683719,-44.4587715324702,13.1412560267153));
#23497=CARTESIAN_POINT('Ctrl Pts',(-11.3826266361238,-47.5552162112105,
13.8634749112255));
#23498=CARTESIAN_POINT('Ctrl Pts',(-12.0684925885286,-50.6516608899508,
14.5856937957357));
#23499=CARTESIAN_POINT('Ctrl Pts',(-12.7543585409334,-53.7481055686911,
13.8634749112255));
#23500=CARTESIAN_POINT('Ctrl Pts',(-10.0094201239375,-35.7793349404725,
0.));
#23501=CARTESIAN_POINT('Ctrl Pts',(-9.80381448673444,-35.8397062026528,
3.38941559469372));
#23502=CARTESIAN_POINT('Ctrl Pts',(-10.0125282162147,-37.3111196447714,
6.44317352589574));
#23503=CARTESIAN_POINT('Ctrl Pts',(-10.221241945695,-38.78253308689,9.49693145709774));
#23504=CARTESIAN_POINT('Ctrl Pts',(-10.7622140099934,-41.3855144999134,
11.6101975146502));
#23505=CARTESIAN_POINT('Ctrl Pts',(-11.3031860742919,-43.9884959129367,
13.7234635722027));
#23506=CARTESIAN_POINT('Ctrl Pts',(-12.0285476034514,-47.2194501734234,
14.4776794959001));
#23507=CARTESIAN_POINT('Ctrl Pts',(-12.753909132611,-50.45040443391,15.2318954195974));
#23508=CARTESIAN_POINT('Ctrl Pts',(-13.4792706617706,-53.6813586943966,
14.4776794959001));
#23509=CARTESIAN_POINT('Ctrl Pts',(-10.9233088493808,-35.5109929990847,
6.24500451351651E-15));
#23510=CARTESIAN_POINT('Ctrl Pts',(-10.7177032121776,-35.571364261265,3.38941559469372));
#23511=CARTESIAN_POINT('Ctrl Pts',(-10.9264169416579,-37.0427777033836,
6.44317352589573));
#23512=CARTESIAN_POINT('Ctrl Pts',(-11.1351306711382,-38.5141911455021,
9.49693145709774));
#23513=CARTESIAN_POINT('Ctrl Pts',(-11.6761027354366,-41.1171725585255,
11.6101975146502));
#23514=CARTESIAN_POINT('Ctrl Pts',(-12.2170747997351,-43.7201539715489,
13.7234635722027));
#23515=CARTESIAN_POINT('Ctrl Pts',(-12.9424363288947,-46.9511082320356,
14.4776794959001));
#23516=CARTESIAN_POINT('Ctrl Pts',(-13.6677978580543,-50.1820624925222,
15.2318954195974));
#23517=CARTESIAN_POINT('Ctrl Pts',(-14.3931593872138,-53.4130167530088,
14.4776794959001));
#23518=CARTESIAN_POINT('Ctrl Pts',(-11.7862169042733,-35.914217116421,0.));
#23519=CARTESIAN_POINT('Ctrl Pts',(-11.5806112670702,-35.9745883786013,
3.24562220582792));
#23520=CARTESIAN_POINT('Ctrl Pts',(-11.7717478112972,-37.3861394252073,
6.16982677025167));
#23521=CARTESIAN_POINT('Ctrl Pts',(-11.9628843555243,-38.7976904718134,
9.09403133467541));
#23522=CARTESIAN_POINT('Ctrl Pts',(-12.4721834264257,-41.2928035754071,
11.1176436806954));
#23523=CARTESIAN_POINT('Ctrl Pts',(-12.9814824973271,-43.7879166790007,
13.1412560267153));
#23524=CARTESIAN_POINT('Ctrl Pts',(-13.6673484497319,-46.884361357741,13.8634749112255));
#23525=CARTESIAN_POINT('Ctrl Pts',(-14.3532144021367,-49.9808060364813,
14.5856937957357));
#23526=CARTESIAN_POINT('Ctrl Pts',(-15.0390803545415,-53.0772507152216,
13.8634749112255));
#23527=CARTESIAN_POINT('',(-10.5170811194434,-35.8178713036885,1.00239475044027E-29));
#23528=CARTESIAN_POINT('Origin',(-11.0241949492052,-37.5449600575353,0.));
#23529=CARTESIAN_POINT('Origin',(-11.0241949492052,-37.5449600575353,0.));
#23530=CARTESIAN_POINT('Ctrl Pts',(-16.7773762111443,-33.8713086176152,
1.04083408558608E-14));
#23531=CARTESIAN_POINT('Ctrl Pts',(-16.5824550692826,-33.9603261204013,
3.24562220582793));
#23532=CARTESIAN_POINT('Ctrl Pts',(-16.9725307779978,-35.3303080462616,
6.16982677025167));
#23533=CARTESIAN_POINT('Ctrl Pts',(-17.362606486713,-36.700289972122,9.0940313346754));
#23534=CARTESIAN_POINT('Ctrl Pts',(-18.2218132452327,-39.097525607069,11.1176436806954));
#23535=CARTESIAN_POINT('Ctrl Pts',(-19.0810200037525,-41.4947612420161,
13.1412560267153));
#23536=CARTESIAN_POINT('Ctrl Pts',(-20.2005748533759,-44.4620796765377,
13.8634749112255));
#23537=CARTESIAN_POINT('Ctrl Pts',(-21.3201297029994,-47.4293981110593,
14.5856937957357));
#23538=CARTESIAN_POINT('Ctrl Pts',(-22.4396845526228,-50.3967165455809,
13.8634749112255));
#23539=CARTESIAN_POINT('Ctrl Pts',(-18.0362202038893,-35.8811107143582,
0.));
#23540=CARTESIAN_POINT('Ctrl Pts',(-17.8412990620276,-35.9701282171443,
2.70899372698069));
#23541=CARTESIAN_POINT('Ctrl Pts',(-18.1346518775201,-37.1283165495983,
5.14971273833323));
#23542=CARTESIAN_POINT('Ctrl Pts',(-18.4280046930126,-38.2865048820523,
7.59043174968578));
#23543=CARTESIAN_POINT('Ctrl Pts',(-19.1129228203181,-40.3021016488387,
9.27946171175752));
#23544=CARTESIAN_POINT('Ctrl Pts',(-19.7978409476237,-42.3176984156251,
10.9684916738293));
#23545=CARTESIAN_POINT('Ctrl Pts',(-20.7000614289633,-44.8091209655646,
11.5712994880388));
#23546=CARTESIAN_POINT('Ctrl Pts',(-21.6022819103028,-47.3005435155041,
12.1741073022483));
#23547=CARTESIAN_POINT('Ctrl Pts',(-22.5045023916423,-49.7919660654436,
11.5712994880388));
#23548=CARTESIAN_POINT('Ctrl Pts',(-19.6629735993423,-37.6067022235297,
0.));
#23549=CARTESIAN_POINT('Ctrl Pts',(-19.4680524574806,-37.6957197263158,
2.19648874705823));
#23550=CARTESIAN_POINT('Ctrl Pts',(-19.6690304430803,-38.6516353959965,
4.17545672685568));
#23551=CARTESIAN_POINT('Ctrl Pts',(-19.87000842868,-39.6075510656772,6.15442470665313));
#23552=CARTESIAN_POINT('Ctrl Pts',(-20.3884728641632,-41.2586650884906,
7.5239130403414));
#23553=CARTESIAN_POINT('Ctrl Pts',(-20.9069372996464,-42.909779111304,8.89340137402967));
#23554=CARTESIAN_POINT('Ctrl Pts',(-21.60159342232,-44.9466991136023,9.3821661014496));
#23555=CARTESIAN_POINT('Ctrl Pts',(-22.2962495449936,-46.9836191159005,
9.87093082886953));
#23556=CARTESIAN_POINT('Ctrl Pts',(-22.9909056676672,-49.0205391181987,
9.3821661014496));
#23557=CARTESIAN_POINT('Ctrl Pts',(-21.595119411647,-38.9817677587448,0.));
#23558=CARTESIAN_POINT('Ctrl Pts',(-21.4001982697853,-39.0707852615309,
1.72780310113343));
#23559=CARTESIAN_POINT('Ctrl Pts',(-21.5166995019649,-39.8417226435485,
3.28449990511991));
#23560=CARTESIAN_POINT('Ctrl Pts',(-21.6332007341444,-40.6126600255661,
4.84119670910639));
#23561=CARTESIAN_POINT('Ctrl Pts',(-21.9994433198417,-41.930454691535,5.91846432228297));
#23562=CARTESIAN_POINT('Ctrl Pts',(-22.3656859055389,-43.2482493575038,
6.99573193545956));
#23563=CARTESIAN_POINT('Ctrl Pts',(-22.8705244862892,-44.8695269202926,
7.38020429521639));
#23564=CARTESIAN_POINT('Ctrl Pts',(-23.3753630670395,-46.4908044830813,
7.76467665497322));
#23565=CARTESIAN_POINT('Ctrl Pts',(-23.8802016477898,-48.1120820458701,
7.38020429521639));
#23566=CARTESIAN_POINT('',(-16.7773762107575,-33.8713086176117,-2.44187790973619E-9));
#23567=CARTESIAN_POINT('Origin',(-32.0320676419192,-24.3164988679737,0.));
#23568=CARTESIAN_POINT('Ctrl Pts',(-16.7773762111443,-33.8713086176152,
1.04083408558608E-14));
#23569=CARTESIAN_POINT('Ctrl Pts',(-16.5824550692826,-33.9603261204013,
3.24562220582793));
#23570=CARTESIAN_POINT('Ctrl Pts',(-16.9725307779978,-35.3303080462616,
6.16982677025167));
#23571=CARTESIAN_POINT('Ctrl Pts',(-17.3001355482564,-36.4808862649314,
8.62571762198518));
#23572=CARTESIAN_POINT('Ctrl Pts',(-17.9679679135938,-38.3823149509186,
10.4701702229062));
#23573=CARTESIAN_POINT('Ctrl Pts',(-15.3186586437008,-41.8481313484578,
0.));
#23574=CARTESIAN_POINT('Ctrl Pts',(-15.1237375018391,-41.9371488512439,
1.72780310113342));
#23575=CARTESIAN_POINT('Ctrl Pts',(-15.2402387340187,-42.7080862332615,
3.28449990511991));
#23576=CARTESIAN_POINT('Ctrl Pts',(-15.3567399661983,-43.4790236152791,
4.84119670910639));
#23577=CARTESIAN_POINT('Ctrl Pts',(-15.7229825518955,-44.796818281248,5.91846432228298));
#23578=CARTESIAN_POINT('Ctrl Pts',(-16.0892251375927,-46.1146129472168,
6.99573193545956));
#23579=CARTESIAN_POINT('Ctrl Pts',(-16.594063718343,-47.7358905100056,7.38020429521639));
#23580=CARTESIAN_POINT('Ctrl Pts',(-17.0989022990933,-49.3571680727943,
7.76467665497322));
#23581=CARTESIAN_POINT('Ctrl Pts',(-17.6037408798436,-50.9784456355831,
7.38020429521639));
#23582=CARTESIAN_POINT('Ctrl Pts',(-15.5447398754879,-39.4874365476044,
0.));
#23583=CARTESIAN_POINT('Ctrl Pts',(-15.3498187336262,-39.5764540503905,
2.19648874705823));
#23584=CARTESIAN_POINT('Ctrl Pts',(-15.5507967192259,-40.5323697200712,
4.17545672685568));
#23585=CARTESIAN_POINT('Ctrl Pts',(-15.7517747048257,-41.4882853897519,
6.15442470665314));
#23586=CARTESIAN_POINT('Ctrl Pts',(-16.2702391403089,-43.1393994125653,
7.5239130403414));
#23587=CARTESIAN_POINT('Ctrl Pts',(-16.788703575792,-44.7905134353787,8.89340137402967));
#23588=CARTESIAN_POINT('Ctrl Pts',(-17.4833596984656,-46.8274334376769,
9.3821661014496));
#23589=CARTESIAN_POINT('Ctrl Pts',(-18.1780158211392,-48.8643534399752,
9.87093082886954));
#23590=CARTESIAN_POINT('Ctrl Pts',(-18.8726719438128,-50.9012734422734,
9.3821661014496));
#23591=CARTESIAN_POINT('Ctrl Pts',(-15.3059217494165,-37.1279962392256,
0.));
#23592=CARTESIAN_POINT('Ctrl Pts',(-15.1110006075549,-37.2170137420117,
2.70899372698069));
#23593=CARTESIAN_POINT('Ctrl Pts',(-15.4043534230473,-38.3752020744657,
5.14971273833323));
#23594=CARTESIAN_POINT('Ctrl Pts',(-15.6977062385398,-39.5333904069197,
7.59043174968577));
#23595=CARTESIAN_POINT('Ctrl Pts',(-16.3826243658454,-41.5489871737062,
9.27946171175751));
#23596=CARTESIAN_POINT('Ctrl Pts',(-17.0675424931509,-43.5645839404925,
10.9684916738293));
#23597=CARTESIAN_POINT('Ctrl Pts',(-17.9697629744905,-46.0560064904321,
11.5712994880388));
#23598=CARTESIAN_POINT('Ctrl Pts',(-18.87198345583,-48.5474290403715,12.1741073022483));
#23599=CARTESIAN_POINT('Ctrl Pts',(-19.7742039371695,-51.038851590311,11.5712994880388));
#23600=CARTESIAN_POINT('Ctrl Pts',(-14.6113821712783,-34.8604849513723,
1.04083408558608E-14));
#23601=CARTESIAN_POINT('Ctrl Pts',(-14.4164610294167,-34.9495024541584,
3.24562220582793));
#23602=CARTESIAN_POINT('Ctrl Pts',(-14.8065367381318,-36.3194843800187,
6.16982677025167));
#23603=CARTESIAN_POINT('Ctrl Pts',(-15.196612446847,-37.6894663058791,9.09403133467541));
#23604=CARTESIAN_POINT('Ctrl Pts',(-16.0558192053667,-40.0867019408261,
11.1176436806954));
#23605=CARTESIAN_POINT('Ctrl Pts',(-16.9150259638865,-42.4839375757732,
13.1412560267153));
#23606=CARTESIAN_POINT('Ctrl Pts',(-18.0345808135099,-45.4512560102948,
13.8634749112255));
#23607=CARTESIAN_POINT('Ctrl Pts',(-19.1541356631334,-48.4185744448164,
14.5856937957357));
#23608=CARTESIAN_POINT('Ctrl Pts',(-20.2736905127569,-51.385892879338,13.8634749112255));
#23609=CARTESIAN_POINT('',(-14.6113821712783,-34.8604849513723,1.04083408558608E-14));
#23610=CARTESIAN_POINT('Ctrl Pts',(-14.6113821712783,-34.8604849513723,
1.04083408558608E-14));
#23611=CARTESIAN_POINT('Ctrl Pts',(-14.4164610294167,-34.9495024541584,
3.24562220582793));
#23612=CARTESIAN_POINT('Ctrl Pts',(-14.8065367381318,-36.3194843800187,
6.16982677025167));
#23613=CARTESIAN_POINT('Ctrl Pts',(-15.1321867744982,-37.4631973926725,
8.61106394926976));
#23614=CARTESIAN_POINT('Ctrl Pts',(-15.7942952127126,-39.3496213890633,
10.4489096280657));
#23615=CARTESIAN_POINT('Origin',(2.59935965651522,-40.1321417817282,0.));
#23616=CARTESIAN_POINT('Ctrl Pts',(-14.6113821712783,-34.8604849513723,
1.04083408558608E-14));
#23617=CARTESIAN_POINT('Ctrl Pts',(-14.4164610294167,-34.9495024541584,
3.24562220582793));
#23618=CARTESIAN_POINT('Ctrl Pts',(-14.8065367381318,-36.3194843800187,
6.16982677025167));
#23619=CARTESIAN_POINT('Ctrl Pts',(-15.196612446847,-37.6894663058791,9.09403133467541));
#23620=CARTESIAN_POINT('Ctrl Pts',(-16.0558192053667,-40.0867019408261,
11.1176436806954));
#23621=CARTESIAN_POINT('Ctrl Pts',(-16.9150259638865,-42.4839375757732,
13.1412560267153));
#23622=CARTESIAN_POINT('Ctrl Pts',(-18.0345808135099,-45.4512560102947,
13.8634749112255));
#23623=CARTESIAN_POINT('Ctrl Pts',(-19.1541356631334,-48.4185744448164,
14.5856937957357));
#23624=CARTESIAN_POINT('Ctrl Pts',(-20.2736905127569,-51.385892879338,13.8634749112255));
#23625=CARTESIAN_POINT('Ctrl Pts',(-14.9994689250469,-33.9906638941718,
0.));
#23626=CARTESIAN_POINT('Ctrl Pts',(-14.8045477831852,-34.0796813969579,
3.38941559469372));
#23627=CARTESIAN_POINT('Ctrl Pts',(-15.220541073888,-35.5064149111823,6.44317352589573));
#23628=CARTESIAN_POINT('Ctrl Pts',(-15.6365343645908,-36.9331484254067,
9.49693145709774));
#23629=CARTESIAN_POINT('Ctrl Pts',(-16.5424429921147,-39.4326468889938,
11.6101975146502));
#23630=CARTESIAN_POINT('Ctrl Pts',(-17.4483516196387,-41.9321453525809,
13.7234635722027));
#23631=CARTESIAN_POINT('Ctrl Pts',(-18.626142747366,-45.0269834486351,14.4776794959001));
#23632=CARTESIAN_POINT('Ctrl Pts',(-19.8039338750932,-48.1218215446893,
15.2318954195974));
#23633=CARTESIAN_POINT('Ctrl Pts',(-20.9817250028204,-51.2166596407435,
14.4776794959001));
#23634=CARTESIAN_POINT('Ctrl Pts',(-15.8658665409933,-33.594993360669,0.));
#23635=CARTESIAN_POINT('Ctrl Pts',(-15.6709453991316,-33.6840108634551,
3.38941559469372));
#23636=CARTESIAN_POINT('Ctrl Pts',(-16.0869386898344,-35.1107443776795,
6.44317352589574));
#23637=CARTESIAN_POINT('Ctrl Pts',(-16.5029319805371,-36.5374778919039,
9.49693145709774));
#23638=CARTESIAN_POINT('Ctrl Pts',(-17.4088406080611,-39.036976355491,11.6101975146502));
#23639=CARTESIAN_POINT('Ctrl Pts',(-18.3147492355851,-41.536474819078,13.7234635722027));
#23640=CARTESIAN_POINT('Ctrl Pts',(-19.4925403633123,-44.6313129151322,
14.4776794959001));
#23641=CARTESIAN_POINT('Ctrl Pts',(-20.6703314910396,-47.7261510111864,
15.2318954195974));
#23642=CARTESIAN_POINT('Ctrl Pts',(-21.8481226187668,-50.8209891072406,
14.4776794959001));
#23643=CARTESIAN_POINT('Ctrl Pts',(-16.7773762111443,-33.8713086176152,
1.04083408558608E-14));
#23644=CARTESIAN_POINT('Ctrl Pts',(-16.5824550692826,-33.9603261204013,
3.24562220582793));
#23645=CARTESIAN_POINT('Ctrl Pts',(-16.9725307779978,-35.3303080462616,
6.16982677025167));
#23646=CARTESIAN_POINT('Ctrl Pts',(-17.362606486713,-36.700289972122,9.0940313346754));
#23647=CARTESIAN_POINT('Ctrl Pts',(-18.2218132452327,-39.097525607069,11.1176436806954));
#23648=CARTESIAN_POINT('Ctrl Pts',(-19.0810200037525,-41.4947612420161,
13.1412560267153));
#23649=CARTESIAN_POINT('Ctrl Pts',(-20.2005748533759,-44.4620796765377,
13.8634749112255));
#23650=CARTESIAN_POINT('Ctrl Pts',(-21.3201297029994,-47.4293981110593,
14.5856937957357));
#23651=CARTESIAN_POINT('Ctrl Pts',(-22.4396845526228,-50.3967165455809,
13.8634749112255));
#23652=CARTESIAN_POINT('',(-15.5074469599351,-33.9565603202878,7.60754902664041E-30));
#23653=CARTESIAN_POINT('Origin',(-16.2551894587639,-35.5938999782223,0.));
#23654=CARTESIAN_POINT('Origin',(-16.2551894587639,-35.5938999782223,0.));
#23655=CARTESIAN_POINT('Ctrl Pts',(-21.4269965203142,-31.1388779521429,
0.));
#23656=CARTESIAN_POINT('Ctrl Pts',(-21.246727906136,-31.2547295558833,3.24562220582792));
#23657=CARTESIAN_POINT('Ctrl Pts',(-21.8278019627954,-32.5552534796891,
6.16982677025168));
#23658=CARTESIAN_POINT('Ctrl Pts',(-22.4088760194547,-33.8557774034949,
9.09403133467542));
#23659=CARTESIAN_POINT('Ctrl Pts',(-23.600499493737,-36.1063347653245,11.1176436806954));
#23660=CARTESIAN_POINT('Ctrl Pts',(-24.7921229680193,-38.356892127154,13.1412560267153));
#23661=CARTESIAN_POINT('Ctrl Pts',(-26.3225758066526,-41.1346782711698,
13.8634749112255));
#23662=CARTESIAN_POINT('Ctrl Pts',(-27.853028645286,-43.9124644151856,14.5856937957357));
#23663=CARTESIAN_POINT('Ctrl Pts',(-29.3834814839194,-46.6902505592015,
13.8634749112255));
#23664=CARTESIAN_POINT('Ctrl Pts',(-22.9590519566755,-32.9490709821975,
0.));
#23665=CARTESIAN_POINT('Ctrl Pts',(-22.7787833424974,-33.064922585938,2.7089937269807));
#23666=CARTESIAN_POINT('Ctrl Pts',(-23.2339776345312,-34.1695737726435,
5.14971273833323));
#23667=CARTESIAN_POINT('Ctrl Pts',(-23.689171926565,-35.2742249593489,7.59043174968578));
#23668=CARTESIAN_POINT('Ctrl Pts',(-24.6539679027943,-37.1718318447821,
9.27946171175752));
#23669=CARTESIAN_POINT('Ctrl Pts',(-25.6187638790236,-39.0694387302152,
10.9684916738293));
#23670=CARTESIAN_POINT('Ctrl Pts',(-26.8663674540227,-41.4071028290423,
11.5712994880388));
#23671=CARTESIAN_POINT('Ctrl Pts',(-28.1139710290218,-43.7447669278694,
12.1741073022483));
#23672=CARTESIAN_POINT('Ctrl Pts',(-29.3615746040208,-46.0824310266965,
11.5712994880388));
#23673=CARTESIAN_POINT('Ctrl Pts',(-24.814824624701,-34.4255873115188,0.));
#23674=CARTESIAN_POINT('Ctrl Pts',(-24.6345560105229,-34.5414389152593,
2.19648874705823));
#23675=CARTESIAN_POINT('Ctrl Pts',(-24.969529313949,-35.4590225922221,4.17545672685568));
#23676=CARTESIAN_POINT('Ctrl Pts',(-25.3045026173751,-36.3766062691848,
6.15442470665313));
#23677=CARTESIAN_POINT('Ctrl Pts',(-26.0526678575965,-37.9371291496696,
7.5239130403414));
#23678=CARTESIAN_POINT('Ctrl Pts',(-26.8008330978179,-39.4976520301544,
8.89340137402968));
#23679=CARTESIAN_POINT('Ctrl Pts',(-27.7783025634768,-41.4149792500715,
9.3821661014496));
#23680=CARTESIAN_POINT('Ctrl Pts',(-28.7557720291356,-43.3323064699886,
9.87093082886954));
#23681=CARTESIAN_POINT('Ctrl Pts',(-29.7332414947946,-45.2496336899057,
9.3821661014496));
#23682=CARTESIAN_POINT('Ctrl Pts',(-26.9229962078199,-35.5116836434676,
0.));
#23683=CARTESIAN_POINT('Ctrl Pts',(-26.7427275936418,-35.6275352472081,
1.72780310113343));
#23684=CARTESIAN_POINT('Ctrl Pts',(-26.9677588400993,-36.3740457442604,
3.28449990511992));
#23685=CARTESIAN_POINT('Ctrl Pts',(-27.1927900865569,-37.1205562413127,
4.84119670910638));
#23686=CARTESIAN_POINT('Ctrl Pts',(-27.7428465855746,-38.3728159033327,
5.91846432228298));
#23687=CARTESIAN_POINT('Ctrl Pts',(-28.2929030845924,-39.6250755653527,
6.99573193545956));
#23688=CARTESIAN_POINT('Ctrl Pts',(-29.0233349906522,-41.1580048392678,
7.38020429521639));
#23689=CARTESIAN_POINT('Ctrl Pts',(-29.753766896712,-42.690934113183,7.76467665497321));
#23690=CARTESIAN_POINT('Ctrl Pts',(-30.4841988027718,-44.2238633870982,
7.38020429521638));
#23691=CARTESIAN_POINT('',(-21.4269965203187,-31.1388779521589,1.57949798001058E-9));
#23692=CARTESIAN_POINT('Origin',(-35.1666259835202,-19.5103534449751,0.));
#23693=CARTESIAN_POINT('Ctrl Pts',(-21.4269965201955,-31.1388779523199,
3.13107077675564E-9));
#23694=CARTESIAN_POINT('Ctrl Pts',(-21.4133865912302,-31.14762452263,0.245038153335643));
#23695=CARTESIAN_POINT('Ctrl Pts',(-21.4030831299566,-31.1617800116156,
0.49079116052204));
#23696=CARTESIAN_POINT('Ctrl Pts',(-21.3961588156768,-31.1813997562909,
0.736766500725851));
#23697=CARTESIAN_POINT('Ctrl Pts',(-21.389257233532,-31.2009550904461,0.981934317701482));
#23698=CARTESIAN_POINT('Ctrl Pts',(-21.3857127259201,-31.2259389327486,
1.22732257376611));
#23699=CARTESIAN_POINT('Ctrl Pts',(-21.3855711085673,-31.2563626765479,
1.47243294816386));
#23700=CARTESIAN_POINT('Ctrl Pts',(-21.385429704495,-31.2867406011578,1.71717417803062));
#23701=CARTESIAN_POINT('Ctrl Pts',(-21.388680999235,-31.3225420796899,1.96163791541631));
#23702=CARTESIAN_POINT('Ctrl Pts',(-21.3953435107757,-31.363734369177,2.2053240877857));
#23703=CARTESIAN_POINT('Ctrl Pts',(-21.4020003082054,-31.4048913300483,
2.4488012624211));
#23704=CARTESIAN_POINT('Ctrl Pts',(-21.4120624904153,-31.4514298295104,
2.69150175431092));
#23705=CARTESIAN_POINT('Ctrl Pts',(-21.4255209532439,-31.5032731891,2.93292951866849));
#23706=CARTESIAN_POINT('Ctrl Pts',(-21.4389766005352,-31.5551057029553,
3.17430677585639));
#23707=CARTESIAN_POINT('Ctrl Pts',(-21.4558270899206,-31.6122407735689,
3.41441139318401));
#23708=CARTESIAN_POINT('Ctrl Pts',(-21.4760357504366,-31.6745585953924,
3.65275710614701));
#23709=CARTESIAN_POINT('Ctrl Pts',(-21.4962700715869,-31.7369555473905,
3.89140546668857));
#23710=CARTESIAN_POINT('Ctrl Pts',(-21.5198710494326,-31.8045482893659,
4.12829002081237));
#23711=CARTESIAN_POINT('Ctrl Pts',(-21.546774712017,-31.877174873993,4.36293874377885));
#23712=CARTESIAN_POINT('Ctrl Pts',(-21.5737058270658,-31.9498755666981,
4.5978269020151));
#23713=CARTESIAN_POINT('Ctrl Pts',(-21.6039462850732,-32.0276201924313,
4.83047425895007));
#23714=CARTESIAN_POINT('Ctrl Pts',(-21.6374057246246,-32.1102069701887,
5.06042975959465));
#23715=CARTESIAN_POINT('Ctrl Pts',(-21.6709629864615,-32.1930351993112,
5.29105755998335));
#23716=CARTESIAN_POINT('Ctrl Pts',(-21.7077579677309,-32.280733707951,5.51897736305714));
#23717=CARTESIAN_POINT('Ctrl Pts',(-21.7476746505214,-32.3730624995606,
5.74376259354354));
#23718=CARTESIAN_POINT('Ctrl Pts',(-21.7731267144332,-32.4319340825843,
5.88709234072634));
#23719=CARTESIAN_POINT('Ctrl Pts',(-21.7998474764587,-32.4926874816773,
6.029148253142));
#23720=CARTESIAN_POINT('Ctrl Pts',(-21.8278019628186,-32.5552534797158,
6.16982677023484));
#23721=CARTESIAN_POINT('Ctrl Pts',(-21.8716354197709,-32.6533588051506,
6.39041482339092));
#23722=CARTESIAN_POINT('Ctrl Pts',(-21.9185984820905,-32.756597406632,6.60890054011809));
#23723=CARTESIAN_POINT('Ctrl Pts',(-21.9686438281945,-32.8648380414542,
6.82480412008047));
#23724=CARTESIAN_POINT('Ctrl Pts',(-22.0185761941209,-32.972834316968,7.04022028559303));
#23725=CARTESIAN_POINT('Ctrl Pts',(-22.0715769175146,-33.0858099774485,
7.25306552029652));
#23726=CARTESIAN_POINT('Ctrl Pts',(-22.1275730571501,-33.2035915933472,
7.46287566269437));
#23727=CARTESIAN_POINT('Ctrl Pts',(-22.1834791320502,-33.3211837681497,
7.67234834441909));
#23728=CARTESIAN_POINT('Ctrl Pts',(-22.2423709378485,-33.4435663083135,
7.87879526533063));
#23729=CARTESIAN_POINT('Ctrl Pts',(-22.3041506139772,-33.5705253659799,
8.08177334612238));
#23730=CARTESIAN_POINT('Ctrl Pts',(-22.3658710102834,-33.6973626018617,
8.28455666214124));
#23731=CARTESIAN_POINT('Ctrl Pts',(-22.430473648954,-33.8287673834107,8.4838773927284));
#23732=CARTESIAN_POINT('Ctrl Pts',(-22.4978367992944,-33.9644877838652,
8.67931873611054));
#23733=CARTESIAN_POINT('Ctrl Pts',(-22.5652031896243,-34.1002147121119,
8.87476947970437));
#23734=CARTESIAN_POINT('Ctrl Pts',(-22.635330240365,-34.2402574360607,9.0663400953276));
#23735=CARTESIAN_POINT('Ctrl Pts',(-22.70807357429,-34.3843285090689,9.25364450340901));
#23736=CARTESIAN_POINT('Ctrl Pts',(-22.7808435933891,-34.5284524331283,
9.44101762226399));
#23737=CARTESIAN_POINT('Ctrl Pts',(-22.8562316704646,-34.6766073801526,
9.62412107874924));
#23738=CARTESIAN_POINT('Ctrl Pts',(-22.9340725908145,-34.8284739876038,
9.80260437466002));
#23739=CARTESIAN_POINT('Ctrl Pts',(-23.0120404858285,-34.9805883209477,
9.98137881379545));
#23740=CARTESIAN_POINT('Ctrl Pts',(-23.0924690655294,-35.13642611801,10.155517727091));
#23741=CARTESIAN_POINT('Ctrl Pts',(-23.1751739070328,-35.2956392414801,
10.3247095747693));
#23742=CARTESIAN_POINT('Ctrl Pts',(-23.1990784057277,-35.3416572234148,
10.3736117457728));
#23743=CARTESIAN_POINT('Ctrl Pts',(-23.223172956478,-35.3879570256956,10.4221009095719));
#23744=CARTESIAN_POINT('Ctrl Pts',(-23.2474528526981,-35.4345298797237,
10.4701702229062));
#23745=CARTESIAN_POINT('Ctrl Pts',(-21.1183468312847,-39.2421052839112,
0.));
#23746=CARTESIAN_POINT('Ctrl Pts',(-20.9380782171066,-39.3579568876517,
1.72780310113342));
#23747=CARTESIAN_POINT('Ctrl Pts',(-21.1631094635642,-40.104467384704,3.28449990511991));
#23748=CARTESIAN_POINT('Ctrl Pts',(-21.3881407100217,-40.8509778817563,
4.84119670910639));
#23749=CARTESIAN_POINT('Ctrl Pts',(-21.9381972090395,-42.1032375437763,
5.91846432228299));
#23750=CARTESIAN_POINT('Ctrl Pts',(-22.4882537080573,-43.3554972057963,
6.99573193545957));
#23751=CARTESIAN_POINT('Ctrl Pts',(-23.218685614117,-44.8884264797115,7.3802042952164));
#23752=CARTESIAN_POINT('Ctrl Pts',(-23.9491175201768,-46.4213557536267,
7.76467665497322));
#23753=CARTESIAN_POINT('Ctrl Pts',(-24.6795494262366,-47.9542850275418,
7.38020429521639));
#23754=CARTESIAN_POINT('Ctrl Pts',(-21.0061649833184,-36.8732642383513,
0.));
#23755=CARTESIAN_POINT('Ctrl Pts',(-20.8258963691403,-36.9891158420918,
2.19648874705823));
#23756=CARTESIAN_POINT('Ctrl Pts',(-21.1608696725665,-37.9066995190545,
4.17545672685567));
#23757=CARTESIAN_POINT('Ctrl Pts',(-21.4958429759926,-38.8242831960173,
6.15442470665314));
#23758=CARTESIAN_POINT('Ctrl Pts',(-22.244008216214,-40.3848060765021,7.5239130403414));
#23759=CARTESIAN_POINT('Ctrl Pts',(-22.9921734564354,-41.9453289569869,
8.89340137402967));
#23760=CARTESIAN_POINT('Ctrl Pts',(-23.9696429220943,-43.862656176904,9.38216610144961));
#23761=CARTESIAN_POINT('Ctrl Pts',(-24.9471123877531,-45.7799833968211,
9.87093082886954));
#23762=CARTESIAN_POINT('Ctrl Pts',(-25.924581853412,-47.6973106167382,9.3821661014496));
#23763=CARTESIAN_POINT('Ctrl Pts',(-20.4339943155208,-34.5718269932684,
0.));
#23764=CARTESIAN_POINT('Ctrl Pts',(-20.2537257013426,-34.6876785970089,
2.70899372698069));
#23765=CARTESIAN_POINT('Ctrl Pts',(-20.7089199933764,-35.7923297837143,
5.14971273833323));
#23766=CARTESIAN_POINT('Ctrl Pts',(-21.1641142854102,-36.8969809704198,
7.59043174968578));
#23767=CARTESIAN_POINT('Ctrl Pts',(-22.1289102616396,-38.7945878558529,
9.27946171175752));
#23768=CARTESIAN_POINT('Ctrl Pts',(-23.0937062378689,-40.6921947412861,
10.9684916738293));
#23769=CARTESIAN_POINT('Ctrl Pts',(-24.341309812868,-43.0298588401132,11.5712994880388));
#23770=CARTESIAN_POINT('Ctrl Pts',(-25.588913387867,-45.3675229389403,12.1741073022483));
#23771=CARTESIAN_POINT('Ctrl Pts',(-26.8365169628661,-47.7051870377674,
11.5712994880388));
#23772=CARTESIAN_POINT('Ctrl Pts',(-19.4238236466309,-32.4262389885812,
0.));
#23773=CARTESIAN_POINT('Ctrl Pts',(-19.2435550324528,-32.5420905923217,
3.24562220582793));
#23774=CARTESIAN_POINT('Ctrl Pts',(-19.8246290891121,-33.8426145161275,
6.16982677025168));
#23775=CARTESIAN_POINT('Ctrl Pts',(-20.4057031457714,-35.1431384399332,
9.09403133467541));
#23776=CARTESIAN_POINT('Ctrl Pts',(-21.5973266200537,-37.3936958017628,
11.1176436806954));
#23777=CARTESIAN_POINT('Ctrl Pts',(-22.788950094336,-39.6442531635924,13.1412560267153));
#23778=CARTESIAN_POINT('Ctrl Pts',(-24.3194029329694,-42.4220393076082,
13.8634749112255));
#23779=CARTESIAN_POINT('Ctrl Pts',(-25.8498557716028,-45.199825451624,14.5856937957357));
#23780=CARTESIAN_POINT('Ctrl Pts',(-27.3803086102361,-47.9776115956398,
13.8634749112255));
#23781=CARTESIAN_POINT('',(-19.4238236466309,-32.4262389885812,0.));
#23782=CARTESIAN_POINT('Ctrl Pts',(-19.4238236466309,-32.4262389885812,
0.));
#23783=CARTESIAN_POINT('Ctrl Pts',(-19.2435550324528,-32.5420905923217,
3.24562220582793));
#23784=CARTESIAN_POINT('Ctrl Pts',(-19.8246290891121,-33.8426145161275,
6.16982677025168));
#23785=CARTESIAN_POINT('Ctrl Pts',(-20.3097318100837,-34.9283413471513,
8.61106394926976));
#23786=CARTESIAN_POINT('Ctrl Pts',(-21.2335670650398,-36.7013364119537,
10.4489096280657));
#23787=CARTESIAN_POINT('Origin',(-3.13849734404819,-40.0935818932913,0.));
#23788=CARTESIAN_POINT('Ctrl Pts',(-19.4238236466309,-32.4262389885812,
0.));
#23789=CARTESIAN_POINT('Ctrl Pts',(-19.2435550324528,-32.5420905923217,
3.24562220582793));
#23790=CARTESIAN_POINT('Ctrl Pts',(-19.8246290891121,-33.8426145161275,
6.16982677025168));
#23791=CARTESIAN_POINT('Ctrl Pts',(-20.4057031457715,-35.1431384399332,
9.09403133467541));
#23792=CARTESIAN_POINT('Ctrl Pts',(-21.5973266200537,-37.3936958017628,
11.1176436806954));
#23793=CARTESIAN_POINT('Ctrl Pts',(-22.7889500943361,-39.6442531635924,
13.1412560267153));
#23794=CARTESIAN_POINT('Ctrl Pts',(-24.3194029329694,-42.4220393076082,
13.8634749112255));
#23795=CARTESIAN_POINT('Ctrl Pts',(-25.8498557716028,-45.199825451624,14.5856937957357));
#23796=CARTESIAN_POINT('Ctrl Pts',(-27.3803086102362,-47.9776115956398,
13.8634749112255));
#23797=CARTESIAN_POINT('Ctrl Pts',(-19.6841717937389,-31.5100409519661,
6.24500451351651E-15));
#23798=CARTESIAN_POINT('Ctrl Pts',(-19.5039031795608,-31.6258925557066,
3.38941559469372));
#23799=CARTESIAN_POINT('Ctrl Pts',(-20.1187076077129,-32.9789019620468,
6.44317352589573));
#23800=CARTESIAN_POINT('Ctrl Pts',(-20.733512035865,-34.3319113683871,9.49693145709774));
#23801=CARTESIAN_POINT('Ctrl Pts',(-21.9859155393829,-36.6770443017776,
11.6101975146502));
#23802=CARTESIAN_POINT('Ctrl Pts',(-23.2383190429008,-39.0221772351682,
13.7234635722027));
#23803=CARTESIAN_POINT('Ctrl Pts',(-24.8445633383042,-41.9178971879303,
14.4776794959001));
#23804=CARTESIAN_POINT('Ctrl Pts',(-26.4508076337078,-44.8136171406925,
15.2318954195974));
#23805=CARTESIAN_POINT('Ctrl Pts',(-28.0570519291113,-47.7093370934547,
14.4776794959001));
#23806=CARTESIAN_POINT('Ctrl Pts',(-20.4854409432122,-30.9950965373907,
6.24500451351651E-15));
#23807=CARTESIAN_POINT('Ctrl Pts',(-20.3051723290341,-31.1109481411312,
3.38941559469371));
#23808=CARTESIAN_POINT('Ctrl Pts',(-20.9199767571862,-32.4639575474715,
6.44317352589574));
#23809=CARTESIAN_POINT('Ctrl Pts',(-21.5347811853383,-33.8169669538118,
9.49693145709774));
#23810=CARTESIAN_POINT('Ctrl Pts',(-22.7871846888562,-36.1620998872023,
11.6101975146502));
#23811=CARTESIAN_POINT('Ctrl Pts',(-24.0395881923741,-38.5072328205928,
13.7234635722027));
#23812=CARTESIAN_POINT('Ctrl Pts',(-25.6458324877776,-41.402952773355,14.4776794959001));
#23813=CARTESIAN_POINT('Ctrl Pts',(-27.2520767831811,-44.2986727261172,
15.2318954195974));
#23814=CARTESIAN_POINT('Ctrl Pts',(-28.8583210785846,-47.1943926788794,
14.4776794959001));
#23815=CARTESIAN_POINT('Ctrl Pts',(-21.4269965203142,-31.1388779521429,
0.));
#23816=CARTESIAN_POINT('Ctrl Pts',(-21.246727906136,-31.2547295558833,3.24562220582792));
#23817=CARTESIAN_POINT('Ctrl Pts',(-21.8278019627954,-32.5552534796891,
6.16982677025168));
#23818=CARTESIAN_POINT('Ctrl Pts',(-22.4088760194547,-33.8557774034949,
9.09403133467542));
#23819=CARTESIAN_POINT('Ctrl Pts',(-23.600499493737,-36.1063347653245,11.1176436806954));
#23820=CARTESIAN_POINT('Ctrl Pts',(-24.7921229680193,-38.356892127154,13.1412560267153));
#23821=CARTESIAN_POINT('Ctrl Pts',(-26.3225758066526,-41.1346782711698,
13.8634749112255));
#23822=CARTESIAN_POINT('Ctrl Pts',(-27.853028645286,-43.9124644151856,14.5856937957357));
#23823=CARTESIAN_POINT('Ctrl Pts',(-29.3834814839194,-46.6902505592015,
13.8634749112255));
#23824=CARTESIAN_POINT('',(-20.1821259000655,-31.4039916914148,5.03628278864507E-30));
#23825=CARTESIAN_POINT('Origin',(-21.1552751870376,-32.9182507396841,0.));
#23826=CARTESIAN_POINT('Origin',(-21.1552751870376,-32.9182507396841,0.));
#23827=CARTESIAN_POINT('Ctrl Pts',(-25.6404249706859,-27.7725495286737,
0.));
#23828=CARTESIAN_POINT('Ctrl Pts',(-25.4784786333242,-27.9128768288048,
3.24562220582792));
#23829=CARTESIAN_POINT('Ctrl Pts',(-26.2387220458134,-29.1174678338686,
6.16982677025167));
#23830=CARTESIAN_POINT('Ctrl Pts',(-26.9989654583024,-30.3220588389324,
9.09403133467541));
#23831=CARTESIAN_POINT('Ctrl Pts',(-28.4987476307692,-32.3801230698292,
11.1176436806954));
#23832=CARTESIAN_POINT('Ctrl Pts',(-29.998529803236,-34.4381873007259,13.1412560267153));
#23833=CARTESIAN_POINT('Ctrl Pts',(-31.9087250245462,-36.9698934388175,
13.8634749112255));
#23834=CARTESIAN_POINT('Ctrl Pts',(-33.8189202458565,-39.5015995769091,
14.5856937957357));
#23835=CARTESIAN_POINT('Ctrl Pts',(-35.7291154671667,-42.0333057150007,
13.8634749112255));
#23836=CARTESIAN_POINT('Ctrl Pts',(-27.4145036200622,-29.3462831821137,
0.));
#23837=CARTESIAN_POINT('Ctrl Pts',(-27.2525572827006,-29.4866104822448,
2.70899372698068));
#23838=CARTESIAN_POINT('Ctrl Pts',(-27.8603266081618,-30.5152370105914,
5.14971273833322));
#23839=CARTESIAN_POINT('Ctrl Pts',(-28.4680959336231,-31.543863538938,7.59043174968577));
#23840=CARTESIAN_POINT('Ctrl Pts',(-29.693129294942,-33.2848507390768,9.27946171175751));
#23841=CARTESIAN_POINT('Ctrl Pts',(-30.9181626562609,-35.0258379392156,
10.9684916738293));
#23842=CARTESIAN_POINT('Ctrl Pts',(-32.4857517139242,-37.1621554871448,
11.5712994880388));
#23843=CARTESIAN_POINT('Ctrl Pts',(-34.0533407715874,-39.298473035074,12.1741073022483));
#23844=CARTESIAN_POINT('Ctrl Pts',(-35.6209298292506,-41.4347905830031,
11.5712994880388));
#23845=CARTESIAN_POINT('Ctrl Pts',(-29.4615173807456,-30.5436667170412,
0.));
#23846=CARTESIAN_POINT('Ctrl Pts',(-29.299571043384,-30.6839940171723,2.19648874705824));
#23847=CARTESIAN_POINT('Ctrl Pts',(-29.761720574162,-31.5445663438471,4.17545672685568));
#23848=CARTESIAN_POINT('Ctrl Pts',(-30.2238701049401,-32.4051386705218,
6.15442470665313));
#23849=CARTESIAN_POINT('Ctrl Pts',(-31.1865056631392,-33.8433026630077,
7.5239130403414));
#23850=CARTESIAN_POINT('Ctrl Pts',(-32.1491412213383,-35.2814666554935,
8.89340137402967));
#23851=CARTESIAN_POINT('Ctrl Pts',(-33.3895255704508,-37.0401698399471,
9.3821661014496));
#23852=CARTESIAN_POINT('Ctrl Pts',(-34.6299099195633,-38.7988730244007,
9.87093082886953));
#23853=CARTESIAN_POINT('Ctrl Pts',(-35.8702942686759,-40.5575762088543,
9.3821661014496));
#23854=CARTESIAN_POINT('Ctrl Pts',(-31.7027984407113,-31.3186840564485,
1.04083408558608E-14));
#23855=CARTESIAN_POINT('Ctrl Pts',(-31.5408521033497,-31.4590113565796,
1.72780310113343));
#23856=CARTESIAN_POINT('Ctrl Pts',(-31.8698323768439,-32.1658981677051,
3.28449990511992));
#23857=CARTESIAN_POINT('Ctrl Pts',(-32.1988126503381,-32.8727849788306,
4.84119670910638));
#23858=CARTESIAN_POINT('Ctrl Pts',(-32.9214854985883,-34.0340172414017,
5.91846432228298));
#23859=CARTESIAN_POINT('Ctrl Pts',(-33.6441583468386,-35.1952495039728,
6.99573193545955));
#23860=CARTESIAN_POINT('Ctrl Pts',(-34.5853140909922,-36.6086244696004,
7.38020429521639));
#23861=CARTESIAN_POINT('Ctrl Pts',(-35.5264698351457,-38.0219994352281,
7.76467665497322));
#23862=CARTESIAN_POINT('Ctrl Pts',(-36.4676255792993,-39.4353744008558,
7.38020429521639));
#23863=CARTESIAN_POINT('',(-25.6404249706926,-27.7725495286889,1.57950248445926E-9));
#23864=CARTESIAN_POINT('Origin',(-37.5852932322717,-14.3070334890501,0.));
#23865=CARTESIAN_POINT('Ctrl Pts',(-25.6404249705937,-27.7725495288658,
3.13107430880991E-9));
#23866=CARTESIAN_POINT('Ctrl Pts',(-25.6281983378204,-27.7831439665413,
0.245038153335578));
#23867=CARTESIAN_POINT('Ctrl Pts',(-25.6200142870519,-27.7986217084844,
0.490791160521907));
#23868=CARTESIAN_POINT('Ctrl Pts',(-25.6159526330979,-27.819027185115,0.736766500725649));
#23869=CARTESIAN_POINT('Ctrl Pts',(-25.6119043133257,-27.8393656717118,
0.981934317701287));
#23870=CARTESIAN_POINT('Ctrl Pts',(-25.6119514551673,-27.8645996505509,
1.22732257376593));
#23871=CARTESIAN_POINT('Ctrl Pts',(-25.6161410294534,-27.8947338787563,
1.47243294816368));
#23872=CARTESIAN_POINT('Ctrl Pts',(-25.6203242940986,-27.9248227237928,
1.71717417803043));
#23873=CARTESIAN_POINT('Ctrl Pts',(-25.6286375769734,-27.9597970874098,
1.96163791541611));
#23874=CARTESIAN_POINT('Ctrl Pts',(-25.6410945477695,-27.9996219245319,
2.20532408778548));
#23875=CARTESIAN_POINT('Ctrl Pts',(-25.6535408348299,-28.0394126058353,
2.44880126242092));
#23876=CARTESIAN_POINT('Ctrl Pts',(-25.6701237175578,-28.084045412642,2.69150175431078));
#23877=CARTESIAN_POINT('Ctrl Pts',(-25.6908232719758,-28.1334457426221,
2.93292951866838));
#23878=CARTESIAN_POINT('Ctrl Pts',(-25.7115184960058,-28.1828357379546,
3.17430677585629));
#23879=CARTESIAN_POINT('Ctrl Pts',(-25.7363286400398,-28.2369911812595,
3.41441139318393));
#23880=CARTESIAN_POINT('Ctrl Pts',(-25.7652003562646,-28.2957987052587,
3.65275710614695));
#23881=CARTESIAN_POINT('Ctrl Pts',(-25.7941087333334,-28.3546809021123,
3.89140546668845));
#23882=CARTESIAN_POINT('Ctrl Pts',(-25.8270889373971,-28.4182268780899,
4.12829002081219));
#23883=CARTESIAN_POINT('Ctrl Pts',(-25.8640546001338,-28.4862854384147,
4.36293874377862));
#23884=CARTESIAN_POINT('Ctrl Pts',(-25.9010579825875,-28.5544134456112,
4.59782690201492));
#23885=CARTESIAN_POINT('Ctrl Pts',(-25.9420548501734,-28.6270630772623,
4.83047425894992));
#23886=CARTESIAN_POINT('Ctrl Pts',(-25.9869270447948,-28.7040474659739,
5.06042975959454));
#23887=CARTESIAN_POINT('Ctrl Pts',(-26.0319304281238,-28.7812569268612,
5.2910575599833));
#23888=CARTESIAN_POINT('Ctrl Pts',(-26.0808316886117,-28.8628263193252,
5.51897736305715));
#23889=CARTESIAN_POINT('Ctrl Pts',(-26.1334818341725,-28.9485346007076,
5.74376259354361));
#23890=CARTESIAN_POINT('Ctrl Pts',(-26.1670531325893,-29.0031847495427,
5.88709234072639));
#23891=CARTESIAN_POINT('Ctrl Pts',(-26.2021480259521,-29.0595170057058,
6.02914825314202));
#23892=CARTESIAN_POINT('Ctrl Pts',(-26.2387220458401,-29.1174678338917,
6.16982677023483));
#23893=CARTESIAN_POINT('Ctrl Pts',(-26.2960711849263,-29.2083364372326,
6.39041482339094));
#23894=CARTESIAN_POINT('Ctrl Pts',(-26.35724861586,-29.3038406779899,6.60890054011813));
#23895=CARTESIAN_POINT('Ctrl Pts',(-26.4221888209395,-29.4038573838826,
6.82480412008054));
#23896=CARTESIAN_POINT('Ctrl Pts',(-26.486982419861,-29.503648296448,7.04022028559293));
#23897=CARTESIAN_POINT('Ctrl Pts',(-26.5555217851613,-29.607931238224,7.25306552029626));
#23898=CARTESIAN_POINT('Ctrl Pts',(-26.6277100364533,-29.7165449255437,
7.46287566269394));
#23899=CARTESIAN_POINT('Ctrl Pts',(-26.6997821794599,-29.8249839175527,
7.6723483444186));
#23900=CARTESIAN_POINT('Ctrl Pts',(-26.7754914030011,-29.9377396021008,
7.87879526533007));
#23901=CARTESIAN_POINT('Ctrl Pts',(-26.8547104088648,-30.0546142350031,
8.08177334612175));
#23902=CARTESIAN_POINT('Ctrl Pts',(-26.9338534012417,-30.1713767224895,
8.2845566621408));
#23903=CARTESIAN_POINT('Ctrl Pts',(-27.0164993284344,-30.292250078758,8.48387739272815));
#23904=CARTESIAN_POINT('Ctrl Pts',(-27.1024918458752,-30.4170022653823,
8.67931873611046));
#23905=CARTESIAN_POINT('Ctrl Pts',(-27.1884884993286,-30.5417604522568,
8.87476947970436));
#23906=CARTESIAN_POINT('Ctrl Pts',(-27.2778319154178,-30.670397623316,9.06634009532763));
#23907=CARTESIAN_POINT('Ctrl Pts',(-27.3703382785457,-30.8026498047313,
9.2536445034091));
#23908=CARTESIAN_POINT('Ctrl Pts',(-27.46287857672,-30.9349505015543,9.44101762226428));
#23909=CARTESIAN_POINT('Ctrl Pts',(-27.5585839591968,-31.0708686028431,
9.62412107874973));
#23910=CARTESIAN_POINT('Ctrl Pts',(-27.6572454428935,-31.2101115092135,
9.80260437466071));
#23911=CARTESIAN_POINT('Ctrl Pts',(-27.7560678639057,-31.3495815496055,
9.98137881379635));
#23912=CARTESIAN_POINT('Ctrl Pts',(-27.8578558275196,-31.4923869622807,
10.1555177270921));
#23913=CARTESIAN_POINT('Ctrl Pts',(-27.9623772429048,-31.6382093995775,
10.3247095747706));
#23914=CARTESIAN_POINT('Ctrl Pts',(-27.992587469928,-31.6803570199438,10.3736117457754));
#23915=CARTESIAN_POINT('Ctrl Pts',(-28.0230259217676,-31.722756544904,10.4221009095756));
#23916=CARTESIAN_POINT('Ctrl Pts',(-28.0536866918425,-31.7653999649279,
10.4701702229111));
#23917=CARTESIAN_POINT('Ctrl Pts',(-26.4881263776669,-35.8372231206709,
1.04083408558608E-14));
#23918=CARTESIAN_POINT('Ctrl Pts',(-26.3261800403053,-35.9775504208021,
1.72780310113342));
#23919=CARTESIAN_POINT('Ctrl Pts',(-26.6551603137995,-36.6844372319276,
3.28449990511991));
#23920=CARTESIAN_POINT('Ctrl Pts',(-26.9841405872937,-37.3913240430531,
4.84119670910638));
#23921=CARTESIAN_POINT('Ctrl Pts',(-27.706813435544,-38.5525563056242,5.91846432228298));
#23922=CARTESIAN_POINT('Ctrl Pts',(-28.4294862837942,-39.7137885681952,
6.99573193545957));
#23923=CARTESIAN_POINT('Ctrl Pts',(-29.3706420279478,-41.1271635338229,
7.38020429521639));
#23924=CARTESIAN_POINT('Ctrl Pts',(-30.3117977721014,-42.5405384994506,
7.76467665497322));
#23925=CARTESIAN_POINT('Ctrl Pts',(-31.2529535162549,-43.9539134650783,
7.3802042952164));
#23926=CARTESIAN_POINT('Ctrl Pts',(-26.0399651488661,-33.5084586029185,
0.));
#23927=CARTESIAN_POINT('Ctrl Pts',(-25.8780188115045,-33.6487859030497,
2.19648874705823));
#23928=CARTESIAN_POINT('Ctrl Pts',(-26.3401683422825,-34.5093582297245,
4.17545672685567));
#23929=CARTESIAN_POINT('Ctrl Pts',(-26.8023178730605,-35.3699305563992,
6.15442470665314));
#23930=CARTESIAN_POINT('Ctrl Pts',(-27.7649534312596,-36.808094548885,7.5239130403414));
#23931=CARTESIAN_POINT('Ctrl Pts',(-28.7275889894587,-38.2462585413709,
8.89340137402967));
#23932=CARTESIAN_POINT('Ctrl Pts',(-29.9679733385713,-40.0049617258244,
9.3821661014496));
#23933=CARTESIAN_POINT('Ctrl Pts',(-31.2083576876838,-41.763664910278,9.87093082886954));
#23934=CARTESIAN_POINT('Ctrl Pts',(-32.4487420367963,-43.5223680947316,
9.3821661014496));
#23935=CARTESIAN_POINT('Ctrl Pts',(-25.1460896841345,-31.3118750466445,
-1.05434036998093E-14));
#23936=CARTESIAN_POINT('Ctrl Pts',(-24.9841433467729,-31.4522023467756,
2.70899372698069));
#23937=CARTESIAN_POINT('Ctrl Pts',(-25.5919126722341,-32.4808288751222,
5.14971273833323));
#23938=CARTESIAN_POINT('Ctrl Pts',(-26.1996819976954,-33.5094554034687,
7.59043174968578));
#23939=CARTESIAN_POINT('Ctrl Pts',(-27.4247153590143,-35.2504426036076,
9.27946171175751));
#23940=CARTESIAN_POINT('Ctrl Pts',(-28.6497487203333,-36.9914298037464,
10.9684916738292));
#23941=CARTESIAN_POINT('Ctrl Pts',(-30.2173377779965,-39.1277473516756,
11.5712994880388));
#23942=CARTESIAN_POINT('Ctrl Pts',(-31.7849268356597,-41.2640648996047,
12.1741073022483));
#23943=CARTESIAN_POINT('Ctrl Pts',(-33.3525158933229,-43.4003824475339,
11.5712994880388));
#23944=CARTESIAN_POINT('Ctrl Pts',(-23.84085208622,-29.3318883095341,0.));
#23945=CARTESIAN_POINT('Ctrl Pts',(-23.6789057488584,-29.4722156096652,
3.24562220582792));
#23946=CARTESIAN_POINT('Ctrl Pts',(-24.4391491613475,-30.676806614729,6.16982677025168));
#23947=CARTESIAN_POINT('Ctrl Pts',(-25.1993925738366,-31.8813976197928,
9.09403133467541));
#23948=CARTESIAN_POINT('Ctrl Pts',(-26.6991747463034,-33.9394618506896,
11.1176436806954));
#23949=CARTESIAN_POINT('Ctrl Pts',(-28.1989569187702,-35.9975260815863,
13.1412560267153));
#23950=CARTESIAN_POINT('Ctrl Pts',(-30.1091521400804,-38.529232219678,13.8634749112255));
#23951=CARTESIAN_POINT('Ctrl Pts',(-32.0193473613906,-41.0609383577696,
14.5856937957357));
#23952=CARTESIAN_POINT('Ctrl Pts',(-33.9295425827008,-43.5926444958612,
13.8634749112255));
#23953=CARTESIAN_POINT('',(-23.84085208622,-29.3318883095341,0.));
#23954=CARTESIAN_POINT('Ctrl Pts',(-23.84085208622,-29.3318883095341,0.));
#23955=CARTESIAN_POINT('Ctrl Pts',(-23.6789057488584,-29.4722156096652,
3.24562220582792));
#23956=CARTESIAN_POINT('Ctrl Pts',(-24.4391491613475,-30.676806614729,6.16982677025167));
#23957=CARTESIAN_POINT('Ctrl Pts',(-25.0738292744461,-31.6824449968208,
8.61106394926976));
#23958=CARTESIAN_POINT('Ctrl Pts',(-26.2405847244738,-33.3059180634111,
10.4489096280657));
#23959=CARTESIAN_POINT('Origin',(-8.81246358936573,-39.2388322978495,1.04083408558608E-14));
#23960=CARTESIAN_POINT('Ctrl Pts',(-23.84085208622,-29.3318883095341,0.));
#23961=CARTESIAN_POINT('Ctrl Pts',(-23.6789057488584,-29.4722156096652,
3.24562220582792));
#23962=CARTESIAN_POINT('Ctrl Pts',(-24.4391491613475,-30.676806614729,6.16982677025167));
#23963=CARTESIAN_POINT('Ctrl Pts',(-25.1993925738366,-31.8813976197928,
9.09403133467541));
#23964=CARTESIAN_POINT('Ctrl Pts',(-26.6991747463034,-33.9394618506896,
11.1176436806954));
#23965=CARTESIAN_POINT('Ctrl Pts',(-28.1989569187702,-35.9975260815863,
13.1412560267153));
#23966=CARTESIAN_POINT('Ctrl Pts',(-30.1091521400804,-38.529232219678,13.8634749112255));
#23967=CARTESIAN_POINT('Ctrl Pts',(-32.0193473613906,-41.0609383577696,
14.5856937957357));
#23968=CARTESIAN_POINT('Ctrl Pts',(-33.9295425827008,-43.5926444958612,
13.8634749112255));
#23969=CARTESIAN_POINT('Ctrl Pts',(-23.9681616891742,-28.3879644434328,
6.24500451351651E-15));
#23970=CARTESIAN_POINT('Ctrl Pts',(-23.8062153518126,-28.5282917435639,
3.38941559469373));
#23971=CARTESIAN_POINT('Ctrl Pts',(-24.6073152722065,-29.780033672264,6.44317352589573));
#23972=CARTESIAN_POINT('Ctrl Pts',(-25.4084151926004,-31.031775600964,9.49693145709775));
#23973=CARTESIAN_POINT('Ctrl Pts',(-26.981818248414,-33.174802860439,11.6101975146502));
#23974=CARTESIAN_POINT('Ctrl Pts',(-28.5552213042276,-35.317830119914,13.7234635722027));
#23975=CARTESIAN_POINT('Ctrl Pts',(-30.557220265479,-37.9554834217127,14.4776794959001));
#23976=CARTESIAN_POINT('Ctrl Pts',(-32.5592192267304,-40.5931367235114,
15.2318954195974));
#23977=CARTESIAN_POINT('Ctrl Pts',(-34.5612181879818,-43.2307900253102,
14.4776794959001));
#23978=CARTESIAN_POINT('Ctrl Pts',(-24.6879908429606,-27.7642289310886,
0.));
#23979=CARTESIAN_POINT('Ctrl Pts',(-24.526044505599,-27.9045562312197,3.38941559469372));
#23980=CARTESIAN_POINT('Ctrl Pts',(-25.3271444259928,-29.1562981599198,
6.44317352589573));
#23981=CARTESIAN_POINT('Ctrl Pts',(-26.1282443463867,-30.4080400886198,
9.49693145709774));
#23982=CARTESIAN_POINT('Ctrl Pts',(-27.7016474022003,-32.5510673480948,
11.6101975146502));
#23983=CARTESIAN_POINT('Ctrl Pts',(-29.2750504580139,-34.6940946075698,
13.7234635722027));
#23984=CARTESIAN_POINT('Ctrl Pts',(-31.2770494192653,-37.3317479093686,
14.4776794959001));
#23985=CARTESIAN_POINT('Ctrl Pts',(-33.2790483805167,-39.9694012111673,
15.2318954195974));
#23986=CARTESIAN_POINT('Ctrl Pts',(-35.2810473417681,-42.607054512966,14.4776794959001));
#23987=CARTESIAN_POINT('Ctrl Pts',(-25.6404249706859,-27.7725495286737,
0.));
#23988=CARTESIAN_POINT('Ctrl Pts',(-25.4784786333242,-27.9128768288048,
3.24562220582792));
#23989=CARTESIAN_POINT('Ctrl Pts',(-26.2387220458134,-29.1174678338686,
6.16982677025167));
#23990=CARTESIAN_POINT('Ctrl Pts',(-26.9989654583024,-30.3220588389324,
9.09403133467541));
#23991=CARTESIAN_POINT('Ctrl Pts',(-28.4987476307692,-32.3801230698292,
11.1176436806954));
#23992=CARTESIAN_POINT('Ctrl Pts',(-29.998529803236,-34.4381873007259,13.1412560267153));
#23993=CARTESIAN_POINT('Ctrl Pts',(-31.9087250245462,-36.9698934388175,
13.8634749112255));
#23994=CARTESIAN_POINT('Ctrl Pts',(-33.8189202458565,-39.5015995769092,
14.5856937957357));
#23995=CARTESIAN_POINT('Ctrl Pts',(-35.7291154671667,-42.0333057150007,
13.8634749112255));
#23996=CARTESIAN_POINT('',(-24.4459549573119,-28.2121283533451,1.04083408558608E-14));
#23997=CARTESIAN_POINT('Origin',(-25.6247005192791,-29.5724808444821,1.04083408558608E-14));
#23998=CARTESIAN_POINT('Origin',(-25.6247005192791,-29.5724808444821,1.04083408558608E-14));
#23999=CARTESIAN_POINT('Ctrl Pts',(-29.3318883095342,-23.8408520862199,
0.));
#24000=CARTESIAN_POINT('Ctrl Pts',(-29.191561009403,-24.0027984235815,3.24562220582793));
#24001=CARTESIAN_POINT('Ctrl Pts',(-30.1154974142046,-25.0869345107939,
6.16982677025168));
#24002=CARTESIAN_POINT('Ctrl Pts',(-31.0394338190061,-26.1710705980062,
9.09403133467541));
#24003=CARTESIAN_POINT('Ctrl Pts',(-32.8168434496406,-27.9947454451963,
11.1176436806954));
#24004=CARTESIAN_POINT('Ctrl Pts',(-34.5942530802751,-29.8184202923863,
13.1412560267153));
#24005=CARTESIAN_POINT('Ctrl Pts',(-36.8453046181045,-32.0525081884198,
13.8634749112255));
#24006=CARTESIAN_POINT('Ctrl Pts',(-39.0963561559338,-34.2865960844532,
14.5856937957357));
#24007=CARTESIAN_POINT('Ctrl Pts',(-41.3474076937632,-36.5206839804867,
13.8634749112255));
#24008=CARTESIAN_POINT('Ctrl Pts',(-31.3118750466446,-25.1460896841344,
0.));
#24009=CARTESIAN_POINT('Ctrl Pts',(-31.1715477465134,-25.308036021496,2.70899372698069));
#24010=CARTESIAN_POINT('Ctrl Pts',(-31.9195196745978,-26.2396980216805,
5.14971273833323));
#24011=CARTESIAN_POINT('Ctrl Pts',(-32.667491602682,-27.171360021865,7.59043174968578));
#24012=CARTESIAN_POINT('Ctrl Pts',(-34.1278242025586,-28.7202860579072,
9.27946171175751));
#24013=CARTESIAN_POINT('Ctrl Pts',(-35.5881568024352,-30.2692120939494,
10.9684916738293));
#24014=CARTESIAN_POINT('Ctrl Pts',(-37.4438197501021,-32.1606938263359,
11.5712994880388));
#24015=CARTESIAN_POINT('Ctrl Pts',(-39.299482697769,-34.0521755587224,12.1741073022483));
#24016=CARTESIAN_POINT('Ctrl Pts',(-41.1551456454359,-35.9436572911088,
11.5712994880388));
#24017=CARTESIAN_POINT('Ctrl Pts',(-33.5084586029187,-26.039965148866,0.));
#24018=CARTESIAN_POINT('Ctrl Pts',(-33.3681313027876,-26.2019114862276,
2.19648874705822));
#24019=CARTESIAN_POINT('Ctrl Pts',(-33.9480490292,-26.9879536917289,4.17545672685568));
#24020=CARTESIAN_POINT('Ctrl Pts',(-34.5279667556125,-27.7739958972302,
6.15442470665313));
#24021=CARTESIAN_POINT('Ctrl Pts',(-35.6854761478361,-29.0605241301525,
7.52391304034139));
#24022=CARTESIAN_POINT('Ctrl Pts',(-36.8429855400596,-30.3470523630749,
8.89340137402966));
#24023=CARTESIAN_POINT('Ctrl Pts',(-38.321034124251,-31.9113293869106,9.3821661014496));
#24024=CARTESIAN_POINT('Ctrl Pts',(-39.7990827084423,-33.4756064107464,
9.87093082886952));
#24025=CARTESIAN_POINT('Ctrl Pts',(-41.2771312926336,-35.0398834345822,
9.3821661014496));
#24026=CARTESIAN_POINT('Ctrl Pts',(-35.837223120671,-26.4881263776668,1.04083408558608E-14));
#24027=CARTESIAN_POINT('Ctrl Pts',(-35.6968958205399,-26.6500727150284,
1.72780310113343));
#24028=CARTESIAN_POINT('Ctrl Pts',(-36.1231280314032,-27.3029456632459,
3.28449990511991));
#24029=CARTESIAN_POINT('Ctrl Pts',(-36.5493602422664,-27.9558186114633,
4.84119670910638));
#24030=CARTESIAN_POINT('Ctrl Pts',(-37.4299379045752,-29.0023841344369,
5.91846432228297));
#24031=CARTESIAN_POINT('Ctrl Pts',(-38.310515566884,-30.0489496574104,6.99573193545955));
#24032=CARTESIAN_POINT('Ctrl Pts',(-39.4432359322495,-31.3139980762872,
7.38020429521638));
#24033=CARTESIAN_POINT('Ctrl Pts',(-40.5759562976149,-32.579046495164,7.76467665497321));
#24034=CARTESIAN_POINT('Ctrl Pts',(-41.7086766629803,-33.8440949140408,
7.38020429521638));
#24035=CARTESIAN_POINT('',(-29.3318883095546,-23.8408520862337,1.57949999773541E-9));
#24036=CARTESIAN_POINT('Origin',(-39.2388322978495,-8.8124635893656,0.));
#24037=CARTESIAN_POINT('Ctrl Pts',(-29.3318883094702,-23.8408520864232,
3.13107478882928E-9));
#24038=CARTESIAN_POINT('Ctrl Pts',(-29.3212938718736,-23.8530787192648,
0.24503815333568));
#24039=CARTESIAN_POINT('Ctrl Pts',(-29.315395835283,-23.8695636319736,0.490791160522109));
#24040=CARTESIAN_POINT('Ctrl Pts',(-29.3142795252164,-23.8903394438999,
0.736766500725953));
#24041=CARTESIAN_POINT('Ctrl Pts',(-29.313166879933,-23.9110470500025,0.981934317701616));
#24042=CARTESIAN_POINT('Ctrl Pts',(-29.3168047115562,-23.9360174743379,
1.22732257376628));
#24043=CARTESIAN_POINT('Ctrl Pts',(-29.3252401898304,-23.9652487409632,
1.47243294816406));
#24044=CARTESIAN_POINT('Ctrl Pts',(-29.3336629639885,-23.9944359843103,
1.71717417803081));
#24045=CARTESIAN_POINT('Ctrl Pts',(-29.3468690005323,-24.0278712558267,
1.96163791541648));
#24046=CARTESIAN_POINT('Ctrl Pts',(-29.3648668425815,-24.0655179217454,
2.20532408778585));
#24047=CARTESIAN_POINT('Ctrl Pts',(-29.3828492487602,-24.1031322999564,
2.44880126242126));
#24048=CARTESIAN_POINT('Ctrl Pts',(-29.4056152523348,-24.1449508188715,
2.69150175431109));
#24049=CARTESIAN_POINT('Ctrl Pts',(-29.4331345151069,-24.1909024709824,
2.93292951866866));
#24050=CARTESIAN_POINT('Ctrl Pts',(-29.4606480207944,-24.236844509916,3.17430677585639));
#24051=CARTESIAN_POINT('Ctrl Pts',(-29.4929127564909,-24.2869178772581,
3.41441139318384));
#24052=CARTESIAN_POINT('Ctrl Pts',(-29.5298597835412,-24.3410179518311,
3.65275710614668));
#24053=CARTESIAN_POINT('Ctrl Pts',(-29.5668537253363,-24.3951867218146,
3.89140546668824));
#24054=CARTESIAN_POINT('Ctrl Pts',(-29.6085417737704,-24.453392318975,4.12829002081204));
#24055=CARTESIAN_POINT('Ctrl Pts',(-29.6548169223662,-24.5154973789739,
4.36293874377852));
#24056=CARTESIAN_POINT('Ctrl Pts',(-29.7011392900671,-24.5776658109002,
4.59782690201493));
#24057=CARTESIAN_POINT('Ctrl Pts',(-29.7520579892327,-24.643741511473,4.83047425895005));
#24058=CARTESIAN_POINT('Ctrl Pts',(-29.8074294704422,-24.7135563309895,
5.06042975959478));
#24059=CARTESIAN_POINT('Ctrl Pts',(-29.8629628361578,-24.7835752616715,
5.29105755998348));
#24060=CARTESIAN_POINT('Ctrl Pts',(-29.9229748872203,-24.8573550203559,
5.51897736305728));
#24061=CARTESIAN_POINT('Ctrl Pts',(-29.9872866904181,-24.9346980180644,
5.74376259354367));
#24062=CARTESIAN_POINT('Ctrl Pts',(-30.028293808516,-24.9840142132785,5.88709234072643));
#24063=CARTESIAN_POINT('Ctrl Pts',(-30.0710484023924,-25.0347785642252,
6.02914825314204));
#24064=CARTESIAN_POINT('Ctrl Pts',(-30.1154974142344,-25.0869345108129,
6.16982677023484));
#24065=CARTESIAN_POINT('Ctrl Pts',(-30.1851947723638,-25.1687165693394,
6.39041482339092));
#24066=CARTESIAN_POINT('Ctrl Pts',(-30.259341175839,-25.2545422584422,6.60890054011809));
#24067=CARTESIAN_POINT('Ctrl Pts',(-30.3378542445905,-25.3442989836977,
6.82480412008047));
#24068=CARTESIAN_POINT('Ctrl Pts',(-30.4161900656827,-25.4338530781082,
7.04022028559297));
#24069=CARTESIAN_POINT('Ctrl Pts',(-30.4988728090634,-25.5273204012125,
7.25306552029641));
#24070=CARTESIAN_POINT('Ctrl Pts',(-30.5857836273892,-25.6245550984955,
7.4628756626942));
#24071=CARTESIAN_POINT('Ctrl Pts',(-30.6725546575098,-25.7216334025459,
7.67234834441867));
#24072=CARTESIAN_POINT('Ctrl Pts',(-30.7635400773297,-25.8224668509014,
7.87879526532997));
#24073=CARTESIAN_POINT('Ctrl Pts',(-30.8585857424178,-25.9268778285524,
8.08177334612148));
#24074=CARTESIAN_POINT('Ctrl Pts',(-30.95354020777,-26.0311886201131,8.28455666214051));
#24075=CARTESIAN_POINT('Ctrl Pts',(-31.0525469907384,-26.1390699181374,
8.48387739272782));
#24076=CARTESIAN_POINT('Ctrl Pts',(-31.1554183156063,-26.2503142961674,
8.67931873611011));
#24077=CARTESIAN_POINT('Ctrl Pts',(-31.2582945883127,-26.3615640247576,
8.87476947970392));
#24078=CARTESIAN_POINT('Ctrl Pts',(-31.3650355954438,-26.4761769610834,
9.06634009532712));
#24079=CARTESIAN_POINT('Ctrl Pts',(-31.4754218249876,-26.5939179778759,
9.25364450340851));
#24080=CARTESIAN_POINT('Ctrl Pts',(-31.5858485486304,-26.7117021867986,
9.44101762226367));
#24081=CARTESIAN_POINT('Ctrl Pts',(-31.6999229509126,-26.8326165417648,
9.62412107874909));
#24082=CARTESIAN_POINT('Ctrl Pts',(-31.8173965346642,-26.956401163024,9.80260437466004));
#24083=CARTESIAN_POINT('Ctrl Pts',(-31.935061742163,-27.0803877026398,9.98137881379573));
#24084=CARTESIAN_POINT('Ctrl Pts',(-32.0561369802829,-27.2072536245426,
10.1555177270915));
#24085=CARTESIAN_POINT('Ctrl Pts',(-32.1803472149474,-27.3367168513597,
10.32470957477));
#24086=CARTESIAN_POINT('Ctrl Pts',(-32.216248177194,-27.3741361061484,10.3736117457733));
#24087=CARTESIAN_POINT('Ctrl Pts',(-32.2524108910189,-27.4117722217276,
10.4221009095721));
#24088=CARTESIAN_POINT('Ctrl Pts',(-32.2888283700867,-27.4496181106866,
10.4701702229062));
#24089=CARTESIAN_POINT('Ctrl Pts',(-31.3186840564486,-31.7027984407112,
0.));
#24090=CARTESIAN_POINT('Ctrl Pts',(-31.1783567563174,-31.8647447780728,
1.72780310113343));
#24091=CARTESIAN_POINT('Ctrl Pts',(-31.6045889671807,-32.5176177262903,
3.28449990511991));
#24092=CARTESIAN_POINT('Ctrl Pts',(-32.030821178044,-33.1704906745077,4.84119670910639));
#24093=CARTESIAN_POINT('Ctrl Pts',(-32.9113988403528,-34.2170561974812,
5.91846432228298));
#24094=CARTESIAN_POINT('Ctrl Pts',(-33.7919765026616,-35.2636217204548,
6.99573193545956));
#24095=CARTESIAN_POINT('Ctrl Pts',(-34.924696868027,-36.5286701393316,7.38020429521639));
#24096=CARTESIAN_POINT('Ctrl Pts',(-36.0574172333924,-37.7937185582084,
7.76467665497322));
#24097=CARTESIAN_POINT('Ctrl Pts',(-37.1901375987578,-39.0587669770852,
7.38020429521639));
#24098=CARTESIAN_POINT('Ctrl Pts',(-30.5436667170413,-29.4615173807455,
0.));
#24099=CARTESIAN_POINT('Ctrl Pts',(-30.4033394169102,-29.6234637181072,
2.19648874705823));
#24100=CARTESIAN_POINT('Ctrl Pts',(-30.9832571433227,-30.4095059236084,
4.17545672685568));
#24101=CARTESIAN_POINT('Ctrl Pts',(-31.5631748697351,-31.1955481291097,
6.15442470665314));
#24102=CARTESIAN_POINT('Ctrl Pts',(-32.7206842619587,-32.4820763620321,
7.5239130403414));
#24103=CARTESIAN_POINT('Ctrl Pts',(-33.8781936541823,-33.7686045949544,
8.89340137402969));
#24104=CARTESIAN_POINT('Ctrl Pts',(-35.3562422383736,-35.3328816187902,
9.38216610144961));
#24105=CARTESIAN_POINT('Ctrl Pts',(-36.834290822565,-36.897158642626,9.87093082886954));
#24106=CARTESIAN_POINT('Ctrl Pts',(-38.3123394067563,-38.4614356664617,
9.38216610144961));
#24107=CARTESIAN_POINT('Ctrl Pts',(-29.3462831821138,-27.4145036200621,
0.));
#24108=CARTESIAN_POINT('Ctrl Pts',(-29.2059558819827,-27.5764499574237,
2.70899372698069));
#24109=CARTESIAN_POINT('Ctrl Pts',(-29.953927810067,-28.5081119576082,5.14971273833323));
#24110=CARTESIAN_POINT('Ctrl Pts',(-30.7018997381513,-29.4397739577927,
7.59043174968578));
#24111=CARTESIAN_POINT('Ctrl Pts',(-32.1622323380279,-30.9886999938349,
9.27946171175751));
#24112=CARTESIAN_POINT('Ctrl Pts',(-33.6225649379044,-32.5376260298771,
10.9684916738292));
#24113=CARTESIAN_POINT('Ctrl Pts',(-35.4782278855713,-34.4291077622636,
11.5712994880388));
#24114=CARTESIAN_POINT('Ctrl Pts',(-37.3338908332383,-36.3205894946501,
12.1741073022483));
#24115=CARTESIAN_POINT('Ctrl Pts',(-39.1895537809052,-38.2120712270365,
11.5712994880388));
#24116=CARTESIAN_POINT('Ctrl Pts',(-27.7725495286738,-25.6404249706858,
0.));
#24117=CARTESIAN_POINT('Ctrl Pts',(-27.6322222285426,-25.8023713080474,
3.24562220582793));
#24118=CARTESIAN_POINT('Ctrl Pts',(-28.5561586333442,-26.8865073952597,
6.16982677025167));
#24119=CARTESIAN_POINT('Ctrl Pts',(-29.4800950381457,-27.9706434824721,
9.09403133467541));
#24120=CARTESIAN_POINT('Ctrl Pts',(-31.2575046687802,-29.7943183296621,
11.1176436806954));
#24121=CARTESIAN_POINT('Ctrl Pts',(-33.0349142994147,-31.6179931768522,
13.1412560267153));
#24122=CARTESIAN_POINT('Ctrl Pts',(-35.2859658372441,-33.8520810728856,
13.8634749112255));
#24123=CARTESIAN_POINT('Ctrl Pts',(-37.5370173750734,-36.0861689689191,
14.5856937957357));
#24124=CARTESIAN_POINT('Ctrl Pts',(-39.7880689129028,-38.3202568649526,
13.8634749112255));
#24125=CARTESIAN_POINT('',(-27.7725495286738,-25.6404249706858,0.));
#24126=CARTESIAN_POINT('Ctrl Pts',(-27.7725495286738,-25.6404249706858,
0.));
#24127=CARTESIAN_POINT('Ctrl Pts',(-27.6322222285426,-25.8023713080474,
3.24562220582793));
#24128=CARTESIAN_POINT('Ctrl Pts',(-28.5561586333442,-26.8865073952597,
6.16982677025167));
#24129=CARTESIAN_POINT('Ctrl Pts',(-29.3274958817334,-27.7915854309818,
8.61106394926976));
#24130=CARTESIAN_POINT('Ctrl Pts',(-30.7134197505151,-29.2324872694338,
10.4489096280657));
#24131=CARTESIAN_POINT('Origin',(-14.3070334890502,-37.5852932322717,1.04083408558608E-14));
#24132=CARTESIAN_POINT('Ctrl Pts',(-27.7725495286738,-25.6404249706858,
0.));
#24133=CARTESIAN_POINT('Ctrl Pts',(-27.6322222285426,-25.8023713080474,
3.24562220582793));
#24134=CARTESIAN_POINT('Ctrl Pts',(-28.5561586333442,-26.8865073952597,
6.16982677025167));
#24135=CARTESIAN_POINT('Ctrl Pts',(-29.4800950381457,-27.9706434824721,
9.09403133467541));
#24136=CARTESIAN_POINT('Ctrl Pts',(-31.2575046687802,-29.7943183296621,
11.1176436806954));
#24137=CARTESIAN_POINT('Ctrl Pts',(-33.0349142994147,-31.6179931768522,
13.1412560267153));
#24138=CARTESIAN_POINT('Ctrl Pts',(-35.2859658372441,-33.8520810728856,
13.8634749112255));
#24139=CARTESIAN_POINT('Ctrl Pts',(-37.5370173750734,-36.0861689689191,
14.5856937957357));
#24140=CARTESIAN_POINT('Ctrl Pts',(-39.7880689129028,-38.3202568649526,
13.8634749112255));
#24141=CARTESIAN_POINT('Ctrl Pts',(-27.7642289310887,-24.6879908429605,
0.));
#24142=CARTESIAN_POINT('Ctrl Pts',(-27.6239016309576,-24.8499371803221,
3.38941559469372));
#24143=CARTESIAN_POINT('Ctrl Pts',(-28.5949889593954,-25.9749297754392,
6.44317352589573));
#24144=CARTESIAN_POINT('Ctrl Pts',(-29.5660762878332,-27.0999223705563,
9.49693145709774));
#24145=CARTESIAN_POINT('Ctrl Pts',(-31.4284489470459,-28.9972181010932,
11.6101975146502));
#24146=CARTESIAN_POINT('Ctrl Pts',(-33.2908216062586,-30.8945138316301,
13.7234635722027));
#24147=CARTESIAN_POINT('Ctrl Pts',(-35.6478203077951,-33.2204054676047,
14.4776794959001));
#24148=CARTESIAN_POINT('Ctrl Pts',(-38.0048190093316,-35.5462971035794,
15.2318954195974));
#24149=CARTESIAN_POINT('Ctrl Pts',(-40.361817710868,-37.872188739554,14.4776794959001));
#24150=CARTESIAN_POINT('Ctrl Pts',(-28.3879644434329,-23.9681616891741,
0.));
#24151=CARTESIAN_POINT('Ctrl Pts',(-28.2476371433017,-24.1301080265358,
3.38941559469373));
#24152=CARTESIAN_POINT('Ctrl Pts',(-29.2187244717395,-25.2551006216529,
6.44317352589574));
#24153=CARTESIAN_POINT('Ctrl Pts',(-30.1898118001773,-26.38009321677,9.49693145709774));
#24154=CARTESIAN_POINT('Ctrl Pts',(-32.05218445939,-28.2773889473069,11.6101975146502));
#24155=CARTESIAN_POINT('Ctrl Pts',(-33.9145571186028,-30.1746846778437,
13.7234635722027));
#24156=CARTESIAN_POINT('Ctrl Pts',(-36.2715558201393,-32.5005763138184,
14.4776794959001));
#24157=CARTESIAN_POINT('Ctrl Pts',(-38.6285545216757,-34.826467949793,15.2318954195974));
#24158=CARTESIAN_POINT('Ctrl Pts',(-40.9855532232122,-37.1523595857677,
14.4776794959001));
#24159=CARTESIAN_POINT('Ctrl Pts',(-29.3318883095342,-23.8408520862199,
0.));
#24160=CARTESIAN_POINT('Ctrl Pts',(-29.191561009403,-24.0027984235816,3.24562220582793));
#24161=CARTESIAN_POINT('Ctrl Pts',(-30.1154974142046,-25.0869345107939,
6.16982677025167));
#24162=CARTESIAN_POINT('Ctrl Pts',(-31.0394338190061,-26.1710705980062,
9.09403133467541));
#24163=CARTESIAN_POINT('Ctrl Pts',(-32.8168434496406,-27.9947454451963,
11.1176436806954));
#24164=CARTESIAN_POINT('Ctrl Pts',(-34.5942530802751,-29.8184202923863,
13.1412560267153));
#24165=CARTESIAN_POINT('Ctrl Pts',(-36.8453046181045,-32.0525081884198,
13.8634749112255));
#24166=CARTESIAN_POINT('Ctrl Pts',(-39.0963561559338,-34.2865960844532,
14.5856937957357));
#24167=CARTESIAN_POINT('Ctrl Pts',(-41.3474076937632,-36.5206839804867,
13.8634749112255));
#24168=CARTESIAN_POINT('',(-28.2121348679537,-24.4459474390529,-3.59391607130504E-31));
#24169=CARTESIAN_POINT('Origin',(-29.5724808444822,-25.624700519279,0.));
#24170=CARTESIAN_POINT('Origin',(-29.5724808444822,-25.624700519279,0.));
#24171=CARTESIAN_POINT('Ctrl Pts',(-32.4262389885813,-19.4238236466308,
0.));
#24172=CARTESIAN_POINT('Ctrl Pts',(-32.3103873848408,-19.6040922608089,
3.24562220582792));
#24173=CARTESIAN_POINT('Ctrl Pts',(-33.3792081011656,-20.5457035458245,
6.16982677025168));
#24174=CARTESIAN_POINT('Ctrl Pts',(-34.4480288174904,-21.48731483084,9.09403133467541));
#24175=CARTESIAN_POINT('Ctrl Pts',(-36.466882971839,-23.0394755334785,11.1176436806954));
#24176=CARTESIAN_POINT('Ctrl Pts',(-38.4857371261876,-24.591636236117,13.1412560267153));
#24177=CARTESIAN_POINT('Ctrl Pts',(-41.0318200627225,-26.4826263031066,
13.8634749112255));
#24178=CARTESIAN_POINT('Ctrl Pts',(-43.5779029992573,-28.3736163700961,
14.5856937957357));
#24179=CARTESIAN_POINT('Ctrl Pts',(-46.1239859357922,-30.2646064370857,
13.8634749112255));
#24180=CARTESIAN_POINT('Ctrl Pts',(-34.5718269932685,-20.4339943155206,
0.));
#24181=CARTESIAN_POINT('Ctrl Pts',(-34.455975389528,-20.6142629296987,2.7089937269807));
#24182=CARTESIAN_POINT('Ctrl Pts',(-35.3289233687525,-21.4299944500888,
5.14971273833323));
#24183=CARTESIAN_POINT('Ctrl Pts',(-36.2018713479769,-22.2457259704788,
7.59043174968578));
#24184=CARTESIAN_POINT('Ctrl Pts',(-37.8677750259291,-23.5710591750643,
9.27946171175751));
#24185=CARTESIAN_POINT('Ctrl Pts',(-39.5336787038813,-24.8963923796499,
10.9684916738293));
#24186=CARTESIAN_POINT('Ctrl Pts',(-41.6396395952274,-26.5045331830051,
11.5712994880388));
#24187=CARTESIAN_POINT('Ctrl Pts',(-43.7456004865736,-28.1126739863604,
12.1741073022483));
#24188=CARTESIAN_POINT('Ctrl Pts',(-45.8515613779198,-29.7208147897157,
11.5712994880388));
#24189=CARTESIAN_POINT('Ctrl Pts',(-36.8732642383513,-21.0061649833183,
0.));
#24190=CARTESIAN_POINT('Ctrl Pts',(-36.7574126346109,-21.1864335974964,
2.19648874705824));
#24191=CARTESIAN_POINT('Ctrl Pts',(-37.4432931040927,-21.8819441292788,
4.17545672685568));
#24192=CARTESIAN_POINT('Ctrl Pts',(-38.1291735735745,-22.5774546610611,
6.15442470665314));
#24193=CARTESIAN_POINT('Ctrl Pts',(-39.4579932465783,-23.6861571296387,
7.5239130403414));
#24194=CARTESIAN_POINT('Ctrl Pts',(-40.7868129195821,-24.7948595982163,
8.89340137402967));
#24195=CARTESIAN_POINT('Ctrl Pts',(-42.4724369320183,-26.1328662922314,
9.38216610144961));
#24196=CARTESIAN_POINT('Ctrl Pts',(-44.1580609444544,-27.4708729862465,
9.87093082886954));
#24197=CARTESIAN_POINT('Ctrl Pts',(-45.8436849568905,-28.8088796802616,
9.38216610144961));
#24198=CARTESIAN_POINT('Ctrl Pts',(-39.2421052839113,-21.1183468312846,
0.));
#24199=CARTESIAN_POINT('Ctrl Pts',(-39.1262536801708,-21.2986154454627,
1.72780310113343));
#24200=CARTESIAN_POINT('Ctrl Pts',(-39.6410609697422,-21.8841839202765,
3.28449990511991));
#24201=CARTESIAN_POINT('Ctrl Pts',(-40.1558682593135,-22.4697523950902,
4.84119670910639));
#24202=CARTESIAN_POINT('Ctrl Pts',(-41.1764247138525,-23.3803461224642,
5.91846432228297));
#24203=CARTESIAN_POINT('Ctrl Pts',(-42.1969811683915,-24.2909398498382,
6.99573193545956));
#24204=CARTESIAN_POINT('Ctrl Pts',(-43.4982072348258,-25.3819089842542,
7.38020429521639));
#24205=CARTESIAN_POINT('Ctrl Pts',(-44.7994333012599,-26.4728781186702,
7.76467665497321));
#24206=CARTESIAN_POINT('Ctrl Pts',(-46.1006593676942,-27.5638472530862,
7.38020429521639));
#24207=CARTESIAN_POINT('',(-32.4262389886035,-19.4238236466415,1.57949966272277E-9));
#24208=CARTESIAN_POINT('Origin',(-40.0935818932913,-3.13849734404805,0.));
#24209=CARTESIAN_POINT('Ctrl Pts',(-32.4262389885469,-19.4238236468412,
3.13107437314513E-9));
#24210=CARTESIAN_POINT('Ctrl Pts',(-32.4174924183246,-19.4374335758629,
0.245038153335358));
#24211=CARTESIAN_POINT('Ctrl Pts',(-32.4140004629283,-19.454590074053,0.490791160521465));
#24212=CARTESIAN_POINT('Ctrl Pts',(-32.4158522216029,-19.4753132856568,
0.736766500724985));
#24213=CARTESIAN_POINT('Ctrl Pts',(-32.4176979010577,-19.4959684641207,
0.981934317700663));
#24214=CARTESIAN_POINT('Ctrl Pts',(-32.4248523667011,-19.5201670081216,
1.22732257376534));
#24215=CARTESIAN_POINT('Ctrl Pts',(-32.4373620269518,-19.5479002488743,
1.47243294816314));
#24216=CARTESIAN_POINT('Ctrl Pts',(-32.4498528472302,-19.5755917224265,
1.7171741780299));
#24217=CARTESIAN_POINT('Ctrl Pts',(-32.4676828006219,-19.6068072561337,
1.96163791541559));
#24218=CARTESIAN_POINT('Ctrl Pts',(-32.4908551297615,-19.6415093732947,
2.20532408778497));
#24219=CARTESIAN_POINT('Ctrl Pts',(-32.5140075851257,-19.676181728144,2.44880126242033));
#24220=CARTESIAN_POINT('Ctrl Pts',(-32.542493259366,-19.7143346547169,2.69150175431012));
#24221=CARTESIAN_POINT('Ctrl Pts',(-32.5762720176611,-19.7559021858353,
2.93292951866765));
#24222=CARTESIAN_POINT('Ctrl Pts',(-32.6100437093726,-19.7974610209433,
3.17430677585542));
#24223=CARTESIAN_POINT('Ctrl Pts',(-32.6491062197567,-19.8424329629631,
3.41441139318292));
#24224=CARTESIAN_POINT('Ctrl Pts',(-32.6933764227083,-19.8907242666035,
3.6527571061458));
#24225=CARTESIAN_POINT('Ctrl Pts',(-32.7377028392565,-19.9390768897698,
3.89140546668732));
#24226=CARTESIAN_POINT('Ctrl Pts',(-32.7872500836132,-19.9907572100057,
4.12829002081109));
#24227=CARTESIAN_POINT('Ctrl Pts',(-32.8418926894892,-20.0456444897535,
4.36293874377754));
#24228=CARTESIAN_POINT('Ctrl Pts',(-32.8965910526135,-20.1005877764144,
4.5978269020138));
#24229=CARTESIAN_POINT('Ctrl Pts',(-32.956395025481,-20.1587444351918,4.83047425894876));
#24230=CARTESIAN_POINT('Ctrl Pts',(-33.0211385895994,-20.2199684571169,
5.06042975959334));
#24231=CARTESIAN_POINT('Ctrl Pts',(-33.0860714385206,-20.281371474083,5.2910575599822));
#24232=CARTESIAN_POINT('Ctrl Pts',(-33.1559726078586,-20.3458596558642,
5.51897736305615));
#24233=CARTESIAN_POINT('Ctrl Pts',(-33.2306368658403,-20.4132628895043,
5.74376259354269));
#24234=CARTESIAN_POINT('Ctrl Pts',(-33.2782450169495,-20.4562411955792,
5.88709234072579));
#24235=CARTESIAN_POINT('Ctrl Pts',(-33.3277889511024,-20.5004042255165,
6.02914825314172));
#24236=CARTESIAN_POINT('Ctrl Pts',(-33.3792081011978,-20.545703545839,6.16982677023484));
#24237=CARTESIAN_POINT('Ctrl Pts',(-33.4598348411496,-20.6167342126795,
6.3904148233909));
#24238=CARTESIAN_POINT('Ctrl Pts',(-33.545440810212,-20.6911341865985,6.60890054011805));
#24239=CARTESIAN_POINT('Ctrl Pts',(-33.6359284429689,-20.7688037431277,
6.82480412008041));
#24240=CARTESIAN_POINT('Ctrl Pts',(-33.726211794816,-20.8462979562737,7.04022028559295));
#24241=CARTESIAN_POINT('Ctrl Pts',(-33.8213547340592,-20.9270469355454,
7.25306552029643));
#24242=CARTESIAN_POINT('Ctrl Pts',(-33.921218865788,-21.0109232247567,7.46287566269427));
#24243=CARTESIAN_POINT('Ctrl Pts',(-34.0209223750762,-21.0946646065288,
7.67234834441895));
#24244=CARTESIAN_POINT('Ctrl Pts',(-34.1253317904079,-21.1815231404631,
7.87879526533046));
#24245=CARTESIAN_POINT('Ctrl Pts',(-34.2342692590684,-21.2713449564543,
8.08177334612217));
#24246=CARTESIAN_POINT('Ctrl Pts',(-34.3431021983076,-21.3610805851809,
8.28455666214149));
#24247=CARTESIAN_POINT('Ctrl Pts',(-34.4564543444627,-21.4537736728373,
8.48387739272907));
#24248=CARTESIAN_POINT('Ctrl Pts',(-34.5741103132399,-21.5492456275387,
8.67931873611163));
#24249=CARTESIAN_POINT('Ctrl Pts',(-34.6917719409579,-21.6447221741884,
8.87476947970546));
#24250=CARTESIAN_POINT('Ctrl Pts',(-34.8137376000415,-21.7429776869136,
9.06634009532869));
#24251=CARTESIAN_POINT('Ctrl Pts',(-34.9397565506953,-21.8438106715187,
9.2536445034101));
#24252=CARTESIAN_POINT('Ctrl Pts',(-35.0658217301577,-21.9446806457091,
9.44101762226536));
#24253=CARTESIAN_POINT('Ctrl Pts',(-35.1959429263785,-22.0481297867741,
9.62412107875087));
#24254=CARTESIAN_POINT('Ctrl Pts',(-35.3298371867857,-22.1539362249986,
9.80260437466191));
#24255=CARTESIAN_POINT('Ctrl Pts',(-35.4639498564648,-22.2599152554393,
9.98137881379736));
#24256=CARTESIAN_POINT('Ctrl Pts',(-35.6018476263945,-22.3682590622507,
10.1555177270929));
#24257=CARTESIAN_POINT('Ctrl Pts',(-35.7432181181532,-22.478727580631,10.3247095747712));
#24258=CARTESIAN_POINT('Ctrl Pts',(-35.7840789755622,-22.5106567217238,
10.3736117457741));
#24259=CARTESIAN_POINT('Ctrl Pts',(-35.8252297828043,-22.5427632651434,
10.4221009095725));
#24260=CARTESIAN_POINT('Ctrl Pts',(-35.866662616011,-22.575041189878,10.4701702229062));
#24261=CARTESIAN_POINT('Ctrl Pts',(-35.5116836434677,-26.9229962078197,
0.));
#24262=CARTESIAN_POINT('Ctrl Pts',(-35.3958320397272,-27.1032648219978,
1.72780310113342));
#24263=CARTESIAN_POINT('Ctrl Pts',(-35.9106393292985,-27.6888332968116,
3.28449990511992));
#24264=CARTESIAN_POINT('Ctrl Pts',(-36.4254466188699,-28.2744017716254,
4.84119670910638));
#24265=CARTESIAN_POINT('Ctrl Pts',(-37.4460030734089,-29.1849954989994,
5.91846432228298));
#24266=CARTESIAN_POINT('Ctrl Pts',(-38.4665595279479,-30.0955892263734,
6.99573193545956));
#24267=CARTESIAN_POINT('Ctrl Pts',(-39.7677855943821,-31.1865583607894,
7.38020429521639));
#24268=CARTESIAN_POINT('Ctrl Pts',(-41.0690116608163,-32.2775274952054,
7.76467665497322));
#24269=CARTESIAN_POINT('Ctrl Pts',(-42.3702377272506,-33.3684966296214,
7.38020429521639));
#24270=CARTESIAN_POINT('Ctrl Pts',(-34.4255873115189,-24.8148246247008,
0.));
#24271=CARTESIAN_POINT('Ctrl Pts',(-34.3097357077784,-24.995093238879,2.19648874705823));
#24272=CARTESIAN_POINT('Ctrl Pts',(-34.9956161772602,-25.6906037706613,
4.17545672685568));
#24273=CARTESIAN_POINT('Ctrl Pts',(-35.681496646742,-26.3861143024436,6.15442470665313));
#24274=CARTESIAN_POINT('Ctrl Pts',(-37.0103163197458,-27.4948167710213,
7.5239130403414));
#24275=CARTESIAN_POINT('Ctrl Pts',(-38.3391359927496,-28.6035192395989,
8.89340137402967));
#24276=CARTESIAN_POINT('Ctrl Pts',(-40.0247600051858,-29.941525933614,9.3821661014496));
#24277=CARTESIAN_POINT('Ctrl Pts',(-41.7103840176219,-31.2795326276291,
9.87093082886954));
#24278=CARTESIAN_POINT('Ctrl Pts',(-43.3960080300581,-32.6175393216441,
9.3821661014496));
#24279=CARTESIAN_POINT('Ctrl Pts',(-32.9490709821976,-22.9590519566754,
-1.05434036998093E-14));
#24280=CARTESIAN_POINT('Ctrl Pts',(-32.8332193784571,-23.1393205708535,
2.70899372698069));
#24281=CARTESIAN_POINT('Ctrl Pts',(-33.7061673576816,-23.9550520912435,
5.14971273833323));
#24282=CARTESIAN_POINT('Ctrl Pts',(-34.5791153369061,-24.7707836116335,
7.59043174968578));
#24283=CARTESIAN_POINT('Ctrl Pts',(-36.2450190148583,-26.096116816219,9.27946171175751));
#24284=CARTESIAN_POINT('Ctrl Pts',(-37.9109226928105,-27.4214500208046,
10.9684916738293));
#24285=CARTESIAN_POINT('Ctrl Pts',(-40.0168835841566,-29.0295908241599,
11.5712994880388));
#24286=CARTESIAN_POINT('Ctrl Pts',(-42.1228444755027,-30.6377316275152,
12.1741073022483));
#24287=CARTESIAN_POINT('Ctrl Pts',(-44.2288053668489,-32.2458724308704,
11.5712994880388));
#24288=CARTESIAN_POINT('Ctrl Pts',(-31.1388779521429,-21.4269965203141,
0.));
#24289=CARTESIAN_POINT('Ctrl Pts',(-31.0230263484024,-21.6072651344922,
3.24562220582793));
#24290=CARTESIAN_POINT('Ctrl Pts',(-32.0918470647272,-22.5488764195077,
6.16982677025168));
#24291=CARTESIAN_POINT('Ctrl Pts',(-33.160667781052,-23.4904877045232,9.09403133467541));
#24292=CARTESIAN_POINT('Ctrl Pts',(-35.1795219354007,-25.0426484071617,
11.1176436806954));
#24293=CARTESIAN_POINT('Ctrl Pts',(-37.1983760897493,-26.5948091098002,
13.1412560267153));
#24294=CARTESIAN_POINT('Ctrl Pts',(-39.7444590262841,-28.4857991767898,
13.8634749112255));
#24295=CARTESIAN_POINT('Ctrl Pts',(-42.2905419628189,-30.3767892437794,
14.5856937957357));
#24296=CARTESIAN_POINT('Ctrl Pts',(-44.8366248993538,-32.267779310769,13.8634749112255));
#24297=CARTESIAN_POINT('',(-31.1388779521429,-21.4269965203141,0.));
#24298=CARTESIAN_POINT('Ctrl Pts',(-31.1388779521429,-21.4269965203141,
0.));
#24299=CARTESIAN_POINT('Ctrl Pts',(-31.0230263484024,-21.6072651344922,
3.24562220582793));
#24300=CARTESIAN_POINT('Ctrl Pts',(-32.0918470647272,-22.5488764195077,
6.16982677025168));
#24301=CARTESIAN_POINT('Ctrl Pts',(-32.9841392463828,-23.3349693300821,
8.61106394926976));
#24302=CARTESIAN_POINT('Ctrl Pts',(-34.5610181206245,-24.5639673341829,
10.4489096280657));
#24303=CARTESIAN_POINT('Origin',(-19.5103534449752,-35.1666259835201,0.));
#24304=CARTESIAN_POINT('Ctrl Pts',(-31.1388779521429,-21.4269965203141,
0.));
#24305=CARTESIAN_POINT('Ctrl Pts',(-31.0230263484024,-21.6072651344922,
3.24562220582793));
#24306=CARTESIAN_POINT('Ctrl Pts',(-32.0918470647273,-22.5488764195077,
6.16982677025168));
#24307=CARTESIAN_POINT('Ctrl Pts',(-33.160667781052,-23.4904877045232,9.09403133467541));
#24308=CARTESIAN_POINT('Ctrl Pts',(-35.1795219354007,-25.0426484071617,
11.1176436806954));
#24309=CARTESIAN_POINT('Ctrl Pts',(-37.1983760897493,-26.5948091098002,
13.1412560267153));
#24310=CARTESIAN_POINT('Ctrl Pts',(-39.7444590262841,-28.4857991767898,
13.8634749112255));
#24311=CARTESIAN_POINT('Ctrl Pts',(-42.2905419628189,-30.3767892437794,
14.5856937957357));
#24312=CARTESIAN_POINT('Ctrl Pts',(-44.8366248993538,-32.267779310769,13.8634749112255));
#24313=CARTESIAN_POINT('Ctrl Pts',(-30.9950965373908,-20.4854409432121,
0.));
#24314=CARTESIAN_POINT('Ctrl Pts',(-30.8792449336503,-20.6657095573902,
3.38941559469372));
#24315=CARTESIAN_POINT('Ctrl Pts',(-32.0005511325096,-21.6410512138985,
6.44317352589573));
#24316=CARTESIAN_POINT('Ctrl Pts',(-33.121857331369,-22.6163928704068,9.49693145709774));
#24317=CARTESIAN_POINT('Ctrl Pts',(-35.2352870572785,-24.2293336022809,
11.6101975146502));
#24318=CARTESIAN_POINT('Ctrl Pts',(-37.348716783188,-25.842274334155,13.7234635722027));
#24319=CARTESIAN_POINT('Ctrl Pts',(-40.0127335284693,-27.8090558579147,
14.4776794959001));
#24320=CARTESIAN_POINT('Ctrl Pts',(-42.6767502737505,-29.7758373816744,
15.2318954195974));
#24321=CARTESIAN_POINT('Ctrl Pts',(-45.3407670190317,-31.7426189054341,
14.4776794959001));
#24322=CARTESIAN_POINT('Ctrl Pts',(-31.5100409519661,-19.6841717937388,
6.24500451351651E-15));
#24323=CARTESIAN_POINT('Ctrl Pts',(-31.3941893482257,-19.8644404079169,
3.38941559469372));
#24324=CARTESIAN_POINT('Ctrl Pts',(-32.515495547085,-20.8397820644252,6.44317352589573));
#24325=CARTESIAN_POINT('Ctrl Pts',(-33.6368017459443,-21.8151237209335,
9.49693145709774));
#24326=CARTESIAN_POINT('Ctrl Pts',(-35.7502314718538,-23.4280644528076,
11.6101975146502));
#24327=CARTESIAN_POINT('Ctrl Pts',(-37.8636611977633,-25.0410051846817,
13.7234635722027));
#24328=CARTESIAN_POINT('Ctrl Pts',(-40.5276779430446,-27.0077867084414,
14.4776794959001));
#24329=CARTESIAN_POINT('Ctrl Pts',(-43.1916946883258,-28.9745682322011,
15.2318954195974));
#24330=CARTESIAN_POINT('Ctrl Pts',(-45.855711433607,-30.9413497559608,14.4776794959001));
#24331=CARTESIAN_POINT('Ctrl Pts',(-32.4262389885813,-19.4238236466308,
0.));
#24332=CARTESIAN_POINT('Ctrl Pts',(-32.3103873848408,-19.6040922608089,
3.24562220582792));
#24333=CARTESIAN_POINT('Ctrl Pts',(-33.3792081011656,-20.5457035458245,
6.16982677025168));
#24334=CARTESIAN_POINT('Ctrl Pts',(-34.4480288174904,-21.48731483084,9.09403133467541));
#24335=CARTESIAN_POINT('Ctrl Pts',(-36.466882971839,-23.0394755334785,11.1176436806954));
#24336=CARTESIAN_POINT('Ctrl Pts',(-38.4857371261876,-24.591636236117,13.1412560267153));
#24337=CARTESIAN_POINT('Ctrl Pts',(-41.0318200627225,-26.4826263031066,
13.8634749112255));
#24338=CARTESIAN_POINT('Ctrl Pts',(-43.5779029992573,-28.3736163700962,
14.5856937957357));
#24339=CARTESIAN_POINT('Ctrl Pts',(-46.1239859357922,-30.2646064370857,
13.8634749112255));
#24340=CARTESIAN_POINT('',(-31.4039970697396,-20.1821175312286,-3.07395939441906E-30));
#24341=CARTESIAN_POINT('Origin',(-32.9182507396842,-21.1552751870375,0.));
#24342=CARTESIAN_POINT('Origin',(-32.9182507396842,-21.1552751870375,0.));
#24343=CARTESIAN_POINT('Ctrl Pts',(-34.8604849513723,-14.6113821712782,
0.));
#24344=CARTESIAN_POINT('Ctrl Pts',(-34.7714674485862,-14.8063033131399,
3.24562220582793));
#24345=CARTESIAN_POINT('Ctrl Pts',(-35.9634143688743,-15.5862213055784,
6.16982677025167));
#24346=CARTESIAN_POINT('Ctrl Pts',(-37.1553612891624,-16.366139298017,9.09403133467541));
#24347=CARTESIAN_POINT('Ctrl Pts',(-39.3745619185372,-17.6151883402601,
11.1176436806954));
#24348=CARTESIAN_POINT('Ctrl Pts',(-41.593762547912,-18.8642373825032,13.1412560267153));
#24349=CARTESIAN_POINT('Ctrl Pts',(-44.3830459768614,-20.37363451585,13.8634749112255));
#24350=CARTESIAN_POINT('Ctrl Pts',(-47.1723294058108,-21.8830316491968,
14.5856937957357));
#24351=CARTESIAN_POINT('Ctrl Pts',(-49.9616128347602,-23.3924287825436,
13.8634749112255));
#24352=CARTESIAN_POINT('Ctrl Pts',(-37.1279962392257,-15.3059217494164,
0.));
#24353=CARTESIAN_POINT('Ctrl Pts',(-37.0389787364396,-15.5008428912781,
2.70899372698069));
#24354=CARTESIAN_POINT('Ctrl Pts',(-38.0191320633213,-16.1840379904939,
5.14971273833323));
#24355=CARTESIAN_POINT('Ctrl Pts',(-38.9992853902031,-16.8672330897098,
7.59043174968578));
#24356=CARTESIAN_POINT('Ctrl Pts',(-40.8368471514173,-17.9419935007387,
9.2794617117575));
#24357=CARTESIAN_POINT('Ctrl Pts',(-42.6744089126314,-19.0167539117676,
10.9684916738292));
#24358=CARTESIAN_POINT('Ctrl Pts',(-44.9877964569987,-20.3088166768305,
11.5712994880388));
#24359=CARTESIAN_POINT('Ctrl Pts',(-47.301184001366,-21.6008794418934,12.1741073022483));
#24360=CARTESIAN_POINT('Ctrl Pts',(-49.6145715457333,-22.8929422069563,
11.5712994880388));
#24361=CARTESIAN_POINT('Ctrl Pts',(-39.4874365476045,-15.5447398754878,
0.));
#24362=CARTESIAN_POINT('Ctrl Pts',(-39.3984190448183,-15.7396610173495,
2.19648874705824));
#24363=CARTESIAN_POINT('Ctrl Pts',(-40.1762997089267,-16.3304812866725,
4.17545672685568));
#24364=CARTESIAN_POINT('Ctrl Pts',(-40.9541803730352,-16.9213015559956,
6.15442470665314));
#24365=CARTESIAN_POINT('Ctrl Pts',(-42.4272593902764,-17.8296082752022,
7.5239130403414));
#24366=CARTESIAN_POINT('Ctrl Pts',(-43.9003384075176,-18.7379149944087,
8.89340137402967));
#24367=CARTESIAN_POINT('Ctrl Pts',(-45.7592234042436,-19.8224134008056,
9.3821661014496));
#24368=CARTESIAN_POINT('Ctrl Pts',(-47.6181084009696,-20.9069118072026,
9.87093082886953));
#24369=CARTESIAN_POINT('Ctrl Pts',(-49.4769933976956,-21.9914102135995,
9.3821661014496));
#24370=CARTESIAN_POINT('Ctrl Pts',(-41.8481313484579,-15.3186586437006,
0.));
#24371=CARTESIAN_POINT('Ctrl Pts',(-41.7591138456717,-15.5135797855623,
1.72780310113343));
#24372=CARTESIAN_POINT('Ctrl Pts',(-42.3520162221171,-16.0199233014653,
3.28449990511991));
#24373=CARTESIAN_POINT('Ctrl Pts',(-42.9449185985625,-16.5262668173682,
4.84119670910639));
#24374=CARTESIAN_POINT('Ctrl Pts',(-44.0846782589591,-17.2823516867888,
5.91846432228298));
#24375=CARTESIAN_POINT('Ctrl Pts',(-45.2244379193557,-18.0384365562093,
6.99573193545956));
#24376=CARTESIAN_POINT('Ctrl Pts',(-46.6676804765722,-18.933117420683,7.38020429521639));
#24377=CARTESIAN_POINT('Ctrl Pts',(-48.1109230337888,-19.8277982851567,
7.76467665497322));
#24378=CARTESIAN_POINT('Ctrl Pts',(-49.5541655910053,-20.7224791496304,
7.38020429521639));
#24379=CARTESIAN_POINT('',(-34.8604849513958,-14.6113821712857,1.57949297810451E-9));
#24380=CARTESIAN_POINT('Origin',(-40.1321417817282,2.59935965651536,0.));
#24381=CARTESIAN_POINT('Ctrl Pts',(-34.8604849513682,-14.6113821714913,
3.13106096116309E-9));
#24382=CARTESIAN_POINT('Ctrl Pts',(-34.8537643034669,-14.6260983377862,
0.245038153335458));
#24383=CARTESIAN_POINT('Ctrl Pts',(-34.8527495154069,-14.6435771646298,
0.490791160521679));
#24384=CARTESIAN_POINT('Ctrl Pts',(-34.857531646356,-14.6638259110836,0.736766500725313));
#24385=CARTESIAN_POINT('Ctrl Pts',(-34.8622980778378,-14.6840081820399,
0.981934317700944));
#24386=CARTESIAN_POINT('Ctrl Pts',(-34.8728235332128,-14.7069422331334,
1.22732257376558));
#24387=CARTESIAN_POINT('Ctrl Pts',(-34.8891527148321,-14.7326128792078,
1.47243294816333));
#24388=CARTESIAN_POINT('Ctrl Pts',(-34.9054573041505,-14.7582448644192,
1.71717417803007));
#24389=CARTESIAN_POINT('Ctrl Pts',(-34.9275482079565,-14.7866052020689,
1.96163791541575));
#24390=CARTESIAN_POINT('Ctrl Pts',(-34.9554233023887,-14.8176563354397,
2.20532408778512));
#24391=CARTESIAN_POINT('Ctrl Pts',(-34.9832744897133,-14.8486808377692,
2.44880126242062));
#24392=CARTESIAN_POINT('Ctrl Pts',(-35.0168999484377,-14.8823914884391,
2.69150175431054));
#24393=CARTESIAN_POINT('Ctrl Pts',(-35.0562505641469,-14.9187287035023,
2.9329295186682));
#24394=CARTESIAN_POINT('Ctrl Pts',(-35.0955929476288,-14.9550583167477,
3.17430677585629));
#24395=CARTESIAN_POINT('Ctrl Pts',(-35.1406580326361,-14.994013334394,3.41441139318411));
#24396=CARTESIAN_POINT('Ctrl Pts',(-35.1913501978218,-15.0355127954204,
3.65275710614731));
#24397=CARTESIAN_POINT('Ctrl Pts',(-35.2421067311089,-15.0770649517994,
3.89140546668886));
#24398=CARTESIAN_POINT('Ctrl Pts',(-35.2985045323756,-15.1211679328247,
4.12829002081264));
#24399=CARTESIAN_POINT('Ctrl Pts',(-35.3604022296526,-15.1677200855875,
4.36293874377911));
#24400=CARTESIAN_POINT('Ctrl Pts',(-35.4223630872641,-15.21431974011,4.59782690201544));
#24401=CARTESIAN_POINT('Ctrl Pts',(-35.4898348974065,-15.2633734552294,
4.83047425895048));
#24402=CARTESIAN_POINT('Ctrl Pts',(-35.5626325521735,-15.3147603350322,
5.06042975959513));
#24403=CARTESIAN_POINT('Ctrl Pts',(-35.6356430387471,-15.3662974499286,
5.29105755998388));
#24404=CARTESIAN_POINT('Ctrl Pts',(-35.7140103401311,-15.4201812613942,
5.51897736305773));
#24405=CARTESIAN_POINT('Ctrl Pts',(-35.7975071039181,-15.4762725955038,
5.74376259354417));
#24406=CARTESIAN_POINT('Ctrl Pts',(-35.8507471233725,-15.5120380980667,
5.88709234072676));
#24407=CARTESIAN_POINT('Ctrl Pts',(-35.9060718261752,-15.5487007750605,
6.02914825314221));
#24408=CARTESIAN_POINT('Ctrl Pts',(-35.9634143689083,-15.5862213055883,
6.16982677023483));
#24409=CARTESIAN_POINT('Ctrl Pts',(-36.0533291627654,-15.6450546012013,
6.39041482339093));
#24410=CARTESIAN_POINT('Ctrl Pts',(-36.1486520067522,-15.7065142910194,
6.60890054011812));
#24411=CARTESIAN_POINT('Ctrl Pts',(-36.2492721362562,-15.7705155506319,
6.82480412008051));
#24412=CARTESIAN_POINT('Ctrl Pts',(-36.3496651101703,-15.8343723238086,
7.04022028559306));
#24413=CARTESIAN_POINT('Ctrl Pts',(-36.4553314094026,-15.9007591428905,
7.25306552029654));
#24414=CARTESIAN_POINT('Ctrl Pts',(-36.5661159087967,-15.9695695446609,
7.46287566269438));
#24415=CARTESIAN_POINT('Ctrl Pts',(-36.6767222213246,-16.0382692711121,
7.67234834441907));
#24416=CARTESIAN_POINT('Ctrl Pts',(-36.7924301575638,-16.1093847013534,
7.87879526533059));
#24417=CARTESIAN_POINT('Ctrl Pts',(-36.9130417770843,-16.1827888425359,
8.0817733461223));
#24418=CARTESIAN_POINT('Ctrl Pts',(-37.0335376654159,-16.2561225498036,
8.28455666214181));
#24419=CARTESIAN_POINT('Ctrl Pts',(-37.1589276519424,-16.3317404631321,
8.48387739272959));
#24420=CARTESIAN_POINT('Ctrl Pts',(-37.2889731283965,-16.4094964608255,
8.67931873611233));
#24421=CARTESIAN_POINT('Ctrl Pts',(-37.4190248596937,-16.4872561983765,
8.87476947970613));
#24422=CARTESIAN_POINT('Ctrl Pts',(-37.5537323016307,-16.5671540886076,
9.06634009532933));
#24423=CARTESIAN_POINT('Ctrl Pts',(-37.6928185909679,-16.6490263722368,
9.25364450341071));
#24424=CARTESIAN_POINT('Ctrl Pts',(-37.831955902738,-16.7309286899055,9.44101762226605));
#24425=CARTESIAN_POINT('Ctrl Pts',(-37.9754750005807,-16.8148066908797,
9.62412107875164));
#24426=CARTESIAN_POINT('Ctrl Pts',(-38.1230642366208,-16.9004810321079,
9.80260437466275));
#24427=CARTESIAN_POINT('Ctrl Pts',(-38.2708942212748,-16.9862951259321,
9.98137881379835));
#24428=CARTESIAN_POINT('Ctrl Pts',(-38.4228073220832,-17.0739112501833,
10.1555177270941));
#24429=CARTESIAN_POINT('Ctrl Pts',(-38.578460175403,-17.1631362396578,10.3247095747725));
#24430=CARTESIAN_POINT('Ctrl Pts',(-38.6234491187505,-17.1889252818182,
10.373611745775));
#24431=CARTESIAN_POINT('Ctrl Pts',(-38.6687503076433,-17.2148486564419,
10.4221009095729));
#24432=CARTESIAN_POINT('Ctrl Pts',(-38.7143550419872,-17.2409015314864,
10.4701702229062));
#24433=CARTESIAN_POINT('Ctrl Pts',(-38.9817677587449,-21.5951194116468,
0.));
#24434=CARTESIAN_POINT('Ctrl Pts',(-38.8927502559587,-21.7900405535085,
1.72780310113343));
#24435=CARTESIAN_POINT('Ctrl Pts',(-39.4856526324041,-22.2963840694115,
3.28449990511991));
#24436=CARTESIAN_POINT('Ctrl Pts',(-40.0785550088495,-22.8027275853144,
4.84119670910638));
#24437=CARTESIAN_POINT('Ctrl Pts',(-41.2183146692461,-23.558812454735,5.91846432228297));
#24438=CARTESIAN_POINT('Ctrl Pts',(-42.3580743296427,-24.3148973241555,
6.99573193545956));
#24439=CARTESIAN_POINT('Ctrl Pts',(-43.8013168868592,-25.2095781886292,
7.38020429521638));
#24440=CARTESIAN_POINT('Ctrl Pts',(-45.2445594440757,-26.1042590531029,
7.76467665497321));
#24441=CARTESIAN_POINT('Ctrl Pts',(-46.6878020012923,-26.9989399175765,
7.38020429521638));
#24442=CARTESIAN_POINT('Ctrl Pts',(-37.6067022235298,-19.6629735993422,
0.));
#24443=CARTESIAN_POINT('Ctrl Pts',(-37.5176847207437,-19.8578947412039,
2.19648874705822));
#24444=CARTESIAN_POINT('Ctrl Pts',(-38.2955653848521,-20.4487150105269,
4.17545672685568));
#24445=CARTESIAN_POINT('Ctrl Pts',(-39.0734460489605,-21.03953527985,6.15442470665314));
#24446=CARTESIAN_POINT('Ctrl Pts',(-40.5465250662017,-21.9478419990565,
7.5239130403414));
#24447=CARTESIAN_POINT('Ctrl Pts',(-42.0196040834429,-22.8561487182631,
8.89340137402967));
#24448=CARTESIAN_POINT('Ctrl Pts',(-43.8784890801689,-23.94064712466,9.3821661014496));
#24449=CARTESIAN_POINT('Ctrl Pts',(-45.7373740768949,-25.025145531057,9.87093082886954));
#24450=CARTESIAN_POINT('Ctrl Pts',(-47.5962590736209,-26.1096439374539,
9.3821661014496));
#24451=CARTESIAN_POINT('Ctrl Pts',(-35.8811107143583,-18.0362202038892,
0.));
#24452=CARTESIAN_POINT('Ctrl Pts',(-35.7920932115721,-18.2311413457509,
2.70899372698069));
#24453=CARTESIAN_POINT('Ctrl Pts',(-36.7722465384539,-18.9143364449667,
5.14971273833323));
#24454=CARTESIAN_POINT('Ctrl Pts',(-37.7523998653356,-19.5975315441826,
7.59043174968577));
#24455=CARTESIAN_POINT('Ctrl Pts',(-39.5899616265498,-20.6722919552115,
9.27946171175751));
#24456=CARTESIAN_POINT('Ctrl Pts',(-41.427523387764,-21.7470523662404,10.9684916738293));
#24457=CARTESIAN_POINT('Ctrl Pts',(-43.7409109321313,-23.0391151313033,
11.5712994880388));
#24458=CARTESIAN_POINT('Ctrl Pts',(-46.0542984764985,-24.3311778963662,
12.1741073022483));
#24459=CARTESIAN_POINT('Ctrl Pts',(-48.3676860208658,-25.6232406614291,
11.5712994880388));
#24460=CARTESIAN_POINT('Ctrl Pts',(-33.8713086176153,-16.7773762111442,
0.));
#24461=CARTESIAN_POINT('Ctrl Pts',(-33.7822911148291,-16.9722973530059,
3.24562220582793));
#24462=CARTESIAN_POINT('Ctrl Pts',(-34.9742380351172,-17.7522153454444,
6.16982677025168));
#24463=CARTESIAN_POINT('Ctrl Pts',(-36.1661849554053,-18.5321333378829,
9.09403133467541));
#24464=CARTESIAN_POINT('Ctrl Pts',(-38.3853855847801,-19.781182380126,11.1176436806954));
#24465=CARTESIAN_POINT('Ctrl Pts',(-40.604586214155,-21.0302314223691,13.1412560267153));
#24466=CARTESIAN_POINT('Ctrl Pts',(-43.3938696431043,-22.5396285557159,
13.8634749112255));
#24467=CARTESIAN_POINT('Ctrl Pts',(-46.1831530720537,-24.0490256890628,
14.5856937957357));
#24468=CARTESIAN_POINT('Ctrl Pts',(-48.9724365010031,-25.5584228224096,
13.8634749112255));
#24469=CARTESIAN_POINT('',(-33.8713086176152,-16.7773762111442,0.));
#24470=CARTESIAN_POINT('Ctrl Pts',(-33.8713086176152,-16.7773762111442,
0.));
#24471=CARTESIAN_POINT('Ctrl Pts',(-33.7822911148291,-16.9722973530059,
3.24562220582793));
#24472=CARTESIAN_POINT('Ctrl Pts',(-34.9742380351172,-17.7522153454444,
6.16982677025168));
#24473=CARTESIAN_POINT('Ctrl Pts',(-35.9693206543788,-18.4033205461167,
8.61106394926976));
#24474=CARTESIAN_POINT('Ctrl Pts',(-37.7050538275441,-19.3953958606403,
10.4489096280657));
#24475=CARTESIAN_POINT('Origin',(-24.3164988679738,-32.0320676419191,1.04083408558608E-14));
#24476=CARTESIAN_POINT('Ctrl Pts',(-33.8713086176153,-16.7773762111442,
0.));
#24477=CARTESIAN_POINT('Ctrl Pts',(-33.7822911148291,-16.9722973530059,
3.24562220582793));
#24478=CARTESIAN_POINT('Ctrl Pts',(-34.9742380351173,-17.7522153454444,
6.16982677025168));
#24479=CARTESIAN_POINT('Ctrl Pts',(-36.1661849554053,-18.5321333378829,
9.09403133467541));
#24480=CARTESIAN_POINT('Ctrl Pts',(-38.3853855847801,-19.781182380126,11.1176436806954));
#24481=CARTESIAN_POINT('Ctrl Pts',(-40.604586214155,-21.0302314223691,13.1412560267153));
#24482=CARTESIAN_POINT('Ctrl Pts',(-43.3938696431043,-22.5396285557159,
13.8634749112255));
#24483=CARTESIAN_POINT('Ctrl Pts',(-46.1831530720537,-24.0490256890628,
14.5856937957357));
#24484=CARTESIAN_POINT('Ctrl Pts',(-48.9724365010031,-25.5584228224096,
13.8634749112255));
#24485=CARTESIAN_POINT('Ctrl Pts',(-33.594993360669,-15.8658665409932,0.));
#24486=CARTESIAN_POINT('Ctrl Pts',(-33.5059758578829,-16.0607876828549,
3.38941559469372));
#24487=CARTESIAN_POINT('Ctrl Pts',(-34.7546743665351,-16.866623257281,6.44317352589574));
#24488=CARTESIAN_POINT('Ctrl Pts',(-36.0033728751872,-17.6724588317071,
9.49693145709774));
#24489=CARTESIAN_POINT('Ctrl Pts',(-38.3248363332021,-18.9682097429545,
11.6101975146502));
#24490=CARTESIAN_POINT('Ctrl Pts',(-40.6462997912169,-20.2639606542018,
13.7234635722027));
#24491=CARTESIAN_POINT('Ctrl Pts',(-43.5631028816989,-21.8315940656524,
14.4776794959001));
#24492=CARTESIAN_POINT('Ctrl Pts',(-46.4799059721808,-23.399227477103,15.2318954195974));
#24493=CARTESIAN_POINT('Ctrl Pts',(-49.3967090626628,-24.9668608885536,
14.4776794959001));
#24494=CARTESIAN_POINT('Ctrl Pts',(-33.9906638941719,-14.9994689250468,
0.));
#24495=CARTESIAN_POINT('Ctrl Pts',(-33.9016463913857,-15.1943900669085,
3.38941559469371));
#24496=CARTESIAN_POINT('Ctrl Pts',(-35.1503449000379,-16.0002256413346,
6.44317352589574));
#24497=CARTESIAN_POINT('Ctrl Pts',(-36.3990434086901,-16.8060612157607,
9.49693145709774));
#24498=CARTESIAN_POINT('Ctrl Pts',(-38.7205068667049,-18.1018121270081,
11.6101975146502));
#24499=CARTESIAN_POINT('Ctrl Pts',(-41.0419703247197,-19.3975630382554,
13.7234635722027));
#24500=CARTESIAN_POINT('Ctrl Pts',(-43.9587734152017,-20.965196449706,14.4776794959001));
#24501=CARTESIAN_POINT('Ctrl Pts',(-46.8755765056837,-22.5328298611566,
15.2318954195974));
#24502=CARTESIAN_POINT('Ctrl Pts',(-49.7923795961656,-24.1004632726072,
14.4776794959001));
#24503=CARTESIAN_POINT('Ctrl Pts',(-34.8604849513723,-14.6113821712782,
0.));
#24504=CARTESIAN_POINT('Ctrl Pts',(-34.7714674485862,-14.8063033131399,
3.24562220582793));
#24505=CARTESIAN_POINT('Ctrl Pts',(-35.9634143688743,-15.5862213055784,
6.16982677025167));
#24506=CARTESIAN_POINT('Ctrl Pts',(-37.1553612891624,-16.366139298017,9.09403133467541));
#24507=CARTESIAN_POINT('Ctrl Pts',(-39.3745619185372,-17.6151883402601,
11.1176436806954));
#24508=CARTESIAN_POINT('Ctrl Pts',(-41.593762547912,-18.8642373825032,13.1412560267153));
#24509=CARTESIAN_POINT('Ctrl Pts',(-44.3830459768614,-20.37363451585,13.8634749112255));
#24510=CARTESIAN_POINT('Ctrl Pts',(-47.1723294058108,-21.8830316491968,
14.5856937957357));
#24511=CARTESIAN_POINT('Ctrl Pts',(-49.9616128347602,-23.3924287825436,
13.8634749112255));
#24512=CARTESIAN_POINT('',(-33.9565644528763,-15.5074379108284,-5.72595023222876E-30));
#24513=CARTESIAN_POINT('Origin',(-35.5938999782224,-16.2551894587637,0.));
#24514=CARTESIAN_POINT('Origin',(-35.5938999782224,-16.2551894587637,0.));
#24515=CARTESIAN_POINT('Ctrl Pts',(-36.5850719698905,-9.5014950906651,0.));
#24516=CARTESIAN_POINT('Ctrl Pts',(-36.5247007077102,-9.7071007278682,3.24562220582792));
#24517=CARTESIAN_POINT('Ctrl Pts',(-37.8155092299557,-10.3094485465015,
6.16982677025168));
#24518=CARTESIAN_POINT('Ctrl Pts',(-39.1063177522011,-10.9117963651347,
9.09403133467541));
#24519=CARTESIAN_POINT('Ctrl Pts',(-41.4806883314342,-11.8323067104423,
11.1176436806954));
#24520=CARTESIAN_POINT('Ctrl Pts',(-43.8550589106673,-12.7528170557499,
13.1412560267153));
#24521=CARTESIAN_POINT('Ctrl Pts',(-46.8307610650469,-13.8498942825609,
13.8634749112255));
#24522=CARTESIAN_POINT('Ctrl Pts',(-49.8064632194266,-14.9469715093719,
14.5856937957357));
#24523=CARTESIAN_POINT('Ctrl Pts',(-52.7821653738063,-16.044048736183,13.8634749112255));
#24524=CARTESIAN_POINT('Ctrl Pts',(-38.928346550052,-9.86626475512752,0.));
#24525=CARTESIAN_POINT('Ctrl Pts',(-38.8679752878717,-10.0718703923306,
2.7089937269807));
#24526=CARTESIAN_POINT('Ctrl Pts',(-39.9353808672041,-10.6086211883242,
5.14971273833324));
#24527=CARTESIAN_POINT('Ctrl Pts',(-41.0027864465366,-11.1453719843179,
7.59043174968579));
#24528=CARTESIAN_POINT('Ctrl Pts',(-42.9745988326451,-11.9476805791747,
9.27946171175752));
#24529=CARTESIAN_POINT('Ctrl Pts',(-44.9464112187534,-12.7499891740315,
10.9684916738293));
#24530=CARTESIAN_POINT('Ctrl Pts',(-47.4201315169973,-13.6996712289066,
11.5712994880388));
#24531=CARTESIAN_POINT('Ctrl Pts',(-49.8938518152412,-14.6493532837818,
12.1741073022483));
#24532=CARTESIAN_POINT('Ctrl Pts',(-52.367572113485,-15.599035338657,11.5712994880388));
#24533=CARTESIAN_POINT('Ctrl Pts',(-41.297758521112,-9.76686869112041,0.));
#24534=CARTESIAN_POINT('Ctrl Pts',(-41.2373872589317,-9.97247432832351,
2.19648874705824));
#24535=CARTESIAN_POINT('Ctrl Pts',(-42.0914327105681,-10.4465769382888,
4.17545672685568));
#24536=CARTESIAN_POINT('Ctrl Pts',(-42.9454781622045,-10.9206795482542,
6.15442470665314));
#24537=CARTESIAN_POINT('Ctrl Pts',(-44.5328288829012,-11.6101000126269,
7.5239130403414));
#24538=CARTESIAN_POINT('Ctrl Pts',(-46.1201796035978,-12.2995204769996,
8.89340137402967));
#24539=CARTESIAN_POINT('Ctrl Pts',(-48.114484046662,-13.1084333356593,9.3821661014496));
#24540=CARTESIAN_POINT('Ctrl Pts',(-50.1087884897262,-13.917346194319,9.87093082886953));
#24541=CARTESIAN_POINT('Ctrl Pts',(-52.1030929327903,-14.7262590529787,
9.3821661014496));
#24542=CARTESIAN_POINT('Ctrl Pts',(-43.6022501387951,-9.20712674149459,
0.));
#24543=CARTESIAN_POINT('Ctrl Pts',(-43.5418788766148,-9.4127323786977,1.72780310113343));
#24544=CARTESIAN_POINT('Ctrl Pts',(-44.2008065573391,-9.82954324188014,
3.28449990511991));
#24545=CARTESIAN_POINT('Ctrl Pts',(-44.8597342380633,-10.2463541050626,
4.84119670910639));
#24546=CARTESIAN_POINT('Ctrl Pts',(-46.0954948844273,-10.8325384089571,
5.91846432228298));
#24547=CARTESIAN_POINT('Ctrl Pts',(-47.3312555307912,-11.4187227128515,
6.99573193545956));
#24548=CARTESIAN_POINT('Ctrl Pts',(-48.887134322293,-12.0989021850287,7.38020429521639));
#24549=CARTESIAN_POINT('Ctrl Pts',(-50.4430131137947,-12.7790816572059,
7.76467665497321));
#24550=CARTESIAN_POINT('Ctrl Pts',(-51.9988919052965,-13.4592611293832,
7.38020429521639));
#24551=CARTESIAN_POINT('',(-36.5850719699045,-9.50149509067428,1.57948780722887E-9));
#24552=CARTESIAN_POINT('Origin',(-39.3537269950291,8.28430119040637,0.));
#24553=CARTESIAN_POINT('Ctrl Pts',(-36.5850719699168,-9.5014950908766,3.13105117804127E-9));
#24554=CARTESIAN_POINT('Ctrl Pts',(-36.580514057347,-9.51701791573671,0.245038153335549));
#24555=CARTESIAN_POINT('Ctrl Pts',(-36.5819970947817,-9.53446325272415,
0.490791160521871));
#24556=CARTESIAN_POINT('Ctrl Pts',(-36.5896122476098,-9.55382532794269,
0.736766500725606));
#24557=CARTESIAN_POINT('Ctrl Pts',(-36.5972024003189,-9.57312383855566,
0.981934317701291));
#24558=CARTESIAN_POINT('Ctrl Pts',(-36.610884577507,-9.59432652559767,1.22732257376598));
#24559=CARTESIAN_POINT('Ctrl Pts',(-36.6307008654466,-9.61741199666781,
1.47243294816378));
#24560=CARTESIAN_POINT('Ctrl Pts',(-36.650487309385,-9.64046270023612,1.71717417803054));
#24561=CARTESIAN_POINT('Ctrl Pts',(-36.6763894565087,-9.66539050713831,
1.96163791541623));
#24562=CARTESIAN_POINT('Ctrl Pts',(-36.7083998596961,-9.69215854518743,
2.20532408778562));
#24563=CARTESIAN_POINT('Ctrl Pts',(-36.7403828091233,-9.71890362559706,
2.44880126242105));
#24564=CARTESIAN_POINT('Ctrl Pts',(-36.7784635349599,-9.7474857487296,2.6915017543109));
#24565=CARTESIAN_POINT('Ctrl Pts',(-36.8225849430251,-9.7778529268268,2.93292951866849));
#24566=CARTESIAN_POINT('Ctrl Pts',(-36.8666971208038,-9.8082137520498,3.17430677585641));
#24567=CARTESIAN_POINT('Ctrl Pts',(-36.9168473852604,-9.8403588335004,3.41441139318406));
#24568=CARTESIAN_POINT('Ctrl Pts',(-36.9729295663809,-9.87422164256066,
3.65275710614709));
#24569=CARTESIAN_POINT('Ctrl Pts',(-37.029082959759,-9.90812745007487,3.89140546668862));
#24570=CARTESIAN_POINT('Ctrl Pts',(-37.0911832213397,-9.94375528237833,
4.1282900208124));
#24571=CARTESIAN_POINT('Ctrl Pts',(-37.1590759513992,-9.98102464057122,
4.36293874377885));
#24572=CARTESIAN_POINT('Ctrl Pts',(-37.2270379591174,-10.0183320283716,
4.59782690201515));
#24573=CARTESIAN_POINT('Ctrl Pts',(-37.3008040750528,-10.0572842076522,
4.83047425895016));
#24574=CARTESIAN_POINT('Ctrl Pts',(-37.3801738701483,-10.0977878566476,
5.06042975959479));
#24575=CARTESIAN_POINT('Ctrl Pts',(-37.4597757114126,-10.1384099224358,
5.29105755998349));
#24576=CARTESIAN_POINT('Ctrl Pts',(-37.545013812579,-10.1805924445722,5.51897736305729));
#24577=CARTESIAN_POINT('Ctrl Pts',(-37.6356433288454,-10.2242300213429,
5.74376259354369));
#24578=CARTESIAN_POINT('Ctrl Pts',(-37.6934314033805,-10.252054637901,5.88709234072645));
#24579=CARTESIAN_POINT('Ctrl Pts',(-37.7534106234274,-10.2804706155745,
6.02914825314205));
#24580=CARTESIAN_POINT('Ctrl Pts',(-37.8155092299907,-10.3094485465064,
6.16982677023484));
#24581=CARTESIAN_POINT('Ctrl Pts',(-37.912881671843,-10.3548867946545,6.39041482339099));
#24582=CARTESIAN_POINT('Ctrl Pts',(-38.0159808925391,-10.4021550583221,
6.60890054011821));
#24583=CARTESIAN_POINT('Ctrl Pts',(-38.124685183118,-10.4511851399366,6.82480412008066));
#24584=CARTESIAN_POINT('Ctrl Pts',(-38.2331440676597,-10.5001045333898,
7.0402202855931));
#24585=CARTESIAN_POINT('Ctrl Pts',(-38.3471826657451,-10.5507777480891,
7.25306552029649));
#24586=CARTESIAN_POINT('Ctrl Pts',(-38.4666322798727,-10.6031214810715,
7.46287566269424));
#24587=CARTESIAN_POINT('Ctrl Pts',(-38.5858897700796,-10.6553810238848,
7.67234834441891));
#24588=CARTESIAN_POINT('Ctrl Pts',(-38.7105407473184,-10.7093056453534,
7.87879526533041));
#24589=CARTESIAN_POINT('Ctrl Pts',(-38.8403712129408,-10.7647978150927,
8.0817733461221));
#24590=CARTESIAN_POINT('Ctrl Pts',(-38.9700771015593,-10.8202367380982,
8.28455666214101));
#24591=CARTESIAN_POINT('Ctrl Pts',(-39.1049523499259,-10.8772401144473,
8.48387739272821));
#24592=CARTESIAN_POINT('Ctrl Pts',(-39.2447399831758,-10.9356972672492,
8.67931873611038));
#24593=CARTESIAN_POINT('Ctrl Pts',(-39.3845343398413,-10.9941572316855,
8.87476947970425));
#24594=CARTESIAN_POINT('Ctrl Pts',(-39.5292413095781,-11.0540710087837,
9.0663400953275));
#24595=CARTESIAN_POINT('Ctrl Pts',(-39.6785635418394,-11.1153159078427,
9.25364450340895));
#24596=CARTESIAN_POINT('Ctrl Pts',(-39.8279405514878,-11.1765832739883,
9.44101762226374));
#24597=CARTESIAN_POINT('Ctrl Pts',(-39.9819359159948,-11.2391826206559,
9.62412107874879));
#24598=CARTESIAN_POINT('Ctrl Pts',(-40.1402156364337,-11.3029807823644,
9.80260437465941));
#24599=CARTESIAN_POINT('Ctrl Pts',(-40.2987535438811,-11.3668830120892,
9.98137881379501));
#24600=CARTESIAN_POINT('Ctrl Pts',(-40.4615894629167,-11.4319878421543,
10.1555177270907));
#24601=CARTESIAN_POINT('Ctrl Pts',(-40.6283560345695,-11.4981529392408,
10.3247095747691));
#24602=CARTESIAN_POINT('Ctrl Pts',(-40.6765572187095,-11.5172768919413,
10.3736117457744));
#24603=CARTESIAN_POINT('Ctrl Pts',(-40.7250865876881,-11.5364893726199,
10.4221009095751));
#24604=CARTESIAN_POINT('Ctrl Pts',(-40.7739348422943,-11.5557868365701,
10.4701702229111));
#24605=CARTESIAN_POINT('Ctrl Pts',(-41.6582954965893,-15.8276282594346,
0.));
#24606=CARTESIAN_POINT('Ctrl Pts',(-41.597924234409,-16.0332338966377,1.72780310113342));
#24607=CARTESIAN_POINT('Ctrl Pts',(-42.2568519151332,-16.4500447598202,
3.28449990511991));
#24608=CARTESIAN_POINT('Ctrl Pts',(-42.9157795958575,-16.8668556230026,
4.84119670910638));
#24609=CARTESIAN_POINT('Ctrl Pts',(-44.1515402422214,-17.4530399268971,
5.91846432228298));
#24610=CARTESIAN_POINT('Ctrl Pts',(-45.3873008885854,-18.0392242307915,
6.99573193545957));
#24611=CARTESIAN_POINT('Ctrl Pts',(-46.9431796800871,-18.7194037029688,
7.3802042952164));
#24612=CARTESIAN_POINT('Ctrl Pts',(-48.4990584715889,-19.399583175146,7.76467665497322));
#24613=CARTESIAN_POINT('Ctrl Pts',(-50.0549372630907,-20.0797626473232,
7.3802042952164));
#24614=CARTESIAN_POINT('Ctrl Pts',(-40.0222531270434,-14.1108411348343,
0.));
#24615=CARTESIAN_POINT('Ctrl Pts',(-39.9618818648631,-14.3164467720375,
2.19648874705823));
#24616=CARTESIAN_POINT('Ctrl Pts',(-40.8159273164995,-14.7905493820028,
4.17545672685568));
#24617=CARTESIAN_POINT('Ctrl Pts',(-41.6699727681359,-15.2646519919681,
6.15442470665314));
#24618=CARTESIAN_POINT('Ctrl Pts',(-43.2573234888326,-15.9540724563408,
7.5239130403414));
#24619=CARTESIAN_POINT('Ctrl Pts',(-44.8446742095292,-16.6434929207135,
8.89340137402967));
#24620=CARTESIAN_POINT('Ctrl Pts',(-46.8389786525934,-17.4524057793732,
9.3821661014496));
#24621=CARTESIAN_POINT('Ctrl Pts',(-48.8332830956575,-18.2613186380329,
9.87093082886954));
#24622=CARTESIAN_POINT('Ctrl Pts',(-50.8275875387217,-19.0702314966926,
9.38216610144961));
#24623=CARTESIAN_POINT('Ctrl Pts',(-38.0827145049533,-12.7462230199159,
0.));
#24624=CARTESIAN_POINT('Ctrl Pts',(-38.022343242773,-12.951828657119,2.70899372698069));
#24625=CARTESIAN_POINT('Ctrl Pts',(-39.0897488221055,-13.4885794531126,
5.14971273833323));
#24626=CARTESIAN_POINT('Ctrl Pts',(-40.157154401438,-14.0253302491062,7.59043174968578));
#24627=CARTESIAN_POINT('Ctrl Pts',(-42.1289667875464,-14.827638843963,9.27946171175752));
#24628=CARTESIAN_POINT('Ctrl Pts',(-44.1007791736548,-15.6299474388198,
10.9684916738293));
#24629=CARTESIAN_POINT('Ctrl Pts',(-46.5744994718987,-16.579629493695,11.5712994880388));
#24630=CARTESIAN_POINT('Ctrl Pts',(-49.0482197701425,-17.5293115485701,
12.1741073022483));
#24631=CARTESIAN_POINT('Ctrl Pts',(-51.5219400683864,-18.4789936034453,
11.5712994880388));
#24632=CARTESIAN_POINT('Ctrl Pts',(-35.914217116421,-11.7862169042732,0.));
#24633=CARTESIAN_POINT('Ctrl Pts',(-35.8538458542407,-11.9918225414763,
3.24562220582792));
#24634=CARTESIAN_POINT('Ctrl Pts',(-37.1446543764862,-12.5941703601095,
6.16982677025167));
#24635=CARTESIAN_POINT('Ctrl Pts',(-38.4354628987316,-13.1965181787427,
9.09403133467541));
#24636=CARTESIAN_POINT('Ctrl Pts',(-40.8098334779647,-14.1170285240504,
11.1176436806954));
#24637=CARTESIAN_POINT('Ctrl Pts',(-43.1842040571977,-15.037538869358,13.1412560267153));
#24638=CARTESIAN_POINT('Ctrl Pts',(-46.1599062115774,-16.134616096169,13.8634749112255));
#24639=CARTESIAN_POINT('Ctrl Pts',(-49.1356083659571,-17.23169332298,14.5856937957357));
#24640=CARTESIAN_POINT('Ctrl Pts',(-52.1113105203367,-18.328770549791,13.8634749112255));
#24641=CARTESIAN_POINT('',(-35.914217116421,-11.7862169042732,0.));
#24642=CARTESIAN_POINT('Ctrl Pts',(-35.914217116421,-11.7862169042732,0.));
#24643=CARTESIAN_POINT('Ctrl Pts',(-35.8538458542407,-11.9918225414763,
3.24562220582792));
#24644=CARTESIAN_POINT('Ctrl Pts',(-37.1446543764862,-12.5941703601095,
6.16982677025167));
#24645=CARTESIAN_POINT('Ctrl Pts',(-38.2222704208069,-13.0970332266264,
8.61106394926975));
#24646=CARTESIAN_POINT('Ctrl Pts',(-40.0815233709313,-13.831990059078,10.4489096280657));
#24647=CARTESIAN_POINT('Origin',(-28.6276304970126,-28.2454287759837,0.));
#24648=CARTESIAN_POINT('Ctrl Pts',(-35.914217116421,-11.7862169042732,0.));
#24649=CARTESIAN_POINT('Ctrl Pts',(-35.8538458542407,-11.9918225414763,
3.24562220582792));
#24650=CARTESIAN_POINT('Ctrl Pts',(-37.1446543764862,-12.5941703601095,
6.16982677025167));
#24651=CARTESIAN_POINT('Ctrl Pts',(-38.4354628987316,-13.1965181787427,
9.09403133467541));
#24652=CARTESIAN_POINT('Ctrl Pts',(-40.8098334779647,-14.1170285240504,
11.1176436806954));
#24653=CARTESIAN_POINT('Ctrl Pts',(-43.1842040571977,-15.037538869358,13.1412560267153));
#24654=CARTESIAN_POINT('Ctrl Pts',(-46.1599062115774,-16.134616096169,13.8634749112255));
#24655=CARTESIAN_POINT('Ctrl Pts',(-49.1356083659571,-17.23169332298,14.5856937957357));
#24656=CARTESIAN_POINT('Ctrl Pts',(-52.1113105203367,-18.328770549791,13.8634749112255));
#24657=CARTESIAN_POINT('Ctrl Pts',(-35.5109929990848,-10.9233088493806,
0.));
#24658=CARTESIAN_POINT('Ctrl Pts',(-35.4506217369044,-11.1289144865837,
3.38941559469374));
#24659=CARTESIAN_POINT('Ctrl Pts',(-36.8012926546624,-11.7488394904702,
6.44317352589574));
#24660=CARTESIAN_POINT('Ctrl Pts',(-38.1519635724204,-12.3687644943567,
9.49693145709775));
#24661=CARTESIAN_POINT('Ctrl Pts',(-40.6342024610831,-13.3209478330614,
11.6101975146502));
#24662=CARTESIAN_POINT('Ctrl Pts',(-43.1164413497459,-14.273131171766,13.7234635722027));
#24663=CARTESIAN_POINT('Ctrl Pts',(-46.2266530858719,-15.4097039753318,
14.4776794959001));
#24664=CARTESIAN_POINT('Ctrl Pts',(-49.336864821998,-16.5462767788976,15.2318954195974));
#24665=CARTESIAN_POINT('Ctrl Pts',(-52.447076558124,-17.6828495824634,14.4776794959001));
#24666=CARTESIAN_POINT('Ctrl Pts',(-35.7793349404726,-10.0094201239374,
0.));
#24667=CARTESIAN_POINT('Ctrl Pts',(-35.7189636782922,-10.2150257611405,
3.38941559469374));
#24668=CARTESIAN_POINT('Ctrl Pts',(-37.0696345960502,-10.834950765027,6.44317352589574));
#24669=CARTESIAN_POINT('Ctrl Pts',(-38.4203055138082,-11.4548757689135,
9.49693145709775));
#24670=CARTESIAN_POINT('Ctrl Pts',(-40.9025444024709,-12.4070591076181,
11.6101975146502));
#24671=CARTESIAN_POINT('Ctrl Pts',(-43.3847832911337,-13.3592424463228,
13.7234635722027));
#24672=CARTESIAN_POINT('Ctrl Pts',(-46.4949950272597,-14.4958152498886,
14.4776794959001));
#24673=CARTESIAN_POINT('Ctrl Pts',(-49.6052067633858,-15.6323880534543,
15.2318954195974));
#24674=CARTESIAN_POINT('Ctrl Pts',(-52.7154184995118,-16.7689608570201,
14.4776794959001));
#24675=CARTESIAN_POINT('Ctrl Pts',(-36.5850719698906,-9.5014950906651,0.));
#24676=CARTESIAN_POINT('Ctrl Pts',(-36.5247007077102,-9.7071007278682,3.24562220582792));
#24677=CARTESIAN_POINT('Ctrl Pts',(-37.8155092299557,-10.3094485465015,
6.16982677025167));
#24678=CARTESIAN_POINT('Ctrl Pts',(-39.1063177522011,-10.9117963651347,
9.09403133467541));
#24679=CARTESIAN_POINT('Ctrl Pts',(-41.4806883314342,-11.8323067104423,
11.1176436806954));
#24680=CARTESIAN_POINT('Ctrl Pts',(-43.8550589106672,-12.7528170557499,
13.1412560267153));
#24681=CARTESIAN_POINT('Ctrl Pts',(-46.8307610650469,-13.8498942825609,
13.8634749112255));
#24682=CARTESIAN_POINT('Ctrl Pts',(-49.8064632194266,-14.9469715093719,
14.5856937957357));
#24683=CARTESIAN_POINT('Ctrl Pts',(-52.7821653738063,-16.044048736183,13.8634749112255));
#24684=CARTESIAN_POINT('',(-35.817874106385,-10.5170715743355,-8.26137723578747E-30));
#24685=CARTESIAN_POINT('Origin',(-37.5449600575354,-11.024194949205,0.));
#24686=CARTESIAN_POINT('Origin',(-37.5449600575354,-11.024194949205,0.));
#24687=CARTESIAN_POINT('Ctrl Pts',(-37.5648924257372,-4.19818497005524,
0.));
#24688=CARTESIAN_POINT('Ctrl Pts',(-37.5343963889643,-4.410289564744,3.24562220582793));
#24689=CARTESIAN_POINT('Ctrl Pts',(-38.8977893740386,-4.82280514501228,
6.16982677025168));
#24690=CARTESIAN_POINT('Ctrl Pts',(-40.2611823591128,-5.23532072528053,
9.09403133467541));
#24691=CARTESIAN_POINT('Ctrl Pts',(-42.7423875503303,-5.80855343755483,
11.1176436806954));
#24692=CARTESIAN_POINT('Ctrl Pts',(-45.2235927415478,-6.38178614982912,
13.1412560267153));
#24693=CARTESIAN_POINT('Ctrl Pts',(-48.3251369067109,-7.04421014147591,
13.8634749112255));
#24694=CARTESIAN_POINT('Ctrl Pts',(-51.4266810718741,-7.70663413312271,
14.5856937957357));
#24695=CARTESIAN_POINT('Ctrl Pts',(-54.5282252370373,-8.36905812476951,
13.8634749112255));
#24696=CARTESIAN_POINT('Ctrl Pts',(-39.9362279852005,-4.22575906238229,
-1.05434036998093E-14));
#24697=CARTESIAN_POINT('Ctrl Pts',(-39.9057319484276,-4.43786365707106,
2.70899372698069));
#24698=CARTESIAN_POINT('Ctrl Pts',(-41.0386604807592,-4.8172434514975,5.14971273833323));
#24699=CARTESIAN_POINT('Ctrl Pts',(-42.1715890130907,-5.19662324592393,
7.59043174968578));
#24700=CARTESIAN_POINT('Ctrl Pts',(-44.2375116101495,-5.71014733528427,
9.27946171175751));
#24701=CARTESIAN_POINT('Ctrl Pts',(-46.3034342072083,-6.22367142464463,
10.9684916738292));
#24702=CARTESIAN_POINT('Ctrl Pts',(-48.8871294476768,-6.81163998135168,
11.5712994880388));
#24703=CARTESIAN_POINT('Ctrl Pts',(-51.4708246881452,-7.39960853805875,
12.1741073022483));
#24704=CARTESIAN_POINT('Ctrl Pts',(-54.0545199286137,-7.9875770947658,11.5712994880388));
#24705=CARTESIAN_POINT('Ctrl Pts',(-42.2673772240309,-3.79017222552529,
0.));
#24706=CARTESIAN_POINT('Ctrl Pts',(-42.2368811872581,-4.00227682021405,
2.19648874705824));
#24707=CARTESIAN_POINT('Ctrl Pts',(-43.1497055238908,-4.35001040888178,
4.17545672685567));
#24708=CARTESIAN_POINT('Ctrl Pts',(-44.0625298605235,-4.6977439975495,6.15442470665313));
#24709=CARTESIAN_POINT('Ctrl Pts',(-45.7318384015437,-5.15424359455821,
7.5239130403414));
#24710=CARTESIAN_POINT('Ctrl Pts',(-47.4011469425639,-5.61074319156689,
8.89340137402966));
#24711=CARTESIAN_POINT('Ctrl Pts',(-49.4902725446046,-6.1276033693991,9.3821661014496));
#24712=CARTESIAN_POINT('Ctrl Pts',(-51.5793981466452,-6.64446354723128,
9.87093082886953));
#24713=CARTESIAN_POINT('Ctrl Pts',(-53.6685237486859,-7.16132372506348,
9.3821661014496));
#24714=CARTESIAN_POINT('Ctrl Pts',(-44.4687528548128,-2.90816428999269,
0.));
#24715=CARTESIAN_POINT('Ctrl Pts',(-44.4382568180399,-3.12026888468146,
1.72780310113343));
#24716=CARTESIAN_POINT('Ctrl Pts',(-45.149795935654,-3.43906202795228,3.28449990511991));
#24717=CARTESIAN_POINT('Ctrl Pts',(-45.8613350532681,-3.75785517122311,
4.84119670910638));
#24718=CARTESIAN_POINT('Ctrl Pts',(-47.1679401624789,-4.16220588758012,
5.91846432228298));
#24719=CARTESIAN_POINT('Ctrl Pts',(-48.4745452716896,-4.56655660393713,
6.99573193545956));
#24720=CARTESIAN_POINT('Ctrl Pts',(-50.1113870920655,-5.01838819123999,
7.38020429521639));
#24721=CARTESIAN_POINT('Ctrl Pts',(-51.7482289124415,-5.47021977854284,
7.76467665497321));
#24722=CARTESIAN_POINT('Ctrl Pts',(-53.3850707328175,-5.9220513658457,7.38020429521639));
#24723=CARTESIAN_POINT('',(-37.5648924257618,-4.19818497005579,1.57948609960414E-9));
#24724=CARTESIAN_POINT('Origin',(-37.7741838134884,13.8005982420126,0.));
#24725=CARTESIAN_POINT('Ctrl Pts',(-37.5648924257933,-4.19818497026086,
3.13104702311909E-9));
#24726=CARTESIAN_POINT('Ctrl Pts',(-37.562590034511,-4.21419845373618,0.245038153335525));
#24727=CARTESIAN_POINT('Ctrl Pts',(-37.5665407070749,-4.23125516411452,
0.490791160521828));
#24728=CARTESIAN_POINT('Ctrl Pts',(-37.5768338592308,-4.24933641208198,
0.736766500725544));
#24729=CARTESIAN_POINT('Ctrl Pts',(-37.5870932195462,-4.26735830032779,
0.981934317701182));
#24730=CARTESIAN_POINT('Ctrl Pts',(-37.6036535888759,-4.28639799775371,
1.22732257376582));
#24731=CARTESIAN_POINT('Ctrl Pts',(-37.6265535806588,-4.30642834020156,
1.47243294816358));
#24732=CARTESIAN_POINT('Ctrl Pts',(-37.649419084278,-4.32642851627481,1.71717417803032));
#24733=CARTESIAN_POINT('Ctrl Pts',(-37.6786051816996,-4.34741633416683,
1.96163791541599));
#24734=CARTESIAN_POINT('Ctrl Pts',(-37.7140992541435,-4.36935635683226,
2.20532408778536));
#24735=CARTESIAN_POINT('Ctrl Pts',(-37.7495628850543,-4.39127756261129,
2.44880126242071));
#24736=CARTESIAN_POINT('Ctrl Pts',(-37.7913236642409,-4.41414930860358,
2.69150175431049));
#24737=CARTESIAN_POINT('Ctrl Pts',(-37.8393176800295,-4.43792826156041,
2.93292951866801));
#24738=CARTESIAN_POINT('Ctrl Pts',(-37.8873016553743,-4.46170223991287,
3.17430677585588));
#24739=CARTESIAN_POINT('Ctrl Pts',(-37.9415161845174,-4.48638300400817,
3.41441139318348));
#24740=CARTESIAN_POINT('Ctrl Pts',(-38.0018467100928,-4.51191981196215,
3.65275710614646));
#24741=CARTESIAN_POINT('Ctrl Pts',(-38.0622538424057,-4.5374890461469,3.89140546668795));
#24742=CARTESIAN_POINT('Ctrl Pts',(-38.1287923820569,-4.56391644980501,
4.12829002081169));
#24743=CARTESIAN_POINT('Ctrl Pts',(-38.2012980447014,-4.59114431677112,
4.36293874377811));
#24744=CARTESIAN_POINT('Ctrl Pts',(-38.2738776920354,-4.61839996701937,
4.59782690201448));
#24745=CARTESIAN_POINT('Ctrl Pts',(-38.3524364483672,-4.64645765641992,
4.83047425894955));
#24746=CARTESIAN_POINT('Ctrl Pts',(-38.4367626436466,-4.67525353711722,
5.06042975959425));
#24747=CARTESIAN_POINT('Ctrl Pts',(-38.5213353756662,-4.70413360568203,
5.29105755998295));
#24748=CARTESIAN_POINT('Ctrl Pts',(-38.6117090746818,-4.73375612398307,
5.51897736305675));
#24749=CARTESIAN_POINT('Ctrl Pts',(-38.7076263878303,-4.7640516081922,5.74376259354315));
#24750=CARTESIAN_POINT('Ctrl Pts',(-38.7687861188958,-4.78336890979197,
5.88709234072609));
#24751=CARTESIAN_POINT('Ctrl Pts',(-38.8321988522325,-4.80295972078441,
6.02914825314188));
#24752=CARTESIAN_POINT('Ctrl Pts',(-38.8977893740739,-4.82280514501219,
6.16982677023484));
#24753=CARTESIAN_POINT('Ctrl Pts',(-39.0006372418043,-4.8539233539962,6.39041482339094));
#24754=CARTESIAN_POINT('Ctrl Pts',(-39.1094140363897,-4.88603794597538,
6.60890054011812));
#24755=CARTESIAN_POINT('Ctrl Pts',(-39.2239895821647,-4.91909873852119,
6.82480412008052));
#24756=CARTESIAN_POINT('Ctrl Pts',(-39.3383064672143,-4.95208489447222,
7.04022028559309));
#24757=CARTESIAN_POINT('Ctrl Pts',(-39.458395867156,-4.98601294426717,7.25306552029659));
#24758=CARTESIAN_POINT('Ctrl Pts',(-39.5840789463381,-5.02082444100485,
7.46287566269445));
#24759=CARTESIAN_POINT('Ctrl Pts',(-39.7095598756334,-5.05557994659266,
7.67234834441904));
#24760=CARTESIAN_POINT('Ctrl Pts',(-39.840616359439,-5.0912160095013,7.87879526533046));
#24761=CARTESIAN_POINT('Ctrl Pts',(-39.9770226972832,-5.12766654724775,
8.08177334612208));
#24762=CARTESIAN_POINT('Ctrl Pts',(-40.1132981483379,-5.16408210939161,
8.28455666214132));
#24763=CARTESIAN_POINT('Ctrl Pts',(-40.2549129874365,-5.20131052440325,
8.48387739272884));
#24764=CARTESIAN_POINT('Ctrl Pts',(-40.4015971043843,-5.23927881325933,
8.67931873611132));
#24765=CARTESIAN_POINT('Ctrl Pts',(-40.5482882764499,-5.27724892828962,
8.87476947970519));
#24766=CARTESIAN_POINT('Ctrl Pts',(-40.7000489573831,-5.31595892053044,
9.06634009532845));
#24767=CARTESIAN_POINT('Ctrl Pts',(-40.8565673625296,-5.35532966548994,
9.2536445034099));
#24768=CARTESIAN_POINT('Ctrl Pts',(-41.0131431849084,-5.39471485321869,
9.44101762226499));
#24769=CARTESIAN_POINT('Ctrl Pts',(-41.174479914545,-5.4347612034034,9.62412107875033));
#24770=CARTESIAN_POINT('Ctrl Pts',(-41.3402280007163,-5.47538443899895,
9.80260437466121));
#24771=CARTESIAN_POINT('Ctrl Pts',(-41.5062464563473,-5.516073939506,9.98137881379674));
#24772=CARTESIAN_POINT('Ctrl Pts',(-41.6766903238786,-5.55734212879185,
10.1555177270924));
#24773=CARTESIAN_POINT('Ctrl Pts',(-41.8511757273807,-5.59910040291801,
10.3247095747707));
#24774=CARTESIAN_POINT('Ctrl Pts',(-41.9016079151999,-5.61116995762843,
10.3736117457738));
#24775=CARTESIAN_POINT('Ctrl Pts',(-41.9523775462543,-5.62328043365766,
10.4221009095724));
#24776=CARTESIAN_POINT('Ctrl Pts',(-42.0034749115207,-5.63542964579464,
10.4701702229062));
#24777=CARTESIAN_POINT('Ctrl Pts',(-43.4867804707271,-9.73793223897115,
0.));
#24778=CARTESIAN_POINT('Ctrl Pts',(-43.4562844339543,-9.95003683365991,
1.72780310113343));
#24779=CARTESIAN_POINT('Ctrl Pts',(-44.1678235515683,-10.2688299769307,
3.28449990511991));
#24780=CARTESIAN_POINT('Ctrl Pts',(-44.8793626691824,-10.5876231202016,
4.84119670910639));
#24781=CARTESIAN_POINT('Ctrl Pts',(-46.1859677783932,-10.9919738365586,
5.91846432228298));
#24782=CARTESIAN_POINT('Ctrl Pts',(-47.492572887604,-11.3963245529156,6.99573193545957));
#24783=CARTESIAN_POINT('Ctrl Pts',(-49.1294147079799,-11.8481561402184,
7.3802042952164));
#24784=CARTESIAN_POINT('Ctrl Pts',(-50.7662565283558,-12.2999877275213,
7.76467665497322));
#24785=CARTESIAN_POINT('Ctrl Pts',(-52.4030983487318,-12.7518193148241,
7.38020429521639));
#24786=CARTESIAN_POINT('Ctrl Pts',(-41.6230663715377,-8.27145263712683,
0.));
#24787=CARTESIAN_POINT('Ctrl Pts',(-41.5925703347649,-8.4835572318156,2.19648874705823));
#24788=CARTESIAN_POINT('Ctrl Pts',(-42.5053946713976,-8.83129082048332,
4.17545672685568));
#24789=CARTESIAN_POINT('Ctrl Pts',(-43.4182190080304,-9.17902440915105,
6.15442470665314));
#24790=CARTESIAN_POINT('Ctrl Pts',(-45.0875275490506,-9.63552400615975,
7.52391304034141));
#24791=CARTESIAN_POINT('Ctrl Pts',(-46.7568360900708,-10.0920236031684,
8.89340137402968));
#24792=CARTESIAN_POINT('Ctrl Pts',(-48.8459616921114,-10.6088837810006,
9.38216610144961));
#24793=CARTESIAN_POINT('Ctrl Pts',(-50.9350872941521,-11.1257439588328,
9.87093082886955));
#24794=CARTESIAN_POINT('Ctrl Pts',(-53.0242128961928,-11.642604136665,9.38216610144961));
#24795=CARTESIAN_POINT('Ctrl Pts',(-39.5090640497074,-7.19674949232894,
0.));
#24796=CARTESIAN_POINT('Ctrl Pts',(-39.4785680129345,-7.40885408701771,
2.7089937269807));
#24797=CARTESIAN_POINT('Ctrl Pts',(-40.611496545266,-7.78823388144414,5.14971273833323));
#24798=CARTESIAN_POINT('Ctrl Pts',(-41.7444250775976,-8.16761367587058,
7.59043174968577));
#24799=CARTESIAN_POINT('Ctrl Pts',(-43.8103476746564,-8.68113776523092,
9.27946171175751));
#24800=CARTESIAN_POINT('Ctrl Pts',(-45.8762702717152,-9.19466185459128,
10.9684916738293));
#24801=CARTESIAN_POINT('Ctrl Pts',(-48.4599655121837,-9.78263041129834,
11.5712994880388));
#24802=CARTESIAN_POINT('Ctrl Pts',(-51.0436607526521,-10.3705989680054,
12.1741073022483));
#24803=CARTESIAN_POINT('Ctrl Pts',(-53.6273559931206,-10.9585675247124,
11.5712994880388));
#24804=CARTESIAN_POINT('Ctrl Pts',(-37.2260157227863,-6.55512420987395,
0.));
#24805=CARTESIAN_POINT('Ctrl Pts',(-37.1955196860134,-6.76722880456271,
3.24562220582793));
#24806=CARTESIAN_POINT('Ctrl Pts',(-38.5589126710876,-7.17974438483098,
6.16982677025168));
#24807=CARTESIAN_POINT('Ctrl Pts',(-39.9223056561618,-7.59225996509924,
9.09403133467541));
#24808=CARTESIAN_POINT('Ctrl Pts',(-42.4035108473793,-8.16549267737354,
11.1176436806954));
#24809=CARTESIAN_POINT('Ctrl Pts',(-44.8847160385968,-8.73872538964782,
13.1412560267153));
#24810=CARTESIAN_POINT('Ctrl Pts',(-47.98626020376,-9.40114938129462,13.8634749112255));
#24811=CARTESIAN_POINT('Ctrl Pts',(-51.0878043689232,-10.0635733729414,
14.5856937957357));
#24812=CARTESIAN_POINT('Ctrl Pts',(-54.1893485340864,-10.7259973645882,
13.8634749112255));
#24813=CARTESIAN_POINT('',(-37.2260157227863,-6.55512420987395,0.));
#24814=CARTESIAN_POINT('Ctrl Pts',(-37.2260157227863,-6.55512420987395,
0.));
#24815=CARTESIAN_POINT('Ctrl Pts',(-37.1955196860134,-6.76722880456271,
3.24562220582793));
#24816=CARTESIAN_POINT('Ctrl Pts',(-38.5589126710876,-7.17974438483098,
6.16982677025168));
#24817=CARTESIAN_POINT('Ctrl Pts',(-39.6971249853932,-7.52412807936691,
8.61106394926976));
#24818=CARTESIAN_POINT('Ctrl Pts',(-41.6420486840548,-7.98700482807827,
10.4489096280657));
#24819=CARTESIAN_POINT('Origin',(-32.3559861244012,-23.8837944332597,1.04083408558608E-14));
#24820=CARTESIAN_POINT('Ctrl Pts',(-37.2260157227863,-6.55512420987395,
0.));
#24821=CARTESIAN_POINT('Ctrl Pts',(-37.1955196860134,-6.76722880456271,
3.24562220582793));
#24822=CARTESIAN_POINT('Ctrl Pts',(-38.5589126710876,-7.17974438483098,
6.16982677025168));
#24823=CARTESIAN_POINT('Ctrl Pts',(-39.9223056561618,-7.59225996509924,
9.09403133467541));
#24824=CARTESIAN_POINT('Ctrl Pts',(-42.4035108473793,-8.16549267737352,
11.1176436806954));
#24825=CARTESIAN_POINT('Ctrl Pts',(-44.8847160385968,-8.73872538964782,
13.1412560267153));
#24826=CARTESIAN_POINT('Ctrl Pts',(-47.98626020376,-9.40114938129462,13.8634749112255));
#24827=CARTESIAN_POINT('Ctrl Pts',(-51.0878043689232,-10.0635733729414,
14.5856937957357));
#24828=CARTESIAN_POINT('Ctrl Pts',(-54.1893485340864,-10.7259973645882,
13.8634749112255));
#24829=CARTESIAN_POINT('Ctrl Pts',(-36.7040912252865,-5.75838408981617,
6.24500451351651E-15));
#24830=CARTESIAN_POINT('Ctrl Pts',(-36.6735951885137,-5.97048868450495,
3.38941559469373));
#24831=CARTESIAN_POINT('Ctrl Pts',(-38.0987427505052,-6.39188323248875,
6.44317352589574));
#24832=CARTESIAN_POINT('Ctrl Pts',(-39.5238903124967,-6.81327778047256,
9.49693145709775));
#24833=CARTESIAN_POINT('Ctrl Pts',(-42.1163734062201,-7.40250983972848,
11.6101975146502));
#24834=CARTESIAN_POINT('Ctrl Pts',(-44.7088564999434,-7.99174189898442,
13.7234635722027));
#24835=CARTESIAN_POINT('Ctrl Pts',(-47.949161939876,-8.67411674999011,14.4776794959001));
#24836=CARTESIAN_POINT('Ctrl Pts',(-51.1894673798085,-9.35649160099581,
15.2318954195974));
#24837=CARTESIAN_POINT('Ctrl Pts',(-54.429772819741,-10.0388664520015,14.4776794959001));
#24838=CARTESIAN_POINT('Ctrl Pts',(-36.8396419064669,-4.81560839388869,
0.));
#24839=CARTESIAN_POINT('Ctrl Pts',(-36.8091458696941,-5.02771298857746,
3.38941559469373));
#24840=CARTESIAN_POINT('Ctrl Pts',(-38.2342934316856,-5.44910753656127,
6.44317352589573));
#24841=CARTESIAN_POINT('Ctrl Pts',(-39.6594409936771,-5.87050208454507,
9.49693145709775));
#24842=CARTESIAN_POINT('Ctrl Pts',(-42.2519240874005,-6.459734143801,11.6101975146502));
#24843=CARTESIAN_POINT('Ctrl Pts',(-44.8444071811238,-7.04896620305693,
13.7234635722027));
#24844=CARTESIAN_POINT('Ctrl Pts',(-48.0847126210563,-7.73134105406263,
14.4776794959001));
#24845=CARTESIAN_POINT('Ctrl Pts',(-51.3250180609889,-8.41371590506832,
15.2318954195974));
#24846=CARTESIAN_POINT('Ctrl Pts',(-54.5653235009214,-9.09609075607403,
14.4776794959001));
#24847=CARTESIAN_POINT('Ctrl Pts',(-37.5648924257372,-4.19818497005524,
0.));
#24848=CARTESIAN_POINT('Ctrl Pts',(-37.5343963889643,-4.41028956474401,
3.24562220582793));
#24849=CARTESIAN_POINT('Ctrl Pts',(-38.8977893740386,-4.82280514501228,
6.16982677025168));
#24850=CARTESIAN_POINT('Ctrl Pts',(-40.2611823591128,-5.23532072528053,
9.09403133467541));
#24851=CARTESIAN_POINT('Ctrl Pts',(-42.7423875503303,-5.80855343755483,
11.1176436806954));
#24852=CARTESIAN_POINT('Ctrl Pts',(-45.2235927415478,-6.38178614982912,
13.1412560267153));
#24853=CARTESIAN_POINT('Ctrl Pts',(-48.3251369067109,-7.04421014147591,
13.8634749112255));
#24854=CARTESIAN_POINT('Ctrl Pts',(-51.4266810718741,-7.70663413312271,
14.5856937957357));
#24855=CARTESIAN_POINT('Ctrl Pts',(-54.5282252370373,-8.36905812476951,
13.8634749112255));
#24856=CARTESIAN_POINT('',(-36.9500351333142,-5.31260798924485,-1.06286264220349E-29));
#24857=CARTESIAN_POINT('Origin',(-38.731713020801,-5.56877962163353,0.));
#24858=CARTESIAN_POINT('Origin',(-38.731713020801,-5.56877962163353,0.));
#24859=CARTESIAN_POINT('Ctrl Pts',(-37.7800000000001,1.19058808997921,0.));
#24860=CARTESIAN_POINT('Ctrl Pts',(-37.78,0.976302375693506,3.24562220582793));
#24861=CARTESIAN_POINT('Ctrl Pts',(-39.1882226984277,0.762016661407787,
6.16982677025167));
#24862=CARTESIAN_POINT('Ctrl Pts',(-40.5964453968553,0.547730947122094,
9.09403133467541));
#24863=CARTESIAN_POINT('Ctrl Pts',(-43.1339750175689,0.333445232836368,
11.1176436806954));
#24864=CARTESIAN_POINT('Ctrl Pts',(-45.6715046382825,0.119159518550672,
13.1412560267153));
#24865=CARTESIAN_POINT('Ctrl Pts',(-48.8357523191413,-0.0951261957350281,
13.8634749112255));
#24866=CARTESIAN_POINT('Ctrl Pts',(-52.0000000000001,-0.309411910020729,
14.5856937957357));
#24867=CARTESIAN_POINT('Ctrl Pts',(-55.1642476808589,-0.52369762430643,
13.8634749112255));
#24868=CARTESIAN_POINT('Ctrl Pts',(-40.1311229851416,1.5007708987902,0.));
#24869=CARTESIAN_POINT('Ctrl Pts',(-40.1311229851416,1.2864851845045,2.70899372698069));
#24870=CARTESIAN_POINT('Ctrl Pts',(-41.30651131265,1.07219947021879,5.14971273833323));
#24871=CARTESIAN_POINT('Ctrl Pts',(-42.4818996401584,0.857913755933074,
7.59043174968577));
#24872=CARTESIAN_POINT('Ctrl Pts',(-44.5998762217203,0.643628041647366,
9.27946171175751));
#24873=CARTESIAN_POINT('Ctrl Pts',(-46.7178528032822,0.429342327361657,
10.9684916738292));
#24874=CARTESIAN_POINT('Ctrl Pts',(-49.3589264016411,0.215056613075952,
11.5712994880388));
#24875=CARTESIAN_POINT('Ctrl Pts',(-52.0000000000001,0.000770898790245644,
12.1741073022483));
#24876=CARTESIAN_POINT('Ctrl Pts',(-54.641073598359,-0.213514815495465,
11.5712994880388));
#24877=CARTESIAN_POINT('Ctrl Pts',(-42.3765540157191,2.26368121662741,0.));
#24878=CARTESIAN_POINT('Ctrl Pts',(-42.3765540157191,2.04939550234168,2.19648874705823));
#24879=CARTESIAN_POINT('Ctrl Pts',(-43.3295747662223,1.83510978805599,4.17545672685568));
#24880=CARTESIAN_POINT('Ctrl Pts',(-44.2825955167256,1.62082407377026,6.15442470665314));
#24881=CARTESIAN_POINT('Ctrl Pts',(-45.9998795700625,1.40653835948456,7.5239130403414));
#24882=CARTESIAN_POINT('Ctrl Pts',(-47.7171636233994,1.19225264519886,8.89340137402968));
#24883=CARTESIAN_POINT('Ctrl Pts',(-49.8585818116997,0.977966930913157,
9.3821661014496));
#24884=CARTESIAN_POINT('Ctrl Pts',(-52.0000000000001,0.763681216627436,
9.87093082886954));
#24885=CARTESIAN_POINT('Ctrl Pts',(-54.1414181883004,0.54939550234174,9.3821661014496));
#24886=CARTESIAN_POINT('Ctrl Pts',(-44.43,3.45000000000016,0.));
#24887=CARTESIAN_POINT('Ctrl Pts',(-44.43,3.23571428571445,1.72780310113342));
#24888=CARTESIAN_POINT('Ctrl Pts',(-45.1796656699787,3.02142857142873,3.28449990511991));
#24889=CARTESIAN_POINT('Ctrl Pts',(-45.9293313399574,2.80714285714304,4.84119670910638));
#24890=CARTESIAN_POINT('Ctrl Pts',(-47.2801821999295,2.59285714285731,5.91846432228297));
#24891=CARTESIAN_POINT('Ctrl Pts',(-48.6310330599015,2.37857142857161,6.99573193545956));
#24892=CARTESIAN_POINT('Ctrl Pts',(-50.3155165299508,2.1642857142859,7.38020429521639));
#24893=CARTESIAN_POINT('Ctrl Pts',(-52.0000000000001,1.95000000000019,7.76467665497321));
#24894=CARTESIAN_POINT('Ctrl Pts',(-53.6844834700493,1.73571428571448,7.38020429521638));
#24895=CARTESIAN_POINT('',(-37.7800000000897,1.19058809004707,1.57948074790763E-9));
#24896=CARTESIAN_POINT('Origin',(-35.4256671812559,19.0359549110503,0.));
#24897=CARTESIAN_POINT('Ctrl Pts',(-37.7800000000849,1.19058808978368,3.13103676972182E-9));
#24898=CARTESIAN_POINT('Ctrl Pts',(-37.780000000137,1.17440993603763,0.24503815333525));
#24899=CARTESIAN_POINT('Ctrl Pts',(-37.7863378835296,1.15808907770421,0.490791160521286));
#24900=CARTESIAN_POINT('Ctrl Pts',(-37.7990994961183,1.14165673905446,0.736766500724735));
#24901=CARTESIAN_POINT('Ctrl Pts',(-37.8118192130495,1.12527834684966,0.981934317700371));
#24902=CARTESIAN_POINT('Ctrl Pts',(-37.8309206531574,1.10878923237345,1.22732257376501));
#24903=CARTESIAN_POINT('Ctrl Pts',(-37.8564381709891,1.0922217785574,1.47243294816276));
#24904=CARTESIAN_POINT('Ctrl Pts',(-37.881917258574,1.0756792758883,1.71717417802952));
#24905=CARTESIAN_POINT('Ctrl Pts',(-37.9137931615158,1.05905869845488,1.96163791541521));
#24906=CARTESIAN_POINT('Ctrl Pts',(-37.9520483462578,1.0423933267648,2.2053240877846));
#24907=CARTESIAN_POINT('Ctrl Pts',(-37.9902707213954,1.02574224815047,2.44880126242));
#24908=CARTESIAN_POINT('Ctrl Pts',(-38.0348614248958,1.00904648209016,2.69150175430983));
#24909=CARTESIAN_POINT('Ctrl Pts',(-38.0857510286497,0.992339825183044,
2.9329295186674));
#24910=CARTESIAN_POINT('Ctrl Pts',(-38.1366299861971,0.975636663341864,
3.17430677585535));
#24911=CARTESIAN_POINT('Ctrl Pts',(-38.1938051285551,0.95892264578539,3.41441139318303));
#24912=CARTESIAN_POINT('Ctrl Pts',(-38.2571558430635,0.942231694705537,
3.6527571061461));
#24913=CARTESIAN_POINT('Ctrl Pts',(-38.3205869992972,0.925519549722661,
3.89140546668762));
#24914=CARTESIAN_POINT('Ctrl Pts',(-38.390209284233,0.908830560438021,4.12829002081138));
#24915=CARTESIAN_POINT('Ctrl Pts',(-38.4658518732601,0.89219846555144,4.36293874377782));
#24916=CARTESIAN_POINT('Ctrl Pts',(-38.5415716478926,0.875549399295574,
4.59782690201425));
#24917=CARTESIAN_POINT('Ctrl Pts',(-38.6233238148867,0.858957373419583,
4.83047425894938));
#24918=CARTESIAN_POINT('Ctrl Pts',(-38.7108897721909,0.842455462110944,
5.06042975959413));
#24919=CARTESIAN_POINT('Ctrl Pts',(-38.7987117380295,0.82590530568219,5.29105755998297));
#24920=CARTESIAN_POINT('Ctrl Pts',(-38.8923812869985,0.809445820264863,
5.51897736305691));
#24921=CARTESIAN_POINT('Ctrl Pts',(-38.9916337971362,0.79310915731082,5.74376259354344));
#24922=CARTESIAN_POINT('Ctrl Pts',(-39.0549201489775,0.782692415223513,
5.88709234072628));
#24923=CARTESIAN_POINT('Ctrl Pts',(-39.1204754952205,0.772325583328654,
6.02914825314197));
#24924=CARTESIAN_POINT('Ctrl Pts',(-39.1882226984626,0.762016661412907,
6.16982677023484));
#24925=CARTESIAN_POINT('Ctrl Pts',(-39.2944523060728,0.745851968590391,
6.390414823391));
#24926=CARTESIAN_POINT('Ctrl Pts',(-39.4066922926963,0.729544808781451,
6.60890054011824));
#24927=CARTESIAN_POINT('Ctrl Pts',(-39.524806665964,0.713126327701068,6.82480412008069));
#24928=CARTESIAN_POINT('Ctrl Pts',(-39.6426543894045,0.696744912263256,
7.04022028559321));
#24929=CARTESIAN_POINT('Ctrl Pts',(-39.766349917329,0.68025270462606,7.25306552029667));
#24930=CARTESIAN_POINT('Ctrl Pts',(-39.8957079165132,0.663682105818622,
7.46287566269449));
#24931=CARTESIAN_POINT('Ctrl Pts',(-40.0248578550338,0.647138159323428,
7.6723483444192));
#24932=CARTESIAN_POINT('Ctrl Pts',(-40.1596519133317,0.630516102449693,
7.87879526533074));
#24933=CARTESIAN_POINT('Ctrl Pts',(-40.2998572837228,0.613849224529908,
8.08177334612247));
#24934=CARTESIAN_POINT('Ctrl Pts',(-40.4399281220159,0.597198339079233,
8.28455666214167));
#24935=CARTESIAN_POINT('Ctrl Pts',(-40.5853996821057,0.580502748576888,
8.48387739272915));
#24936=CARTESIAN_POINT('Ctrl Pts',(-40.735994217132,0.5637962485363,8.6793187361116));
#24937=CARTESIAN_POINT('Ctrl Pts',(-40.8865959953569,0.547088944957281,
8.87476947970534));
#24938=CARTESIAN_POINT('Ctrl Pts',(-41.0423209776643,0.53037076138554,9.06634009532848));
#24939=CARTESIAN_POINT('Ctrl Pts',(-41.2028492923288,0.513675645357026,
9.2536445034098));
#24940=CARTESIAN_POINT('Ctrl Pts',(-41.3634364952214,0.496974404889944,
9.44101762226492));
#24941=CARTESIAN_POINT('Ctrl Pts',(-41.5288302394286,0.480296279393814,
9.62412107875029));
#24942=CARTESIAN_POINT('Ctrl Pts',(-41.6986725382757,0.463674941840322,
9.8026043746612));
#24943=CARTESIAN_POINT('Ctrl Pts',(-41.8687918850914,0.44702649144251,9.98137881379691));
#24944=CARTESIAN_POINT('Ctrl Pts',(-42.0433739554953,0.430435044262166,
10.1555177270927));
#24945=CARTESIAN_POINT('Ctrl Pts',(-42.2220261712059,0.413933671136578,
10.3247095747712));
#24946=CARTESIAN_POINT('Ctrl Pts',(-42.2736627087968,0.409164215743528,
10.3736117457741));
#24947=CARTESIAN_POINT('Ctrl Pts',(-42.3256390786481,0.404402278731116,
10.4221009095725));
#24948=CARTESIAN_POINT('Ctrl Pts',(-42.3779453595728,0.399648641330075,
10.4701702229062));
#24949=CARTESIAN_POINT('Ctrl Pts',(-44.4300000000001,-3.44999999999985,
0.));
#24950=CARTESIAN_POINT('Ctrl Pts',(-44.4300000000001,-3.66428571428556,
1.72780310113342));
#24951=CARTESIAN_POINT('Ctrl Pts',(-45.1796656699787,-3.87857142857126,
3.28449990511991));
#24952=CARTESIAN_POINT('Ctrl Pts',(-45.9293313399574,-4.09285714285698,
4.84119670910638));
#24953=CARTESIAN_POINT('Ctrl Pts',(-47.2801821999295,-4.30714285714269,
5.91846432228298));
#24954=CARTESIAN_POINT('Ctrl Pts',(-48.6310330599015,-4.52142857142839,
6.99573193545956));
#24955=CARTESIAN_POINT('Ctrl Pts',(-50.3155165299508,-4.73571428571411,
7.38020429521639));
#24956=CARTESIAN_POINT('Ctrl Pts',(-52.0000000000001,-4.94999999999981,
7.76467665497322));
#24957=CARTESIAN_POINT('Ctrl Pts',(-53.6844834700494,-5.16428571428552,
7.38020429521639));
#24958=CARTESIAN_POINT('Ctrl Pts',(-42.3765540157191,-2.2636812166271,0.));
#24959=CARTESIAN_POINT('Ctrl Pts',(-42.3765540157191,-2.47796693091281,
2.19648874705822));
#24960=CARTESIAN_POINT('Ctrl Pts',(-43.3295747662224,-2.69225264519852,
4.17545672685568));
#24961=CARTESIAN_POINT('Ctrl Pts',(-44.2825955167256,-2.90653835948424,
6.15442470665314));
#24962=CARTESIAN_POINT('Ctrl Pts',(-45.9998795700625,-3.12082407376995,
7.52391304034139));
#24963=CARTESIAN_POINT('Ctrl Pts',(-47.7171636233994,-3.33510978805565,
8.89340137402966));
#24964=CARTESIAN_POINT('Ctrl Pts',(-49.8585818116998,-3.54939550234135,
9.38216610144959));
#24965=CARTESIAN_POINT('Ctrl Pts',(-52.0000000000001,-3.76368121662706,
9.87093082886952));
#24966=CARTESIAN_POINT('Ctrl Pts',(-54.1414181883004,-3.97796693091276,
9.38216610144959));
#24967=CARTESIAN_POINT('Ctrl Pts',(-40.1311229851416,-1.50077089878991,
0.));
#24968=CARTESIAN_POINT('Ctrl Pts',(-40.1311229851416,-1.71505661307563,
2.7089937269807));
#24969=CARTESIAN_POINT('Ctrl Pts',(-41.30651131265,-1.92934232736134,5.14971273833323));
#24970=CARTESIAN_POINT('Ctrl Pts',(-42.4818996401584,-2.14362804164706,
7.59043174968577));
#24971=CARTESIAN_POINT('Ctrl Pts',(-44.5998762217203,-2.35791375593276,
9.27946171175751));
#24972=CARTESIAN_POINT('Ctrl Pts',(-46.7178528032822,-2.57219947021846,
10.9684916738293));
#24973=CARTESIAN_POINT('Ctrl Pts',(-49.3589264016412,-2.78648518450417,
11.5712994880388));
#24974=CARTESIAN_POINT('Ctrl Pts',(-52.0000000000001,-3.00077089878988,
12.1741073022483));
#24975=CARTESIAN_POINT('Ctrl Pts',(-54.641073598359,-3.21505661307558,11.5712994880388));
#24976=CARTESIAN_POINT('Ctrl Pts',(-37.7800000000001,-1.19058808997893,
0.));
#24977=CARTESIAN_POINT('Ctrl Pts',(-37.7800000000001,-1.40487380426465,
3.24562220582792));
#24978=CARTESIAN_POINT('Ctrl Pts',(-39.1882226984277,-1.61915951855035,
6.16982677025167));
#24979=CARTESIAN_POINT('Ctrl Pts',(-40.5964453968553,-1.83344523283606,
9.09403133467541));
#24980=CARTESIAN_POINT('Ctrl Pts',(-43.1339750175689,-2.04773094712177,
11.1176436806954));
#24981=CARTESIAN_POINT('Ctrl Pts',(-45.6715046382825,-2.26201666140747,
13.1412560267153));
#24982=CARTESIAN_POINT('Ctrl Pts',(-48.8357523191413,-2.47630237569317,
13.8634749112255));
#24983=CARTESIAN_POINT('Ctrl Pts',(-52.0000000000001,-2.69058808997887,
14.5856937957357));
#24984=CARTESIAN_POINT('Ctrl Pts',(-55.1642476808589,-2.90487380426458,
13.8634749112255));
#24985=CARTESIAN_POINT('',(-37.7800000000001,-1.19058808997893,0.));
#24986=CARTESIAN_POINT('Ctrl Pts',(-37.7800000000001,-1.19058808997893,
0.));
#24987=CARTESIAN_POINT('Ctrl Pts',(-37.7800000000001,-1.40487380426465,
3.24562220582792));
#24988=CARTESIAN_POINT('Ctrl Pts',(-39.1882226984277,-1.61915951855035,
6.16982677025167));
#24989=CARTESIAN_POINT('Ctrl Pts',(-40.3638605623321,-1.79805338220513,
8.61106394926977));
#24990=CARTESIAN_POINT('Ctrl Pts',(-42.3548619717231,-1.97942721139887,
10.4489096280657));
#24991=CARTESIAN_POINT('Origin',(-35.425667181256,-19.03595491105,0.));
#24992=CARTESIAN_POINT('Ctrl Pts',(-37.7800000000001,-1.19058808997893,
0.));
#24993=CARTESIAN_POINT('Ctrl Pts',(-37.7800000000001,-1.40487380426465,
3.24562220582792));
#24994=CARTESIAN_POINT('Ctrl Pts',(-39.1882226984277,-1.61915951855037,
6.16982677025167));
#24995=CARTESIAN_POINT('Ctrl Pts',(-40.5964453968553,-1.83344523283606,
9.09403133467541));
#24996=CARTESIAN_POINT('Ctrl Pts',(-43.1339750175689,-2.04773094712178,
11.1176436806954));
#24997=CARTESIAN_POINT('Ctrl Pts',(-45.6715046382825,-2.26201666140747,
13.1412560267153));
#24998=CARTESIAN_POINT('Ctrl Pts',(-48.8357523191413,-2.47630237569318,
13.8634749112255));
#24999=CARTESIAN_POINT('Ctrl Pts',(-52.0000000000001,-2.69058808997887,
14.5856937957357));
#25000=CARTESIAN_POINT('Ctrl Pts',(-55.1642476808589,-2.90487380426458,
13.8634749112255));
#25001=CARTESIAN_POINT('Ctrl Pts',(-37.1500000000001,-0.476235235991505,
0.));
#25002=CARTESIAN_POINT('Ctrl Pts',(-37.15,-0.690520950277214,3.38941559469372));
#25003=CARTESIAN_POINT('Ctrl Pts',(-38.6206123116491,-0.904806664562923,
6.44317352589573));
#25004=CARTESIAN_POINT('Ctrl Pts',(-40.0912246232982,-1.11909237884862,
9.49693145709775));
#25005=CARTESIAN_POINT('Ctrl Pts',(-42.7411764423979,-1.33337809313434,
11.6101975146502));
#25006=CARTESIAN_POINT('Ctrl Pts',(-45.3911282614975,-1.54766380742003,
13.7234635722027));
#25007=CARTESIAN_POINT('Ctrl Pts',(-48.6955641307488,-1.76194952170574,
14.4776794959001));
#25008=CARTESIAN_POINT('Ctrl Pts',(-52.0000000000001,-1.97623523599144,
15.2318954195974));
#25009=CARTESIAN_POINT('Ctrl Pts',(-55.3044358692513,-2.19052095027714,
14.4776794959001));
#25010=CARTESIAN_POINT('Ctrl Pts',(-37.1500000000001,0.476235235991757,
0.));
#25011=CARTESIAN_POINT('Ctrl Pts',(-37.15,0.261949521706039,3.38941559469373));
#25012=CARTESIAN_POINT('Ctrl Pts',(-38.6206123116491,0.0476638074203333,
6.44317352589573));
#25013=CARTESIAN_POINT('Ctrl Pts',(-40.0912246232982,-0.166621906865366,
9.49693145709774));
#25014=CARTESIAN_POINT('Ctrl Pts',(-42.7411764423979,-0.380907621151074,
11.6101975146502));
#25015=CARTESIAN_POINT('Ctrl Pts',(-45.3911282614975,-0.595193335436777,
13.7234635722027));
#25016=CARTESIAN_POINT('Ctrl Pts',(-48.6955641307488,-0.809479049722483,
14.4776794959001));
#25017=CARTESIAN_POINT('Ctrl Pts',(-52.0000000000001,-1.02376476400818,
15.2318954195974));
#25018=CARTESIAN_POINT('Ctrl Pts',(-55.3044358692513,-1.23805047829389,
14.4776794959001));
#25019=CARTESIAN_POINT('Ctrl Pts',(-37.7800000000001,1.1905880899792,0.));
#25020=CARTESIAN_POINT('Ctrl Pts',(-37.78,0.976302375693499,3.24562220582793));
#25021=CARTESIAN_POINT('Ctrl Pts',(-39.1882226984276,0.762016661407785,
6.16982677025167));
#25022=CARTESIAN_POINT('Ctrl Pts',(-40.5964453968553,0.547730947122086,
9.09403133467541));
#25023=CARTESIAN_POINT('Ctrl Pts',(-43.1339750175689,0.333445232836365,
11.1176436806954));
#25024=CARTESIAN_POINT('Ctrl Pts',(-45.6715046382825,0.119159518550669,
13.1412560267153));
#25025=CARTESIAN_POINT('Ctrl Pts',(-48.8357523191413,-0.0951261957350281,
13.8634749112255));
#25026=CARTESIAN_POINT('Ctrl Pts',(-52.0000000000001,-0.309411910020738,
14.5856937957357));
#25027=CARTESIAN_POINT('Ctrl Pts',(-55.1642476808589,-0.52369762430644,
13.8634749112255));
#25028=CARTESIAN_POINT('',(-37.3300000000069,4.97394955414463E-6,-1.27795074269892E-29));
#25029=CARTESIAN_POINT('Origin',(-39.1300000000001,1.37043154602168E-13,
0.));
#25030=CARTESIAN_POINT('Origin',(-39.1300000000001,1.37043154602168E-13,
0.));
#25031=CARTESIAN_POINT('Ctrl Pts',(-37.2260157227862,6.5551242098742,0.));
#25032=CARTESIAN_POINT('Ctrl Pts',(-37.256511759559,6.34301961518543,3.24562220582793));
#25033=CARTESIAN_POINT('Ctrl Pts',(-38.680896818179,6.33132600607616,6.16982677025168));
#25034=CARTESIAN_POINT('Ctrl Pts',(-40.1052818767989,6.31963239696691,9.09403133467542));
#25035=CARTESIAN_POINT('Ctrl Pts',(-42.647479141562,6.46865591986365,11.1176436806954));
#25036=CARTESIAN_POINT('Ctrl Pts',(-45.1896764063252,6.61767944276043,13.1412560267153));
#25037=CARTESIAN_POINT('Ctrl Pts',(-48.3522126450341,6.85589424502971,13.8634749112255));
#25038=CARTESIAN_POINT('Ctrl Pts',(-51.514748883743,7.09410904729899,14.5856937957357));
#25039=CARTESIAN_POINT('Ctrl Pts',(-54.6772851224519,7.33232384956826,13.8634749112255));
#25040=CARTESIAN_POINT('Ctrl Pts',(-39.5090640497073,7.19674949232921,0.));
#25041=CARTESIAN_POINT('Ctrl Pts',(-39.5395600864801,6.98464489764044,2.70899372698069));
#25042=CARTESIAN_POINT('Ctrl Pts',(-40.7334806923574,6.93981550268934,5.14971273833323));
#25043=CARTESIAN_POINT('Ctrl Pts',(-41.9274012982346,6.89498610773823,7.59043174968578));
#25044=CARTESIAN_POINT('Ctrl Pts',(-44.0543159688391,6.98430100772104,9.27946171175752));
#25045=CARTESIAN_POINT('Ctrl Pts',(-46.1812306394436,7.07361590770388,10.9684916738293));
#25046=CARTESIAN_POINT('Ctrl Pts',(-48.8259179534578,7.2373752750334,11.5712994880388));
#25047=CARTESIAN_POINT('Ctrl Pts',(-51.4706052674719,7.40113464236295,12.1741073022483));
#25048=CARTESIAN_POINT('Ctrl Pts',(-54.1152925814861,7.56489400969249,11.5712994880388));
#25049=CARTESIAN_POINT('Ctrl Pts',(-41.6230663715377,8.27145263712713,-1.05434036998093E-14));
#25050=CARTESIAN_POINT('Ctrl Pts',(-41.6535624083105,8.05934804243833,2.19648874705823));
#25051=CARTESIAN_POINT('Ctrl Pts',(-42.6273788184889,7.98287244172854,4.17545672685567));
#25052=CARTESIAN_POINT('Ctrl Pts',(-43.6011952286674,7.90639684101872,6.15442470665313));
#25053=CARTESIAN_POINT('Ctrl Pts',(-45.3314958432333,7.93868724864988,7.5239130403414));
#25054=CARTESIAN_POINT('Ctrl Pts',(-47.0617964577992,7.97097765628105,8.89340137402968));
#25055=CARTESIAN_POINT('Ctrl Pts',(-49.2119141333855,8.06362864473573,9.3821661014496));
#25056=CARTESIAN_POINT('Ctrl Pts',(-51.3620318089719,8.1562796331904,9.87093082886953));
#25057=CARTESIAN_POINT('Ctrl Pts',(-53.5121494845583,8.24893062164507,9.3821661014496));
#25058=CARTESIAN_POINT('Ctrl Pts',(-43.486780470727,9.73793223897145,0.));
#25059=CARTESIAN_POINT('Ctrl Pts',(-43.5172765074999,9.52582764428269,1.72780310113343));
#25060=CARTESIAN_POINT('Ctrl Pts',(-44.2898076986597,9.42041159817596,3.28449990511991));
#25061=CARTESIAN_POINT('Ctrl Pts',(-45.0623388898194,9.31499555206925,4.84119670910638));
#25062=CARTESIAN_POINT('Ctrl Pts',(-46.4299360725759,9.29513707904871,5.91846432228298));
#25063=CARTESIAN_POINT('Ctrl Pts',(-47.7975332553324,9.27527860602821,6.99573193545956));
#25064=CARTESIAN_POINT('Ctrl Pts',(-49.495367149254,9.30290100395352,7.38020429521639));
#25065=CARTESIAN_POINT('Ctrl Pts',(-51.1932010431756,9.33052340187885,7.76467665497322));
#25066=CARTESIAN_POINT('Ctrl Pts',(-52.8910349370973,9.35814579980418,7.38020429521639));
#25067=CARTESIAN_POINT('',(-37.2260157226851,6.55512420967627,-1.21941363803477E-9));
#25068=CARTESIAN_POINT('Origin',(-32.3559861244011,23.8837944332599,1.04083408558608E-14));
#25069=CARTESIAN_POINT('Ctrl Pts',(-37.2260157227862,6.5551242098742,0.));
#25070=CARTESIAN_POINT('Ctrl Pts',(-37.256511759559,6.34301961518543,3.24562220582793));
#25071=CARTESIAN_POINT('Ctrl Pts',(-38.680896818179,6.33132600607616,6.16982677025168));
#25072=CARTESIAN_POINT('Ctrl Pts',(-39.8771654641449,6.32150513786997,8.6257176219852));
#25073=CARTESIAN_POINT('Ctrl Pts',(-41.8897230480067,6.4265912346088,10.4701702229062));
#25074=CARTESIAN_POINT('Ctrl Pts',(-44.4687528548127,2.90816428999302,0.));
#25075=CARTESIAN_POINT('Ctrl Pts',(-44.4992488915856,2.69605969530425,1.72780310113343));
#25076=CARTESIAN_POINT('Ctrl Pts',(-45.2717800827454,2.59064364919753,3.28449990511991));
#25077=CARTESIAN_POINT('Ctrl Pts',(-46.0443112739052,2.48522760309082,4.84119670910639));
#25078=CARTESIAN_POINT('Ctrl Pts',(-47.4119084566616,2.46536913007028,5.91846432228298));
#25079=CARTESIAN_POINT('Ctrl Pts',(-48.7795056394181,2.44551065704976,6.99573193545956));
#25080=CARTESIAN_POINT('Ctrl Pts',(-50.4773395333397,2.47313305497509,7.38020429521639));
#25081=CARTESIAN_POINT('Ctrl Pts',(-52.1751734272613,2.50075545290041,7.76467665497322));
#25082=CARTESIAN_POINT('Ctrl Pts',(-53.873007321183,2.52837785082574,7.38020429521639));
#25083=CARTESIAN_POINT('Ctrl Pts',(-42.2673772240309,3.79017222552557,0.));
#25084=CARTESIAN_POINT('Ctrl Pts',(-42.2978732608037,3.57806763083681,2.19648874705823));
#25085=CARTESIAN_POINT('Ctrl Pts',(-43.2716896709821,3.501592030127,4.17545672685568));
#25086=CARTESIAN_POINT('Ctrl Pts',(-44.2455060811606,3.42511642941718,6.15442470665314));
#25087=CARTESIAN_POINT('Ctrl Pts',(-45.9758066957265,3.45740683704835,7.52391304034141));
#25088=CARTESIAN_POINT('Ctrl Pts',(-47.7061073102924,3.48969724467951,8.89340137402968));
#25089=CARTESIAN_POINT('Ctrl Pts',(-49.8562249858787,3.5823482331342,9.38216610144962));
#25090=CARTESIAN_POINT('Ctrl Pts',(-52.0063426614651,3.67499922158886,9.87093082886955));
#25091=CARTESIAN_POINT('Ctrl Pts',(-54.1564603370514,3.76765021004354,9.38216610144961));
#25092=CARTESIAN_POINT('Ctrl Pts',(-39.9362279852004,4.22575906238256,0.));
#25093=CARTESIAN_POINT('Ctrl Pts',(-39.9667240219733,4.0136544676938,2.70899372698069));
#25094=CARTESIAN_POINT('Ctrl Pts',(-41.1606446278505,3.9688250727427,5.14971273833323));
#25095=CARTESIAN_POINT('Ctrl Pts',(-42.3545652337277,3.92399567779159,7.59043174968578));
#25096=CARTESIAN_POINT('Ctrl Pts',(-44.4814799043322,4.01331057777441,9.27946171175751));
#25097=CARTESIAN_POINT('Ctrl Pts',(-46.6083945749367,4.10262547775725,10.9684916738293));
#25098=CARTESIAN_POINT('Ctrl Pts',(-49.2530818889509,4.26638484508678,11.5712994880388));
#25099=CARTESIAN_POINT('Ctrl Pts',(-51.8977692029651,4.43014421241632,12.1741073022483));
#25100=CARTESIAN_POINT('Ctrl Pts',(-54.5424565169792,4.59390357974585,11.5712994880388));
#25101=CARTESIAN_POINT('Ctrl Pts',(-37.5648924257371,4.19818497005551,0.));
#25102=CARTESIAN_POINT('Ctrl Pts',(-37.59538846251,3.98608037536675,3.24562220582792));
#25103=CARTESIAN_POINT('Ctrl Pts',(-39.0197735211299,3.97438676625746,6.16982677025168));
#25104=CARTESIAN_POINT('Ctrl Pts',(-40.4441585797498,3.96269315714822,9.09403133467541));
#25105=CARTESIAN_POINT('Ctrl Pts',(-42.986355844513,4.11171668004496,11.1176436806954));
#25106=CARTESIAN_POINT('Ctrl Pts',(-45.5285531092762,4.26074020294174,13.1412560267153));
#25107=CARTESIAN_POINT('Ctrl Pts',(-48.691089347985,4.49895500521102,13.8634749112255));
#25108=CARTESIAN_POINT('Ctrl Pts',(-51.8536255866939,4.73716980748029,14.5856937957357));
#25109=CARTESIAN_POINT('Ctrl Pts',(-55.0161618254028,4.97538460974957,13.8634749112255));
#25110=CARTESIAN_POINT('',(-37.5648924257371,4.19818497005551,0.));
#25111=CARTESIAN_POINT('Ctrl Pts',(-37.5648924257371,4.19818497005551,0.));
#25112=CARTESIAN_POINT('Ctrl Pts',(-37.59538846251,3.98608037536675,3.24562220582792));
#25113=CARTESIAN_POINT('Ctrl Pts',(-39.0197735211299,3.97438676625746,6.16982677025168));
#25114=CARTESIAN_POINT('Ctrl Pts',(-40.2089043379837,3.96462449666056,8.61106394926976));
#25115=CARTESIAN_POINT('Ctrl Pts',(-42.2054524109828,4.06844583510791,10.4489096280657));
#25116=CARTESIAN_POINT('Origin',(-37.7741838134885,-13.8005982420123,1.04083408558608E-14));
#25117=CARTESIAN_POINT('Ctrl Pts',(-37.5648924257371,4.19818497005551,0.));
#25118=CARTESIAN_POINT('Ctrl Pts',(-37.59538846251,3.98608037536675,3.24562220582792));
#25119=CARTESIAN_POINT('Ctrl Pts',(-39.0197735211299,3.97438676625746,6.16982677025168));
#25120=CARTESIAN_POINT('Ctrl Pts',(-40.4441585797498,3.96269315714822,9.09403133467541));
#25121=CARTESIAN_POINT('Ctrl Pts',(-42.986355844513,4.11171668004496,11.1176436806954));
#25122=CARTESIAN_POINT('Ctrl Pts',(-45.5285531092762,4.26074020294174,13.1412560267153));
#25123=CARTESIAN_POINT('Ctrl Pts',(-48.691089347985,4.49895500521102,13.8634749112255));
#25124=CARTESIAN_POINT('Ctrl Pts',(-51.8536255866939,4.73716980748029,14.5856937957357));
#25125=CARTESIAN_POINT('Ctrl Pts',(-55.0161618254028,4.97538460974957,13.8634749112255));
#25126=CARTESIAN_POINT('Ctrl Pts',(-36.8396419064669,4.81560839388895,0.));
#25127=CARTESIAN_POINT('Ctrl Pts',(-36.8701379432397,4.60350379920018,3.38941559469373));
#25128=CARTESIAN_POINT('Ctrl Pts',(-38.3562775787769,4.60068915780645,6.44317352589574));
#25129=CARTESIAN_POINT('Ctrl Pts',(-39.8424172143141,4.59787451641272,9.49693145709774));
#25130=CARTESIAN_POINT('Ctrl Pts',(-42.4958923815832,4.76289738629114,11.6101975146502));
#25131=CARTESIAN_POINT('Ctrl Pts',(-45.1493675488523,4.92792025616953,13.7234635722027));
#25132=CARTESIAN_POINT('Ctrl Pts',(-48.4506650623305,5.18608591779772,14.4776794959001));
#25133=CARTESIAN_POINT('Ctrl Pts',(-51.7519625758087,5.44425157942588,15.2318954195974));
#25134=CARTESIAN_POINT('Ctrl Pts',(-55.0532600892869,5.70241724105408,14.4776794959001));
#25135=CARTESIAN_POINT('Ctrl Pts',(-36.7040912252865,5.75838408981643,6.24500451351651E-15));
#25136=CARTESIAN_POINT('Ctrl Pts',(-36.7345872620593,5.54627949512765,3.38941559469373));
#25137=CARTESIAN_POINT('Ctrl Pts',(-38.2207268975965,5.54346485373394,6.44317352589574));
#25138=CARTESIAN_POINT('Ctrl Pts',(-39.7068665331337,5.54065021234019,9.49693145709775));
#25139=CARTESIAN_POINT('Ctrl Pts',(-42.3603417004028,5.70567308221862,11.6101975146502));
#25140=CARTESIAN_POINT('Ctrl Pts',(-45.0138168676718,5.87069595209702,13.7234635722027));
#25141=CARTESIAN_POINT('Ctrl Pts',(-48.3151143811501,6.12886161372521,14.4776794959001));
#25142=CARTESIAN_POINT('Ctrl Pts',(-51.6164118946283,6.38702727535337,15.2318954195974));
#25143=CARTESIAN_POINT('Ctrl Pts',(-54.9177094081065,6.64519293698155,14.4776794959001));
#25144=CARTESIAN_POINT('Ctrl Pts',(-37.2260157227862,6.5551242098742,0.));
#25145=CARTESIAN_POINT('Ctrl Pts',(-37.2565117595591,6.34301961518544,3.24562220582793));
#25146=CARTESIAN_POINT('Ctrl Pts',(-38.680896818179,6.33132600607617,6.16982677025167));
#25147=CARTESIAN_POINT('Ctrl Pts',(-40.1052818767989,6.31963239696691,9.09403133467541));
#25148=CARTESIAN_POINT('Ctrl Pts',(-42.647479141562,6.46865591986366,11.1176436806954));
#25149=CARTESIAN_POINT('Ctrl Pts',(-45.1896764063252,6.61767944276043,13.1412560267153));
#25150=CARTESIAN_POINT('Ctrl Pts',(-48.3522126450341,6.85589424502971,13.8634749112255));
#25151=CARTESIAN_POINT('Ctrl Pts',(-51.514748883743,7.09410904729899,14.5856937957357));
#25152=CARTESIAN_POINT('Ctrl Pts',(-54.6772851224519,7.33232384956826,13.8634749112255));
#25153=CARTESIAN_POINT('',(-36.9500337175364,5.31261783619598,-1.46702345113165E-29));
#25154=CARTESIAN_POINT('Origin',(-38.7317130208009,5.56877962163379,0.));
#25155=CARTESIAN_POINT('Origin',(-38.7317130208009,5.56877962163379,0.));
#25156=CARTESIAN_POINT('Ctrl Pts',(-35.914217116421,11.7862169042734,0.));
#25157=CARTESIAN_POINT('Ctrl Pts',(-35.9745883786013,11.5806112670703,3.24562220582793));
#25158=CARTESIAN_POINT('Ctrl Pts',(-37.3861394252073,11.7717478112973,6.16982677025167));
#25159=CARTESIAN_POINT('Ctrl Pts',(-38.7976904718133,11.9628843555244,9.09403133467541));
#25160=CARTESIAN_POINT('Ctrl Pts',(-41.292803575407,12.4721834264258,11.1176436806954));
#25161=CARTESIAN_POINT('Ctrl Pts',(-43.7879166790007,12.9814824973272,13.1412560267153));
#25162=CARTESIAN_POINT('Ctrl Pts',(-46.884361357741,13.667348449732,13.8634749112255));
#25163=CARTESIAN_POINT('Ctrl Pts',(-49.9808060364813,14.3532144021369,14.5856937957357));
#25164=CARTESIAN_POINT('Ctrl Pts',(-53.0772507152215,15.0390803545417,13.8634749112255));
#25165=CARTESIAN_POINT('Ctrl Pts',(-38.0827145049532,12.7462230199162,0.));
#25166=CARTESIAN_POINT('Ctrl Pts',(-38.1430857671335,12.540617382713,2.7089937269807));
#25167=CARTESIAN_POINT('Ctrl Pts',(-39.3312338708267,12.6661569043005,5.14971273833323));
#25168=CARTESIAN_POINT('Ctrl Pts',(-40.5193819745197,12.7916964258879,7.59043174968578));
#25169=CARTESIAN_POINT('Ctrl Pts',(-42.6119368849888,13.1827937463385,9.27946171175751));
#25170=CARTESIAN_POINT('Ctrl Pts',(-44.7044917954577,13.5738910667891,10.9684916738293));
#25171=CARTESIAN_POINT('Ctrl Pts',(-47.2989546180622,14.1123618472581,11.5712994880388));
#25172=CARTESIAN_POINT('Ctrl Pts',(-49.8934174406667,14.650832627727,12.1741073022483));
#25173=CARTESIAN_POINT('Ctrl Pts',(-52.4878802632712,15.189303408196,11.5712994880388));
#25174=CARTESIAN_POINT('Ctrl Pts',(-40.0222531270433,14.1108411348346,0.));
#25175=CARTESIAN_POINT('Ctrl Pts',(-40.0826243892236,13.9052354976315,2.19648874705823));
#25176=CARTESIAN_POINT('Ctrl Pts',(-41.0574123652206,13.9681268331906,4.17545672685568));
#25177=CARTESIAN_POINT('Ctrl Pts',(-42.0322003412176,14.0310181687497,6.15442470665314));
#25178=CARTESIAN_POINT('Ctrl Pts',(-43.7402935862749,14.3092273587163,7.5239130403414));
#25179=CARTESIAN_POINT('Ctrl Pts',(-45.4483868313321,14.5874365486828,8.89340137402967));
#25180=CARTESIAN_POINT('Ctrl Pts',(-47.5634337987569,14.9851381329363,9.3821661014496));
#25181=CARTESIAN_POINT('Ctrl Pts',(-49.6784807661817,15.3828397171898,9.87093082886953));
#25182=CARTESIAN_POINT('Ctrl Pts',(-51.7935277336065,15.7805413014433,9.3821661014496));
#25183=CARTESIAN_POINT('Ctrl Pts',(-41.6582954965892,15.8276282594349,0.));
#25184=CARTESIAN_POINT('Ctrl Pts',(-41.7186667587695,15.6220226222318,1.72780310113342));
#25185=CARTESIAN_POINT('Ctrl Pts',(-42.4983369638544,15.6276222110081,3.28449990511991));
#25186=CARTESIAN_POINT('Ctrl Pts',(-43.2780071689392,15.6332217997843,4.84119670910639));
#25187=CARTESIAN_POINT('Ctrl Pts',(-44.6345103396638,15.8081948292726,5.91846432228298));
#25188=CARTESIAN_POINT('Ctrl Pts',(-45.9910135103883,15.9831678587608,6.99573193545956));
#25189=CARTESIAN_POINT('Ctrl Pts',(-47.6676348262507,16.2521360565318,7.38020429521639));
#25190=CARTESIAN_POINT('Ctrl Pts',(-49.3442561421131,16.5211042543028,7.76467665497322));
#25191=CARTESIAN_POINT('Ctrl Pts',(-51.0208774579755,16.7900724520738,7.38020429521639));
#25192=CARTESIAN_POINT('',(-35.9142171164436,11.7862169042832,1.57948959448622E-9));
#25193=CARTESIAN_POINT('Origin',(-28.6276304970124,28.2454287759839,0.));
#25194=CARTESIAN_POINT('Ctrl Pts',(-35.9142171165574,11.7862169041097,3.13105427371818E-9));
#25195=CARTESIAN_POINT('Ctrl Pts',(-35.9187750292273,11.770694079279,0.245038153335573));
#25196=CARTESIAN_POINT('Ctrl Pts',(-35.9294543009582,11.7568199184778,0.490791160521916));
#25197=CARTESIAN_POINT('Ctrl Pts',(-35.9463285033518,11.7446485667474,0.736766500725672));
#25198=CARTESIAN_POINT('Ctrl Pts',(-35.9631473086865,11.7325171728811,0.981934317701321));
#25199=CARTESIAN_POINT('Ctrl Pts',(-35.9861205266374,11.722077480961,1.22732257376597));
#25200=CARTESIAN_POINT('Ctrl Pts',(-36.0152719968249,11.7133702409768,1.47243294816374));
#25201=CARTESIAN_POINT('Ctrl Pts',(-36.0443795639103,11.7046761143911,1.7171741780305));
#25202=CARTESIAN_POINT('Ctrl Pts',(-36.0796468265871,11.6977092667637,1.96163791541619));
#25203=CARTESIAN_POINT('Ctrl Pts',(-36.1210475853283,11.6924966907342,2.20532408778557));
#25204=CARTESIAN_POINT('Ctrl Pts',(-36.1624128366599,11.6872885852767,2.44880126242097));
#25205=CARTESIAN_POINT('Ctrl Pts',(-36.2099010442177,11.6838317679613,2.69150175431078));
#25206=CARTESIAN_POINT('Ctrl Pts',(-36.2634360706164,11.6821391062286,2.93292951866834));
#25207=CARTESIAN_POINT('Ctrl Pts',(-36.3169598973807,11.6804467986041,3.17430677585616));
#25208=CARTESIAN_POINT('Ctrl Pts',(-36.3765279276399,11.6805179152421,3.41441139318369));
#25209=CARTESIAN_POINT('Ctrl Pts',(-36.442014877408,11.6823510237342,3.65275710614662));
#25210=CARTESIAN_POINT('Ctrl Pts',(-36.5075849814587,11.6841864598782,3.89140546668812));
#25211=CARTESIAN_POINT('Ctrl Pts',(-36.5790889062839,11.687788356271,4.12829002081188));
#25212=CARTESIAN_POINT('Ctrl Pts',(-36.6563532415795,11.6931409581035,4.36293874377831));
#25213=CARTESIAN_POINT('Ctrl Pts',(-36.7336964173083,11.6984990217245,4.59782690201468));
#25214=CARTESIAN_POINT('Ctrl Pts',(-36.8168115609901,11.705611336513,4.83047425894976));
#25215=CARTESIAN_POINT('Ctrl Pts',(-36.9054796074171,11.7144480496047,5.06042975959445));
#25216=CARTESIAN_POINT('Ctrl Pts',(-36.994406884455,11.7233105977817,5.29105755998327));
#25217=CARTESIAN_POINT('Ctrl Pts',(-37.0889193314433,11.7339075987037,5.51897736305718));
#25218=CARTESIAN_POINT('Ctrl Pts',(-37.1887539873583,11.746195348841,5.74376259354369));
#25219=CARTESIAN_POINT('Ctrl Pts',(-37.2524115326579,11.7540303837176,5.88709234072645));
#25220=CARTESIAN_POINT('Ctrl Pts',(-37.318232100817,11.7625525566675,6.02914825314205));
#25221=CARTESIAN_POINT('Ctrl Pts',(-37.3861394252394,11.7717478113121,6.16982677023484));
#25222=CARTESIAN_POINT('Ctrl Pts',(-37.4926201075706,11.7861662410925,6.39041482339092));
#25223=CARTESIAN_POINT('Ctrl Pts',(-37.6049078439222,11.8021412942475,6.60890054011809));
#25224=CARTESIAN_POINT('Ctrl Pts',(-37.7228633758096,11.8196645413939,6.82480412008048));
#25225=CARTESIAN_POINT('Ctrl Pts',(-37.8405526164633,11.8371482288263,7.04022028559302));
#25226=CARTESIAN_POINT('Ctrl Pts',(-37.9638839981999,11.856173128831,7.2530655202965));
#25227=CARTESIAN_POINT('Ctrl Pts',(-38.0926705666684,11.8767181155648,7.46287566269434));
#25228=CARTESIAN_POINT('Ctrl Pts',(-38.221249993568,11.8972300575421,7.67234834441899));
#25229=CARTESIAN_POINT('Ctrl Pts',(-38.3552669199728,11.919257185456,7.87879526533047));
#25230=CARTESIAN_POINT('Ctrl Pts',(-38.4944885898569,11.9427658506831,8.08177334612215));
#25231=CARTESIAN_POINT('Ctrl Pts',(-38.6335766715388,11.9662519584999,8.28455666214102));
#25232=CARTESIAN_POINT('Ctrl Pts',(-38.7778593027057,11.9912167312943,8.48387739272819));
#25233=CARTESIAN_POINT('Ctrl Pts',(-38.9270604659003,12.0176143452909,8.67931873611034));
#25234=CARTESIAN_POINT('Ctrl Pts',(-39.0762688052762,12.044013228943,8.87476947970419));
#25235=CARTESIAN_POINT('Ctrl Pts',(-39.2303958882198,12.0718450467039,9.06634009532744));
#25236=CARTESIAN_POINT('Ctrl Pts',(-39.3891252359321,12.1010522527167,9.25364450340887));
#25237=CARTESIAN_POINT('Ctrl Pts',(-39.5479128119392,12.1302701731048,9.44101762226405));
#25238=CARTESIAN_POINT('Ctrl Pts',(-39.7113057183253,12.1608644313193,9.62412107874949));
#25239=CARTESIAN_POINT('Ctrl Pts',(-39.8789509826186,12.1927664798387,9.80260437466047));
#25240=CARTESIAN_POINT('Ctrl Pts',(-40.0468697110622,12.224720567207,9.98137881379611));
#25241=CARTESIAN_POINT('Ctrl Pts',(-40.2190543317695,12.2579866432889,10.1555177270919));
#25242=CARTESIAN_POINT('Ctrl Pts',(-40.3951188515065,12.2924858372374,10.3247095747703));
#25243=CARTESIAN_POINT('Ctrl Pts',(-40.4460074573697,12.3024572720618,10.3736117457735));
#25244=CARTESIAN_POINT('Ctrl Pts',(-40.4972200117263,12.3125316625312,10.4221009095722));
#25245=CARTESIAN_POINT('Ctrl Pts',(-40.548746775169,12.3227069631096,10.4701702229062));
#25246=CARTESIAN_POINT('Ctrl Pts',(-43.6022501387951,9.2071267414949,0.));
#25247=CARTESIAN_POINT('Ctrl Pts',(-43.6626214009754,9.0015211042918,1.72780310113343));
#25248=CARTESIAN_POINT('Ctrl Pts',(-44.4422916060602,9.00712069306803,3.28449990511991));
#25249=CARTESIAN_POINT('Ctrl Pts',(-45.2219618111451,9.01272028184427,4.84119670910639));
#25250=CARTESIAN_POINT('Ctrl Pts',(-46.5784649818697,9.18769331133252,5.91846432228298));
#25251=CARTESIAN_POINT('Ctrl Pts',(-47.9349681525942,9.36266634082079,6.99573193545957));
#25252=CARTESIAN_POINT('Ctrl Pts',(-49.6115894684566,9.6316345385918,7.3802042952164));
#25253=CARTESIAN_POINT('Ctrl Pts',(-51.288210784319,9.90060273636281,7.76467665497322));
#25254=CARTESIAN_POINT('Ctrl Pts',(-52.9648321001814,10.1695709341338,7.3802042952164));
#25255=CARTESIAN_POINT('Ctrl Pts',(-41.297758521112,9.7668686911207,0.));
#25256=CARTESIAN_POINT('Ctrl Pts',(-41.3581297832923,9.56126305391757,2.19648874705824));
#25257=CARTESIAN_POINT('Ctrl Pts',(-42.3329177592893,9.6241543894767,4.17545672685568));
#25258=CARTESIAN_POINT('Ctrl Pts',(-43.3077057352862,9.68704572503582,6.15442470665313));
#25259=CARTESIAN_POINT('Ctrl Pts',(-45.0157989803435,9.96525491500233,7.5239130403414));
#25260=CARTESIAN_POINT('Ctrl Pts',(-46.7238922254008,10.2434641049689,8.89340137402967));
#25261=CARTESIAN_POINT('Ctrl Pts',(-48.8389391928256,10.6411656892224,9.3821661014496));
#25262=CARTESIAN_POINT('Ctrl Pts',(-50.9539861602504,11.0388672734759,9.87093082886954));
#25263=CARTESIAN_POINT('Ctrl Pts',(-53.0690331276751,11.4365688577294,9.3821661014496));
#25264=CARTESIAN_POINT('Ctrl Pts',(-38.9283465500519,9.8662647551278,-1.05434036998093E-14));
#25265=CARTESIAN_POINT('Ctrl Pts',(-38.9887178122322,9.66065911792467,2.70899372698069));
#25266=CARTESIAN_POINT('Ctrl Pts',(-40.1768659159253,9.78619863951209,5.14971273833323));
#25267=CARTESIAN_POINT('Ctrl Pts',(-41.3650140196184,9.9117381610995,7.59043174968577));
#25268=CARTESIAN_POINT('Ctrl Pts',(-43.4575689300874,10.3028354815501,9.27946171175751));
#25269=CARTESIAN_POINT('Ctrl Pts',(-45.5501238405564,10.6939328020007,10.9684916738292));
#25270=CARTESIAN_POINT('Ctrl Pts',(-48.1445866631609,11.2324035824697,11.5712994880388));
#25271=CARTESIAN_POINT('Ctrl Pts',(-50.7390494857654,11.7708743629386,12.1741073022483));
#25272=CARTESIAN_POINT('Ctrl Pts',(-53.3335123083699,12.3093451434076,11.5712994880388));
#25273=CARTESIAN_POINT('Ctrl Pts',(-36.5850719698905,9.50149509066535,0.));
#25274=CARTESIAN_POINT('Ctrl Pts',(-36.6454432320708,9.29588945346225,3.24562220582793));
#25275=CARTESIAN_POINT('Ctrl Pts',(-38.0569942786769,9.4870259976893,6.16982677025167));
#25276=CARTESIAN_POINT('Ctrl Pts',(-39.4685453252829,9.67816254191635,9.0940313346754));
#25277=CARTESIAN_POINT('Ctrl Pts',(-41.9636584288765,10.1874616128177,11.1176436806954));
#25278=CARTESIAN_POINT('Ctrl Pts',(-44.4587715324702,10.6967606837192,13.1412560267153));
#25279=CARTESIAN_POINT('Ctrl Pts',(-47.5552162112105,11.382626636124,13.8634749112255));
#25280=CARTESIAN_POINT('Ctrl Pts',(-50.6516608899508,12.0684925885288,14.5856937957357));
#25281=CARTESIAN_POINT('Ctrl Pts',(-53.7481055686911,12.7543585409336,13.8634749112255));
#25282=CARTESIAN_POINT('',(-36.5850719698905,9.50149509066535,0.));
#25283=CARTESIAN_POINT('Ctrl Pts',(-36.5850719698905,9.50149509066535,0.));
#25284=CARTESIAN_POINT('Ctrl Pts',(-36.6454432320708,9.29588945346226,3.24562220582793));
#25285=CARTESIAN_POINT('Ctrl Pts',(-38.0569942786768,9.4870259976893,6.16982677025168));
#25286=CARTESIAN_POINT('Ctrl Pts',(-39.235410774219,9.64659405380718,8.61106394926975));
#25287=CARTESIAN_POINT('Ctrl Pts',(-41.1968615496291,10.0334970568409,10.4489096280657));
#25288=CARTESIAN_POINT('Origin',(-39.3537269950292,-8.28430119040609,0.));
#25289=CARTESIAN_POINT('Ctrl Pts',(-36.5850719698905,9.50149509066535,0.));
#25290=CARTESIAN_POINT('Ctrl Pts',(-36.6454432320708,9.29588945346225,3.24562220582793));
#25291=CARTESIAN_POINT('Ctrl Pts',(-38.0569942786768,9.4870259976893,6.16982677025168));
#25292=CARTESIAN_POINT('Ctrl Pts',(-39.4685453252829,9.67816254191635,9.0940313346754));
#25293=CARTESIAN_POINT('Ctrl Pts',(-41.9636584288765,10.1874616128177,11.1176436806954));
#25294=CARTESIAN_POINT('Ctrl Pts',(-44.4587715324702,10.6967606837192,13.1412560267153));
#25295=CARTESIAN_POINT('Ctrl Pts',(-47.5552162112105,11.382626636124,13.8634749112255));
#25296=CARTESIAN_POINT('Ctrl Pts',(-50.6516608899508,12.0684925885288,14.5856937957357));
#25297=CARTESIAN_POINT('Ctrl Pts',(-53.7481055686911,12.7543585409336,13.8634749112255));
#25298=CARTESIAN_POINT('Ctrl Pts',(-35.7793349404725,10.0094201239377,0.));
#25299=CARTESIAN_POINT('Ctrl Pts',(-35.8397062026528,9.80381448673455,3.38941559469372));
#25300=CARTESIAN_POINT('Ctrl Pts',(-37.3111196447714,10.0125282162148,6.44317352589574));
#25301=CARTESIAN_POINT('Ctrl Pts',(-38.78253308689,10.2212419456951,9.49693145709775));
#25302=CARTESIAN_POINT('Ctrl Pts',(-41.3855144999133,10.7622140099936,11.6101975146502));
#25303=CARTESIAN_POINT('Ctrl Pts',(-43.9884959129367,11.303186074292,13.7234635722027));
#25304=CARTESIAN_POINT('Ctrl Pts',(-47.2194501734233,12.0285476034516,14.4776794959001));
#25305=CARTESIAN_POINT('Ctrl Pts',(-50.45040443391,12.7539091326112,15.2318954195974));
#25306=CARTESIAN_POINT('Ctrl Pts',(-53.6813586943966,13.4792706617708,14.4776794959001));
#25307=CARTESIAN_POINT('Ctrl Pts',(-35.5109929990847,10.9233088493809,6.24500451351652E-15));
#25308=CARTESIAN_POINT('Ctrl Pts',(-35.571364261265,10.7177032121778,3.38941559469373));
#25309=CARTESIAN_POINT('Ctrl Pts',(-37.0427777033836,10.9264169416581,6.44317352589575));
#25310=CARTESIAN_POINT('Ctrl Pts',(-38.5141911455021,11.1351306711383,9.49693145709774));
#25311=CARTESIAN_POINT('Ctrl Pts',(-41.1171725585255,11.6761027354368,11.6101975146502));
#25312=CARTESIAN_POINT('Ctrl Pts',(-43.7201539715489,12.2170747997352,13.7234635722027));
#25313=CARTESIAN_POINT('Ctrl Pts',(-46.9511082320355,12.9424363288948,14.4776794959001));
#25314=CARTESIAN_POINT('Ctrl Pts',(-50.1820624925221,13.6677978580544,15.2318954195974));
#25315=CARTESIAN_POINT('Ctrl Pts',(-53.4130167530088,14.393159387214,14.4776794959001));
#25316=CARTESIAN_POINT('Ctrl Pts',(-35.914217116421,11.7862169042734,0.));
#25317=CARTESIAN_POINT('Ctrl Pts',(-35.9745883786013,11.5806112670703,3.24562220582793));
#25318=CARTESIAN_POINT('Ctrl Pts',(-37.3861394252073,11.7717478112973,6.16982677025167));
#25319=CARTESIAN_POINT('Ctrl Pts',(-38.7976904718133,11.9628843555244,9.09403133467541));
#25320=CARTESIAN_POINT('Ctrl Pts',(-41.292803575407,12.4721834264258,11.1176436806954));
#25321=CARTESIAN_POINT('Ctrl Pts',(-43.7879166790007,12.9814824973272,13.1412560267153));
#25322=CARTESIAN_POINT('Ctrl Pts',(-46.884361357741,13.667348449732,13.8634749112255));
#25323=CARTESIAN_POINT('Ctrl Pts',(-49.9808060364812,14.3532144021369,14.5856937957357));
#25324=CARTESIAN_POINT('Ctrl Pts',(-53.0772507152215,15.0390803545417,13.8634749112255));
#25325=CARTESIAN_POINT('',(-35.817871303676,10.5170811194858,-1.62623179275245E-29));
#25326=CARTESIAN_POINT('Origin',(-37.5449600575353,11.0241949492053,0.));
#25327=CARTESIAN_POINT('Origin',(-37.5449600575353,11.0241949492053,0.));
#25328=CARTESIAN_POINT('Ctrl Pts',(-33.8713086176151,16.7773762111444,0.));
#25329=CARTESIAN_POINT('Ctrl Pts',(-33.9603261204012,16.5824550692827,3.24562220582792));
#25330=CARTESIAN_POINT('Ctrl Pts',(-35.3303080462616,16.9725307779979,6.16982677025168));
#25331=CARTESIAN_POINT('Ctrl Pts',(-36.7002899721219,17.3626064867131,9.09403133467542));
#25332=CARTESIAN_POINT('Ctrl Pts',(-39.097525607069,18.2218132452328,11.1176436806954));
#25333=CARTESIAN_POINT('Ctrl Pts',(-41.494761242016,19.0810200037526,13.1412560267153));
#25334=CARTESIAN_POINT('Ctrl Pts',(-44.4620796765376,20.2005748533761,13.8634749112255));
#25335=CARTESIAN_POINT('Ctrl Pts',(-47.4293981110592,21.3201297029996,14.5856937957357));
#25336=CARTESIAN_POINT('Ctrl Pts',(-50.3967165455808,22.439684552623,13.8634749112255));
#25337=CARTESIAN_POINT('Ctrl Pts',(-35.8811107143581,18.0362202038895,-1.05434036998093E-14));
#25338=CARTESIAN_POINT('Ctrl Pts',(-35.9701282171443,17.8412990620278,2.7089937269807));
#25339=CARTESIAN_POINT('Ctrl Pts',(-37.1283165495982,18.1346518775203,5.14971273833323));
#25340=CARTESIAN_POINT('Ctrl Pts',(-38.2865048820522,18.4280046930127,7.59043174968579));
#25341=CARTESIAN_POINT('Ctrl Pts',(-40.3021016488386,19.1129228203183,9.27946171175751));
#25342=CARTESIAN_POINT('Ctrl Pts',(-42.317698415625,19.7978409476239,10.9684916738293));
#25343=CARTESIAN_POINT('Ctrl Pts',(-44.8091209655645,20.7000614289634,11.5712994880388));
#25344=CARTESIAN_POINT('Ctrl Pts',(-47.300543515504,21.602281910303,12.1741073022483));
#25345=CARTESIAN_POINT('Ctrl Pts',(-49.7919660654436,22.5045023916425,11.5712994880388));
#25346=CARTESIAN_POINT('Ctrl Pts',(-37.6067022235296,19.6629735993424,0.));
#25347=CARTESIAN_POINT('Ctrl Pts',(-37.6957197263158,19.4680524574808,2.19648874705824));
#25348=CARTESIAN_POINT('Ctrl Pts',(-38.6516353959964,19.6690304430805,4.17545672685568));
#25349=CARTESIAN_POINT('Ctrl Pts',(-39.6075510656771,19.8700084286802,6.15442470665314));
#25350=CARTESIAN_POINT('Ctrl Pts',(-41.2586650884905,20.3884728641634,7.52391304034141));
#25351=CARTESIAN_POINT('Ctrl Pts',(-42.909779111304,20.9069372996466,8.89340137402968));
#25352=CARTESIAN_POINT('Ctrl Pts',(-44.9466991136022,21.6015934223202,9.38216610144961));
#25353=CARTESIAN_POINT('Ctrl Pts',(-46.9836191159004,22.2962495449937,9.87093082886954));
#25354=CARTESIAN_POINT('Ctrl Pts',(-49.0205391181987,22.9909056676674,9.38216610144961));
#25355=CARTESIAN_POINT('Ctrl Pts',(-38.9817677587447,21.5951194116471,1.04083408558608E-14));
#25356=CARTESIAN_POINT('Ctrl Pts',(-39.0707852615308,21.4001982697854,1.72780310113343));
#25357=CARTESIAN_POINT('Ctrl Pts',(-39.8417226435484,21.516699501965,3.28449990511991));
#25358=CARTESIAN_POINT('Ctrl Pts',(-40.6126600255661,21.6332007341446,4.84119670910638));
#25359=CARTESIAN_POINT('Ctrl Pts',(-41.9304546915349,21.9994433198418,5.91846432228298));
#25360=CARTESIAN_POINT('Ctrl Pts',(-43.2482493575037,22.365685905539,6.99573193545957));
#25361=CARTESIAN_POINT('Ctrl Pts',(-44.8695269202925,22.8705244862893,7.38020429521639));
#25362=CARTESIAN_POINT('Ctrl Pts',(-46.4908044830812,23.3753630670397,7.76467665497322));
#25363=CARTESIAN_POINT('Ctrl Pts',(-48.11208204587,23.88020164779,7.38020429521639));
#25364=CARTESIAN_POINT('',(-33.8713086176317,16.7773762111466,1.5794947023715E-9));
#25365=CARTESIAN_POINT('Origin',(-24.3164988679736,32.0320676419193,0.));
#25366=CARTESIAN_POINT('Ctrl Pts',(-33.8713086177735,16.7773762110018,3.13106388084265E-9));
#25367=CARTESIAN_POINT('Ctrl Pts',(-33.8780292657697,16.7626600447503,0.245038153335515));
#25368=CARTESIAN_POINT('Ctrl Pts',(-33.8905743368632,16.7504469217305,0.490791160521789));
#25369=CARTESIAN_POINT('Ctrl Pts',(-33.9090089481601,16.7408009061956,0.736766500725478));
#25370=CARTESIAN_POINT('Ctrl Pts',(-33.9273830396633,16.731186557988,0.981934317701124));
#25371=CARTESIAN_POINT('Ctrl Pts',(-33.9516081464474,16.7241225568762,1.22732257376577));
#25372=CARTESIAN_POINT('Ctrl Pts',(-33.9817020661515,16.7196526308054,1.47243294816354));
#25373=CARTESIAN_POINT('Ctrl Pts',(-34.0117506633926,16.7151894365947,1.71717417803031));
#25374=CARTESIAN_POINT('Ctrl Pts',(-34.0476504419798,16.713312556215,1.96163791541602));
#25375=CARTESIAN_POINT('Ctrl Pts',(-34.0893716276067,16.7140449789782,2.20532408778542));
#25376=CARTESIAN_POINT('Ctrl Pts',(-34.1310570310094,16.7147767735782,2.44880126242085));
#25377=CARTESIAN_POINT('Ctrl Pts',(-34.1785538334838,16.7181134182572,2.6915017543107));
#25378=CARTESIAN_POINT('Ctrl Pts',(-34.2317848413855,16.7240568140042,2.9329295186683));
#25379=CARTESIAN_POINT('Ctrl Pts',(-34.2850047132543,16.7299989663809,3.17430677585617));
#25380=CARTESIAN_POINT('Ctrl Pts',(-34.3439563059026,16.7385467737467,3.41441139318376));
#25381=CARTESIAN_POINT('Ctrl Pts',(-34.4085158144079,16.7496809885027,3.65275710614674));
#25382=CARTESIAN_POINT('Ctrl Pts',(-34.4731572995457,16.7608293413068,3.89140546668823));
#25383=CARTESIAN_POINT('Ctrl Pts',(-34.5434208142137,16.7745706450852,4.12829002081196));
#25384=CARTESIAN_POINT('Ctrl Pts',(-34.6191369553178,16.7908646265308,4.36293874377837));
#25385=CARTESIAN_POINT('Ctrl Pts',(-34.6949303570796,16.8071752343352,4.59782690201464));
#25386=CARTESIAN_POINT('Ctrl Pts',(-34.7761873205119,16.8260436742454,4.83047425894961));
#25387=CARTESIAN_POINT('Ctrl Pts',(-34.8626952586805,16.8474092210266,5.0604297595942));
#25388=CARTESIAN_POINT('Ctrl Pts',(-34.9494561121503,16.8688372322916,5.29105755998298));
#25389=CARTESIAN_POINT('Ctrl Pts',(-35.0414984482315,16.8927768946317,5.51897736305686));
#25390=CARTESIAN_POINT('Ctrl Pts',(-35.1385682021254,16.9191475261007,5.74376259354333));
#25391=CARTESIAN_POINT('Ctrl Pts',(-35.2004627636792,16.9359622248837,5.88709234072621));
#25392=CARTESIAN_POINT('Ctrl Pts',(-35.2644005416947,16.9537648979136,6.02914825314193));
#25393=CARTESIAN_POINT('Ctrl Pts',(-35.3303080462913,16.9725307780171,6.16982677023484));
#25394=CARTESIAN_POINT('Ctrl Pts',(-35.4336529523065,17.0019562300572,6.39041482339095));
#25395=CARTESIAN_POINT('Ctrl Pts',(-35.5425242743014,17.0337488912442,6.60890054011814));
#25396=CARTESIAN_POINT('Ctrl Pts',(-35.6567853708684,17.067880599445,6.82480412008055));
#25397=CARTESIAN_POINT('Ctrl Pts',(-35.7707885165966,17.1019352533989,7.04022028559297));
#25398=CARTESIAN_POINT('Ctrl Pts',(-35.8901570371289,17.138318392999,7.25306552029633));
#25399=CARTESIAN_POINT('Ctrl Pts',(-36.0147088875609,17.1769825010546,7.46287566269405));
#25400=CARTESIAN_POINT('Ctrl Pts',(-36.1390604075859,17.2155844213829,7.67234834441897));
#25401=CARTESIAN_POINT('Ctrl Pts',(-36.2685784477697,17.2564599421024,7.8787952653307));
#25402=CARTESIAN_POINT('Ctrl Pts',(-36.4030374099059,17.2995426324479,8.08177334612262));
#25403=CARTESIAN_POINT('Ctrl Pts',(-36.5373673538294,17.3425839834017,8.28455666214181));
#25404=CARTESIAN_POINT('Ctrl Pts',(-36.6766285382468,17.3878282101255,8.48387739272927));
#25405=CARTESIAN_POINT('Ctrl Pts',(-36.8205542765639,17.4351906738842,8.67931873611171));
#25406=CARTESIAN_POINT('Ctrl Pts',(-36.9644869373279,17.482555415652,8.87476947970536));
#25407=CARTESIAN_POINT('Ctrl Pts',(-37.1130843481565,17.5320385165208,9.06634009532841));
#25408=CARTESIAN_POINT('Ctrl Pts',(-37.2660414411776,17.5835379767386,9.25364450340966));
#25409=CARTESIAN_POINT('Ctrl Pts',(-37.419054644999,17.6350563290252,9.44101762226471));
#25410=CARTESIAN_POINT('Ctrl Pts',(-37.5764304302811,17.6885924168517,9.62412107875002));
#25411=CARTESIAN_POINT('Ctrl Pts',(-37.7378291726328,17.7440281571912,9.80260437466088));
#25412=CARTESIAN_POINT('Ctrl Pts',(-37.8994911897636,17.7995543247056,9.98137881379651));
#25413=CARTESIAN_POINT('Ctrl Pts',(-38.0651889630643,17.8569862265478,10.1555177270923));
#25414=CARTESIAN_POINT('Ctrl Pts',(-38.2345516526471,17.9161908620977,10.3247095747707));
#25415=CARTESIAN_POINT('Ctrl Pts',(-38.2835032027434,17.9333030058065,10.3736117457738));
#25416=CARTESIAN_POINT('Ctrl Pts',(-38.3327607518886,17.9505631598978,10.4221009095723));
#25417=CARTESIAN_POINT('Ctrl Pts',(-38.3823149509186,17.967967913594,10.4701702229062));
#25418=CARTESIAN_POINT('Ctrl Pts',(-41.8481313484578,15.3186586437009,0.));
#25419=CARTESIAN_POINT('Ctrl Pts',(-41.9371488512439,15.1237375018392,1.72780310113342));
#25420=CARTESIAN_POINT('Ctrl Pts',(-42.7080862332615,15.2402387340188,3.28449990511991));
#25421=CARTESIAN_POINT('Ctrl Pts',(-43.4790236152791,15.3567399661984,4.84119670910639));
#25422=CARTESIAN_POINT('Ctrl Pts',(-44.796818281248,15.7229825518956,5.91846432228298));
#25423=CARTESIAN_POINT('Ctrl Pts',(-46.1146129472168,16.0892251375928,6.99573193545957));
#25424=CARTESIAN_POINT('Ctrl Pts',(-47.7358905100055,16.5940637183432,7.38020429521639));
#25425=CARTESIAN_POINT('Ctrl Pts',(-49.3571680727943,17.0989022990935,7.76467665497321));
#25426=CARTESIAN_POINT('Ctrl Pts',(-50.978445635583,17.6037408798438,7.38020429521639));
#25427=CARTESIAN_POINT('Ctrl Pts',(-39.4874365476043,15.5447398754881,0.));
#25428=CARTESIAN_POINT('Ctrl Pts',(-39.5764540503904,15.3498187336264,2.19648874705823));
#25429=CARTESIAN_POINT('Ctrl Pts',(-40.5323697200711,15.5507967192261,4.17545672685568));
#25430=CARTESIAN_POINT('Ctrl Pts',(-41.4882853897518,15.7517747048258,6.15442470665314));
#25431=CARTESIAN_POINT('Ctrl Pts',(-43.1393994125653,16.270239140309,7.5239130403414));
#25432=CARTESIAN_POINT('Ctrl Pts',(-44.7905134353787,16.7887035757922,8.89340137402966));
#25433=CARTESIAN_POINT('Ctrl Pts',(-46.8274334376769,17.4833596984658,9.3821661014496));
#25434=CARTESIAN_POINT('Ctrl Pts',(-48.8643534399751,18.1780158211394,9.87093082886953));
#25435=CARTESIAN_POINT('Ctrl Pts',(-50.9012734422734,18.872671943813,9.3821661014496));
#25436=CARTESIAN_POINT('Ctrl Pts',(-37.1279962392256,15.3059217494167,0.));
#25437=CARTESIAN_POINT('Ctrl Pts',(-37.2170137420117,15.111000607555,2.70899372698069));
#25438=CARTESIAN_POINT('Ctrl Pts',(-38.3752020744657,15.4043534230475,5.14971273833323));
#25439=CARTESIAN_POINT('Ctrl Pts',(-39.5333904069197,15.69770623854,7.59043174968578));
#25440=CARTESIAN_POINT('Ctrl Pts',(-41.5489871737061,16.3826243658455,9.27946171175751));
#25441=CARTESIAN_POINT('Ctrl Pts',(-43.5645839404925,17.0675424931511,10.9684916738293));
#25442=CARTESIAN_POINT('Ctrl Pts',(-46.056006490432,17.9697629744906,11.5712994880388));
#25443=CARTESIAN_POINT('Ctrl Pts',(-48.5474290403715,18.8719834558302,12.1741073022483));
#25444=CARTESIAN_POINT('Ctrl Pts',(-51.038851590311,19.7742039371697,11.5712994880388));
#25445=CARTESIAN_POINT('Ctrl Pts',(-34.8604849513722,14.6113821712785,0.));
#25446=CARTESIAN_POINT('Ctrl Pts',(-34.9495024541584,14.4164610294168,3.24562220582793));
#25447=CARTESIAN_POINT('Ctrl Pts',(-36.3194843800187,14.806536738132,6.16982677025168));
#25448=CARTESIAN_POINT('Ctrl Pts',(-37.6894663058791,15.1966124468471,9.09403133467541));
#25449=CARTESIAN_POINT('Ctrl Pts',(-40.0867019408261,16.0558192053669,11.1176436806954));
#25450=CARTESIAN_POINT('Ctrl Pts',(-42.4839375757731,16.9150259638866,13.1412560267153));
#25451=CARTESIAN_POINT('Ctrl Pts',(-45.4512560102947,18.0345808135101,13.8634749112255));
#25452=CARTESIAN_POINT('Ctrl Pts',(-48.4185744448163,19.1541356631336,14.5856937957357));
#25453=CARTESIAN_POINT('Ctrl Pts',(-51.3858928793379,20.2736905127571,13.8634749112255));
#25454=CARTESIAN_POINT('',(-34.8604849513722,14.6113821712785,0.));
#25455=CARTESIAN_POINT('Ctrl Pts',(-34.8604849513722,14.6113821712785,0.));
#25456=CARTESIAN_POINT('Ctrl Pts',(-34.9495024541584,14.4164610294168,3.24562220582793));
#25457=CARTESIAN_POINT('Ctrl Pts',(-36.3194843800187,14.806536738132,6.16982677025168));
#25458=CARTESIAN_POINT('Ctrl Pts',(-37.4631973926725,15.1321867744983,8.61106394926977));
#25459=CARTESIAN_POINT('Ctrl Pts',(-39.3496213890632,15.7942952127127,10.4489096280657));
#25460=CARTESIAN_POINT('Origin',(-40.1321417817282,-2.59935965651507,0.));
#25461=CARTESIAN_POINT('Ctrl Pts',(-34.8604849513722,14.6113821712785,0.));
#25462=CARTESIAN_POINT('Ctrl Pts',(-34.9495024541584,14.4164610294168,3.24562220582793));
#25463=CARTESIAN_POINT('Ctrl Pts',(-36.3194843800187,14.806536738132,6.16982677025168));
#25464=CARTESIAN_POINT('Ctrl Pts',(-37.6894663058791,15.1966124468471,9.09403133467541));
#25465=CARTESIAN_POINT('Ctrl Pts',(-40.0867019408261,16.0558192053669,11.1176436806954));
#25466=CARTESIAN_POINT('Ctrl Pts',(-42.4839375757731,16.9150259638866,13.1412560267153));
#25467=CARTESIAN_POINT('Ctrl Pts',(-45.4512560102947,18.0345808135101,13.8634749112255));
#25468=CARTESIAN_POINT('Ctrl Pts',(-48.4185744448163,19.1541356631336,14.5856937957357));
#25469=CARTESIAN_POINT('Ctrl Pts',(-51.3858928793379,20.2736905127571,13.8634749112255));
#25470=CARTESIAN_POINT('Ctrl Pts',(-33.9906638941717,14.9994689250471,0.));
#25471=CARTESIAN_POINT('Ctrl Pts',(-34.0796813969579,14.8045477831854,3.38941559469373));
#25472=CARTESIAN_POINT('Ctrl Pts',(-35.5064149111822,15.2205410738881,6.44317352589574));
#25473=CARTESIAN_POINT('Ctrl Pts',(-36.9331484254066,15.6365343645909,9.49693145709775));
#25474=CARTESIAN_POINT('Ctrl Pts',(-39.4326468889937,16.5424429921149,11.6101975146502));
#25475=CARTESIAN_POINT('Ctrl Pts',(-41.9321453525808,17.4483516196389,13.7234635722027));
#25476=CARTESIAN_POINT('Ctrl Pts',(-45.026983448635,18.6261427473661,14.4776794959001));
#25477=CARTESIAN_POINT('Ctrl Pts',(-48.1218215446892,19.8039338750934,15.2318954195974));
#25478=CARTESIAN_POINT('Ctrl Pts',(-51.2166596407434,20.9817250028206,14.4776794959001));
#25479=CARTESIAN_POINT('Ctrl Pts',(-33.5949933606689,15.8658665409935,0.));
#25480=CARTESIAN_POINT('Ctrl Pts',(-33.684010863455,15.6709453991318,3.38941559469373));
#25481=CARTESIAN_POINT('Ctrl Pts',(-35.1107443776794,16.0869386898345,6.44317352589574));
#25482=CARTESIAN_POINT('Ctrl Pts',(-36.5374778919038,16.5029319805373,9.49693145709774));
#25483=CARTESIAN_POINT('Ctrl Pts',(-39.0369763554909,17.4088406080613,11.6101975146502));
#25484=CARTESIAN_POINT('Ctrl Pts',(-41.536474819078,18.3147492355853,13.7234635722027));
#25485=CARTESIAN_POINT('Ctrl Pts',(-44.6313129151321,19.4925403633125,14.4776794959001));
#25486=CARTESIAN_POINT('Ctrl Pts',(-47.7261510111863,20.6703314910398,15.2318954195974));
#25487=CARTESIAN_POINT('Ctrl Pts',(-50.8209891072405,21.848122618767,14.4776794959001));
#25488=CARTESIAN_POINT('Ctrl Pts',(-33.8713086176151,16.7773762111444,0.));
#25489=CARTESIAN_POINT('Ctrl Pts',(-33.9603261204012,16.5824550692827,3.24562220582792));
#25490=CARTESIAN_POINT('Ctrl Pts',(-35.3303080462616,16.9725307779979,6.16982677025167));
#25491=CARTESIAN_POINT('Ctrl Pts',(-36.7002899721219,17.3626064867131,9.09403133467541));
#25492=CARTESIAN_POINT('Ctrl Pts',(-39.097525607069,18.2218132452328,11.1176436806954));
#25493=CARTESIAN_POINT('Ctrl Pts',(-41.494761242016,19.0810200037526,13.1412560267153));
#25494=CARTESIAN_POINT('Ctrl Pts',(-44.4620796765376,20.2005748533761,13.8634749112255));
#25495=CARTESIAN_POINT('Ctrl Pts',(-47.4293981110592,21.3201297029996,14.5856937957357));
#25496=CARTESIAN_POINT('Ctrl Pts',(-50.3967165455808,22.439684552623,13.8634749112255));
#25497=CARTESIAN_POINT('',(-33.9565603202845,15.5074469599424,-1.75233474473625E-29));
#25498=CARTESIAN_POINT('Origin',(-35.5938999782223,16.255189458764,0.));
#25499=CARTESIAN_POINT('Origin',(-35.5938999782223,16.255189458764,0.));
#25500=CARTESIAN_POINT('Ctrl Pts',(-39.2421052839111,21.1183468312849,1.04083408558608E-14));
#25501=CARTESIAN_POINT('Ctrl Pts',(-39.3579568876516,20.9380782171067,1.72780310113343));
#25502=CARTESIAN_POINT('Ctrl Pts',(-40.1044673847039,21.1631094635643,3.28449990511991));
#25503=CARTESIAN_POINT('Ctrl Pts',(-40.8509778817562,21.3881407100219,4.84119670910639));
#25504=CARTESIAN_POINT('Ctrl Pts',(-42.1032375437762,21.9381972090397,5.91846432228298));
#25505=CARTESIAN_POINT('Ctrl Pts',(-43.3554972057962,22.4882537080574,6.99573193545956));
#25506=CARTESIAN_POINT('Ctrl Pts',(-44.8884264797114,23.2186856141172,7.38020429521639));
#25507=CARTESIAN_POINT('Ctrl Pts',(-45.6451607014124,23.5792650807263,7.56999999999999));
#25508=CARTESIAN_POINT('Ctrl Pts',(-46.4213557536266,23.949117520177,7.56999999999998));
#25509=CARTESIAN_POINT('Ctrl Pts',(-36.8732642383512,21.0061649833186,-1.05434036998093E-14));
#25510=CARTESIAN_POINT('Ctrl Pts',(-36.9891158420917,20.8258963691405,2.19648874705824));
#25511=CARTESIAN_POINT('Ctrl Pts',(-37.9066995190544,21.1608696725666,4.17545672685568));
#25512=CARTESIAN_POINT('Ctrl Pts',(-38.8242831960172,21.4958429759927,6.15442470665315));
#25513=CARTESIAN_POINT('Ctrl Pts',(-40.384806076502,22.2440082162141,7.52391304034141));
#25514=CARTESIAN_POINT('Ctrl Pts',(-41.9453289569868,22.9921734564355,8.89340137402968));
#25515=CARTESIAN_POINT('Ctrl Pts',(-43.8626561769039,23.9696429220944,9.38216610144962));
#25516=CARTESIAN_POINT('Ctrl Pts',(-44.8091493688595,24.4521730739537,9.62344598428098));
#25517=CARTESIAN_POINT('Ctrl Pts',(-45.779983396821,24.9471123877533,9.62344598428098));
#25518=CARTESIAN_POINT('Ctrl Pts',(-34.5718269932683,20.4339943155209,-1.05434036998093E-14));
#25519=CARTESIAN_POINT('Ctrl Pts',(-34.6876785970088,20.2537257013428,2.70899372698069));
#25520=CARTESIAN_POINT('Ctrl Pts',(-35.7923297837143,20.7089199933766,5.14971273833323));
#25521=CARTESIAN_POINT('Ctrl Pts',(-36.8969809704197,21.1641142854104,7.59043174968577));
#25522=CARTESIAN_POINT('Ctrl Pts',(-38.7945878558529,22.1289102616397,9.27946171175752));
#25523=CARTESIAN_POINT('Ctrl Pts',(-40.692194741286,23.0937062378691,10.9684916738293));
#25524=CARTESIAN_POINT('Ctrl Pts',(-43.0298588401131,24.3413098128681,11.5712994880388));
#25525=CARTESIAN_POINT('Ctrl Pts',(-44.1838523429616,24.9571923172886,11.8688770148585));
#25526=CARTESIAN_POINT('Ctrl Pts',(-45.3675229389402,25.5889133878672,11.8688770148585));
#25527=CARTESIAN_POINT('Ctrl Pts',(-32.4262389885812,19.423823646631,1.04083408558608E-14));
#25528=CARTESIAN_POINT('Ctrl Pts',(-32.5420905923217,19.2435550324529,3.24562220582793));
#25529=CARTESIAN_POINT('Ctrl Pts',(-33.8426145161274,19.8246290891123,6.16982677025167));
#25530=CARTESIAN_POINT('Ctrl Pts',(-35.1431384399332,20.4057031457716,9.09403133467541));
#25531=CARTESIAN_POINT('Ctrl Pts',(-37.3936958017627,21.5973266200539,11.1176436806954));
#25532=CARTESIAN_POINT('Ctrl Pts',(-39.6442531635923,22.7889500943362,13.1412560267153));
#25533=CARTESIAN_POINT('Ctrl Pts',(-42.4220393076081,24.3194029329696,13.8634749112255));
#25534=CARTESIAN_POINT('Ctrl Pts',(-43.7933001162526,25.0749146564396,14.22));
#25535=CARTESIAN_POINT('Ctrl Pts',(-45.199825451624,25.849855771603,14.22));
#25536=CARTESIAN_POINT('',(-32.4262389885812,19.423823646631,6.93889390390723E-15));
#25537=CARTESIAN_POINT('Ctrl Pts',(-32.4262389885812,19.423823646631,6.93889390390723E-15));
#25538=CARTESIAN_POINT('Ctrl Pts',(-32.5420905923217,19.2435550324529,3.24562220582793));
#25539=CARTESIAN_POINT('Ctrl Pts',(-33.8426145161274,19.8246290891123,6.16982677025167));
#25540=CARTESIAN_POINT('Ctrl Pts',(-34.9283413471526,20.3097318100845,8.61106394927297));
#25541=CARTESIAN_POINT('Ctrl Pts',(-36.7013364119536,21.2335670650399,10.4489096280657));
#25542=CARTESIAN_POINT('Origin',(-40.0935818932913,3.13849734404836,0.));
#25543=CARTESIAN_POINT('Ctrl Pts',(-31.1388779521428,21.4269965203143,0.));
#25544=CARTESIAN_POINT('Ctrl Pts',(-31.2547295558833,21.2467279061362,3.24562220582793));
#25545=CARTESIAN_POINT('Ctrl Pts',(-32.555253479689,21.8278019627955,6.16982677025167));
#25546=CARTESIAN_POINT('Ctrl Pts',(-33.8557774034948,22.4088760194548,9.09403133467541));
#25547=CARTESIAN_POINT('Ctrl Pts',(-36.1063347653244,23.6004994937371,11.1176436806954));
#25548=CARTESIAN_POINT('Ctrl Pts',(-38.3568921271539,24.7921229680194,13.1412560267153));
#25549=CARTESIAN_POINT('Ctrl Pts',(-41.1346782711698,26.3225758066528,13.8634749112255));
#25550=CARTESIAN_POINT('Ctrl Pts',(-42.5059390798142,27.0780875301229,14.22));
#25551=CARTESIAN_POINT('Ctrl Pts',(-43.9124644151856,27.8530286452862,14.22));
#25552=CARTESIAN_POINT('Ctrl Pts',(-32.9490709821975,22.9590519566756,-1.05434036998093E-14));
#25553=CARTESIAN_POINT('Ctrl Pts',(-33.0649225859379,22.7787833424975,2.70899372698069));
#25554=CARTESIAN_POINT('Ctrl Pts',(-34.1695737726434,23.2339776345313,5.14971273833322));
#25555=CARTESIAN_POINT('Ctrl Pts',(-35.2742249593488,23.6891719265651,7.59043174968576));
#25556=CARTESIAN_POINT('Ctrl Pts',(-37.171831844782,24.6539679027944,9.27946171175751));
#25557=CARTESIAN_POINT('Ctrl Pts',(-39.0694387302151,25.6187638790238,10.9684916738292));
#25558=CARTESIAN_POINT('Ctrl Pts',(-41.4071028290422,26.8663674540228,11.5712994880388));
#25559=CARTESIAN_POINT('Ctrl Pts',(-42.5610963318907,27.4822499584433,11.8688770148585));
#25560=CARTESIAN_POINT('Ctrl Pts',(-43.7447669278693,28.1139710290219,11.8688770148584));
#25561=CARTESIAN_POINT('Ctrl Pts',(-34.4255873115187,24.8148246247011,0.));
#25562=CARTESIAN_POINT('Ctrl Pts',(-34.5414389152592,24.634556010523,2.19648874705822));
#25563=CARTESIAN_POINT('Ctrl Pts',(-35.459022592222,24.9695293139491,4.17545672685568));
#25564=CARTESIAN_POINT('Ctrl Pts',(-36.3766062691848,25.3045026173752,6.15442470665313));
#25565=CARTESIAN_POINT('Ctrl Pts',(-37.9371291496695,26.0526678575966,7.52391304034139));
#25566=CARTESIAN_POINT('Ctrl Pts',(-39.4976520301543,26.800833097818,8.89340137402967));
#25567=CARTESIAN_POINT('Ctrl Pts',(-41.4149792500714,27.7783025634769,9.38216610144959));
#25568=CARTESIAN_POINT('Ctrl Pts',(-42.361472442027,28.2608327153362,9.62344598428098));
#25569=CARTESIAN_POINT('Ctrl Pts',(-43.3323064699885,28.7557720291358,9.62344598428096));
#25570=CARTESIAN_POINT('Ctrl Pts',(-35.5116836434675,26.92299620782,0.));
#25571=CARTESIAN_POINT('Ctrl Pts',(-35.627535247208,26.7427275936419,1.72780310113342));
#25572=CARTESIAN_POINT('Ctrl Pts',(-36.3740457442603,26.9677588400994,3.28449990511991));
#25573=CARTESIAN_POINT('Ctrl Pts',(-37.1205562413126,27.192790086557,4.84119670910638));
#25574=CARTESIAN_POINT('Ctrl Pts',(-38.3728159033326,27.7428465855748,5.91846432228297));
#25575=CARTESIAN_POINT('Ctrl Pts',(-39.6250755653526,28.2929030845925,6.99573193545956));
#25576=CARTESIAN_POINT('Ctrl Pts',(-41.1580048392677,29.0233349906523,7.38020429521639));
#25577=CARTESIAN_POINT('Ctrl Pts',(-41.9147390609688,29.3839144572614,7.56999999999998));
#25578=CARTESIAN_POINT('Ctrl Pts',(-42.6909341131829,29.7537668967121,7.56999999999998));
#25579=CARTESIAN_POINT('',(-31.1388779521918,21.4269965202911,2.36793890025575E-9));
#25580=CARTESIAN_POINT('Origin',(-19.5103534449751,35.1666259835202,0.));
#25581=CARTESIAN_POINT('Ctrl Pts',(-31.1388779521428,21.4269965203143,0.));
#25582=CARTESIAN_POINT('Ctrl Pts',(-31.2547295558833,21.2467279061362,3.24562220582793));
#25583=CARTESIAN_POINT('Ctrl Pts',(-32.555253479689,21.8278019627955,6.16982677025167));
#25584=CARTESIAN_POINT('Ctrl Pts',(-33.6474974511926,22.3158165419706,8.62571762198518));
#25585=CARTESIAN_POINT('Ctrl Pts',(-35.4345298797236,23.2474528526982,10.4701702229061));
#25586=CARTESIAN_POINT('Ctrl Pts',(-32.4262389885812,19.423823646631,1.04083408558608E-14));
#25587=CARTESIAN_POINT('Ctrl Pts',(-32.5420905923217,19.2435550324529,3.24562220582793));
#25588=CARTESIAN_POINT('Ctrl Pts',(-33.8426145161274,19.8246290891122,6.16982677025167));
#25589=CARTESIAN_POINT('Ctrl Pts',(-35.1431384399332,20.4057031457716,9.09403133467541));
#25590=CARTESIAN_POINT('Ctrl Pts',(-37.3936958017627,21.5973266200539,11.1176436806954));
#25591=CARTESIAN_POINT('Ctrl Pts',(-39.6442531635923,22.7889500943362,13.1412560267153));
#25592=CARTESIAN_POINT('Ctrl Pts',(-42.4220393076081,24.3194029329696,13.8634749112255));
#25593=CARTESIAN_POINT('Ctrl Pts',(-43.7933001162526,25.0749146564396,14.22));
#25594=CARTESIAN_POINT('Ctrl Pts',(-45.199825451624,25.849855771603,14.22));
#25595=CARTESIAN_POINT('Ctrl Pts',(-31.510040951966,19.684171793739,0.));
#25596=CARTESIAN_POINT('Ctrl Pts',(-31.6258925557065,19.5039031795609,3.38941559469373));
#25597=CARTESIAN_POINT('Ctrl Pts',(-32.9789019620468,20.118707607713,6.44317352589574));
#25598=CARTESIAN_POINT('Ctrl Pts',(-34.3319113683871,20.7335120358651,9.49693145709775));
#25599=CARTESIAN_POINT('Ctrl Pts',(-36.6770443017776,21.985915539383,11.6101975146502));
#25600=CARTESIAN_POINT('Ctrl Pts',(-39.0221772351681,23.2383190429009,13.7234635722027));
#25601=CARTESIAN_POINT('Ctrl Pts',(-41.9178971879302,24.8445633383044,14.4776794959001));
#25602=CARTESIAN_POINT('Ctrl Pts',(-43.3473763048115,25.637489696635,14.85));
#25603=CARTESIAN_POINT('Ctrl Pts',(-44.8136171406925,26.4508076337079,14.85));
#25604=CARTESIAN_POINT('Ctrl Pts',(-30.9950965373907,20.4854409432123,0.));
#25605=CARTESIAN_POINT('Ctrl Pts',(-31.1109481411311,20.3051723290341,3.38941559469373));
#25606=CARTESIAN_POINT('Ctrl Pts',(-32.4639575474714,20.9199767571863,6.44317352589574));
#25607=CARTESIAN_POINT('Ctrl Pts',(-33.8169669538117,21.5347811853384,9.49693145709776));
#25608=CARTESIAN_POINT('Ctrl Pts',(-36.1620998872022,22.7871846888563,11.6101975146503));
#25609=CARTESIAN_POINT('Ctrl Pts',(-38.5072328205927,24.0395881923742,13.7234635722027));
#25610=CARTESIAN_POINT('Ctrl Pts',(-41.4029527733549,25.6458324877777,14.4776794959001));
#25611=CARTESIAN_POINT('Ctrl Pts',(-42.8324318902361,26.4387588461083,14.85));
#25612=CARTESIAN_POINT('Ctrl Pts',(-44.2986727261171,27.2520767831812,14.85));
#25613=CARTESIAN_POINT('Ctrl Pts',(-31.1388779521428,21.4269965203143,0.));
#25614=CARTESIAN_POINT('Ctrl Pts',(-31.2547295558833,21.2467279061362,3.24562220582793));
#25615=CARTESIAN_POINT('Ctrl Pts',(-32.555253479689,21.8278019627955,6.16982677025168));
#25616=CARTESIAN_POINT('Ctrl Pts',(-33.8557774034948,22.4088760194548,9.09403133467541));
#25617=CARTESIAN_POINT('Ctrl Pts',(-36.1063347653244,23.6004994937371,11.1176436806954));
#25618=CARTESIAN_POINT('Ctrl Pts',(-38.3568921271539,24.7921229680194,13.1412560267153));
#25619=CARTESIAN_POINT('Ctrl Pts',(-41.1346782711697,26.3225758066528,13.8634749112255));
#25620=CARTESIAN_POINT('Ctrl Pts',(-42.5059390798142,27.0780875301229,14.22));
#25621=CARTESIAN_POINT('Ctrl Pts',(-43.9124644151856,27.8530286452862,14.22));
#25622=CARTESIAN_POINT('',(-31.403991691448,20.1821259000137,-1.84276521465446E-29));
#25623=CARTESIAN_POINT('Origin',(-32.9182507396841,21.1552751870377,0.));
#25624=CARTESIAN_POINT('Origin',(-32.9182507396841,21.1552751870377,0.));
#25625=CARTESIAN_POINT('Ctrl Pts',(-27.7725495286736,25.640424970686,0.));
#25626=CARTESIAN_POINT('Ctrl Pts',(-27.9128768288047,25.4784786333244,3.24562220582793));
#25627=CARTESIAN_POINT('Ctrl Pts',(-29.1174678338685,26.2387220458134,6.16982677025167));
#25628=CARTESIAN_POINT('Ctrl Pts',(-30.3220588389323,26.9989654583025,9.09403133467541));
#25629=CARTESIAN_POINT('Ctrl Pts',(-32.3801230698291,28.4987476307693,11.1176436806954));
#25630=CARTESIAN_POINT('Ctrl Pts',(-34.4381873007258,29.9985298032361,13.1412560267153));
#25631=CARTESIAN_POINT('Ctrl Pts',(-36.9698934388174,31.9087250245464,13.8634749112255));
#25632=CARTESIAN_POINT('Ctrl Pts',(-39.501599576909,33.8189202458566,14.5856937957357));
#25633=CARTESIAN_POINT('Ctrl Pts',(-42.0333057150006,35.7291154671669,13.8634749112255));
#25634=CARTESIAN_POINT('Ctrl Pts',(-29.3462831821136,27.4145036200623,0.));
#25635=CARTESIAN_POINT('Ctrl Pts',(-29.4866104822448,27.2525572827007,2.70899372698069));
#25636=CARTESIAN_POINT('Ctrl Pts',(-30.5152370105913,27.8603266081619,5.14971273833323));
#25637=CARTESIAN_POINT('Ctrl Pts',(-31.5438635389379,28.4680959336232,7.59043174968578));
#25638=CARTESIAN_POINT('Ctrl Pts',(-33.2848507390767,29.6931292949421,9.27946171175752));
#25639=CARTESIAN_POINT('Ctrl Pts',(-35.0258379392155,30.9181626562611,10.9684916738293));
#25640=CARTESIAN_POINT('Ctrl Pts',(-37.1621554871447,32.4857517139243,11.5712994880388));
#25641=CARTESIAN_POINT('Ctrl Pts',(-39.2984730350738,34.0533407715876,12.1741073022483));
#25642=CARTESIAN_POINT('Ctrl Pts',(-41.434790583003,35.6209298292508,11.5712994880388));
#25643=CARTESIAN_POINT('Ctrl Pts',(-30.5436667170411,29.4615173807457,0.));
#25644=CARTESIAN_POINT('Ctrl Pts',(-30.6839940171722,29.2995710433841,2.19648874705824));
#25645=CARTESIAN_POINT('Ctrl Pts',(-31.544566343847,29.7617205741622,4.17545672685568));
#25646=CARTESIAN_POINT('Ctrl Pts',(-32.4051386705217,30.2238701049402,6.15442470665313));
#25647=CARTESIAN_POINT('Ctrl Pts',(-33.8433026630076,31.1865056631393,7.5239130403414));
#25648=CARTESIAN_POINT('Ctrl Pts',(-35.2814666554934,32.1491412213384,8.89340137402968));
#25649=CARTESIAN_POINT('Ctrl Pts',(-37.040169839947,33.3895255704509,9.3821661014496));
#25650=CARTESIAN_POINT('Ctrl Pts',(-38.7988730244006,34.6299099195635,9.87093082886954));
#25651=CARTESIAN_POINT('Ctrl Pts',(-40.5575762088542,35.870294268676,9.38216610144961));
#25652=CARTESIAN_POINT('Ctrl Pts',(-31.3186840564483,31.7027984407114,0.));
#25653=CARTESIAN_POINT('Ctrl Pts',(-31.4590113565795,31.5408521033498,1.72780310113343));
#25654=CARTESIAN_POINT('Ctrl Pts',(-32.165898167705,31.869832376844,3.28449990511991));
#25655=CARTESIAN_POINT('Ctrl Pts',(-32.8727849788305,32.1988126503382,4.84119670910639));
#25656=CARTESIAN_POINT('Ctrl Pts',(-34.0340172414016,32.9214854985885,5.91846432228298));
#25657=CARTESIAN_POINT('Ctrl Pts',(-35.1952495039727,33.6441583468387,6.99573193545957));
#25658=CARTESIAN_POINT('Ctrl Pts',(-36.6086244696003,34.5853140909923,7.38020429521639));
#25659=CARTESIAN_POINT('Ctrl Pts',(-38.021999435228,35.5264698351459,7.76467665497321));
#25660=CARTESIAN_POINT('Ctrl Pts',(-39.4353744008557,36.4676255792995,7.38020429521639));
#25661=CARTESIAN_POINT('',(-27.7725495286901,25.6404249707042,1.57950157595365E-9));
#25662=CARTESIAN_POINT('Origin',(-14.30703348905,37.5852932322718,0.));
#25663=CARTESIAN_POINT('Ctrl Pts',(-27.7725495288657,25.6404249705938,3.13107855620726E-9));
#25664=CARTESIAN_POINT('Ctrl Pts',(-27.7831439665412,25.6281983378205,0.245038153335483));
#25665=CARTESIAN_POINT('Ctrl Pts',(-27.7986217084843,25.620014287052,0.490791160521711));
#25666=CARTESIAN_POINT('Ctrl Pts',(-27.8190271851149,25.615952633098,0.736766500725353));
#25667=CARTESIAN_POINT('Ctrl Pts',(-27.8393656717117,25.6119043133258,0.981934317701018));
#25668=CARTESIAN_POINT('Ctrl Pts',(-27.8645996505508,25.6119514551674,1.22732257376568));
#25669=CARTESIAN_POINT('Ctrl Pts',(-27.8947338787562,25.6161410294535,1.47243294816347));
#25670=CARTESIAN_POINT('Ctrl Pts',(-27.9248227237927,25.6203242940987,1.7171741780302));
#25671=CARTESIAN_POINT('Ctrl Pts',(-27.9597970874097,25.6286375769735,1.96163791541586));
#25672=CARTESIAN_POINT('Ctrl Pts',(-27.9996219245318,25.6410945477696,2.20532408778522));
#25673=CARTESIAN_POINT('Ctrl Pts',(-28.0394126058352,25.65354083483,2.44880126242065));
#25674=CARTESIAN_POINT('Ctrl Pts',(-28.0840454126419,25.6701237175579,2.69150175431052));
#25675=CARTESIAN_POINT('Ctrl Pts',(-28.1334457426219,25.6908232719759,2.93292951866812));
#25676=CARTESIAN_POINT('Ctrl Pts',(-28.1828357379544,25.7115184960059,3.17430677585587));
#25677=CARTESIAN_POINT('Ctrl Pts',(-28.2369911812593,25.7363286400398,3.41441139318335));
#25678=CARTESIAN_POINT('Ctrl Pts',(-28.2957987052584,25.7652003562646,3.65275710614621));
#25679=CARTESIAN_POINT('Ctrl Pts',(-28.354680902112,25.7941087333334,3.89140546668766));
#25680=CARTESIAN_POINT('Ctrl Pts',(-28.4182268780896,25.8270889373971,4.12829002081136));
#25681=CARTESIAN_POINT('Ctrl Pts',(-28.4862854384143,25.8640546001338,4.36293874377775));
#25682=CARTESIAN_POINT('Ctrl Pts',(-28.5544134456108,25.9010579825875,4.59782690201417));
#25683=CARTESIAN_POINT('Ctrl Pts',(-28.6270630772619,25.9420548501734,4.83047425894929));
#25684=CARTESIAN_POINT('Ctrl Pts',(-28.7040474659736,25.9869270447948,5.06042975959402));
#25685=CARTESIAN_POINT('Ctrl Pts',(-28.781256926861,26.0319304281238,5.29105755998291));
#25686=CARTESIAN_POINT('Ctrl Pts',(-28.862826319325,26.0808316886118,5.51897736305688));
#25687=CARTESIAN_POINT('Ctrl Pts',(-28.9485346007075,26.1334818341725,5.74376259354345));
#25688=CARTESIAN_POINT('Ctrl Pts',(-29.0031847495426,26.1670531325894,5.88709234072629));
#25689=CARTESIAN_POINT('Ctrl Pts',(-29.0595170057057,26.2021480259522,6.02914825314197));
#25690=CARTESIAN_POINT('Ctrl Pts',(-29.1174678338916,26.2387220458402,6.16982677023484));
#25691=CARTESIAN_POINT('Ctrl Pts',(-29.2083364372325,26.2960711849263,6.39041482339091));
#25692=CARTESIAN_POINT('Ctrl Pts',(-29.3038406779898,26.3572486158601,6.60890054011807));
#25693=CARTESIAN_POINT('Ctrl Pts',(-29.4038573838825,26.4221888209395,6.82480412008045));
#25694=CARTESIAN_POINT('Ctrl Pts',(-29.5036482964479,26.4869824198611,7.04022028559295));
#25695=CARTESIAN_POINT('Ctrl Pts',(-29.607931238224,26.5555217851615,7.25306552029639));
#25696=CARTESIAN_POINT('Ctrl Pts',(-29.7165449255438,26.6277100364535,7.46287566269419));
#25697=CARTESIAN_POINT('Ctrl Pts',(-29.8249839175527,26.6997821794601,7.67234834441887));
#25698=CARTESIAN_POINT('Ctrl Pts',(-29.9377396021008,26.7754914030013,7.87879526533038));
#25699=CARTESIAN_POINT('Ctrl Pts',(-30.0546142350032,26.854710408865,8.08177334612208));
#25700=CARTESIAN_POINT('Ctrl Pts',(-30.1713767224895,26.9338534012418,8.28455666214101));
#25701=CARTESIAN_POINT('Ctrl Pts',(-30.2922500787579,27.0164993284346,8.48387739272823));
#25702=CARTESIAN_POINT('Ctrl Pts',(-30.4170022653822,27.1024918458753,8.67931873611042));
#25703=CARTESIAN_POINT('Ctrl Pts',(-30.5417604522567,27.1884884993287,8.87476947970428));
#25704=CARTESIAN_POINT('Ctrl Pts',(-30.6703976233159,27.2778319154178,9.06634009532753));
#25705=CARTESIAN_POINT('Ctrl Pts',(-30.8026498047312,27.3703382785457,9.25364450340897));
#25706=CARTESIAN_POINT('Ctrl Pts',(-30.934950501554,27.46287857672,9.44101762226397));
#25707=CARTESIAN_POINT('Ctrl Pts',(-31.0708686028426,27.5585839591967,9.62412107874923));
#25708=CARTESIAN_POINT('Ctrl Pts',(-31.2101115092129,27.6572454428932,9.80260437466004));
#25709=CARTESIAN_POINT('Ctrl Pts',(-31.3495815496047,27.7560678639054,9.98137881379558));
#25710=CARTESIAN_POINT('Ctrl Pts',(-31.4923869622799,27.8578558275192,10.1555177270912));
#25711=CARTESIAN_POINT('Ctrl Pts',(-31.6382093995766,27.9623772429043,10.3247095747696));
#25712=CARTESIAN_POINT('Ctrl Pts',(-31.6803570199432,27.9925874699277,10.3736117457747));
#25713=CARTESIAN_POINT('Ctrl Pts',(-31.7227565449037,28.0230259217675,10.4221009095753));
#25714=CARTESIAN_POINT('Ctrl Pts',(-31.7653999649278,28.0536866918426,10.4701702229111));
#25715=CARTESIAN_POINT('Ctrl Pts',(-35.8372231206708,26.488126377667,1.04083408558608E-14));
#25716=CARTESIAN_POINT('Ctrl Pts',(-35.977550420802,26.3261800403054,1.72780310113343));
#25717=CARTESIAN_POINT('Ctrl Pts',(-36.6844372319275,26.6551603137996,3.28449990511992));
#25718=CARTESIAN_POINT('Ctrl Pts',(-37.391324043053,26.9841405872938,4.84119670910639));
#25719=CARTESIAN_POINT('Ctrl Pts',(-38.5525563056241,27.7068134355441,5.91846432228298));
#25720=CARTESIAN_POINT('Ctrl Pts',(-39.7137885681951,28.4294862837944,6.99573193545956));
#25721=CARTESIAN_POINT('Ctrl Pts',(-41.1271635338228,29.3706420279479,7.3802042952164));
#25722=CARTESIAN_POINT('Ctrl Pts',(-42.5405384994505,30.3117977721015,7.76467665497322));
#25723=CARTESIAN_POINT('Ctrl Pts',(-43.9539134650781,31.2529535162551,7.38020429521639));
#25724=CARTESIAN_POINT('Ctrl Pts',(-33.5084586029185,26.0399651488662,-1.05434036998093E-14));
#25725=CARTESIAN_POINT('Ctrl Pts',(-33.6487859030496,25.8780188115046,2.19648874705822));
#25726=CARTESIAN_POINT('Ctrl Pts',(-34.5093582297244,26.3401683422826,4.17545672685568));
#25727=CARTESIAN_POINT('Ctrl Pts',(-35.3699305563991,26.8023178730606,6.15442470665313));
#25728=CARTESIAN_POINT('Ctrl Pts',(-36.8080945488849,27.7649534312597,7.5239130403414));
#25729=CARTESIAN_POINT('Ctrl Pts',(-38.2462585413708,28.7275889894589,8.89340137402966));
#25730=CARTESIAN_POINT('Ctrl Pts',(-40.0049617258244,29.9679733385714,9.3821661014496));
#25731=CARTESIAN_POINT('Ctrl Pts',(-41.7636649102779,31.2083576876839,9.87093082886953));
#25732=CARTESIAN_POINT('Ctrl Pts',(-43.5223680947315,32.4487420367965,9.3821661014496));
#25733=CARTESIAN_POINT('Ctrl Pts',(-31.3118750466444,25.1460896841346,0.));
#25734=CARTESIAN_POINT('Ctrl Pts',(-31.4522023467755,24.984143346773,2.7089937269807));
#25735=CARTESIAN_POINT('Ctrl Pts',(-32.4808288751221,25.5919126722343,5.14971273833323));
#25736=CARTESIAN_POINT('Ctrl Pts',(-33.5094554034686,26.1996819976955,7.59043174968577));
#25737=CARTESIAN_POINT('Ctrl Pts',(-35.2504426036075,27.4247153590145,9.27946171175751));
#25738=CARTESIAN_POINT('Ctrl Pts',(-36.9914298037463,28.6497487203334,10.9684916738293));
#25739=CARTESIAN_POINT('Ctrl Pts',(-39.1277473516755,30.2173377779966,11.5712994880388));
#25740=CARTESIAN_POINT('Ctrl Pts',(-41.2640648996046,31.7849268356598,12.1741073022483));
#25741=CARTESIAN_POINT('Ctrl Pts',(-43.4003824475338,33.3525158933231,11.5712994880388));
#25742=CARTESIAN_POINT('Ctrl Pts',(-29.331888309534,23.8408520862201,0.));
#25743=CARTESIAN_POINT('Ctrl Pts',(-29.4722156096651,23.6789057488585,3.24562220582793));
#25744=CARTESIAN_POINT('Ctrl Pts',(-30.6768066147289,24.4391491613476,6.16982677025168));
#25745=CARTESIAN_POINT('Ctrl Pts',(-31.8813976197927,25.1993925738367,9.09403133467541));
#25746=CARTESIAN_POINT('Ctrl Pts',(-33.9394618506895,26.6991747463035,11.1176436806954));
#25747=CARTESIAN_POINT('Ctrl Pts',(-35.9975260815862,28.1989569187703,13.1412560267153));
#25748=CARTESIAN_POINT('Ctrl Pts',(-38.5292322196779,30.1091521400805,13.8634749112255));
#25749=CARTESIAN_POINT('Ctrl Pts',(-41.0609383577695,32.0193473613908,14.5856937957357));
#25750=CARTESIAN_POINT('Ctrl Pts',(-43.5926444958611,33.929542582701,13.8634749112255));
#25751=CARTESIAN_POINT('',(-29.331888309534,23.8408520862201,0.));
#25752=CARTESIAN_POINT('Ctrl Pts',(-29.331888309534,23.8408520862201,0.));
#25753=CARTESIAN_POINT('Ctrl Pts',(-29.4722156096651,23.6789057488585,3.24562220582793));
#25754=CARTESIAN_POINT('Ctrl Pts',(-30.6768066147289,24.4391491613476,6.16982677025168));
#25755=CARTESIAN_POINT('Ctrl Pts',(-31.6824449968207,25.0738292744462,8.61106394926976));
#25756=CARTESIAN_POINT('Ctrl Pts',(-33.305918063411,26.2405847244739,10.4489096280657));
#25757=CARTESIAN_POINT('Origin',(-39.2388322978494,8.81246358936587,0.));
#25758=CARTESIAN_POINT('Ctrl Pts',(-29.331888309534,23.8408520862201,0.));
#25759=CARTESIAN_POINT('Ctrl Pts',(-29.4722156096651,23.6789057488585,3.24562220582793));
#25760=CARTESIAN_POINT('Ctrl Pts',(-30.6768066147289,24.4391491613476,6.16982677025168));
#25761=CARTESIAN_POINT('Ctrl Pts',(-31.8813976197927,25.1993925738367,9.09403133467541));
#25762=CARTESIAN_POINT('Ctrl Pts',(-33.9394618506895,26.6991747463035,11.1176436806954));
#25763=CARTESIAN_POINT('Ctrl Pts',(-35.9975260815862,28.1989569187703,13.1412560267153));
#25764=CARTESIAN_POINT('Ctrl Pts',(-38.5292322196779,30.1091521400805,13.8634749112255));
#25765=CARTESIAN_POINT('Ctrl Pts',(-41.0609383577695,32.0193473613908,14.5856937957357));
#25766=CARTESIAN_POINT('Ctrl Pts',(-43.5926444958611,33.929542582701,13.8634749112255));
#25767=CARTESIAN_POINT('Ctrl Pts',(-28.3879644434327,23.9681616891744,0.));
#25768=CARTESIAN_POINT('Ctrl Pts',(-28.5282917435638,23.8062153518127,3.38941559469371));
#25769=CARTESIAN_POINT('Ctrl Pts',(-29.7800336722639,24.6073152722066,6.44317352589573));
#25770=CARTESIAN_POINT('Ctrl Pts',(-31.0317756009639,25.4084151926005,9.49693145709774));
#25771=CARTESIAN_POINT('Ctrl Pts',(-33.1748028604389,26.9818182484141,11.6101975146502));
#25772=CARTESIAN_POINT('Ctrl Pts',(-35.3178301199139,28.5552213042277,13.7234635722027));
#25773=CARTESIAN_POINT('Ctrl Pts',(-37.9554834217126,30.5572202654791,14.4776794959001));
#25774=CARTESIAN_POINT('Ctrl Pts',(-40.5931367235113,32.5592192267305,15.2318954195974));
#25775=CARTESIAN_POINT('Ctrl Pts',(-43.23079002531,34.5612181879819,14.4776794959001));
#25776=CARTESIAN_POINT('Ctrl Pts',(-27.7642289310885,24.6879908429607,6.24500451351651E-15));
#25777=CARTESIAN_POINT('Ctrl Pts',(-27.9045562312196,24.5260445055991,3.38941559469371));
#25778=CARTESIAN_POINT('Ctrl Pts',(-29.1562981599197,25.3271444259929,6.44317352589573));
#25779=CARTESIAN_POINT('Ctrl Pts',(-30.4080400886198,26.1282443463868,9.49693145709773));
#25780=CARTESIAN_POINT('Ctrl Pts',(-32.5510673480947,27.7016474022004,11.6101975146502));
#25781=CARTESIAN_POINT('Ctrl Pts',(-34.6940946075697,29.275050458014,13.7234635722027));
#25782=CARTESIAN_POINT('Ctrl Pts',(-37.3317479093684,31.2770494192654,14.4776794959001));
#25783=CARTESIAN_POINT('Ctrl Pts',(-39.9694012111672,33.2790483805169,15.2318954195974));
#25784=CARTESIAN_POINT('Ctrl Pts',(-42.6070545129659,35.2810473417683,14.4776794959001));
#25785=CARTESIAN_POINT('Ctrl Pts',(-27.7725495286736,25.640424970686,0.));
#25786=CARTESIAN_POINT('Ctrl Pts',(-27.9128768288047,25.4784786333244,3.24562220582793));
#25787=CARTESIAN_POINT('Ctrl Pts',(-29.1174678338685,26.2387220458134,6.16982677025167));
#25788=CARTESIAN_POINT('Ctrl Pts',(-30.3220588389323,26.9989654583025,9.09403133467541));
#25789=CARTESIAN_POINT('Ctrl Pts',(-32.3801230698291,28.4987476307693,11.1176436806954));
#25790=CARTESIAN_POINT('Ctrl Pts',(-34.4381873007258,29.9985298032361,13.1412560267153));
#25791=CARTESIAN_POINT('Ctrl Pts',(-36.9698934388174,31.9087250245464,13.8634749112255));
#25792=CARTESIAN_POINT('Ctrl Pts',(-39.501599576909,33.8189202458566,14.5856937957357));
#25793=CARTESIAN_POINT('Ctrl Pts',(-42.0333057150006,35.7291154671669,13.8634749112255));
#25794=CARTESIAN_POINT('',(-28.2121283533394,24.4459549573185,-1.89568229885776E-29));
#25795=CARTESIAN_POINT('Origin',(-29.572480844482,25.6247005192792,0.));
#25796=CARTESIAN_POINT('Origin',(-29.572480844482,25.6247005192792,0.));
#25797=CARTESIAN_POINT('Ctrl Pts',(-23.8408520862198,29.3318883095343,0.));
#25798=CARTESIAN_POINT('Ctrl Pts',(-24.0027984235814,29.1915610094031,3.24562220582793));
#25799=CARTESIAN_POINT('Ctrl Pts',(-25.0869345107938,30.1154974142047,6.16982677025168));
#25800=CARTESIAN_POINT('Ctrl Pts',(-26.1710705980061,31.0394338190062,9.09403133467542));
#25801=CARTESIAN_POINT('Ctrl Pts',(-27.9947454451961,32.8168434496407,11.1176436806954));
#25802=CARTESIAN_POINT('Ctrl Pts',(-29.8184202923862,34.5942530802753,13.1412560267153));
#25803=CARTESIAN_POINT('Ctrl Pts',(-32.0525081884196,36.8453046181046,13.8634749112255));
#25804=CARTESIAN_POINT('Ctrl Pts',(-34.2865960844531,39.096356155934,14.5856937957357));
#25805=CARTESIAN_POINT('Ctrl Pts',(-36.5206839804866,41.3474076937634,13.8634749112255));
#25806=CARTESIAN_POINT('Ctrl Pts',(-25.1460896841343,31.3118750466447,0.));
#25807=CARTESIAN_POINT('Ctrl Pts',(-25.3080360214959,31.1715477465136,2.70899372698069));
#25808=CARTESIAN_POINT('Ctrl Pts',(-26.2396980216804,31.9195196745979,5.14971273833323));
#25809=CARTESIAN_POINT('Ctrl Pts',(-27.1713600218649,32.6674916026822,7.59043174968577));
#25810=CARTESIAN_POINT('Ctrl Pts',(-28.7202860579071,34.1278242025587,9.27946171175752));
#25811=CARTESIAN_POINT('Ctrl Pts',(-30.2692120939493,35.5881568024353,10.9684916738293));
#25812=CARTESIAN_POINT('Ctrl Pts',(-32.1606938263357,37.4438197501022,11.5712994880388));
#25813=CARTESIAN_POINT('Ctrl Pts',(-34.0521755587222,39.2994826977691,12.1741073022483));
#25814=CARTESIAN_POINT('Ctrl Pts',(-35.9436572911087,41.1551456454361,11.5712994880388));
#25815=CARTESIAN_POINT('Ctrl Pts',(-26.0399651488659,33.5084586029188,0.));
#25816=CARTESIAN_POINT('Ctrl Pts',(-26.2019114862275,33.3681313027876,2.19648874705823));
#25817=CARTESIAN_POINT('Ctrl Pts',(-26.9879536917288,33.9480490292001,4.17545672685568));
#25818=CARTESIAN_POINT('Ctrl Pts',(-27.7739958972301,34.5279667556126,6.15442470665314));
#25819=CARTESIAN_POINT('Ctrl Pts',(-29.0605241301524,35.6854761478362,7.5239130403414));
#25820=CARTESIAN_POINT('Ctrl Pts',(-30.3470523630747,36.8429855400598,8.89340137402968));
#25821=CARTESIAN_POINT('Ctrl Pts',(-31.9113293869105,38.3210341242511,9.38216610144961));
#25822=CARTESIAN_POINT('Ctrl Pts',(-33.4756064107463,39.7990827084424,9.87093082886954));
#25823=CARTESIAN_POINT('Ctrl Pts',(-35.039883434582,41.2771312926338,9.38216610144961));
#25824=CARTESIAN_POINT('Ctrl Pts',(-26.4881263776667,35.8372231206711,0.));
#25825=CARTESIAN_POINT('Ctrl Pts',(-26.6500727150283,35.69689582054,1.72780310113343));
#25826=CARTESIAN_POINT('Ctrl Pts',(-27.3029456632458,36.1231280314033,3.28449990511992));
#25827=CARTESIAN_POINT('Ctrl Pts',(-27.9558186114632,36.5493602422666,4.84119670910639));
#25828=CARTESIAN_POINT('Ctrl Pts',(-29.0023841344367,37.4299379045754,5.91846432228298));
#25829=CARTESIAN_POINT('Ctrl Pts',(-30.0489496574102,38.3105155668841,6.99573193545957));
#25830=CARTESIAN_POINT('Ctrl Pts',(-31.313998076287,39.4432359322496,7.3802042952164));
#25831=CARTESIAN_POINT('Ctrl Pts',(-32.5790464951638,40.575956297615,7.76467665497322));
#25832=CARTESIAN_POINT('Ctrl Pts',(-33.8440949140406,41.7086766629804,7.38020429521639));
#25833=CARTESIAN_POINT('',(-23.8408520862339,29.3318883095431,1.5794998097385E-9));
#25834=CARTESIAN_POINT('Origin',(-8.81246358936545,39.2388322978495,0.));
#25835=CARTESIAN_POINT('Ctrl Pts',(-23.8408520864231,29.3318883094703,3.1310741434434E-9));
#25836=CARTESIAN_POINT('Ctrl Pts',(-23.8530787192647,29.3212938718737,0.24503815333526));
#25837=CARTESIAN_POINT('Ctrl Pts',(-23.8695636319734,29.3153958352831,0.490791160521269));
#25838=CARTESIAN_POINT('Ctrl Pts',(-23.8903394438997,29.3142795252165,0.736766500724692));
#25839=CARTESIAN_POINT('Ctrl Pts',(-23.9110470500023,29.3131668799331,0.981934317700348));
#25840=CARTESIAN_POINT('Ctrl Pts',(-23.9360174743377,29.3168047115562,1.22732257376501));
#25841=CARTESIAN_POINT('Ctrl Pts',(-23.965248740963,29.3252401898305,1.47243294816278));
#25842=CARTESIAN_POINT('Ctrl Pts',(-23.99443598431,29.3336629639885,1.71717417802956));
#25843=CARTESIAN_POINT('Ctrl Pts',(-24.0278712558265,29.3468690005323,1.96163791541528));
#25844=CARTESIAN_POINT('Ctrl Pts',(-24.0655179217451,29.3648668425815,2.20532408778468));
#25845=CARTESIAN_POINT('Ctrl Pts',(-24.1031322999561,29.3828492487602,2.44880126242007));
#25846=CARTESIAN_POINT('Ctrl Pts',(-24.1449508188712,29.4056152523348,2.69150175430988));
#25847=CARTESIAN_POINT('Ctrl Pts',(-24.190902470982,29.4331345151068,2.93292951866742));
#25848=CARTESIAN_POINT('Ctrl Pts',(-24.2368445099157,29.4606480207943,3.17430677585524));
#25849=CARTESIAN_POINT('Ctrl Pts',(-24.2869178772577,29.4929127564908,3.41441139318279));
#25850=CARTESIAN_POINT('Ctrl Pts',(-24.3410179518308,29.5298597835412,3.65275710614572));
#25851=CARTESIAN_POINT('Ctrl Pts',(-24.3951867218143,29.5668537253362,3.89140546668722));
#25852=CARTESIAN_POINT('Ctrl Pts',(-24.4533923189746,29.6085417737703,4.12829002081097));
#25853=CARTESIAN_POINT('Ctrl Pts',(-24.5154973789735,29.6548169223661,4.3629387437774));
#25854=CARTESIAN_POINT('Ctrl Pts',(-24.5776658108998,29.7011392900669,4.59782690201371));
#25855=CARTESIAN_POINT('Ctrl Pts',(-24.6437415114725,29.7520579892324,4.83047425894872));
#25856=CARTESIAN_POINT('Ctrl Pts',(-24.7135563309889,29.8074294704419,5.06042975959335));
#25857=CARTESIAN_POINT('Ctrl Pts',(-24.783575261671,29.8629628361575,5.29105755998213));
#25858=CARTESIAN_POINT('Ctrl Pts',(-24.8573550203554,29.92297488722,5.51897736305601));
#25859=CARTESIAN_POINT('Ctrl Pts',(-24.9346980180639,29.9872866904179,5.7437625935425));
#25860=CARTESIAN_POINT('Ctrl Pts',(-24.9840142132781,30.0282938085158,5.88709234072565));
#25861=CARTESIAN_POINT('Ctrl Pts',(-25.0347785642249,30.0710484023923,6.02914825314166));
#25862=CARTESIAN_POINT('Ctrl Pts',(-25.0869345108128,30.1154974142344,6.16982677023484));
#25863=CARTESIAN_POINT('Ctrl Pts',(-25.1687165693393,30.1851947723639,6.39041482339095));
#25864=CARTESIAN_POINT('Ctrl Pts',(-25.2545422584421,30.2593411758391,6.60890054011814));
#25865=CARTESIAN_POINT('Ctrl Pts',(-25.3442989836977,30.3378542445906,6.82480412008054));
#25866=CARTESIAN_POINT('Ctrl Pts',(-25.4338530781081,30.4161900656827,7.040220285593));
#25867=CARTESIAN_POINT('Ctrl Pts',(-25.5273204012124,30.4988728090635,7.2530655202964));
#25868=CARTESIAN_POINT('Ctrl Pts',(-25.6245550984954,30.5857836273893,7.46287566269415));
#25869=CARTESIAN_POINT('Ctrl Pts',(-25.7216334025458,30.6725546575099,7.6723483444188));
#25870=CARTESIAN_POINT('Ctrl Pts',(-25.8224668509014,30.76354007733,7.87879526533026));
#25871=CARTESIAN_POINT('Ctrl Pts',(-25.9268778285525,30.8585857424181,8.08177334612193));
#25872=CARTESIAN_POINT('Ctrl Pts',(-26.0311886201134,30.9535402077704,8.2845566621412));
#25873=CARTESIAN_POINT('Ctrl Pts',(-26.1390699181377,31.052546990739,8.48387739272874));
#25874=CARTESIAN_POINT('Ctrl Pts',(-26.2503142961679,31.155418315607,8.67931873611125));
#25875=CARTESIAN_POINT('Ctrl Pts',(-26.3615640247582,31.2582945883135,8.8747694797051));
#25876=CARTESIAN_POINT('Ctrl Pts',(-26.476176961084,31.3650355954446,9.06634009532834));
#25877=CARTESIAN_POINT('Ctrl Pts',(-26.5939179778766,31.4754218249885,9.25364450340976));
#25878=CARTESIAN_POINT('Ctrl Pts',(-26.7117021867993,31.5858485486313,9.44101762226492));
#25879=CARTESIAN_POINT('Ctrl Pts',(-26.8326165417655,31.6999229509135,9.62412107875032));
#25880=CARTESIAN_POINT('Ctrl Pts',(-26.9564011630247,31.8173965346651,9.80260437466126));
#25881=CARTESIAN_POINT('Ctrl Pts',(-27.0803877026406,31.935061742164,9.98137881379697));
#25882=CARTESIAN_POINT('Ctrl Pts',(-27.2072536245434,32.0561369802839,10.1555177270928));
#25883=CARTESIAN_POINT('Ctrl Pts',(-27.3367168513606,32.1803472149485,10.3247095747713));
#25884=CARTESIAN_POINT('Ctrl Pts',(-27.3741361061489,32.2162481771947,10.3736117457742));
#25885=CARTESIAN_POINT('Ctrl Pts',(-27.4117722217278,32.2524108910194,10.4221009095725));
#25886=CARTESIAN_POINT('Ctrl Pts',(-27.4496181106865,32.2888283700868,10.4701702229062));
#25887=CARTESIAN_POINT('Ctrl Pts',(-31.7027984407111,31.3186840564487,0.));
#25888=CARTESIAN_POINT('Ctrl Pts',(-31.8647447780727,31.1783567563176,1.72780310113342));
#25889=CARTESIAN_POINT('Ctrl Pts',(-32.5176177262902,31.6045889671808,3.28449990511991));
#25890=CARTESIAN_POINT('Ctrl Pts',(-33.1704906745076,32.0308211780441,4.84119670910638));
#25891=CARTESIAN_POINT('Ctrl Pts',(-34.2170561974811,32.9113988403529,5.91846432228298));
#25892=CARTESIAN_POINT('Ctrl Pts',(-35.2636217204547,33.7919765026617,6.99573193545956));
#25893=CARTESIAN_POINT('Ctrl Pts',(-36.5286701393314,34.9246968680271,7.38020429521639));
#25894=CARTESIAN_POINT('Ctrl Pts',(-37.7937185582083,36.0574172333925,7.76467665497321));
#25895=CARTESIAN_POINT('Ctrl Pts',(-39.0587669770851,37.1901375987579,7.38020429521639));
#25896=CARTESIAN_POINT('Ctrl Pts',(-29.4615173807454,30.5436667170414,0.));
#25897=CARTESIAN_POINT('Ctrl Pts',(-29.6234637181071,30.4033394169103,2.19648874705824));
#25898=CARTESIAN_POINT('Ctrl Pts',(-30.4095059236083,30.9832571433228,4.17545672685567));
#25899=CARTESIAN_POINT('Ctrl Pts',(-31.1955481291096,31.5631748697353,6.15442470665313));
#25900=CARTESIAN_POINT('Ctrl Pts',(-32.4820763620319,32.7206842619589,7.5239130403414));
#25901=CARTESIAN_POINT('Ctrl Pts',(-33.7686045949543,33.8781936541824,8.89340137402967));
#25902=CARTESIAN_POINT('Ctrl Pts',(-35.3328816187901,35.3562422383738,9.3821661014496));
#25903=CARTESIAN_POINT('Ctrl Pts',(-36.8971586426258,36.8342908225651,9.87093082886954));
#25904=CARTESIAN_POINT('Ctrl Pts',(-38.4614356664616,38.3123394067564,9.3821661014496));
#25905=CARTESIAN_POINT('Ctrl Pts',(-27.414503620062,29.3462831821139,0.));
#25906=CARTESIAN_POINT('Ctrl Pts',(-27.5764499574236,29.2059558819828,2.70899372698069));
#25907=CARTESIAN_POINT('Ctrl Pts',(-28.5081119576081,29.9539278100671,5.14971273833323));
#25908=CARTESIAN_POINT('Ctrl Pts',(-29.4397739577926,30.7018997381514,7.59043174968578));
#25909=CARTESIAN_POINT('Ctrl Pts',(-30.9886999938348,32.162232338028,9.27946171175752));
#25910=CARTESIAN_POINT('Ctrl Pts',(-32.537626029877,33.6225649379046,10.9684916738293));
#25911=CARTESIAN_POINT('Ctrl Pts',(-34.4291077622634,35.4782278855715,11.5712994880388));
#25912=CARTESIAN_POINT('Ctrl Pts',(-36.3205894946499,37.3338908332384,12.1741073022483));
#25913=CARTESIAN_POINT('Ctrl Pts',(-38.2120712270364,39.1895537809053,11.5712994880388));
#25914=CARTESIAN_POINT('Ctrl Pts',(-25.6404249706857,27.7725495286739,1.04083408558608E-14));
#25915=CARTESIAN_POINT('Ctrl Pts',(-25.8023713080473,27.6322222285427,3.24562220582793));
#25916=CARTESIAN_POINT('Ctrl Pts',(-26.8865073952596,28.5561586333443,6.16982677025167));
#25917=CARTESIAN_POINT('Ctrl Pts',(-27.970643482472,29.4800950381458,9.09403133467541));
#25918=CARTESIAN_POINT('Ctrl Pts',(-29.794318329662,31.2575046687803,11.1176436806954));
#25919=CARTESIAN_POINT('Ctrl Pts',(-31.617993176852,33.0349142994148,13.1412560267153));
#25920=CARTESIAN_POINT('Ctrl Pts',(-33.8520810728855,35.2859658372442,13.8634749112255));
#25921=CARTESIAN_POINT('Ctrl Pts',(-36.086168968919,37.5370173750736,14.5856937957357));
#25922=CARTESIAN_POINT('Ctrl Pts',(-38.3202568649525,39.7880689129029,13.8634749112255));
#25923=CARTESIAN_POINT('',(-25.6404249706857,27.7725495286739,1.04083408558608E-14));
#25924=CARTESIAN_POINT('Ctrl Pts',(-25.6404249706857,27.7725495286739,1.04083408558608E-14));
#25925=CARTESIAN_POINT('Ctrl Pts',(-25.8023713080473,27.6322222285427,3.24562220582793));
#25926=CARTESIAN_POINT('Ctrl Pts',(-26.8865073952596,28.5561586333443,6.16982677025167));
#25927=CARTESIAN_POINT('Ctrl Pts',(-27.7915854309816,29.3274958817335,8.61106394926976));
#25928=CARTESIAN_POINT('Ctrl Pts',(-29.2324872694337,30.7134197505152,10.4489096280657));
#25929=CARTESIAN_POINT('Origin',(-37.5852932322716,14.3070334890504,0.));
#25930=CARTESIAN_POINT('Ctrl Pts',(-25.6404249706857,27.7725495286739,1.04083408558608E-14));
#25931=CARTESIAN_POINT('Ctrl Pts',(-25.8023713080473,27.6322222285427,3.24562220582793));
#25932=CARTESIAN_POINT('Ctrl Pts',(-26.8865073952596,28.5561586333443,6.16982677025167));
#25933=CARTESIAN_POINT('Ctrl Pts',(-27.970643482472,29.4800950381458,9.09403133467541));
#25934=CARTESIAN_POINT('Ctrl Pts',(-29.794318329662,31.2575046687803,11.1176436806954));
#25935=CARTESIAN_POINT('Ctrl Pts',(-31.617993176852,33.0349142994148,13.1412560267153));
#25936=CARTESIAN_POINT('Ctrl Pts',(-33.8520810728855,35.2859658372442,13.8634749112255));
#25937=CARTESIAN_POINT('Ctrl Pts',(-36.086168968919,37.5370173750736,14.5856937957357));
#25938=CARTESIAN_POINT('Ctrl Pts',(-38.3202568649525,39.7880689129029,13.8634749112255));
#25939=CARTESIAN_POINT('Ctrl Pts',(-24.6879908429604,27.7642289310888,0.));
#25940=CARTESIAN_POINT('Ctrl Pts',(-24.849937180322,27.6239016309577,3.38941559469372));
#25941=CARTESIAN_POINT('Ctrl Pts',(-25.9749297754391,28.5949889593955,6.44317352589574));
#25942=CARTESIAN_POINT('Ctrl Pts',(-27.0999223705562,29.5660762878332,9.49693145709774));
#25943=CARTESIAN_POINT('Ctrl Pts',(-28.9972181010931,31.428448947046,11.6101975146502));
#25944=CARTESIAN_POINT('Ctrl Pts',(-30.89451383163,33.2908216062587,13.7234635722027));
#25945=CARTESIAN_POINT('Ctrl Pts',(-33.2204054676046,35.6478203077952,14.4776794959001));
#25946=CARTESIAN_POINT('Ctrl Pts',(-35.5462971035792,38.0048190093317,15.2318954195974));
#25947=CARTESIAN_POINT('Ctrl Pts',(-37.8721887395538,40.3618177108681,14.4776794959001));
#25948=CARTESIAN_POINT('Ctrl Pts',(-23.9681616891741,28.3879644434329,0.));
#25949=CARTESIAN_POINT('Ctrl Pts',(-24.1301080265357,28.2476371433018,3.38941559469372));
#25950=CARTESIAN_POINT('Ctrl Pts',(-25.2551006216528,29.2187244717396,6.44317352589574));
#25951=CARTESIAN_POINT('Ctrl Pts',(-26.3800932167699,30.1898118001774,9.49693145709774));
#25952=CARTESIAN_POINT('Ctrl Pts',(-28.2773889473068,32.0521844593901,11.6101975146502));
#25953=CARTESIAN_POINT('Ctrl Pts',(-30.1746846778436,33.9145571186029,13.7234635722027));
#25954=CARTESIAN_POINT('Ctrl Pts',(-32.5005763138183,36.2715558201394,14.4776794959001));
#25955=CARTESIAN_POINT('Ctrl Pts',(-34.8264679497929,38.6285545216759,15.2318954195974));
#25956=CARTESIAN_POINT('Ctrl Pts',(-37.1523595857675,40.9855532232123,14.4776794959001));
#25957=CARTESIAN_POINT('Ctrl Pts',(-23.8408520862198,29.3318883095343,0.));
#25958=CARTESIAN_POINT('Ctrl Pts',(-24.0027984235814,29.1915610094031,3.24562220582793));
#25959=CARTESIAN_POINT('Ctrl Pts',(-25.0869345107938,30.1154974142047,6.16982677025168));
#25960=CARTESIAN_POINT('Ctrl Pts',(-26.1710705980061,31.0394338190062,9.09403133467541));
#25961=CARTESIAN_POINT('Ctrl Pts',(-27.9947454451961,32.8168434496407,11.1176436806954));
#25962=CARTESIAN_POINT('Ctrl Pts',(-29.8184202923862,34.5942530802752,13.1412560267153));
#25963=CARTESIAN_POINT('Ctrl Pts',(-32.0525081884196,36.8453046181046,13.8634749112255));
#25964=CARTESIAN_POINT('Ctrl Pts',(-34.2865960844531,39.096356155934,14.5856937957357));
#25965=CARTESIAN_POINT('Ctrl Pts',(-36.5206839804866,41.3474076937634,13.8634749112255));
#25966=CARTESIAN_POINT('',(-24.4459474390652,28.212134867943,-1.91000875816707E-29));
#25967=CARTESIAN_POINT('Origin',(-25.6247005192789,29.5724808444823,0.));
#25968=CARTESIAN_POINT('Origin',(-25.6247005192789,29.5724808444823,0.));
#25969=CARTESIAN_POINT('Ctrl Pts',(-19.4238236466307,32.4262389885814,0.));
#25970=CARTESIAN_POINT('Ctrl Pts',(-19.6040922608088,32.3103873848409,3.24562220582793));
#25971=CARTESIAN_POINT('Ctrl Pts',(-20.5457035458243,33.3792081011657,6.16982677025167));
#25972=CARTESIAN_POINT('Ctrl Pts',(-21.4873148308399,34.4480288174905,9.09403133467541));
#25973=CARTESIAN_POINT('Ctrl Pts',(-23.0394755334784,36.4668829718391,11.1176436806954));
#25974=CARTESIAN_POINT('Ctrl Pts',(-24.5916362361169,38.4857371261877,13.1412560267153));
#25975=CARTESIAN_POINT('Ctrl Pts',(-26.4826263031064,41.0318200627226,13.8634749112255));
#25976=CARTESIAN_POINT('Ctrl Pts',(-28.373616370096,43.5779029992574,14.5856937957357));
#25977=CARTESIAN_POINT('Ctrl Pts',(-30.2646064370856,46.1239859357923,13.8634749112255));
#25978=CARTESIAN_POINT('Ctrl Pts',(-20.4339943155205,34.5718269932685,0.));
#25979=CARTESIAN_POINT('Ctrl Pts',(-20.6142629296986,34.4559753895281,2.70899372698069));
#25980=CARTESIAN_POINT('Ctrl Pts',(-21.4299944500886,35.3289233687526,5.14971273833323));
#25981=CARTESIAN_POINT('Ctrl Pts',(-22.2457259704786,36.201871347977,7.59043174968577));
#25982=CARTESIAN_POINT('Ctrl Pts',(-23.5710591750642,37.8677750259292,9.27946171175751));
#25983=CARTESIAN_POINT('Ctrl Pts',(-24.8963923796497,39.5336787038814,10.9684916738292));
#25984=CARTESIAN_POINT('Ctrl Pts',(-26.504533183005,41.6396395952276,11.5712994880388));
#25985=CARTESIAN_POINT('Ctrl Pts',(-28.1126739863603,43.7456004865737,12.1741073022483));
#25986=CARTESIAN_POINT('Ctrl Pts',(-29.7208147897155,45.8515613779198,11.5712994880388));
#25987=CARTESIAN_POINT('Ctrl Pts',(-21.0061649833182,36.8732642383514,0.));
#25988=CARTESIAN_POINT('Ctrl Pts',(-21.1864335974963,36.7574126346109,2.19648874705823));
#25989=CARTESIAN_POINT('Ctrl Pts',(-21.8819441292786,37.4432931040927,4.17545672685567));
#25990=CARTESIAN_POINT('Ctrl Pts',(-22.577454661061,38.1291735735745,6.15442470665313));
#25991=CARTESIAN_POINT('Ctrl Pts',(-23.6861571296386,39.4579932465784,7.5239130403414));
#25992=CARTESIAN_POINT('Ctrl Pts',(-24.7948595982162,40.7868129195822,8.89340137402966));
#25993=CARTESIAN_POINT('Ctrl Pts',(-26.1328662922313,42.4724369320184,9.3821661014496));
#25994=CARTESIAN_POINT('Ctrl Pts',(-27.4708729862464,44.1580609444545,9.87093082886953));
#25995=CARTESIAN_POINT('Ctrl Pts',(-28.8088796802615,45.8436849568906,9.3821661014496));
#25996=CARTESIAN_POINT('Ctrl Pts',(-21.1183468312844,39.2421052839113,0.));
#25997=CARTESIAN_POINT('Ctrl Pts',(-21.2986154454625,39.1262536801709,1.72780310113342));
#25998=CARTESIAN_POINT('Ctrl Pts',(-21.8841839202763,39.6410609697422,3.28449990511991));
#25999=CARTESIAN_POINT('Ctrl Pts',(-22.4697523950901,40.1558682593136,4.84119670910639));
#26000=CARTESIAN_POINT('Ctrl Pts',(-23.3803461224641,41.1764247138526,5.91846432228298));
#26001=CARTESIAN_POINT('Ctrl Pts',(-24.2909398498381,42.1969811683916,6.99573193545957));
#26002=CARTESIAN_POINT('Ctrl Pts',(-25.381908984254,43.4982072348258,7.3802042952164));
#26003=CARTESIAN_POINT('Ctrl Pts',(-26.4728781186701,44.7994333012601,7.76467665497322));
#26004=CARTESIAN_POINT('Ctrl Pts',(-27.563847253086,46.1006593676943,7.3802042952164));
#26005=CARTESIAN_POINT('',(-19.4238236466434,32.4262389885921,1.57949801804089E-9));
#26006=CARTESIAN_POINT('Origin',(-3.13849734404791,40.0935818932913,0.));
#26007=CARTESIAN_POINT('Ctrl Pts',(-19.423823646841,32.426238988547,3.13107091193051E-9));
#26008=CARTESIAN_POINT('Ctrl Pts',(-19.4374335758628,32.4174924183247,0.24503815333528));
#26009=CARTESIAN_POINT('Ctrl Pts',(-19.4545900740529,32.4140004629284,0.490791160521312));
#26010=CARTESIAN_POINT('Ctrl Pts',(-19.4753132856567,32.415852221603,0.736766500724757));
#26011=CARTESIAN_POINT('Ctrl Pts',(-19.4959684641206,32.4176979010578,0.981934317700416));
#26012=CARTESIAN_POINT('Ctrl Pts',(-19.5201670081215,32.4248523667012,1.22732257376508));
#26013=CARTESIAN_POINT('Ctrl Pts',(-19.5479002488742,32.4373620269519,1.47243294816285));
#26014=CARTESIAN_POINT('Ctrl Pts',(-19.5755917224264,32.4498528472302,1.71717417802963));
#26015=CARTESIAN_POINT('Ctrl Pts',(-19.6068072561335,32.467682800622,1.96163791541534));
#26016=CARTESIAN_POINT('Ctrl Pts',(-19.6415093732946,32.4908551297616,2.20532408778474));
#26017=CARTESIAN_POINT('Ctrl Pts',(-19.6761817281438,32.5140075851257,2.44880126242014));
#26018=CARTESIAN_POINT('Ctrl Pts',(-19.7143346547168,32.542493259366,2.69150175430997));
#26019=CARTESIAN_POINT('Ctrl Pts',(-19.7559021858352,32.5762720176612,2.93292951866755));
#26020=CARTESIAN_POINT('Ctrl Pts',(-19.7974610209432,32.6100437093727,3.17430677585542));
#26021=CARTESIAN_POINT('Ctrl Pts',(-19.842432962963,32.6491062197568,3.41441139318301));
#26022=CARTESIAN_POINT('Ctrl Pts',(-19.8907242666034,32.6933764227085,3.65275710614599));
#26023=CARTESIAN_POINT('Ctrl Pts',(-19.9390768897698,32.7377028392566,3.89140546668751));
#26024=CARTESIAN_POINT('Ctrl Pts',(-19.9907572100057,32.7872500836133,4.12829002081127));
#26025=CARTESIAN_POINT('Ctrl Pts',(-20.0456444897535,32.8418926894894,4.36293874377772));
#26026=CARTESIAN_POINT('Ctrl Pts',(-20.1005877764144,32.8965910526137,4.59782690201416));
#26027=CARTESIAN_POINT('Ctrl Pts',(-20.1587444351919,32.9563950254812,4.83047425894931));
#26028=CARTESIAN_POINT('Ctrl Pts',(-20.219968457117,33.0211385895997,5.06042975959406));
#26029=CARTESIAN_POINT('Ctrl Pts',(-20.2813714740831,33.0860714385209,5.29105755998281));
#26030=CARTESIAN_POINT('Ctrl Pts',(-20.3458596558643,33.1559726078588,5.51897736305664));
#26031=CARTESIAN_POINT('Ctrl Pts',(-20.4132628895043,33.2306368658405,5.74376259354308));
#26032=CARTESIAN_POINT('Ctrl Pts',(-20.4562411955792,33.2782450169497,5.88709234072604));
#26033=CARTESIAN_POINT('Ctrl Pts',(-20.5004042255164,33.3277889511026,6.02914825314185));
#26034=CARTESIAN_POINT('Ctrl Pts',(-20.5457035458389,33.3792081011979,6.16982677023484));
#26035=CARTESIAN_POINT('Ctrl Pts',(-20.6167342126794,33.4598348411497,6.39041482339097));
#26036=CARTESIAN_POINT('Ctrl Pts',(-20.6911341865984,33.5454408102122,6.60890054011819));
#26037=CARTESIAN_POINT('Ctrl Pts',(-20.7688037431277,33.635928442969,6.82480412008062));
#26038=CARTESIAN_POINT('Ctrl Pts',(-20.8462979562736,33.7262117948161,7.04022028559307));
#26039=CARTESIAN_POINT('Ctrl Pts',(-20.9270469355453,33.8213547340593,7.25306552029646));
#26040=CARTESIAN_POINT('Ctrl Pts',(-21.0109232247565,33.921218865788,7.46287566269421));
#26041=CARTESIAN_POINT('Ctrl Pts',(-21.0946646065287,34.0209223750762,7.67234834441885));
#26042=CARTESIAN_POINT('Ctrl Pts',(-21.1815231404629,34.1253317904079,7.87879526533032));
#26043=CARTESIAN_POINT('Ctrl Pts',(-21.2713449564541,34.2342692590683,8.08177334612198));
#26044=CARTESIAN_POINT('Ctrl Pts',(-21.3610805851806,34.3431021983075,8.28455666214104));
#26045=CARTESIAN_POINT('Ctrl Pts',(-21.4537736728368,34.4564543444623,8.48387739272837));
#26046=CARTESIAN_POINT('Ctrl Pts',(-21.5492456275381,34.5741103132394,8.67931873611069));
#26047=CARTESIAN_POINT('Ctrl Pts',(-21.6447221741878,34.6917719409573,8.87476947970451));
#26048=CARTESIAN_POINT('Ctrl Pts',(-21.742977686913,34.8137376000409,9.06634009532771));
#26049=CARTESIAN_POINT('Ctrl Pts',(-21.843810671518,34.9397565506947,9.25364450340911));
#26050=CARTESIAN_POINT('Ctrl Pts',(-21.9446806457083,35.0658217301568,9.44101762226398));
#26051=CARTESIAN_POINT('Ctrl Pts',(-22.048129786773,35.1959429263773,9.62412107874912));
#26052=CARTESIAN_POINT('Ctrl Pts',(-22.1539362249973,35.3298371867842,9.80260437465981));
#26053=CARTESIAN_POINT('Ctrl Pts',(-22.259915255438,35.4639498564633,9.98137881379536));
#26054=CARTESIAN_POINT('Ctrl Pts',(-22.3682590622493,35.601847626393,10.155517727091));
#26055=CARTESIAN_POINT('Ctrl Pts',(-22.4787275806297,35.7432181181518,10.3247095747694));
#26056=CARTESIAN_POINT('Ctrl Pts',(-22.5106567217229,35.7840789755613,10.3736117457729));
#26057=CARTESIAN_POINT('Ctrl Pts',(-22.5427632651429,35.8252297828039,10.4221009095719));
#26058=CARTESIAN_POINT('Ctrl Pts',(-22.5750411898779,35.8666626160111,10.4701702229062));
#26059=CARTESIAN_POINT('Ctrl Pts',(-26.9229962078196,35.5116836434678,0.));
#26060=CARTESIAN_POINT('Ctrl Pts',(-27.1032648219977,35.3958320397273,1.72780310113342));
#26061=CARTESIAN_POINT('Ctrl Pts',(-27.6888332968115,35.9106393292986,3.28449990511991));
#26062=CARTESIAN_POINT('Ctrl Pts',(-28.2744017716253,36.42544661887,4.84119670910639));
#26063=CARTESIAN_POINT('Ctrl Pts',(-29.1849954989993,37.446003073409,5.91846432228298));
#26064=CARTESIAN_POINT('Ctrl Pts',(-30.0955892263732,38.466559527948,6.99573193545957));
#26065=CARTESIAN_POINT('Ctrl Pts',(-31.1865583607892,39.7677855943822,7.38020429521639));
#26066=CARTESIAN_POINT('Ctrl Pts',(-32.2775274952052,41.0690116608165,7.76467665497322));
#26067=CARTESIAN_POINT('Ctrl Pts',(-33.3684966296212,42.3702377272507,7.38020429521639));
#26068=CARTESIAN_POINT('Ctrl Pts',(-24.8148246247007,34.425587311519,0.));
#26069=CARTESIAN_POINT('Ctrl Pts',(-24.9950932388788,34.3097357077785,2.19648874705824));
#26070=CARTESIAN_POINT('Ctrl Pts',(-25.6906037706612,34.9956161772603,4.17545672685568));
#26071=CARTESIAN_POINT('Ctrl Pts',(-26.3861143024435,35.6814966467421,6.15442470665314));
#26072=CARTESIAN_POINT('Ctrl Pts',(-27.4948167710211,37.0103163197459,7.5239130403414));
#26073=CARTESIAN_POINT('Ctrl Pts',(-28.6035192395987,38.3391359927498,8.89340137402968));
#26074=CARTESIAN_POINT('Ctrl Pts',(-29.9415259336138,40.0247600051859,9.38216610144961));
#26075=CARTESIAN_POINT('Ctrl Pts',(-31.2795326276289,41.710384017622,9.87093082886954));
#26076=CARTESIAN_POINT('Ctrl Pts',(-32.617539321644,43.3960080300582,9.38216610144961));
#26077=CARTESIAN_POINT('Ctrl Pts',(-22.9590519566753,32.9490709821977,0.));
#26078=CARTESIAN_POINT('Ctrl Pts',(-23.1393205708534,32.8332193784572,2.70899372698069));
#26079=CARTESIAN_POINT('Ctrl Pts',(-23.9550520912434,33.7061673576817,5.14971273833323));
#26080=CARTESIAN_POINT('Ctrl Pts',(-24.7707836116334,34.5791153369062,7.59043174968577));
#26081=CARTESIAN_POINT('Ctrl Pts',(-26.0961168162189,36.2450190148584,9.27946171175751));
#26082=CARTESIAN_POINT('Ctrl Pts',(-27.4214500208045,37.9109226928106,10.9684916738293));
#26083=CARTESIAN_POINT('Ctrl Pts',(-29.0295908241597,40.0168835841567,11.5712994880388));
#26084=CARTESIAN_POINT('Ctrl Pts',(-30.637731627515,42.1228444755028,12.1741073022483));
#26085=CARTESIAN_POINT('Ctrl Pts',(-32.2458724308703,44.228805366849,11.5712994880388));
#26086=CARTESIAN_POINT('Ctrl Pts',(-21.4269965203139,31.138877952143,0.));
#26087=CARTESIAN_POINT('Ctrl Pts',(-21.6072651344921,31.0230263484025,3.24562220582793));
#26088=CARTESIAN_POINT('Ctrl Pts',(-22.5488764195076,32.0918470647273,6.16982677025168));
#26089=CARTESIAN_POINT('Ctrl Pts',(-23.4904877045231,33.1606677810521,9.0940313346754));
#26090=CARTESIAN_POINT('Ctrl Pts',(-25.0426484071616,35.1795219354007,11.1176436806954));
#26091=CARTESIAN_POINT('Ctrl Pts',(-26.5948091098001,37.1983760897494,13.1412560267153));
#26092=CARTESIAN_POINT('Ctrl Pts',(-28.4857991767897,39.7444590262842,13.8634749112255));
#26093=CARTESIAN_POINT('Ctrl Pts',(-30.3767892437793,42.2905419628191,14.5856937957357));
#26094=CARTESIAN_POINT('Ctrl Pts',(-32.2677793107688,44.8366248993539,13.8634749112255));
#26095=CARTESIAN_POINT('',(-21.4269965203139,31.138877952143,0.));
#26096=CARTESIAN_POINT('Ctrl Pts',(-21.4269965203139,31.138877952143,0.));
#26097=CARTESIAN_POINT('Ctrl Pts',(-21.6072651344921,31.0230263484025,3.24562220582793));
#26098=CARTESIAN_POINT('Ctrl Pts',(-22.5488764195076,32.0918470647273,6.16982677025167));
#26099=CARTESIAN_POINT('Ctrl Pts',(-23.334969330082,32.9841392463829,8.61106394926975));
#26100=CARTESIAN_POINT('Ctrl Pts',(-24.5639673341827,34.5610181206246,10.4489096280657));
#26101=CARTESIAN_POINT('Origin',(-35.1666259835201,19.5103534449754,0.));
#26102=CARTESIAN_POINT('Ctrl Pts',(-21.4269965203139,31.138877952143,0.));
#26103=CARTESIAN_POINT('Ctrl Pts',(-21.6072651344921,31.0230263484025,3.24562220582793));
#26104=CARTESIAN_POINT('Ctrl Pts',(-22.5488764195076,32.0918470647273,6.16982677025167));
#26105=CARTESIAN_POINT('Ctrl Pts',(-23.4904877045231,33.1606677810521,9.0940313346754));
#26106=CARTESIAN_POINT('Ctrl Pts',(-25.0426484071616,35.1795219354008,11.1176436806954));
#26107=CARTESIAN_POINT('Ctrl Pts',(-26.5948091098001,37.1983760897494,13.1412560267153));
#26108=CARTESIAN_POINT('Ctrl Pts',(-28.4857991767897,39.7444590262842,13.8634749112255));
#26109=CARTESIAN_POINT('Ctrl Pts',(-30.3767892437793,42.2905419628191,14.5856937957357));
#26110=CARTESIAN_POINT('Ctrl Pts',(-32.2677793107688,44.8366248993539,13.8634749112255));
#26111=CARTESIAN_POINT('Ctrl Pts',(-20.4854409432119,30.9950965373909,0.));
#26112=CARTESIAN_POINT('Ctrl Pts',(-20.6657095573901,30.8792449336504,3.38941559469373));
#26113=CARTESIAN_POINT('Ctrl Pts',(-21.6410512138984,32.0005511325097,6.44317352589574));
#26114=CARTESIAN_POINT('Ctrl Pts',(-22.6163928704067,33.1218573313691,9.49693145709775));
#26115=CARTESIAN_POINT('Ctrl Pts',(-24.2293336022808,35.2352870572786,11.6101975146502));
#26116=CARTESIAN_POINT('Ctrl Pts',(-25.8422743341549,37.3487167831881,13.7234635722027));
#26117=CARTESIAN_POINT('Ctrl Pts',(-27.8090558579146,40.0127335284694,14.4776794959001));
#26118=CARTESIAN_POINT('Ctrl Pts',(-29.7758373816743,42.6767502737506,15.2318954195974));
#26119=CARTESIAN_POINT('Ctrl Pts',(-31.742618905434,45.3407670190318,14.4776794959001));
#26120=CARTESIAN_POINT('Ctrl Pts',(-19.6841717937386,31.5100409519662,0.));
#26121=CARTESIAN_POINT('Ctrl Pts',(-19.8644404079168,31.3941893482258,3.38941559469373));
#26122=CARTESIAN_POINT('Ctrl Pts',(-20.8397820644251,32.5154955470851,6.44317352589574));
#26123=CARTESIAN_POINT('Ctrl Pts',(-21.8151237209334,33.6368017459444,9.49693145709774));
#26124=CARTESIAN_POINT('Ctrl Pts',(-23.4280644528075,35.7502314718539,11.6101975146502));
#26125=CARTESIAN_POINT('Ctrl Pts',(-25.0410051846816,37.8636611977635,13.7234635722027));
#26126=CARTESIAN_POINT('Ctrl Pts',(-27.0077867084413,40.5276779430447,14.4776794959001));
#26127=CARTESIAN_POINT('Ctrl Pts',(-28.974568232201,43.191694688326,15.2318954195974));
#26128=CARTESIAN_POINT('Ctrl Pts',(-30.9413497559607,45.8557114336071,14.4776794959001));
#26129=CARTESIAN_POINT('Ctrl Pts',(-19.4238236466307,32.4262389885814,0.));
#26130=CARTESIAN_POINT('Ctrl Pts',(-19.6040922608088,32.3103873848409,3.24562220582793));
#26131=CARTESIAN_POINT('Ctrl Pts',(-20.5457035458243,33.3792081011657,6.16982677025167));
#26132=CARTESIAN_POINT('Ctrl Pts',(-21.4873148308399,34.4480288174905,9.09403133467541));
#26133=CARTESIAN_POINT('Ctrl Pts',(-23.0394755334784,36.4668829718391,11.1176436806954));
#26134=CARTESIAN_POINT('Ctrl Pts',(-24.5916362361169,38.4857371261877,13.1412560267153));
#26135=CARTESIAN_POINT('Ctrl Pts',(-26.4826263031064,41.0318200627226,13.8634749112255));
#26136=CARTESIAN_POINT('Ctrl Pts',(-28.373616370096,43.5779029992574,14.5856937957357));
#26137=CARTESIAN_POINT('Ctrl Pts',(-30.2646064370856,46.1239859357923,13.8634749112255));
#26138=CARTESIAN_POINT('',(-20.1821175312213,31.4039970697443,-1.88545294716389E-29));
#26139=CARTESIAN_POINT('Origin',(-21.1552751870374,32.9182507396843,0.));
#26140=CARTESIAN_POINT('Origin',(-21.1552751870374,32.9182507396843,0.));
#26141=CARTESIAN_POINT('Ctrl Pts',(-14.6113821712781,34.8604849513724,0.));
#26142=CARTESIAN_POINT('Ctrl Pts',(-14.8063033131398,34.7714674485863,3.24562220582792));
#26143=CARTESIAN_POINT('Ctrl Pts',(-15.5862213055783,35.9634143688744,6.16982677025168));
#26144=CARTESIAN_POINT('Ctrl Pts',(-16.3661392980168,37.1553612891625,9.09403133467541));
#26145=CARTESIAN_POINT('Ctrl Pts',(-17.6151883402599,39.3745619185373,11.1176436806954));
#26146=CARTESIAN_POINT('Ctrl Pts',(-18.864237382503,41.5937625479121,13.1412560267153));
#26147=CARTESIAN_POINT('Ctrl Pts',(-20.3736345158498,44.3830459768615,13.8634749112255));
#26148=CARTESIAN_POINT('Ctrl Pts',(-21.8830316491966,47.1723294058109,14.5856937957357));
#26149=CARTESIAN_POINT('Ctrl Pts',(-23.3924287825434,49.9616128347603,13.8634749112255));
#26150=CARTESIAN_POINT('Ctrl Pts',(-15.3059217494163,37.1279962392257,0.));
#26151=CARTESIAN_POINT('Ctrl Pts',(-15.500842891278,37.0389787364396,2.70899372698069));
#26152=CARTESIAN_POINT('Ctrl Pts',(-16.1840379904938,38.0191320633214,5.14971273833323));
#26153=CARTESIAN_POINT('Ctrl Pts',(-16.8672330897096,38.9992853902031,7.59043174968578));
#26154=CARTESIAN_POINT('Ctrl Pts',(-17.9419935007385,40.8368471514173,9.27946171175752));
#26155=CARTESIAN_POINT('Ctrl Pts',(-19.0167539117674,42.6744089126315,10.9684916738293));
#26156=CARTESIAN_POINT('Ctrl Pts',(-20.3088166768303,44.9877964569988,11.5712994880388));
#26157=CARTESIAN_POINT('Ctrl Pts',(-21.6008794418932,47.3011840013661,12.1741073022483));
#26158=CARTESIAN_POINT('Ctrl Pts',(-22.8929422069561,49.6145715457333,11.5712994880388));
#26159=CARTESIAN_POINT('Ctrl Pts',(-15.5447398754877,39.4874365476045,0.));
#26160=CARTESIAN_POINT('Ctrl Pts',(-15.7396610173493,39.3984190448184,2.19648874705824));
#26161=CARTESIAN_POINT('Ctrl Pts',(-16.3304812866724,40.1762997089268,4.17545672685568));
#26162=CARTESIAN_POINT('Ctrl Pts',(-16.9213015559955,40.9541803730352,6.15442470665313));
#26163=CARTESIAN_POINT('Ctrl Pts',(-17.829608275202,42.4272593902765,7.5239130403414));
#26164=CARTESIAN_POINT('Ctrl Pts',(-18.7379149944086,43.9003384075177,8.89340137402968));
#26165=CARTESIAN_POINT('Ctrl Pts',(-19.8224134008055,45.7592234042437,9.3821661014496));
#26166=CARTESIAN_POINT('Ctrl Pts',(-20.9069118072024,47.6181084009697,9.87093082886953));
#26167=CARTESIAN_POINT('Ctrl Pts',(-21.9914102135993,49.4769933976957,9.3821661014496));
#26168=CARTESIAN_POINT('Ctrl Pts',(-15.3186586437005,41.8481313484579,0.));
#26169=CARTESIAN_POINT('Ctrl Pts',(-15.5135797855622,41.7591138456718,1.72780310113343));
#26170=CARTESIAN_POINT('Ctrl Pts',(-16.0199233014651,42.3520162221172,3.28449990511991));
#26171=CARTESIAN_POINT('Ctrl Pts',(-16.5262668173681,42.9449185985626,4.84119670910638));
#26172=CARTESIAN_POINT('Ctrl Pts',(-17.2823516867886,44.0846782589592,5.91846432228297));
#26173=CARTESIAN_POINT('Ctrl Pts',(-18.0384365562092,45.2244379193558,6.99573193545956));
#26174=CARTESIAN_POINT('Ctrl Pts',(-18.9331174206828,46.6676804765723,7.38020429521639));
#26175=CARTESIAN_POINT('Ctrl Pts',(-19.8277982851565,48.1109230337888,7.76467665497321));
#26176=CARTESIAN_POINT('Ctrl Pts',(-20.7224791496302,49.5541655910054,7.38020429521638));
#26177=CARTESIAN_POINT('',(-14.6113821712892,34.8604849513849,1.57949266918924E-9));
#26178=CARTESIAN_POINT('Origin',(2.5993596565155,40.1321417817282,0.));
#26179=CARTESIAN_POINT('Ctrl Pts',(-14.6113821714912,34.8604849513683,3.13106059869152E-9));
#26180=CARTESIAN_POINT('Ctrl Pts',(-14.626098337786,34.853764303467,0.245038153335648));
#26181=CARTESIAN_POINT('Ctrl Pts',(-14.6435771646297,34.8527495154069,0.490791160522061));
#26182=CARTESIAN_POINT('Ctrl Pts',(-14.6638259110835,34.8575316463561,0.736766500725887));
#26183=CARTESIAN_POINT('Ctrl Pts',(-14.6840081820399,34.8622980778379,0.981934317701575));
#26184=CARTESIAN_POINT('Ctrl Pts',(-14.7069422331333,34.8728235332129,1.22732257376626));
#26185=CARTESIAN_POINT('Ctrl Pts',(-14.7326128792078,34.8891527148322,1.47243294816407));
#26186=CARTESIAN_POINT('Ctrl Pts',(-14.7582448644192,34.9054573041506,1.71717417803084));
#26187=CARTESIAN_POINT('Ctrl Pts',(-14.7866052020689,34.9275482079566,1.96163791541655));
#26188=CARTESIAN_POINT('Ctrl Pts',(-14.8176563354397,34.9554233023889,2.20532408778594));
#26189=CARTESIAN_POINT('Ctrl Pts',(-14.8486808377692,34.9832744897134,2.44880126242133));
#26190=CARTESIAN_POINT('Ctrl Pts',(-14.882391488439,35.0168999484378,2.69150175431114));
#26191=CARTESIAN_POINT('Ctrl Pts',(-14.9187287035022,35.056250564147,2.9329295186687));
#26192=CARTESIAN_POINT('Ctrl Pts',(-14.9550583167476,35.0955929476289,3.17430677585636));
#26193=CARTESIAN_POINT('Ctrl Pts',(-14.9940133343939,35.1406580326361,3.41441139318375));
#26194=CARTESIAN_POINT('Ctrl Pts',(-15.0355127954201,35.1913501978217,3.65275710614652));
#26195=CARTESIAN_POINT('Ctrl Pts',(-15.0770649517991,35.2421067311088,3.89140546668806));
#26196=CARTESIAN_POINT('Ctrl Pts',(-15.1211679328244,35.2985045323754,4.12829002081184));
#26197=CARTESIAN_POINT('Ctrl Pts',(-15.1677200855872,35.3604022296524,4.3629387437783));
#26198=CARTESIAN_POINT('Ctrl Pts',(-15.2143197401098,35.422363087264,4.59782690201477));
#26199=CARTESIAN_POINT('Ctrl Pts',(-15.2633734552291,35.4898348974064,4.83047425894994));
#26200=CARTESIAN_POINT('Ctrl Pts',(-15.314760335032,35.5626325521734,5.06042975959473));
#26201=CARTESIAN_POINT('Ctrl Pts',(-15.3662974499284,35.6356430387471,5.2910575599835));
#26202=CARTESIAN_POINT('Ctrl Pts',(-15.4201812613939,35.714010340131,5.51897736305736));
#26203=CARTESIAN_POINT('Ctrl Pts',(-15.4762725955035,35.797507103918,5.74376259354382));
#26204=CARTESIAN_POINT('Ctrl Pts',(-15.5120380980665,35.8507471233724,5.88709234072653));
#26205=CARTESIAN_POINT('Ctrl Pts',(-15.5487007750603,35.9060718261752,6.0291482531421));
#26206=CARTESIAN_POINT('Ctrl Pts',(-15.5862213055882,35.9634143689083,6.16982677023484));
#26207=CARTESIAN_POINT('Ctrl Pts',(-15.6450546012012,36.0533291627655,6.39041482339101));
#26208=CARTESIAN_POINT('Ctrl Pts',(-15.7065142910193,36.1486520067523,6.60890054011825));
#26209=CARTESIAN_POINT('Ctrl Pts',(-15.7705155506318,36.2492721362564,6.82480412008071));
#26210=CARTESIAN_POINT('Ctrl Pts',(-15.8343723238085,36.3496651101705,7.04022028559322));
#26211=CARTESIAN_POINT('Ctrl Pts',(-15.9007591428904,36.4553314094027,7.25306552029667));
#26212=CARTESIAN_POINT('Ctrl Pts',(-15.9695695446608,36.5661159087968,7.46287566269448));
#26213=CARTESIAN_POINT('Ctrl Pts',(-16.038269271112,36.6767222213247,7.67234834441917));
#26214=CARTESIAN_POINT('Ctrl Pts',(-16.1093847013533,36.7924301575639,7.87879526533069));
#26215=CARTESIAN_POINT('Ctrl Pts',(-16.1827888425358,36.9130417770844,8.0817733461224));
#26216=CARTESIAN_POINT('Ctrl Pts',(-16.2561225498034,37.0335376654159,8.28455666214169));
#26217=CARTESIAN_POINT('Ctrl Pts',(-16.3317404631319,37.1589276519422,8.48387739272926));
#26218=CARTESIAN_POINT('Ctrl Pts',(-16.4094964608252,37.2889731283962,8.67931873611179));
#26219=CARTESIAN_POINT('Ctrl Pts',(-16.4872561983762,37.4190248596934,8.87476947970566));
#26220=CARTESIAN_POINT('Ctrl Pts',(-16.5671540886073,37.5537323016305,9.06634009532891));
#26221=CARTESIAN_POINT('Ctrl Pts',(-16.6490263722365,37.6928185909677,9.25364450341035));
#26222=CARTESIAN_POINT('Ctrl Pts',(-16.7309286899051,37.8319559027375,9.44101762226545));
#26223=CARTESIAN_POINT('Ctrl Pts',(-16.8148066908792,37.9754750005801,9.62412107875081));
#26224=CARTESIAN_POINT('Ctrl Pts',(-16.9004810321072,38.12306423662,9.80260437466171));
#26225=CARTESIAN_POINT('Ctrl Pts',(-16.9862951259314,38.2708942212739,9.98137881379724));
#26226=CARTESIAN_POINT('Ctrl Pts',(-17.0739112501825,38.4228073220822,10.1555177270929));
#26227=CARTESIAN_POINT('Ctrl Pts',(-17.163136239657,38.5784601754019,10.3247095747712));
#26228=CARTESIAN_POINT('Ctrl Pts',(-17.1889252818185,38.6234491187513,10.3736117457758));
#26229=CARTESIAN_POINT('Ctrl Pts',(-17.2148486564433,38.6687503076461,10.4221009095758));
#26230=CARTESIAN_POINT('Ctrl Pts',(-17.2409015314889,38.7143550419919,10.4701702229111));
#26231=CARTESIAN_POINT('Ctrl Pts',(-21.5951194116467,38.9817677587449,1.04083408558608E-14));
#26232=CARTESIAN_POINT('Ctrl Pts',(-21.7900405535084,38.8927502559588,1.72780310113342));
#26233=CARTESIAN_POINT('Ctrl Pts',(-22.2963840694113,39.4856526324042,3.28449990511991));
#26234=CARTESIAN_POINT('Ctrl Pts',(-22.8027275853143,40.0785550088496,4.84119670910639));
#26235=CARTESIAN_POINT('Ctrl Pts',(-23.5588124547348,41.2183146692462,5.91846432228298));
#26236=CARTESIAN_POINT('Ctrl Pts',(-24.3148973241554,42.3580743296428,6.99573193545956));
#26237=CARTESIAN_POINT('Ctrl Pts',(-25.209578188629,43.8013168868593,7.38020429521639));
#26238=CARTESIAN_POINT('Ctrl Pts',(-26.1042590531027,45.2445594440758,7.76467665497322));
#26239=CARTESIAN_POINT('Ctrl Pts',(-26.9989399175764,46.6878020012924,7.38020429521639));
#26240=CARTESIAN_POINT('Ctrl Pts',(-19.662973599342,37.6067022235299,0.));
#26241=CARTESIAN_POINT('Ctrl Pts',(-19.8578947412037,37.5176847207437,2.19648874705823));
#26242=CARTESIAN_POINT('Ctrl Pts',(-20.4487150105268,38.2955653848522,4.17545672685568));
#26243=CARTESIAN_POINT('Ctrl Pts',(-21.0395352798499,39.0734460489606,6.15442470665314));
#26244=CARTESIAN_POINT('Ctrl Pts',(-21.9478419990564,40.5465250662018,7.5239130403414));
#26245=CARTESIAN_POINT('Ctrl Pts',(-22.856148718263,42.019604083443,8.89340137402967));
#26246=CARTESIAN_POINT('Ctrl Pts',(-23.9406471246599,43.878489080169,9.38216610144961));
#26247=CARTESIAN_POINT('Ctrl Pts',(-25.0251455310568,45.737374076895,9.87093082886953));
#26248=CARTESIAN_POINT('Ctrl Pts',(-26.1096439374538,47.596259073621,9.3821661014496));
#26249=CARTESIAN_POINT('Ctrl Pts',(-18.0362202038891,35.8811107143583,0.));
#26250=CARTESIAN_POINT('Ctrl Pts',(-18.2311413457508,35.7920932115722,2.70899372698069));
#26251=CARTESIAN_POINT('Ctrl Pts',(-18.9143364449666,36.772246538454,5.14971273833323));
#26252=CARTESIAN_POINT('Ctrl Pts',(-19.5975315441824,37.7523998653357,7.59043174968577));
#26253=CARTESIAN_POINT('Ctrl Pts',(-20.6722919552113,39.5899616265499,9.27946171175751));
#26254=CARTESIAN_POINT('Ctrl Pts',(-21.7470523662402,41.4275233877641,10.9684916738293));
#26255=CARTESIAN_POINT('Ctrl Pts',(-23.0391151313031,43.7409109321314,11.5712994880388));
#26256=CARTESIAN_POINT('Ctrl Pts',(-24.331177896366,46.0542984764986,12.1741073022483));
#26257=CARTESIAN_POINT('Ctrl Pts',(-25.6232406614289,48.3676860208659,11.5712994880388));
#26258=CARTESIAN_POINT('Ctrl Pts',(-16.7773762111441,33.8713086176153,0.));
#26259=CARTESIAN_POINT('Ctrl Pts',(-16.9722973530057,33.7822911148292,3.24562220582792));
#26260=CARTESIAN_POINT('Ctrl Pts',(-17.7522153454443,34.9742380351173,6.16982677025168));
#26261=CARTESIAN_POINT('Ctrl Pts',(-18.5321333378828,36.1661849554054,9.09403133467541));
#26262=CARTESIAN_POINT('Ctrl Pts',(-19.7811823801259,38.3853855847802,11.1176436806954));
#26263=CARTESIAN_POINT('Ctrl Pts',(-21.030231422369,40.604586214155,13.1412560267153));
#26264=CARTESIAN_POINT('Ctrl Pts',(-22.5396285557158,43.3938696431044,13.8634749112255));
#26265=CARTESIAN_POINT('Ctrl Pts',(-24.0490256890626,46.1831530720538,14.5856937957357));
#26266=CARTESIAN_POINT('Ctrl Pts',(-25.5584228224094,48.9724365010032,13.8634749112255));
#26267=CARTESIAN_POINT('',(-16.7773762111441,33.8713086176153,0.));
#26268=CARTESIAN_POINT('Ctrl Pts',(-16.7773762111441,33.8713086176153,0.));
#26269=CARTESIAN_POINT('Ctrl Pts',(-16.9722973530058,33.7822911148292,3.24562220582792));
#26270=CARTESIAN_POINT('Ctrl Pts',(-17.7522153454443,34.9742380351173,6.16982677025168));
#26271=CARTESIAN_POINT('Ctrl Pts',(-18.4033205461166,35.9693206543789,8.61106394926976));
#26272=CARTESIAN_POINT('Ctrl Pts',(-19.3953958606401,37.7050538275442,10.4489096280657));
#26273=CARTESIAN_POINT('Origin',(-32.032067641919,24.3164988679739,0.));
#26274=CARTESIAN_POINT('Ctrl Pts',(-16.7773762111441,33.8713086176153,0.));
#26275=CARTESIAN_POINT('Ctrl Pts',(-16.9722973530058,33.7822911148292,3.24562220582792));
#26276=CARTESIAN_POINT('Ctrl Pts',(-17.7522153454443,34.9742380351173,6.16982677025167));
#26277=CARTESIAN_POINT('Ctrl Pts',(-18.5321333378828,36.1661849554054,9.09403133467541));
#26278=CARTESIAN_POINT('Ctrl Pts',(-19.7811823801259,38.3853855847802,11.1176436806954));
#26279=CARTESIAN_POINT('Ctrl Pts',(-21.030231422369,40.604586214155,13.1412560267153));
#26280=CARTESIAN_POINT('Ctrl Pts',(-22.5396285557158,43.3938696431044,13.8634749112255));
#26281=CARTESIAN_POINT('Ctrl Pts',(-24.0490256890626,46.1831530720538,14.5856937957357));
#26282=CARTESIAN_POINT('Ctrl Pts',(-25.5584228224094,48.9724365010032,13.8634749112255));
#26283=CARTESIAN_POINT('Ctrl Pts',(-15.8658665409931,33.5949933606691,6.24500451351651E-15));
#26284=CARTESIAN_POINT('Ctrl Pts',(-16.0607876828548,33.505975857883,3.38941559469373));
#26285=CARTESIAN_POINT('Ctrl Pts',(-16.8666232572809,34.7546743665351,6.44317352589573));
#26286=CARTESIAN_POINT('Ctrl Pts',(-17.672458831707,36.0033728751873,9.49693145709774));
#26287=CARTESIAN_POINT('Ctrl Pts',(-18.9682097429543,38.3248363332021,11.6101975146502));
#26288=CARTESIAN_POINT('Ctrl Pts',(-20.2639606542016,40.646299791217,13.7234635722027));
#26289=CARTESIAN_POINT('Ctrl Pts',(-21.8315940656522,43.5631028816989,14.4776794959001));
#26290=CARTESIAN_POINT('Ctrl Pts',(-23.3992274771028,46.4799059721809,15.2318954195974));
#26291=CARTESIAN_POINT('Ctrl Pts',(-24.9668608885534,49.3967090626629,14.4776794959001));
#26292=CARTESIAN_POINT('Ctrl Pts',(-14.9994689250467,33.9906638941719,0.));
#26293=CARTESIAN_POINT('Ctrl Pts',(-15.1943900669084,33.9016463913858,3.38941559469373));
#26294=CARTESIAN_POINT('Ctrl Pts',(-16.0002256413345,35.150344900038,6.44317352589574));
#26295=CARTESIAN_POINT('Ctrl Pts',(-16.8060612157606,36.3990434086901,9.49693145709774));
#26296=CARTESIAN_POINT('Ctrl Pts',(-18.1018121270079,38.7205068667049,11.6101975146502));
#26297=CARTESIAN_POINT('Ctrl Pts',(-19.3975630382553,41.0419703247198,13.7234635722027));
#26298=CARTESIAN_POINT('Ctrl Pts',(-20.9651964497058,43.9587734152018,14.4776794959001));
#26299=CARTESIAN_POINT('Ctrl Pts',(-22.5328298611564,46.8755765056838,15.2318954195974));
#26300=CARTESIAN_POINT('Ctrl Pts',(-24.100463272607,49.7923795961657,14.4776794959001));
#26301=CARTESIAN_POINT('Ctrl Pts',(-14.6113821712781,34.8604849513724,0.));
#26302=CARTESIAN_POINT('Ctrl Pts',(-14.8063033131398,34.7714674485863,3.24562220582792));
#26303=CARTESIAN_POINT('Ctrl Pts',(-15.5862213055783,35.9634143688743,6.16982677025168));
#26304=CARTESIAN_POINT('Ctrl Pts',(-16.3661392980168,37.1553612891625,9.09403133467541));
#26305=CARTESIAN_POINT('Ctrl Pts',(-17.6151883402599,39.3745619185373,11.1176436806954));
#26306=CARTESIAN_POINT('Ctrl Pts',(-18.864237382503,41.5937625479121,13.1412560267153));
#26307=CARTESIAN_POINT('Ctrl Pts',(-20.3736345158498,44.3830459768615,13.8634749112255));
#26308=CARTESIAN_POINT('Ctrl Pts',(-21.8830316491966,47.1723294058109,14.5856937957357));
#26309=CARTESIAN_POINT('Ctrl Pts',(-23.3924287825434,49.9616128347603,13.8634749112255));
#26310=CARTESIAN_POINT('',(-15.507437910779,33.9565644528989,-1.82251475137849E-29));
#26311=CARTESIAN_POINT('Origin',(-16.2551894587636,35.5938999782225,0.));
#26312=CARTESIAN_POINT('Origin',(-16.2551894587636,35.5938999782225,0.));
#26313=CARTESIAN_POINT('Ctrl Pts',(-9.50149509066497,36.5850719698906,0.));
#26314=CARTESIAN_POINT('Ctrl Pts',(-9.70710072786806,36.5247007077103,3.24562220582793));
#26315=CARTESIAN_POINT('Ctrl Pts',(-10.3094485465013,37.8155092299557,6.16982677025168));
#26316=CARTESIAN_POINT('Ctrl Pts',(-10.9117963651345,39.1063177522011,9.09403133467541));
#26317=CARTESIAN_POINT('Ctrl Pts',(-11.8323067104422,41.4806883314342,11.1176436806954));
#26318=CARTESIAN_POINT('Ctrl Pts',(-12.7528170557497,43.8550589106673,13.1412560267153));
#26319=CARTESIAN_POINT('Ctrl Pts',(-13.8498942825608,46.830761065047,13.8634749112255));
#26320=CARTESIAN_POINT('Ctrl Pts',(-14.9469715093718,49.8064632194267,14.5856937957357));
#26321=CARTESIAN_POINT('Ctrl Pts',(-16.0440487361828,52.7821653738064,13.8634749112255));
#26322=CARTESIAN_POINT('Ctrl Pts',(-9.86626475512738,38.928346550052,0.));
#26323=CARTESIAN_POINT('Ctrl Pts',(-10.0718703923305,38.8679752878717,2.7089937269807));
#26324=CARTESIAN_POINT('Ctrl Pts',(-10.6086211883241,39.9353808672042,5.14971273833323));
#26325=CARTESIAN_POINT('Ctrl Pts',(-11.1453719843177,41.0027864465367,7.59043174968578));
#26326=CARTESIAN_POINT('Ctrl Pts',(-11.9476805791745,42.9745988326451,9.27946171175752));
#26327=CARTESIAN_POINT('Ctrl Pts',(-12.7499891740313,44.9464112187535,10.9684916738293));
#26328=CARTESIAN_POINT('Ctrl Pts',(-13.6996712289065,47.4201315169974,11.5712994880388));
#26329=CARTESIAN_POINT('Ctrl Pts',(-14.6493532837816,49.8938518152412,12.1741073022483));
#26330=CARTESIAN_POINT('Ctrl Pts',(-15.5990353386568,52.3675721134851,11.5712994880388));
#26331=CARTESIAN_POINT('Ctrl Pts',(-9.76686869112026,41.297758521112,0.));
#26332=CARTESIAN_POINT('Ctrl Pts',(-9.97247432832337,41.2373872589318,2.19648874705823));
#26333=CARTESIAN_POINT('Ctrl Pts',(-10.4465769382887,42.0914327105681,4.17545672685568));
#26334=CARTESIAN_POINT('Ctrl Pts',(-10.920679548254,42.9454781622045,6.15442470665314));
#26335=CARTESIAN_POINT('Ctrl Pts',(-11.6101000126267,44.5328288829012,7.5239130403414));
#26336=CARTESIAN_POINT('Ctrl Pts',(-12.2995204769994,46.1201796035979,8.89340137402967));
#26337=CARTESIAN_POINT('Ctrl Pts',(-13.1084333356591,48.114484046662,9.38216610144961));
#26338=CARTESIAN_POINT('Ctrl Pts',(-13.9173461943188,50.1087884897262,9.87093082886954));
#26339=CARTESIAN_POINT('Ctrl Pts',(-14.7262590529785,52.1030929327904,9.3821661014496));
#26340=CARTESIAN_POINT('Ctrl Pts',(-9.20712674149444,43.6022501387952,0.));
#26341=CARTESIAN_POINT('Ctrl Pts',(-9.41273237869755,43.5418788766149,1.72780310113343));
#26342=CARTESIAN_POINT('Ctrl Pts',(-9.82954324187999,44.2008065573391,3.28449990511991));
#26343=CARTESIAN_POINT('Ctrl Pts',(-10.2463541050624,44.8597342380634,4.84119670910639));
#26344=CARTESIAN_POINT('Ctrl Pts',(-10.8325384089569,46.0954948844273,5.91846432228299));
#26345=CARTESIAN_POINT('Ctrl Pts',(-11.4187227128513,47.3312555307913,6.99573193545957));
#26346=CARTESIAN_POINT('Ctrl Pts',(-12.0989021850286,48.887134322293,7.3802042952164));
#26347=CARTESIAN_POINT('Ctrl Pts',(-12.7790816572058,50.4430131137948,7.76467665497322));
#26348=CARTESIAN_POINT('Ctrl Pts',(-13.459261129383,51.9988919052966,7.38020429521639));
#26349=CARTESIAN_POINT('',(-9.50149509067415,36.5850719699045,1.57949201998838E-9));
#26350=CARTESIAN_POINT('Origin',(8.2843011904065,39.3537269950291,0.));
#26351=CARTESIAN_POINT('Ctrl Pts',(-9.50149509087647,36.5850719699169,3.13105443220166E-9));
#26352=CARTESIAN_POINT('Ctrl Pts',(-9.51701791573658,36.5805140573471,0.24503815333567));
#26353=CARTESIAN_POINT('Ctrl Pts',(-9.53446325272403,36.5819970947817,0.49079116052211));
#26354=CARTESIAN_POINT('Ctrl Pts',(-9.55382532794258,36.5896122476099,0.736766500725963));
#26355=CARTESIAN_POINT('Ctrl Pts',(-9.57312383855555,36.597202400319,0.981934317701606));
#26356=CARTESIAN_POINT('Ctrl Pts',(-9.59432652559756,36.6108845775071,1.22732257376625));
#26357=CARTESIAN_POINT('Ctrl Pts',(-9.6174119966677,36.6307008654467,1.47243294816401));
#26358=CARTESIAN_POINT('Ctrl Pts',(-9.64046270023601,36.650487309385,1.71717417803076));
#26359=CARTESIAN_POINT('Ctrl Pts',(-9.6653905071382,36.6763894565088,1.96163791541645));
#26360=CARTESIAN_POINT('Ctrl Pts',(-9.69215854518732,36.7083998596961,2.20532408778582));
#26361=CARTESIAN_POINT('Ctrl Pts',(-9.71890362559695,36.7403828091233,2.44880126242125));
#26362=CARTESIAN_POINT('Ctrl Pts',(-9.74748574872948,36.77846353496,2.6915017543111));
#26363=CARTESIAN_POINT('Ctrl Pts',(-9.77785292682669,36.8225849430252,2.9329295186687));
#26364=CARTESIAN_POINT('Ctrl Pts',(-9.80821375204967,36.8666971208038,3.17430677585648));
#26365=CARTESIAN_POINT('Ctrl Pts',(-9.84035883350025,36.9168473852605,3.41441139318398));
#26366=CARTESIAN_POINT('Ctrl Pts',(-9.87422164256049,36.9729295663809,3.65275710614687));
#26367=CARTESIAN_POINT('Ctrl Pts',(-9.9081274500747,37.029082959759,3.89140546668844));
#26368=CARTESIAN_POINT('Ctrl Pts',(-9.94375528237817,37.0911832213397,4.12829002081224));
#26369=CARTESIAN_POINT('Ctrl Pts',(-9.98102464057106,37.1590759513992,4.36293874377873));
#26370=CARTESIAN_POINT('Ctrl Pts',(-10.0183320283715,37.2270379591174,4.59782690201505));
#26371=CARTESIAN_POINT('Ctrl Pts',(-10.0572842076521,37.3008040750528,4.83047425895008));
#26372=CARTESIAN_POINT('Ctrl Pts',(-10.0977878566475,37.3801738701483,5.06042975959472));
#26373=CARTESIAN_POINT('Ctrl Pts',(-10.1384099224356,37.4597757114126,5.29105755998346));
#26374=CARTESIAN_POINT('Ctrl Pts',(-10.1805924445721,37.5450138125791,5.5189773630573));
#26375=CARTESIAN_POINT('Ctrl Pts',(-10.2242300213428,37.6356433288454,5.74376259354374));
#26376=CARTESIAN_POINT('Ctrl Pts',(-10.2520546379009,37.6934314033806,5.88709234072648));
#26377=CARTESIAN_POINT('Ctrl Pts',(-10.2804706155743,37.7534106234275,6.02914825314207));
#26378=CARTESIAN_POINT('Ctrl Pts',(-10.3094485465063,37.8155092299907,6.16982677023484));
#26379=CARTESIAN_POINT('Ctrl Pts',(-10.3548867946544,37.912881671843,6.39041482339094));
#26380=CARTESIAN_POINT('Ctrl Pts',(-10.4021550583219,38.015980892539,6.60890054011811));
#26381=CARTESIAN_POINT('Ctrl Pts',(-10.4511851399364,38.124685183118,6.8248041200805));
#26382=CARTESIAN_POINT('Ctrl Pts',(-10.5001045333897,38.2331440676597,7.04022028559304));
#26383=CARTESIAN_POINT('Ctrl Pts',(-10.550777748089,38.3471826657451,7.25306552029652));
#26384=CARTESIAN_POINT('Ctrl Pts',(-10.6031214810714,38.4666322798728,7.46287566269435));
#26385=CARTESIAN_POINT('Ctrl Pts',(-10.6553810238846,38.5858897700797,7.672348344419));
#26386=CARTESIAN_POINT('Ctrl Pts',(-10.7093056453533,38.7105407473185,7.87879526533047));
#26387=CARTESIAN_POINT('Ctrl Pts',(-10.7647978150926,38.8403712129408,8.08177334612214));
#26388=CARTESIAN_POINT('Ctrl Pts',(-10.8202367380982,38.9700771015595,8.28455666214125));
#26389=CARTESIAN_POINT('Ctrl Pts',(-10.8772401144473,39.1049523499262,8.48387739272865));
#26390=CARTESIAN_POINT('Ctrl Pts',(-10.9356972672492,39.2447399831763,8.67931873611101));
#26391=CARTESIAN_POINT('Ctrl Pts',(-10.9941572316855,39.3845343398417,8.87476947970485));
#26392=CARTESIAN_POINT('Ctrl Pts',(-11.0540710087838,39.5292413095786,9.06634009532808));
#26393=CARTESIAN_POINT('Ctrl Pts',(-11.1153159078427,39.6785635418399,9.25364450340949));
#26394=CARTESIAN_POINT('Ctrl Pts',(-11.1765832739884,39.8279405514883,9.4410176222643));
#26395=CARTESIAN_POINT('Ctrl Pts',(-11.2391826206559,39.9819359159954,9.62412107874938));
#26396=CARTESIAN_POINT('Ctrl Pts',(-11.3029807823645,40.1402156364342,9.80260437466002));
#26397=CARTESIAN_POINT('Ctrl Pts',(-11.3668830120893,40.2987535438817,9.98137881379555));
#26398=CARTESIAN_POINT('Ctrl Pts',(-11.4319878421544,40.4615894629173,10.1555177270912));
#26399=CARTESIAN_POINT('Ctrl Pts',(-11.4981529392408,40.62835603457,10.3247095747696));
#26400=CARTESIAN_POINT('Ctrl Pts',(-11.5172768919406,40.6765572187082,10.373611745773));
#26401=CARTESIAN_POINT('Ctrl Pts',(-11.5364893726185,40.725086587685,10.422100909572));
#26402=CARTESIAN_POINT('Ctrl Pts',(-11.5557868365679,40.7739348422893,10.4701702229062));
#26403=CARTESIAN_POINT('Ctrl Pts',(-15.8276282594345,41.6582954965894,0.));
#26404=CARTESIAN_POINT('Ctrl Pts',(-16.0332338966376,41.597924234409,1.72780310113343));
#26405=CARTESIAN_POINT('Ctrl Pts',(-16.45004475982,42.2568519151333,3.28449990511991));
#26406=CARTESIAN_POINT('Ctrl Pts',(-16.8668556230025,42.9157795958576,4.84119670910639));
#26407=CARTESIAN_POINT('Ctrl Pts',(-17.4530399268969,44.1515402422215,5.91846432228299));
#26408=CARTESIAN_POINT('Ctrl Pts',(-18.0392242307914,45.3873008885855,6.99573193545956));
#26409=CARTESIAN_POINT('Ctrl Pts',(-18.7194037029686,46.9431796800872,7.38020429521639));
#26410=CARTESIAN_POINT('Ctrl Pts',(-19.3995831751458,48.499058471589,7.76467665497322));
#26411=CARTESIAN_POINT('Ctrl Pts',(-20.079762647323,50.0549372630908,7.38020429521639));
#26412=CARTESIAN_POINT('Ctrl Pts',(-14.1108411348342,40.0222531270434,0.));
#26413=CARTESIAN_POINT('Ctrl Pts',(-14.3164467720373,39.9618818648631,2.19648874705823));
#26414=CARTESIAN_POINT('Ctrl Pts',(-14.7905493820026,40.8159273164995,4.17545672685568));
#26415=CARTESIAN_POINT('Ctrl Pts',(-15.264651991968,41.6699727681359,6.15442470665314));
#26416=CARTESIAN_POINT('Ctrl Pts',(-15.9540724563407,43.2573234888326,7.52391304034139));
#26417=CARTESIAN_POINT('Ctrl Pts',(-16.6434929207134,44.8446742095293,8.89340137402967));
#26418=CARTESIAN_POINT('Ctrl Pts',(-17.4524057793731,46.8389786525934,9.38216610144961));
#26419=CARTESIAN_POINT('Ctrl Pts',(-18.2613186380328,48.8332830956576,9.87093082886954));
#26420=CARTESIAN_POINT('Ctrl Pts',(-19.0702314966925,50.8275875387218,9.3821661014496));
#26421=CARTESIAN_POINT('Ctrl Pts',(-12.7462230199157,38.0827145049534,0.));
#26422=CARTESIAN_POINT('Ctrl Pts',(-12.9518286571189,38.0223432427731,2.70899372698069));
#26423=CARTESIAN_POINT('Ctrl Pts',(-13.4885794531125,39.0897488221056,5.14971273833323));
#26424=CARTESIAN_POINT('Ctrl Pts',(-14.0253302491061,40.1571544014381,7.59043174968578));
#26425=CARTESIAN_POINT('Ctrl Pts',(-14.8276388439629,42.1289667875465,9.27946171175752));
#26426=CARTESIAN_POINT('Ctrl Pts',(-15.6299474388197,44.1007791736549,10.9684916738293));
#26427=CARTESIAN_POINT('Ctrl Pts',(-16.5796294936948,46.5744994718987,11.5712994880388));
#26428=CARTESIAN_POINT('Ctrl Pts',(-17.52931154857,49.0482197701426,12.1741073022483));
#26429=CARTESIAN_POINT('Ctrl Pts',(-18.4789936034451,51.5219400683864,11.5712994880388));
#26430=CARTESIAN_POINT('Ctrl Pts',(-11.786216904273,35.9142171164211,0.));
#26431=CARTESIAN_POINT('Ctrl Pts',(-11.9918225414761,35.8538458542408,3.24562220582793));
#26432=CARTESIAN_POINT('Ctrl Pts',(-12.5941703601094,37.1446543764862,6.16982677025168));
#26433=CARTESIAN_POINT('Ctrl Pts',(-13.1965181787426,38.4354628987316,9.09403133467541));
#26434=CARTESIAN_POINT('Ctrl Pts',(-14.1170285240502,40.8098334779647,11.1176436806954));
#26435=CARTESIAN_POINT('Ctrl Pts',(-15.0375388693578,43.1842040571978,13.1412560267153));
#26436=CARTESIAN_POINT('Ctrl Pts',(-16.1346160961688,46.1599062115775,13.8634749112255));
#26437=CARTESIAN_POINT('Ctrl Pts',(-17.2316933229798,49.1356083659572,14.5856937957357));
#26438=CARTESIAN_POINT('Ctrl Pts',(-18.3287705497908,52.1113105203369,13.8634749112255));
#26439=CARTESIAN_POINT('',(-11.786216904273,35.9142171164211,0.));
#26440=CARTESIAN_POINT('Ctrl Pts',(-11.786216904273,35.9142171164211,0.));
#26441=CARTESIAN_POINT('Ctrl Pts',(-11.9918225414761,35.8538458542408,3.24562220582793));
#26442=CARTESIAN_POINT('Ctrl Pts',(-12.5941703601094,37.1446543764862,6.16982677025168));
#26443=CARTESIAN_POINT('Ctrl Pts',(-13.0970332266263,38.2222704208069,8.61106394926976));
#26444=CARTESIAN_POINT('Ctrl Pts',(-13.8319900590778,40.0815233709313,10.4489096280657));
#26445=CARTESIAN_POINT('Origin',(-28.2454287759836,28.6276304970127,1.04083408558608E-14));
#26446=CARTESIAN_POINT('Ctrl Pts',(-11.786216904273,35.9142171164211,0.));
#26447=CARTESIAN_POINT('Ctrl Pts',(-11.9918225414761,35.8538458542408,3.24562220582793));
#26448=CARTESIAN_POINT('Ctrl Pts',(-12.5941703601094,37.1446543764862,6.16982677025168));
#26449=CARTESIAN_POINT('Ctrl Pts',(-13.1965181787426,38.4354628987316,9.09403133467541));
#26450=CARTESIAN_POINT('Ctrl Pts',(-14.1170285240502,40.8098334779647,11.1176436806954));
#26451=CARTESIAN_POINT('Ctrl Pts',(-15.0375388693578,43.1842040571978,13.1412560267153));
#26452=CARTESIAN_POINT('Ctrl Pts',(-16.1346160961688,46.1599062115775,13.8634749112255));
#26453=CARTESIAN_POINT('Ctrl Pts',(-17.2316933229798,49.1356083659571,14.5856937957357));
#26454=CARTESIAN_POINT('Ctrl Pts',(-18.3287705497908,52.1113105203369,13.8634749112255));
#26455=CARTESIAN_POINT('Ctrl Pts',(-10.9233088493805,35.5109929990848,6.24500451351651E-15));
#26456=CARTESIAN_POINT('Ctrl Pts',(-11.1289144865836,35.4506217369045,3.38941559469372));
#26457=CARTESIAN_POINT('Ctrl Pts',(-11.7488394904701,36.8012926546625,6.44317352589573));
#26458=CARTESIAN_POINT('Ctrl Pts',(-12.3687644943566,38.1519635724204,9.49693145709774));
#26459=CARTESIAN_POINT('Ctrl Pts',(-13.3209478330612,40.6342024610832,11.6101975146502));
#26460=CARTESIAN_POINT('Ctrl Pts',(-14.2731311717658,43.116441349746,13.7234635722027));
#26461=CARTESIAN_POINT('Ctrl Pts',(-15.4097039753316,46.226653085872,14.4776794959001));
#26462=CARTESIAN_POINT('Ctrl Pts',(-16.5462767788974,49.336864821998,15.2318954195974));
#26463=CARTESIAN_POINT('Ctrl Pts',(-17.6828495824632,52.447076558124,14.4776794959001));
#26464=CARTESIAN_POINT('Ctrl Pts',(-10.0094201239373,35.7793349404726,6.24500451351651E-15));
#26465=CARTESIAN_POINT('Ctrl Pts',(-10.2150257611404,35.7189636782923,3.38941559469372));
#26466=CARTESIAN_POINT('Ctrl Pts',(-10.8349507650269,37.0696345960502,6.44317352589573));
#26467=CARTESIAN_POINT('Ctrl Pts',(-11.4548757689134,38.4203055138082,9.49693145709774));
#26468=CARTESIAN_POINT('Ctrl Pts',(-12.407059107618,40.902544402471,11.6101975146502));
#26469=CARTESIAN_POINT('Ctrl Pts',(-13.3592424463226,43.3847832911338,13.7234635722027));
#26470=CARTESIAN_POINT('Ctrl Pts',(-14.4958152498884,46.4949950272598,14.4776794959001));
#26471=CARTESIAN_POINT('Ctrl Pts',(-15.6323880534542,49.6052067633858,15.2318954195974));
#26472=CARTESIAN_POINT('Ctrl Pts',(-16.7689608570199,52.7154184995118,14.4776794959001));
#26473=CARTESIAN_POINT('Ctrl Pts',(-9.50149509066497,36.5850719698906,0.));
#26474=CARTESIAN_POINT('Ctrl Pts',(-9.70710072786808,36.5247007077103,3.24562220582793));
#26475=CARTESIAN_POINT('Ctrl Pts',(-10.3094485465013,37.8155092299557,6.16982677025168));
#26476=CARTESIAN_POINT('Ctrl Pts',(-10.9117963651345,39.1063177522011,9.09403133467541));
#26477=CARTESIAN_POINT('Ctrl Pts',(-11.8323067104422,41.4806883314342,11.1176436806954));
#26478=CARTESIAN_POINT('Ctrl Pts',(-12.7528170557497,43.8550589106673,13.1412560267153));
#26479=CARTESIAN_POINT('Ctrl Pts',(-13.8498942825608,46.830761065047,13.8634749112255));
#26480=CARTESIAN_POINT('Ctrl Pts',(-14.9469715093718,49.8064632194267,14.5856937957357));
#26481=CARTESIAN_POINT('Ctrl Pts',(-16.0440487361828,52.7821653738064,13.8634749112255));
#26482=CARTESIAN_POINT('',(-10.5170715742812,35.817874106401,1.04083408558608E-14));
#26483=CARTESIAN_POINT('Origin',(-11.0241949492049,37.5449600575354,1.04083408558608E-14));
#26484=CARTESIAN_POINT('Origin',(-11.0241949492049,37.5449600575354,1.04083408558608E-14));
#26485=CARTESIAN_POINT('Ctrl Pts',(-4.19818497005511,37.5648924257372,0.));
#26486=CARTESIAN_POINT('Ctrl Pts',(-4.41028956474387,37.5343963889644,3.24562220582793));
#26487=CARTESIAN_POINT('Ctrl Pts',(-4.82280514501214,38.8977893740386,6.16982677025167));
#26488=CARTESIAN_POINT('Ctrl Pts',(-5.23532072528038,40.2611823591128,9.09403133467542));
#26489=CARTESIAN_POINT('Ctrl Pts',(-5.80855343755468,42.7423875503303,11.1176436806954));
#26490=CARTESIAN_POINT('Ctrl Pts',(-6.38178614982895,45.2235927415478,13.1412560267153));
#26491=CARTESIAN_POINT('Ctrl Pts',(-7.04421014147575,48.325136906711,13.8634749112255));
#26492=CARTESIAN_POINT('Ctrl Pts',(-7.70663413312253,51.4266810718742,14.5856937957357));
#26493=CARTESIAN_POINT('Ctrl Pts',(-8.36905812476932,54.5282252370374,13.8634749112255));
#26494=CARTESIAN_POINT('Ctrl Pts',(-4.22575906238214,39.9362279852005,0.));
#26495=CARTESIAN_POINT('Ctrl Pts',(-4.43786365707092,39.9057319484276,2.70899372698069));
#26496=CARTESIAN_POINT('Ctrl Pts',(-4.81724345149735,41.0386604807592,5.14971273833323));
#26497=CARTESIAN_POINT('Ctrl Pts',(-5.19662324592377,42.1715890130907,7.59043174968577));
#26498=CARTESIAN_POINT('Ctrl Pts',(-5.71014733528412,44.2375116101495,9.27946171175751));
#26499=CARTESIAN_POINT('Ctrl Pts',(-6.22367142464447,46.3034342072084,10.9684916738293));
#26500=CARTESIAN_POINT('Ctrl Pts',(-6.81163998135152,48.8871294476768,11.5712994880388));
#26501=CARTESIAN_POINT('Ctrl Pts',(-7.39960853805857,51.4708246881453,12.1741073022483));
#26502=CARTESIAN_POINT('Ctrl Pts',(-7.98757709476562,54.0545199286138,11.5712994880388));
#26503=CARTESIAN_POINT('Ctrl Pts',(-3.79017222552514,42.2673772240309,0.));
#26504=CARTESIAN_POINT('Ctrl Pts',(-4.00227682021391,42.2368811872581,2.19648874705823));
#26505=CARTESIAN_POINT('Ctrl Pts',(-4.35001040888163,43.1497055238908,4.17545672685568));
#26506=CARTESIAN_POINT('Ctrl Pts',(-4.69774399754935,44.0625298605236,6.15442470665314));
#26507=CARTESIAN_POINT('Ctrl Pts',(-5.15424359455804,45.7318384015438,7.5239130403414));
#26508=CARTESIAN_POINT('Ctrl Pts',(-5.61074319156672,47.401146942564,8.89340137402968));
#26509=CARTESIAN_POINT('Ctrl Pts',(-6.12760336939892,49.4902725446046,9.38216610144961));
#26510=CARTESIAN_POINT('Ctrl Pts',(-6.64446354723112,51.5793981466453,9.87093082886954));
#26511=CARTESIAN_POINT('Ctrl Pts',(-7.1613237250633,53.668523748686,9.38216610144961));
#26512=CARTESIAN_POINT('Ctrl Pts',(-2.90816428999254,44.4687528548128,0.));
#26513=CARTESIAN_POINT('Ctrl Pts',(-3.12026888468131,44.4382568180399,1.72780310113343));
#26514=CARTESIAN_POINT('Ctrl Pts',(-3.43906202795212,45.149795935654,3.28449990511991));
#26515=CARTESIAN_POINT('Ctrl Pts',(-3.75785517122293,45.8613350532681,4.84119670910639));
#26516=CARTESIAN_POINT('Ctrl Pts',(-4.16220588757996,47.1679401624789,5.91846432228298));
#26517=CARTESIAN_POINT('Ctrl Pts',(-4.56655660393696,48.4745452716896,6.99573193545957));
#26518=CARTESIAN_POINT('Ctrl Pts',(-5.0183881912398,50.1113870920656,7.3802042952164));
#26519=CARTESIAN_POINT('Ctrl Pts',(-5.47021977854266,51.7482289124415,7.76467665497322));
#26520=CARTESIAN_POINT('Ctrl Pts',(-5.9220513658455,53.3850707328175,7.38020429521639));
#26521=CARTESIAN_POINT('',(-4.19818497005564,37.5648924257619,1.57948538796959E-9));
#26522=CARTESIAN_POINT('Origin',(13.8005982420127,37.7741838134884,0.));
#26523=CARTESIAN_POINT('Ctrl Pts',(-4.19818497026072,37.5648924257933,3.13104705197686E-9));
#26524=CARTESIAN_POINT('Ctrl Pts',(-4.21419845373604,37.562590034511,0.245038153335374));
#26525=CARTESIAN_POINT('Ctrl Pts',(-4.23125516411437,37.5665407070749,0.490791160521525));
#26526=CARTESIAN_POINT('Ctrl Pts',(-4.24933641208181,37.5768338592308,0.736766500725089));
#26527=CARTESIAN_POINT('Ctrl Pts',(-4.26735830032762,37.5870932195462,0.981934317700738));
#26528=CARTESIAN_POINT('Ctrl Pts',(-4.28639799775355,37.6036535888759,1.22732257376539));
#26529=CARTESIAN_POINT('Ctrl Pts',(-4.30642834020139,37.6265535806588,1.47243294816316));
#26530=CARTESIAN_POINT('Ctrl Pts',(-4.32642851627465,37.649419084278,1.71717417802993));
#26531=CARTESIAN_POINT('Ctrl Pts',(-4.34741633416666,37.6786051816996,1.96163791541563));
#26532=CARTESIAN_POINT('Ctrl Pts',(-4.3693563568321,37.7140992541435,2.20532408778503));
#26533=CARTESIAN_POINT('Ctrl Pts',(-4.39127756261114,37.7495628850543,2.44880126242043));
#26534=CARTESIAN_POINT('Ctrl Pts',(-4.41414930860342,37.7913236642408,2.69150175431026));
#26535=CARTESIAN_POINT('Ctrl Pts',(-4.43792826156026,37.8393176800295,2.93292951866782));
#26536=CARTESIAN_POINT('Ctrl Pts',(-4.46170223991271,37.8873016553743,3.17430677585565));
#26537=CARTESIAN_POINT('Ctrl Pts',(-4.48638300400801,37.9415161845174,3.4144113931832));
#26538=CARTESIAN_POINT('Ctrl Pts',(-4.51191981196198,38.0018467100927,3.65275710614614));
#26539=CARTESIAN_POINT('Ctrl Pts',(-4.53748904614673,38.0622538424056,3.89140546668764));
#26540=CARTESIAN_POINT('Ctrl Pts',(-4.56391644980485,38.1287923820568,4.1282900208114));
#26541=CARTESIAN_POINT('Ctrl Pts',(-4.59114431677095,38.2012980447013,4.36293874377783));
#26542=CARTESIAN_POINT('Ctrl Pts',(-4.61839996701919,38.2738776920353,4.59782690201414));
#26543=CARTESIAN_POINT('Ctrl Pts',(-4.64645765641973,38.3524364483671,4.83047425894916));
#26544=CARTESIAN_POINT('Ctrl Pts',(-4.67525353711703,38.4367626436465,5.06042975959379));
#26545=CARTESIAN_POINT('Ctrl Pts',(-4.70413360568184,38.5213353756661,5.29105755998255));
#26546=CARTESIAN_POINT('Ctrl Pts',(-4.73375612398288,38.6117090746817,5.5189773630564));
#26547=CARTESIAN_POINT('Ctrl Pts',(-4.76405160819203,38.7076263878302,5.74376259354286));
#26548=CARTESIAN_POINT('Ctrl Pts',(-4.78336890979181,38.7687861188957,5.88709234072589));
#26549=CARTESIAN_POINT('Ctrl Pts',(-4.80295972078426,38.8321988522325,6.02914825314178));
#26550=CARTESIAN_POINT('Ctrl Pts',(-4.82280514501204,38.8977893740739,6.16982677023483));
#26551=CARTESIAN_POINT('Ctrl Pts',(-4.85392335399607,39.0006372418043,6.39041482339097));
#26552=CARTESIAN_POINT('Ctrl Pts',(-4.88603794597525,39.1094140363897,6.60890054011818));
#26553=CARTESIAN_POINT('Ctrl Pts',(-4.91909873852106,39.2239895821647,6.82480412008061));
#26554=CARTESIAN_POINT('Ctrl Pts',(-4.95208489447207,39.3383064672143,7.04022028559306));
#26555=CARTESIAN_POINT('Ctrl Pts',(-4.986012944267,39.458395867156,7.25306552029644));
#26556=CARTESIAN_POINT('Ctrl Pts',(-5.02082444100466,39.5840789463379,7.46287566269419));
#26557=CARTESIAN_POINT('Ctrl Pts',(-5.05557994659247,39.7095598756332,7.67234834441872));
#26558=CARTESIAN_POINT('Ctrl Pts',(-5.09121600950109,39.8406163594388,7.87879526533008));
#26559=CARTESIAN_POINT('Ctrl Pts',(-5.12766654724752,39.9770226972829,8.08177334612164));
#26560=CARTESIAN_POINT('Ctrl Pts',(-5.16408210939133,40.1132981483374,8.2845566621406));
#26561=CARTESIAN_POINT('Ctrl Pts',(-5.20131052440292,40.2549129874358,8.48387739272784));
#26562=CARTESIAN_POINT('Ctrl Pts',(-5.23927881325894,40.4015971043833,8.67931873611006));
#26563=CARTESIAN_POINT('Ctrl Pts',(-5.27724892828921,40.5482882764489,8.87476947970389));
#26564=CARTESIAN_POINT('Ctrl Pts',(-5.31595892053002,40.700048957382,9.0663400953271));
#26565=CARTESIAN_POINT('Ctrl Pts',(-5.3553296654895,40.8565673625284,9.25364450340851));
#26566=CARTESIAN_POINT('Ctrl Pts',(-5.39471485321827,41.0131431849073,9.44101762226374));
#26567=CARTESIAN_POINT('Ctrl Pts',(-5.434761203403,41.174479914544,9.62412107874923));
#26568=CARTESIAN_POINT('Ctrl Pts',(-5.47538443899858,41.3402280007153,9.80260437466025));
#26569=CARTESIAN_POINT('Ctrl Pts',(-5.51607393950566,41.5062464563465,9.98137881379592));
#26570=CARTESIAN_POINT('Ctrl Pts',(-5.55734212879153,41.6766903238779,10.1555177270917));
#26571=CARTESIAN_POINT('Ctrl Pts',(-5.59910040291772,41.8511757273801,10.3247095747702));
#26572=CARTESIAN_POINT('Ctrl Pts',(-5.61116995762818,41.9016079151995,10.3736117457735));
#26573=CARTESIAN_POINT('Ctrl Pts',(-5.62328043365746,41.952377546254,10.4221009095722));
#26574=CARTESIAN_POINT('Ctrl Pts',(-5.63542964579449,42.0034749115207,10.4701702229062));
#26575=CARTESIAN_POINT('Ctrl Pts',(-9.73793223897099,43.4867804707271,0.));
#26576=CARTESIAN_POINT('Ctrl Pts',(-9.95003683365976,43.4562844339543,1.72780310113343));
#26577=CARTESIAN_POINT('Ctrl Pts',(-10.2688299769306,44.1678235515684,3.28449990511991));
#26578=CARTESIAN_POINT('Ctrl Pts',(-10.5876231202014,44.8793626691825,4.84119670910639));
#26579=CARTESIAN_POINT('Ctrl Pts',(-10.9919738365584,46.1859677783933,5.91846432228298));
#26580=CARTESIAN_POINT('Ctrl Pts',(-11.3963245529154,47.492572887604,6.99573193545957));
#26581=CARTESIAN_POINT('Ctrl Pts',(-11.8481561402183,49.1294147079799,7.3802042952164));
#26582=CARTESIAN_POINT('Ctrl Pts',(-12.2999877275211,50.7662565283559,7.76467665497323));
#26583=CARTESIAN_POINT('Ctrl Pts',(-12.751819314824,52.4030983487319,7.3802042952164));
#26584=CARTESIAN_POINT('Ctrl Pts',(-8.27145263712669,41.6230663715378,0.));
#26585=CARTESIAN_POINT('Ctrl Pts',(-8.48355723181546,41.5925703347649,2.19648874705823));
#26586=CARTESIAN_POINT('Ctrl Pts',(-8.83129082048318,42.5053946713977,4.17545672685569));
#26587=CARTESIAN_POINT('Ctrl Pts',(-9.1790244091509,43.4182190080304,6.15442470665315));
#26588=CARTESIAN_POINT('Ctrl Pts',(-9.6355240061596,45.0875275490506,7.52391304034141));
#26589=CARTESIAN_POINT('Ctrl Pts',(-10.0920236031683,46.7568360900709,8.89340137402968));
#26590=CARTESIAN_POINT('Ctrl Pts',(-10.6088837810005,48.8459616921115,9.38216610144962));
#26591=CARTESIAN_POINT('Ctrl Pts',(-11.1257439588327,50.9350872941522,9.87093082886955));
#26592=CARTESIAN_POINT('Ctrl Pts',(-11.6426041366649,53.0242128961928,9.38216610144962));
#26593=CARTESIAN_POINT('Ctrl Pts',(-7.1967494923288,39.5090640497074,0.));
#26594=CARTESIAN_POINT('Ctrl Pts',(-7.40885408701757,39.4785680129345,2.70899372698069));
#26595=CARTESIAN_POINT('Ctrl Pts',(-7.78823388144401,40.6114965452661,5.14971273833323));
#26596=CARTESIAN_POINT('Ctrl Pts',(-8.16761367587042,41.7444250775976,7.59043174968577));
#26597=CARTESIAN_POINT('Ctrl Pts',(-8.68113776523077,43.8103476746564,9.27946171175751));
#26598=CARTESIAN_POINT('Ctrl Pts',(-9.19466185459112,45.8762702717153,10.9684916738292));
#26599=CARTESIAN_POINT('Ctrl Pts',(-9.78263041129817,48.4599655121837,11.5712994880388));
#26600=CARTESIAN_POINT('Ctrl Pts',(-10.3705989680052,51.0436607526522,12.1741073022483));
#26601=CARTESIAN_POINT('Ctrl Pts',(-10.9585675247123,53.6273559931207,11.5712994880388));
#26602=CARTESIAN_POINT('Ctrl Pts',(-6.55512420987382,37.2260157227863,1.04083408558608E-14));
#26603=CARTESIAN_POINT('Ctrl Pts',(-6.76722880456258,37.1955196860134,3.24562220582793));
#26604=CARTESIAN_POINT('Ctrl Pts',(-7.17974438483085,38.5589126710877,6.16982677025168));
#26605=CARTESIAN_POINT('Ctrl Pts',(-7.5922599650991,39.9223056561619,9.09403133467541));
#26606=CARTESIAN_POINT('Ctrl Pts',(-8.16549267737338,42.4035108473794,11.1176436806954));
#26607=CARTESIAN_POINT('Ctrl Pts',(-8.73872538964765,44.8847160385968,13.1412560267153));
#26608=CARTESIAN_POINT('Ctrl Pts',(-9.40114938129445,47.9862602037601,13.8634749112255));
#26609=CARTESIAN_POINT('Ctrl Pts',(-10.0635733729412,51.0878043689232,14.5856937957357));
#26610=CARTESIAN_POINT('Ctrl Pts',(-10.725997364588,54.1893485340865,13.8634749112255));
#26611=CARTESIAN_POINT('',(-6.55512420987382,37.2260157227863,1.04083408558608E-14));
#26612=CARTESIAN_POINT('Ctrl Pts',(-6.55512420987382,37.2260157227863,1.04083408558608E-14));
#26613=CARTESIAN_POINT('Ctrl Pts',(-6.76722880456259,37.1955196860134,3.24562220582793));
#26614=CARTESIAN_POINT('Ctrl Pts',(-7.17974438483084,38.5589126710876,6.16982677025168));
#26615=CARTESIAN_POINT('Ctrl Pts',(-7.52412807936677,39.6971249853932,8.61106394926976));
#26616=CARTESIAN_POINT('Ctrl Pts',(-7.98700482807814,41.6420486840549,10.4489096280657));
#26617=CARTESIAN_POINT('Origin',(-23.8837944332596,32.3559861244013,0.));
#26618=CARTESIAN_POINT('Ctrl Pts',(-6.55512420987382,37.2260157227863,1.04083408558608E-14));
#26619=CARTESIAN_POINT('Ctrl Pts',(-6.76722880456258,37.1955196860134,3.24562220582793));
#26620=CARTESIAN_POINT('Ctrl Pts',(-7.17974438483084,38.5589126710876,6.16982677025167));
#26621=CARTESIAN_POINT('Ctrl Pts',(-7.59225996509909,39.9223056561619,9.09403133467541));
#26622=CARTESIAN_POINT('Ctrl Pts',(-8.16549267737337,42.4035108473794,11.1176436806954));
#26623=CARTESIAN_POINT('Ctrl Pts',(-8.73872538964765,44.8847160385968,13.1412560267153));
#26624=CARTESIAN_POINT('Ctrl Pts',(-9.40114938129445,47.9862602037601,13.8634749112255));
#26625=CARTESIAN_POINT('Ctrl Pts',(-10.0635733729412,51.0878043689232,14.5856937957357));
#26626=CARTESIAN_POINT('Ctrl Pts',(-10.725997364588,54.1893485340865,13.8634749112255));
#26627=CARTESIAN_POINT('Ctrl Pts',(-5.75838408981604,36.7040912252865,0.));
#26628=CARTESIAN_POINT('Ctrl Pts',(-5.97048868450482,36.6735951885138,3.38941559469372));
#26629=CARTESIAN_POINT('Ctrl Pts',(-6.39188323248862,38.0987427505052,6.44317352589573));
#26630=CARTESIAN_POINT('Ctrl Pts',(-6.81327778047242,39.5238903124967,9.49693145709775));
#26631=CARTESIAN_POINT('Ctrl Pts',(-7.40250983972833,42.1163734062201,11.6101975146502));
#26632=CARTESIAN_POINT('Ctrl Pts',(-7.99174189898427,44.7088564999435,13.7234635722027));
#26633=CARTESIAN_POINT('Ctrl Pts',(-8.67411674998994,47.949161939876,14.4776794959001));
#26634=CARTESIAN_POINT('Ctrl Pts',(-9.35649160099562,51.1894673798086,15.2318954195974));
#26635=CARTESIAN_POINT('Ctrl Pts',(-10.0388664520013,54.4297728197411,14.4776794959001));
#26636=CARTESIAN_POINT('Ctrl Pts',(-4.81560839388856,36.8396419064669,0.));
#26637=CARTESIAN_POINT('Ctrl Pts',(-5.02771298857735,36.8091458696941,3.38941559469373));
#26638=CARTESIAN_POINT('Ctrl Pts',(-5.44910753656113,38.2342934316856,6.44317352589574));
#26639=CARTESIAN_POINT('Ctrl Pts',(-5.87050208454493,39.6594409936771,9.49693145709774));
#26640=CARTESIAN_POINT('Ctrl Pts',(-6.45973414380086,42.2519240874005,11.6101975146502));
#26641=CARTESIAN_POINT('Ctrl Pts',(-7.04896620305677,44.8444071811238,13.7234635722027));
#26642=CARTESIAN_POINT('Ctrl Pts',(-7.73134105406246,48.0847126210563,14.4776794959001));
#26643=CARTESIAN_POINT('Ctrl Pts',(-8.41371590506814,51.3250180609889,15.2318954195974));
#26644=CARTESIAN_POINT('Ctrl Pts',(-9.09609075607382,54.5653235009214,14.4776794959001));
#26645=CARTESIAN_POINT('Ctrl Pts',(-4.19818497005511,37.5648924257372,0.));
#26646=CARTESIAN_POINT('Ctrl Pts',(-4.41028956474389,37.5343963889644,3.24562220582793));
#26647=CARTESIAN_POINT('Ctrl Pts',(-4.82280514501214,38.8977893740386,6.16982677025167));
#26648=CARTESIAN_POINT('Ctrl Pts',(-5.2353207252804,40.2611823591128,9.09403133467541));
#26649=CARTESIAN_POINT('Ctrl Pts',(-5.80855343755469,42.7423875503303,11.1176436806954));
#26650=CARTESIAN_POINT('Ctrl Pts',(-6.38178614982895,45.2235927415478,13.1412560267153));
#26651=CARTESIAN_POINT('Ctrl Pts',(-7.04421014147574,48.325136906711,13.8634749112255));
#26652=CARTESIAN_POINT('Ctrl Pts',(-7.70663413312253,51.4266810718742,14.5856937957357));
#26653=CARTESIAN_POINT('Ctrl Pts',(-8.36905812476932,54.5282252370374,13.8634749112255));
#26654=CARTESIAN_POINT('',(-5.31260798925235,36.9500351333131,-1.58737143836679E-29));
#26655=CARTESIAN_POINT('Origin',(-5.56877962163339,38.731713020801,0.));
#26656=CARTESIAN_POINT('Origin',(-5.56877962163339,38.731713020801,0.));
#26657=CARTESIAN_POINT('Ctrl Pts',(1.19058808997905,37.78,0.));
#26658=CARTESIAN_POINT('Ctrl Pts',(0.976302375693351,37.7800000000001,3.24562220582793));
#26659=CARTESIAN_POINT('Ctrl Pts',(0.762016661407626,39.1882226984276,6.16982677025168));
#26660=CARTESIAN_POINT('Ctrl Pts',(0.547730947121928,40.5964453968553,9.09403133467541));
#26661=CARTESIAN_POINT('Ctrl Pts',(0.333445232836203,43.1339750175689,11.1176436806954));
#26662=CARTESIAN_POINT('Ctrl Pts',(0.119159518550494,45.6715046382825,13.1412560267153));
#26663=CARTESIAN_POINT('Ctrl Pts',(-0.095126195735231,48.8357523191413,
13.8634749112255));
#26664=CARTESIAN_POINT('Ctrl Pts',(-0.309411910020934,52.0000000000001,
14.5856937957357));
#26665=CARTESIAN_POINT('Ctrl Pts',(-0.523697624306645,55.1642476808589,
13.8634749112255));
#26666=CARTESIAN_POINT('Ctrl Pts',(1.50077089879005,40.1311229851416,0.));
#26667=CARTESIAN_POINT('Ctrl Pts',(1.28648518450433,40.1311229851416,2.7089937269807));
#26668=CARTESIAN_POINT('Ctrl Pts',(1.07219947021862,41.30651131265,5.14971273833323));
#26669=CARTESIAN_POINT('Ctrl Pts',(0.857913755932912,42.4818996401584,7.59043174968578));
#26670=CARTESIAN_POINT('Ctrl Pts',(0.643628041647182,44.5998762217203,9.27946171175751));
#26671=CARTESIAN_POINT('Ctrl Pts',(0.429342327361475,46.7178528032822,10.9684916738293));
#26672=CARTESIAN_POINT('Ctrl Pts',(0.215056613075752,49.3589264016411,11.5712994880388));
#26673=CARTESIAN_POINT('Ctrl Pts',(0.000770898790061796,52.0000000000001,
12.1741073022483));
#26674=CARTESIAN_POINT('Ctrl Pts',(-0.213514815495672,54.641073598359,11.5712994880388));
#26675=CARTESIAN_POINT('Ctrl Pts',(2.26368121662724,42.3765540157191,0.));
#26676=CARTESIAN_POINT('Ctrl Pts',(2.04939550234153,42.3765540157191,2.19648874705824));
#26677=CARTESIAN_POINT('Ctrl Pts',(1.83510978805581,43.3295747662223,4.17545672685568));
#26678=CARTESIAN_POINT('Ctrl Pts',(1.62082407377009,44.2825955167256,6.15442470665314));
#26679=CARTESIAN_POINT('Ctrl Pts',(1.40653835948437,45.9998795700625,7.5239130403414));
#26680=CARTESIAN_POINT('Ctrl Pts',(1.19225264519867,47.7171636233994,8.89340137402968));
#26681=CARTESIAN_POINT('Ctrl Pts',(0.97796693091297,49.8585818116997,9.3821661014496));
#26682=CARTESIAN_POINT('Ctrl Pts',(0.763681216627241,52.0000000000001,9.87093082886954));
#26683=CARTESIAN_POINT('Ctrl Pts',(0.549395502341525,54.1414181883004,9.3821661014496));
#26684=CARTESIAN_POINT('Ctrl Pts',(3.44999999999997,44.4300000000001,0.));
#26685=CARTESIAN_POINT('Ctrl Pts',(3.23571428571429,44.43,1.72780310113342));
#26686=CARTESIAN_POINT('Ctrl Pts',(3.02142857142856,45.1796656699788,3.28449990511991));
#26687=CARTESIAN_POINT('Ctrl Pts',(2.80714285714285,45.9293313399575,4.84119670910638));
#26688=CARTESIAN_POINT('Ctrl Pts',(2.59285714285713,47.2801821999295,5.91846432228297));
#26689=CARTESIAN_POINT('Ctrl Pts',(2.37857142857142,48.6310330599015,6.99573193545956));
#26690=CARTESIAN_POINT('Ctrl Pts',(2.16428571428571,50.3155165299508,7.38020429521639));
#26691=CARTESIAN_POINT('Ctrl Pts',(1.95,52.0000000000001,7.76467665497322));
#26692=CARTESIAN_POINT('Ctrl Pts',(1.73571428571429,53.6844834700494,7.38020429521638));
#26693=CARTESIAN_POINT('',(1.19058808997418,37.780000000016,1.57947905961937E-9));
#26694=CARTESIAN_POINT('Origin',(19.0359549110502,35.425667181256,0.));
#26695=CARTESIAN_POINT('Ctrl Pts',(1.19058808978352,37.7800000000849,3.13103292922399E-9));
#26696=CARTESIAN_POINT('Ctrl Pts',(1.17440993603746,37.7800000001371,0.245038153335428));
#26697=CARTESIAN_POINT('Ctrl Pts',(1.15808907770404,37.7863378835296,0.490791160521648));
#26698=CARTESIAN_POINT('Ctrl Pts',(1.14165673905428,37.7990994961183,0.73676650072528));
#26699=CARTESIAN_POINT('Ctrl Pts',(1.12527834684947,37.8118192130496,0.981934317700951));
#26700=CARTESIAN_POINT('Ctrl Pts',(1.10878923237326,37.8309206531575,1.22732257376562));
#26701=CARTESIAN_POINT('Ctrl Pts',(1.09222177855721,37.8564381709892,1.47243294816341));
#26702=CARTESIAN_POINT('Ctrl Pts',(1.0756792758881,37.8819172585741,1.7171741780302));
#26703=CARTESIAN_POINT('Ctrl Pts',(1.05905869845468,37.9137931615159,1.96163791541591));
#26704=CARTESIAN_POINT('Ctrl Pts',(1.0423933267646,37.952048346258,2.20532408778532));
#26705=CARTESIAN_POINT('Ctrl Pts',(1.02574224815027,37.9902707213956,2.44880126242073));
#26706=CARTESIAN_POINT('Ctrl Pts',(1.00904648208995,38.034861424896,2.69150175431056));
#26707=CARTESIAN_POINT('Ctrl Pts',(0.992339825182841,38.0857510286499,2.93292951866814));
#26708=CARTESIAN_POINT('Ctrl Pts',(0.97563666334167,38.1366299861973,3.17430677585596));
#26709=CARTESIAN_POINT('Ctrl Pts',(0.958922645785205,38.1938051285552,3.4144113931835));
#26710=CARTESIAN_POINT('Ctrl Pts',(0.942231694705361,38.2571558430637,3.65275710614643));
#26711=CARTESIAN_POINT('Ctrl Pts',(0.925519549722483,38.3205869992973,3.89140546668797));
#26712=CARTESIAN_POINT('Ctrl Pts',(0.908830560437842,38.3902092842331,4.12829002081175));
#26713=CARTESIAN_POINT('Ctrl Pts',(0.892198465551259,38.4658518732603,4.36293874377821));
#26714=CARTESIAN_POINT('Ctrl Pts',(0.875549399295395,38.5415716478927,4.59782690201461));
#26715=CARTESIAN_POINT('Ctrl Pts',(0.858957373419405,38.6233238148868,4.83047425894972));
#26716=CARTESIAN_POINT('Ctrl Pts',(0.842455462110767,38.7108897721911,5.06042975959445));
#26717=CARTESIAN_POINT('Ctrl Pts',(0.825905305682021,38.7987117380296,5.29105755998316));
#26718=CARTESIAN_POINT('Ctrl Pts',(0.809445820264702,38.8923812869986,5.51897736305698));
#26719=CARTESIAN_POINT('Ctrl Pts',(0.793109157310668,38.9916337971362,5.74376259354339));
#26720=CARTESIAN_POINT('Ctrl Pts',(0.78269241522336,39.0549201489775,5.88709234072624));
#26721=CARTESIAN_POINT('Ctrl Pts',(0.7723255833285,39.1204754952205,6.02914825314194));
#26722=CARTESIAN_POINT('Ctrl Pts',(0.762016661412751,39.1882226984626,6.16982677023482));
#26723=CARTESIAN_POINT('Ctrl Pts',(0.745851968590237,39.2944523060728,6.39041482339095));
#26724=CARTESIAN_POINT('Ctrl Pts',(0.729544808781299,39.4066922926963,6.60890054011817));
#26725=CARTESIAN_POINT('Ctrl Pts',(0.713126327700918,39.524806665964,6.8248041200806));
#26726=CARTESIAN_POINT('Ctrl Pts',(0.696744912263108,39.6426543894045,7.04022028559308));
#26727=CARTESIAN_POINT('Ctrl Pts',(0.680252704625916,39.7663499173289,7.2530655202965));
#26728=CARTESIAN_POINT('Ctrl Pts',(0.663682105818481,39.8957079165131,7.46287566269427));
#26729=CARTESIAN_POINT('Ctrl Pts',(0.647138159323281,40.0248578550338,7.67234834441905));
#26730=CARTESIAN_POINT('Ctrl Pts',(0.63051610244954,40.1596519133317,7.87879526533066));
#26731=CARTESIAN_POINT('Ctrl Pts',(0.61384922452975,40.2998572837229,8.08177334612246));
#26732=CARTESIAN_POINT('Ctrl Pts',(0.597198339079101,40.4399281220157,8.28455666214133));
#26733=CARTESIAN_POINT('Ctrl Pts',(0.580502748576783,40.5853996821053,8.4838773927285));
#26734=CARTESIAN_POINT('Ctrl Pts',(0.563796248536221,40.7359942171314,8.67931873611065));
#26735=CARTESIAN_POINT('Ctrl Pts',(0.547088944957196,40.8865959953563,8.87476947970448));
#26736=CARTESIAN_POINT('Ctrl Pts',(0.530370761385448,41.0423209776637,9.06634009532769));
#26737=CARTESIAN_POINT('Ctrl Pts',(0.513675645356928,41.2028492923282,9.2536445034091));
#26738=CARTESIAN_POINT('Ctrl Pts',(0.496974404889857,41.3634364952207,9.4410176222641));
#26739=CARTESIAN_POINT('Ctrl Pts',(0.480296279393738,41.5288302394279,9.62412107874937));
#26740=CARTESIAN_POINT('Ctrl Pts',(0.463674941840256,41.6986725382748,9.80260437466018));
#26741=CARTESIAN_POINT('Ctrl Pts',(0.447026491442446,41.8687918850905,9.98137881379588));
#26742=CARTESIAN_POINT('Ctrl Pts',(0.430435044262104,42.0433739554943,10.1555177270917));
#26743=CARTESIAN_POINT('Ctrl Pts',(0.413933671136519,42.2220261712049,10.3247095747702));
#26744=CARTESIAN_POINT('Ctrl Pts',(0.409164215743436,42.2736627087962,10.3736117457734));
#26745=CARTESIAN_POINT('Ctrl Pts',(0.40440227873099,42.3256390786478,10.4221009095721));
#26746=CARTESIAN_POINT('Ctrl Pts',(0.399648641329916,42.3779453595728,10.4701702229061));
#26747=CARTESIAN_POINT('Ctrl Pts',(-3.45000000000002,44.43,0.));
#26748=CARTESIAN_POINT('Ctrl Pts',(-3.66428571428572,44.43,1.72780310113343));
#26749=CARTESIAN_POINT('Ctrl Pts',(-3.87857142857143,45.1796656699787,3.28449990511991));
#26750=CARTESIAN_POINT('Ctrl Pts',(-4.09285714285714,45.9293313399575,4.84119670910638));
#26751=CARTESIAN_POINT('Ctrl Pts',(-4.30714285714287,47.2801821999295,5.91846432228298));
#26752=CARTESIAN_POINT('Ctrl Pts',(-4.52142857142858,48.6310330599015,6.99573193545957));
#26753=CARTESIAN_POINT('Ctrl Pts',(-4.73571428571429,50.3155165299508,7.38020429521639));
#26754=CARTESIAN_POINT('Ctrl Pts',(-4.95000000000001,52.0000000000001,7.76467665497321));
#26755=CARTESIAN_POINT('Ctrl Pts',(-5.16428571428572,53.6844834700494,7.38020429521639));
#26756=CARTESIAN_POINT('Ctrl Pts',(-2.26368121662727,42.3765540157191,0.));
#26757=CARTESIAN_POINT('Ctrl Pts',(-2.47796693091298,42.3765540157191,2.19648874705824));
#26758=CARTESIAN_POINT('Ctrl Pts',(-2.6922526451987,43.3295747662223,4.17545672685568));
#26759=CARTESIAN_POINT('Ctrl Pts',(-2.90653835948441,44.2825955167256,6.15442470665314));
#26760=CARTESIAN_POINT('Ctrl Pts',(-3.12082407377012,45.9998795700625,7.5239130403414));
#26761=CARTESIAN_POINT('Ctrl Pts',(-3.33510978805584,47.7171636233994,8.89340137402967));
#26762=CARTESIAN_POINT('Ctrl Pts',(-3.54939550234154,49.8585818116997,9.38216610144961));
#26763=CARTESIAN_POINT('Ctrl Pts',(-3.76368121662726,52.0000000000001,9.87093082886954));
#26764=CARTESIAN_POINT('Ctrl Pts',(-3.97796693091297,54.1414181883004,9.3821661014496));
#26765=CARTESIAN_POINT('Ctrl Pts',(-1.50077089879007,40.1311229851416,0.));
#26766=CARTESIAN_POINT('Ctrl Pts',(-1.71505661307578,40.1311229851416,2.70899372698069));
#26767=CARTESIAN_POINT('Ctrl Pts',(-1.9293423273615,41.30651131265,5.14971273833323));
#26768=CARTESIAN_POINT('Ctrl Pts',(-2.14362804164721,42.4818996401584,7.59043174968578));
#26769=CARTESIAN_POINT('Ctrl Pts',(-2.35791375593293,44.5998762217203,9.27946171175751));
#26770=CARTESIAN_POINT('Ctrl Pts',(-2.57219947021866,46.7178528032822,10.9684916738293));
#26771=CARTESIAN_POINT('Ctrl Pts',(-2.78648518450437,49.3589264016411,11.5712994880388));
#26772=CARTESIAN_POINT('Ctrl Pts',(-3.00077089879007,52.0000000000001,12.1741073022483));
#26773=CARTESIAN_POINT('Ctrl Pts',(-3.21505661307579,54.641073598359,11.5712994880388));
#26774=CARTESIAN_POINT('Ctrl Pts',(-1.19058808997908,37.7800000000001,0.));
#26775=CARTESIAN_POINT('Ctrl Pts',(-1.40487380426479,37.7800000000001,3.24562220582792));
#26776=CARTESIAN_POINT('Ctrl Pts',(-1.61915951855051,39.1882226984277,6.16982677025167));
#26777=CARTESIAN_POINT('Ctrl Pts',(-1.83344523283622,40.5964453968552,9.09403133467541));
#26778=CARTESIAN_POINT('Ctrl Pts',(-2.04773094712195,43.1339750175689,11.1176436806954));
#26779=CARTESIAN_POINT('Ctrl Pts',(-2.26201666140765,45.6715046382825,13.1412560267153));
#26780=CARTESIAN_POINT('Ctrl Pts',(-2.47630237569339,48.8357523191413,13.8634749112255));
#26781=CARTESIAN_POINT('Ctrl Pts',(-2.69058808997909,52.0000000000001,14.5856937957357));
#26782=CARTESIAN_POINT('Ctrl Pts',(-2.90487380426479,55.1642476808589,13.8634749112255));
#26783=CARTESIAN_POINT('',(-1.19058808997908,37.7800000000001,0.));
#26784=CARTESIAN_POINT('Ctrl Pts',(-1.19058808997908,37.7800000000001,0.));
#26785=CARTESIAN_POINT('Ctrl Pts',(-1.40487380426479,37.7800000000001,3.24562220582792));
#26786=CARTESIAN_POINT('Ctrl Pts',(-1.61915951855051,39.1882226984277,6.16982677025167));
#26787=CARTESIAN_POINT('Ctrl Pts',(-1.79805338220529,40.363860562332,8.61106394926976));
#26788=CARTESIAN_POINT('Ctrl Pts',(-1.97942721139903,42.3548619717231,10.4489096280657));
#26789=CARTESIAN_POINT('Origin',(-19.0359549110502,35.425667181256,0.));
#26790=CARTESIAN_POINT('Ctrl Pts',(-1.19058808997907,37.7800000000001,0.));
#26791=CARTESIAN_POINT('Ctrl Pts',(-1.40487380426479,37.7800000000001,3.24562220582792));
#26792=CARTESIAN_POINT('Ctrl Pts',(-1.61915951855051,39.1882226984277,6.16982677025167));
#26793=CARTESIAN_POINT('Ctrl Pts',(-1.83344523283622,40.5964453968552,9.09403133467541));
#26794=CARTESIAN_POINT('Ctrl Pts',(-2.04773094712195,43.1339750175689,11.1176436806954));
#26795=CARTESIAN_POINT('Ctrl Pts',(-2.26201666140765,45.6715046382825,13.1412560267153));
#26796=CARTESIAN_POINT('Ctrl Pts',(-2.47630237569337,48.8357523191413,13.8634749112255));
#26797=CARTESIAN_POINT('Ctrl Pts',(-2.69058808997909,52.0000000000001,14.5856937957357));
#26798=CARTESIAN_POINT('Ctrl Pts',(-2.90487380426479,55.1642476808589,13.8634749112255));
#26799=CARTESIAN_POINT('Ctrl Pts',(-0.476235235991634,37.15,0.));
#26800=CARTESIAN_POINT('Ctrl Pts',(-0.690520950277348,37.15,3.38941559469372));
#26801=CARTESIAN_POINT('Ctrl Pts',(-0.904806664563067,38.6206123116491,
6.44317352589574));
#26802=CARTESIAN_POINT('Ctrl Pts',(-1.11909237884878,40.0912246232982,9.49693145709776));
#26803=CARTESIAN_POINT('Ctrl Pts',(-1.33337809313449,42.7411764423978,11.6101975146502));
#26804=CARTESIAN_POINT('Ctrl Pts',(-1.54766380742021,45.3911282614975,13.7234635722027));
#26805=CARTESIAN_POINT('Ctrl Pts',(-1.76194952170592,48.6955641307488,14.4776794959001));
#26806=CARTESIAN_POINT('Ctrl Pts',(-1.97623523599165,52.0000000000001,15.2318954195974));
#26807=CARTESIAN_POINT('Ctrl Pts',(-2.19052095027734,55.3044358692513,14.4776794959001));
#26808=CARTESIAN_POINT('Ctrl Pts',(0.476235235991609,37.15,0.));
#26809=CARTESIAN_POINT('Ctrl Pts',(0.261949521705892,37.15,3.38941559469373));
#26810=CARTESIAN_POINT('Ctrl Pts',(0.0476638074201876,38.6206123116491,
6.44317352589573));
#26811=CARTESIAN_POINT('Ctrl Pts',(-0.166621906865532,40.0912246232982,
9.49693145709774));
#26812=CARTESIAN_POINT('Ctrl Pts',(-0.38090762115124,42.7411764423979,11.6101975146502));
#26813=CARTESIAN_POINT('Ctrl Pts',(-0.595193335436943,45.3911282614975,
13.7234635722027));
#26814=CARTESIAN_POINT('Ctrl Pts',(-0.809479049722658,48.6955641307488,
14.4776794959001));
#26815=CARTESIAN_POINT('Ctrl Pts',(-1.02376476400838,52.0000000000001,15.2318954195974));
#26816=CARTESIAN_POINT('Ctrl Pts',(-1.23805047829409,55.3044358692513,14.4776794959001));
#26817=CARTESIAN_POINT('Ctrl Pts',(1.19058808997905,37.7800000000001,0.));
#26818=CARTESIAN_POINT('Ctrl Pts',(0.976302375693353,37.7800000000001,3.24562220582793));
#26819=CARTESIAN_POINT('Ctrl Pts',(0.762016661407622,39.1882226984276,6.16982677025167));
#26820=CARTESIAN_POINT('Ctrl Pts',(0.547730947121925,40.5964453968553,9.09403133467541));
#26821=CARTESIAN_POINT('Ctrl Pts',(0.333445232836203,43.1339750175689,11.1176436806954));
#26822=CARTESIAN_POINT('Ctrl Pts',(0.119159518550494,45.6715046382825,13.1412560267153));
#26823=CARTESIAN_POINT('Ctrl Pts',(-0.095126195735231,48.8357523191413,
13.8634749112255));
#26824=CARTESIAN_POINT('Ctrl Pts',(-0.309411910020934,52.0000000000001,
14.5856937957357));
#26825=CARTESIAN_POINT('Ctrl Pts',(-0.523697624306645,55.1642476808589,
13.8634749112255));
#26826=CARTESIAN_POINT('',(4.974042353288E-6,37.3300000000069,-1.41995316083721E-29));
#26827=CARTESIAN_POINT('Origin',(-1.04083408558608E-14,39.13,0.));
#26828=CARTESIAN_POINT('Origin',(-1.04083408558608E-14,39.13,0.));
#26829=CARTESIAN_POINT('Ctrl Pts',(6.55512420987434,37.2260157227862,0.));
#26830=CARTESIAN_POINT('Ctrl Pts',(6.34301961518558,37.256511759559,3.24562220582793));
#26831=CARTESIAN_POINT('Ctrl Pts',(6.33132600607631,38.6808968181789,6.16982677025168));
#26832=CARTESIAN_POINT('Ctrl Pts',(6.31963239696705,40.1052818767988,9.09403133467542));
#26833=CARTESIAN_POINT('Ctrl Pts',(6.46865591986383,42.647479141562,11.1176436806954));
#26834=CARTESIAN_POINT('Ctrl Pts',(6.61767944276062,45.1896764063252,13.1412560267153));
#26835=CARTESIAN_POINT('Ctrl Pts',(6.8558942450299,48.3522126450341,13.8634749112255));
#26836=CARTESIAN_POINT('Ctrl Pts',(7.09410904729919,51.514748883743,14.5856937957357));
#26837=CARTESIAN_POINT('Ctrl Pts',(7.33232384956847,54.6772851224519,13.8634749112255));
#26838=CARTESIAN_POINT('Ctrl Pts',(7.19674949232937,39.5090640497073,0.));
#26839=CARTESIAN_POINT('Ctrl Pts',(6.98464489764059,39.5395600864802,2.7089937269807));
#26840=CARTESIAN_POINT('Ctrl Pts',(6.93981550268949,40.7334806923574,5.14971273833323));
#26841=CARTESIAN_POINT('Ctrl Pts',(6.8949861077384,41.9274012982346,7.59043174968578));
#26842=CARTESIAN_POINT('Ctrl Pts',(6.98430100772122,44.0543159688391,9.27946171175751));
#26843=CARTESIAN_POINT('Ctrl Pts',(7.07361590770406,46.1812306394436,10.9684916738293));
#26844=CARTESIAN_POINT('Ctrl Pts',(7.23737527503361,48.8259179534577,11.5712994880388));
#26845=CARTESIAN_POINT('Ctrl Pts',(7.40113464236316,51.4706052674719,12.1741073022483));
#26846=CARTESIAN_POINT('Ctrl Pts',(7.5648940096927,54.1152925814861,11.5712994880388));
#26847=CARTESIAN_POINT('Ctrl Pts',(8.27145263712728,41.6230663715376,0.));
#26848=CARTESIAN_POINT('Ctrl Pts',(8.0593480424385,41.6535624083105,2.19648874705824));
#26849=CARTESIAN_POINT('Ctrl Pts',(7.98287244172871,42.6273788184889,4.17545672685568));
#26850=CARTESIAN_POINT('Ctrl Pts',(7.90639684101889,43.6011952286674,6.15442470665314));
#26851=CARTESIAN_POINT('Ctrl Pts',(7.93868724865007,45.3314958432333,7.5239130403414));
#26852=CARTESIAN_POINT('Ctrl Pts',(7.97097765628125,47.0617964577992,8.89340137402968));
#26853=CARTESIAN_POINT('Ctrl Pts',(8.06362864473592,49.2119141333855,9.38216610144961));
#26854=CARTESIAN_POINT('Ctrl Pts',(8.1562796331906,51.3620318089719,9.87093082886954));
#26855=CARTESIAN_POINT('Ctrl Pts',(8.24893062164529,53.5121494845582,9.38216610144961));
#26856=CARTESIAN_POINT('Ctrl Pts',(9.7379322389716,43.486780470727,1.04083408558608E-14));
#26857=CARTESIAN_POINT('Ctrl Pts',(9.52582764428285,43.5172765074998,1.72780310113343));
#26858=CARTESIAN_POINT('Ctrl Pts',(9.42041159817612,44.2898076986596,3.28449990511991));
#26859=CARTESIAN_POINT('Ctrl Pts',(9.31499555206944,45.0623388898195,4.84119670910639));
#26860=CARTESIAN_POINT('Ctrl Pts',(9.2951370790489,46.4299360725759,5.91846432228298));
#26861=CARTESIAN_POINT('Ctrl Pts',(9.27527860602838,47.7975332553323,6.99573193545956));
#26862=CARTESIAN_POINT('Ctrl Pts',(9.30290100395372,49.495367149254,7.38020429521639));
#26863=CARTESIAN_POINT('Ctrl Pts',(9.33052340187904,51.1932010431756,7.76467665497322));
#26864=CARTESIAN_POINT('Ctrl Pts',(9.35814579980438,52.8910349370973,7.38020429521639));
#26865=CARTESIAN_POINT('',(6.55512420987177,37.2260157228026,1.57948610458898E-9));
#26866=CARTESIAN_POINT('Origin',(23.88379443326,32.355986124401,0.));
#26867=CARTESIAN_POINT('Ctrl Pts',(6.55512420969287,37.2260157228979,3.13104631369862E-9));
#26868=CARTESIAN_POINT('Ctrl Pts',(6.5391107262324,37.2283181142835,0.245038153335441));
#26869=CARTESIAN_POINT('Ctrl Pts',(6.52385796555408,37.2369141874758,0.490791160521659));
#26870=CARTESIAN_POINT('Ctrl Pts',(6.50940905124996,37.2518844708665,0.736766500725291));
#26871=CARTESIAN_POINT('Ctrl Pts',(6.49500757192006,37.2668056076575,0.981934317700964));
#26872=CARTESIAN_POINT('Ctrl Pts',(6.48140471121363,37.2880592683071,1.22732257376564));
#26873=CARTESIAN_POINT('Ctrl Pts',(6.46863741161248,37.3156748491109,1.47243294816343));
#26874=CARTESIAN_POINT('Ctrl Pts',(6.45588933999723,37.343248839914,1.71717417803015));
#26875=CARTESIAN_POINT('Ctrl Pts',(6.44397435004916,37.3771656469145,1.9616379154158));
#26876=CARTESIAN_POINT('Ctrl Pts',(6.43292288824308,37.4174031787121,2.20532408778515));
#26877=CARTESIAN_POINT('Ctrl Pts',(6.4218809047363,37.457606200743,2.44880126242052));
#26878=CARTESIAN_POINT('Ctrl Pts',(6.41170099625834,37.5041190904231,2.69150175431031));
#26879=CARTESIAN_POINT('Ctrl Pts',(6.40240673475756,37.5568683165633,2.93292951866785));
#26880=CARTESIAN_POINT('Ctrl Pts',(6.39311441763482,37.6096065074603,3.17430677585579));
#26881=CARTESIAN_POINT('Ctrl Pts',(6.38470739581538,37.6685783420143,3.41441139318347));
#26882=CARTESIAN_POINT('Ctrl Pts',(6.37720208124093,37.7336596075968,3.65275710614652));
#26883=CARTESIAN_POINT('Ctrl Pts',(6.36968723653793,37.7988235123306,3.89140546668802));
#26884=CARTESIAN_POINT('Ctrl Pts',(6.36307640132153,37.8701122336038,4.12829002081177));
#26885=CARTESIAN_POINT('Ctrl Pts',(6.35737866000337,37.9473518840362,4.3629387437782));
#26886=CARTESIAN_POINT('Ctrl Pts',(6.35167510471693,38.0246703497133,4.59782690201454));
#26887=CARTESIAN_POINT('Ctrl Pts',(6.34688650816488,38.1079516890035,4.83047425894959));
#26888=CARTESIAN_POINT('Ctrl Pts',(6.34301449757158,38.1969748179611,5.06042975959426));
#26889=CARTESIAN_POINT('Ctrl Pts',(6.33913116673708,38.2862582156518,5.291057559983));
#26890=CARTESIAN_POINT('Ctrl Pts',(6.33616978186134,38.3813167726778,5.51897736305682));
#26891=CARTESIAN_POINT('Ctrl Pts',(6.33412450750911,38.4818839849188,5.74376259354325));
#26892=CARTESIAN_POINT('Ctrl Pts',(6.33282037976375,38.5460086299152,5.88709234072615));
#26893=CARTESIAN_POINT('Ctrl Pts',(6.33188856576836,38.612372071261,6.0291482531419));
#26894=CARTESIAN_POINT('Ctrl Pts',(6.33132600608635,38.6808968182128,6.16982677023484));
#26895=CARTESIAN_POINT('Ctrl Pts',(6.33044389595609,38.7883456372327,6.39041482339094));
#26896=CARTESIAN_POINT('Ctrl Pts',(6.33027613506514,38.90176393344,6.60890054011813));
#26897=CARTESIAN_POINT('Ctrl Pts',(6.330834198378,39.0210126661743,6.82480412008054));
#26898=CARTESIAN_POINT('Ctrl Pts',(6.33139100183161,39.1399921882013,7.04022028559307));
#26899=CARTESIAN_POINT('Ctrl Pts',(6.33267037014005,39.2647757598683,7.25306552029654));
#26900=CARTESIAN_POINT('Ctrl Pts',(6.33467799886891,39.3951753232291,7.46287566269436));
#26901=CARTESIAN_POINT('Ctrl Pts',(6.3366823985082,39.5253651506641,7.67234834441888));
#26902=CARTESIAN_POINT('Ctrl Pts',(6.33941272481327,39.6611527651411,7.87879526533023));
#26903=CARTESIAN_POINT('Ctrl Pts',(6.34286879629131,39.8023029910567,8.08177334612178));
#26904=CARTESIAN_POINT('Ctrl Pts',(6.3463215515444,39.9433177782513,8.28455666214088));
#26905=CARTESIAN_POINT('Ctrl Pts',(6.35049865962787,40.0896846778742,8.48387739272826));
#26906=CARTESIAN_POINT('Ctrl Pts',(6.35539404456602,40.2411239605247,8.67931873611061));
#26907=CARTESIAN_POINT('Ctrl Pts',(6.36028966495923,40.3925705270039,8.87476947970449));
#26908=CARTESIAN_POINT('Ctrl Pts',(6.3659036240628,40.5490896991196,9.06634009532774));
#26909=CARTESIAN_POINT('Ctrl Pts',(6.37222400138285,40.7103600297412,9.25364450340919));
#26910=CARTESIAN_POINT('Ctrl Pts',(6.37854669727095,40.871689520792,9.44101762226431));
#26911=CARTESIAN_POINT('Ctrl Pts',(6.38557631500277,41.037773339894,9.62412107874969));
#26912=CARTESIAN_POINT('Ctrl Pts',(6.39329523799196,41.2082523519969,9.80260437466061));
#26913=CARTESIAN_POINT('Ctrl Pts',(6.40102675214335,41.3790094506796,9.98137881379614));
#26914=CARTESIAN_POINT('Ctrl Pts',(6.40944980108734,41.5541757364553,10.1555177270918));
#26915=CARTESIAN_POINT('Ctrl Pts',(6.41854124933317,41.7333579204527,10.3247095747701));
#26916=CARTESIAN_POINT('Ctrl Pts',(6.42116898561529,41.7851476368179,10.3736117457734));
#26917=CARTESIAN_POINT('Ctrl Pts',(6.42385252692496,41.8372726564641,10.4221009095722));
#26918=CARTESIAN_POINT('Ctrl Pts',(6.42659123460897,41.8897230480066,10.4701702229062));
#26919=CARTESIAN_POINT('Ctrl Pts',(2.90816428999319,44.4687528548127,0.));
#26920=CARTESIAN_POINT('Ctrl Pts',(2.69605969530443,44.4992488915856,1.72780310113343));
#26921=CARTESIAN_POINT('Ctrl Pts',(2.5906436491977,45.2717800827453,3.28449990511991));
#26922=CARTESIAN_POINT('Ctrl Pts',(2.48522760309099,46.0443112739052,4.84119670910639));
#26923=CARTESIAN_POINT('Ctrl Pts',(2.46536913007047,47.4119084566616,5.91846432228298));
#26924=CARTESIAN_POINT('Ctrl Pts',(2.44551065704996,48.7795056394181,6.99573193545957));
#26925=CARTESIAN_POINT('Ctrl Pts',(2.47313305497529,50.4773395333397,7.38020429521639));
#26926=CARTESIAN_POINT('Ctrl Pts',(2.50075545290062,52.1751734272613,7.76467665497322));
#26927=CARTESIAN_POINT('Ctrl Pts',(2.52837785082596,53.873007321183,7.3802042952164));
#26928=CARTESIAN_POINT('Ctrl Pts',(3.79017222552573,42.2673772240308,0.));
#26929=CARTESIAN_POINT('Ctrl Pts',(3.57806763083696,42.2978732608037,2.19648874705823));
#26930=CARTESIAN_POINT('Ctrl Pts',(3.50159203012716,43.2716896709821,4.17545672685568));
#26931=CARTESIAN_POINT('Ctrl Pts',(3.42511642941735,44.2455060811606,6.15442470665314));
#26932=CARTESIAN_POINT('Ctrl Pts',(3.45740683704852,45.9758066957265,7.5239130403414));
#26933=CARTESIAN_POINT('Ctrl Pts',(3.48969724467969,47.7061073102924,8.89340137402968));
#26934=CARTESIAN_POINT('Ctrl Pts',(3.58234823313438,49.8562249858787,9.38216610144961));
#26935=CARTESIAN_POINT('Ctrl Pts',(3.67499922158908,52.006342661465,9.87093082886954));
#26936=CARTESIAN_POINT('Ctrl Pts',(3.76765021004374,54.1564603370514,9.38216610144961));
#26937=CARTESIAN_POINT('Ctrl Pts',(4.22575906238271,39.9362279852004,0.));
#26938=CARTESIAN_POINT('Ctrl Pts',(4.01365446769395,39.9667240219733,2.7089937269807));
#26939=CARTESIAN_POINT('Ctrl Pts',(3.96882507274284,41.1606446278505,5.14971273833323));
#26940=CARTESIAN_POINT('Ctrl Pts',(3.92399567779176,42.3545652337277,7.59043174968578));
#26941=CARTESIAN_POINT('Ctrl Pts',(4.01331057777458,44.4814799043322,9.27946171175752));
#26942=CARTESIAN_POINT('Ctrl Pts',(4.10262547775741,46.6083945749368,10.9684916738293));
#26943=CARTESIAN_POINT('Ctrl Pts',(4.26638484508696,49.2530818889509,11.5712994880388));
#26944=CARTESIAN_POINT('Ctrl Pts',(4.43014421241652,51.8977692029651,12.1741073022483));
#26945=CARTESIAN_POINT('Ctrl Pts',(4.59390357974606,54.5424565169792,11.5712994880388));
#26946=CARTESIAN_POINT('Ctrl Pts',(4.19818497005566,37.5648924257371,0.));
#26947=CARTESIAN_POINT('Ctrl Pts',(3.98608037536688,37.59538846251,3.24562220582792));
#26948=CARTESIAN_POINT('Ctrl Pts',(3.97438676625761,39.0197735211299,6.16982677025168));
#26949=CARTESIAN_POINT('Ctrl Pts',(3.96269315714836,40.4441585797498,9.09403133467541));
#26950=CARTESIAN_POINT('Ctrl Pts',(4.11171668004512,42.986355844513,11.1176436806954));
#26951=CARTESIAN_POINT('Ctrl Pts',(4.26074020294192,45.5285531092761,13.1412560267153));
#26952=CARTESIAN_POINT('Ctrl Pts',(4.49895500521119,48.6910893479851,13.8634749112255));
#26953=CARTESIAN_POINT('Ctrl Pts',(4.73716980748048,51.853625586694,14.5856937957357));
#26954=CARTESIAN_POINT('Ctrl Pts',(4.97538460974978,55.0161618254029,13.8634749112255));
#26955=CARTESIAN_POINT('',(4.19818497005567,37.5648924257371,0.));
#26956=CARTESIAN_POINT('Ctrl Pts',(4.19818497005567,37.5648924257371,0.));
#26957=CARTESIAN_POINT('Ctrl Pts',(3.98608037536688,37.59538846251,3.24562220582792));
#26958=CARTESIAN_POINT('Ctrl Pts',(3.97438676625761,39.0197735211299,6.16982677025168));
#26959=CARTESIAN_POINT('Ctrl Pts',(3.96462449666071,40.2089043379837,8.61106394926976));
#26960=CARTESIAN_POINT('Ctrl Pts',(4.06844583510807,42.2054524109828,10.4489096280657));
#26961=CARTESIAN_POINT('Origin',(-13.8005982420121,37.7741838134886,0.));
#26962=CARTESIAN_POINT('Ctrl Pts',(4.19818497005566,37.5648924257371,0.));
#26963=CARTESIAN_POINT('Ctrl Pts',(3.98608037536688,37.59538846251,3.24562220582792));
#26964=CARTESIAN_POINT('Ctrl Pts',(3.97438676625761,39.0197735211299,6.16982677025168));
#26965=CARTESIAN_POINT('Ctrl Pts',(3.96269315714836,40.4441585797498,9.09403133467541));
#26966=CARTESIAN_POINT('Ctrl Pts',(4.11171668004512,42.986355844513,11.1176436806954));
#26967=CARTESIAN_POINT('Ctrl Pts',(4.26074020294192,45.5285531092761,13.1412560267153));
#26968=CARTESIAN_POINT('Ctrl Pts',(4.49895500521119,48.6910893479851,13.8634749112255));
#26969=CARTESIAN_POINT('Ctrl Pts',(4.73716980748048,51.853625586694,14.5856937957357));
#26970=CARTESIAN_POINT('Ctrl Pts',(4.97538460974978,55.0161618254029,13.8634749112255));
#26971=CARTESIAN_POINT('Ctrl Pts',(4.81560839388908,36.8396419064669,6.24500451351651E-15));
#26972=CARTESIAN_POINT('Ctrl Pts',(4.60350379920032,36.8701379432397,3.38941559469373));
#26973=CARTESIAN_POINT('Ctrl Pts',(4.60068915780659,38.3562775787769,6.44317352589574));
#26974=CARTESIAN_POINT('Ctrl Pts',(4.59787451641287,39.8424172143141,9.49693145709774));
#26975=CARTESIAN_POINT('Ctrl Pts',(4.7628973862913,42.4958923815831,11.6101975146502));
#26976=CARTESIAN_POINT('Ctrl Pts',(4.92792025616971,45.1493675488522,13.7234635722027));
#26977=CARTESIAN_POINT('Ctrl Pts',(5.18608591779791,48.4506650623305,14.4776794959001));
#26978=CARTESIAN_POINT('Ctrl Pts',(5.4442515794261,51.7519625758087,15.2318954195974));
#26979=CARTESIAN_POINT('Ctrl Pts',(5.70241724105428,55.0532600892868,14.4776794959001));
#26980=CARTESIAN_POINT('Ctrl Pts',(5.75838408981657,36.7040912252865,0.));
#26981=CARTESIAN_POINT('Ctrl Pts',(5.54627949512779,36.7345872620593,3.38941559469373));
#26982=CARTESIAN_POINT('Ctrl Pts',(5.54346485373408,38.2207268975965,6.44317352589574));
#26983=CARTESIAN_POINT('Ctrl Pts',(5.54065021234035,39.7068665331337,9.49693145709774));
#26984=CARTESIAN_POINT('Ctrl Pts',(5.70567308221878,42.3603417004028,11.6101975146502));
#26985=CARTESIAN_POINT('Ctrl Pts',(5.87069595209718,45.0138168676718,13.7234635722027));
#26986=CARTESIAN_POINT('Ctrl Pts',(6.12886161372538,48.31511438115,14.4776794959001));
#26987=CARTESIAN_POINT('Ctrl Pts',(6.38702727535358,51.6164118946283,15.2318954195974));
#26988=CARTESIAN_POINT('Ctrl Pts',(6.64519293698177,54.9177094081064,14.4776794959001));
#26989=CARTESIAN_POINT('Ctrl Pts',(6.55512420987434,37.2260157227862,0.));
#26990=CARTESIAN_POINT('Ctrl Pts',(6.34301961518558,37.2565117595591,3.24562220582793));
#26991=CARTESIAN_POINT('Ctrl Pts',(6.33132600607631,38.6808968181789,6.16982677025167));
#26992=CARTESIAN_POINT('Ctrl Pts',(6.31963239696705,40.1052818767988,9.09403133467541));
#26993=CARTESIAN_POINT('Ctrl Pts',(6.46865591986383,42.647479141562,11.1176436806954));
#26994=CARTESIAN_POINT('Ctrl Pts',(6.61767944276062,45.1896764063252,13.1412560267153));
#26995=CARTESIAN_POINT('Ctrl Pts',(6.85589424502988,48.3522126450341,13.8634749112255));
#26996=CARTESIAN_POINT('Ctrl Pts',(7.09410904729919,51.514748883743,14.5856937957357));
#26997=CARTESIAN_POINT('Ctrl Pts',(7.33232384956847,54.6772851224519,13.8634749112255));
#26998=CARTESIAN_POINT('',(5.3126178361619,36.9500337175413,-1.22362873180948E-29));
#26999=CARTESIAN_POINT('Origin',(5.56877962163395,38.7317130208009,0.));
#27000=CARTESIAN_POINT('Origin',(5.56877962163395,38.7317130208009,0.));
#27001=CARTESIAN_POINT('Ctrl Pts',(11.7862169042735,35.9142171164209,0.));
#27002=CARTESIAN_POINT('Ctrl Pts',(11.5806112670704,35.9745883786013,3.24562220582793));
#27003=CARTESIAN_POINT('Ctrl Pts',(11.7717478112975,37.3861394252072,6.16982677025168));
#27004=CARTESIAN_POINT('Ctrl Pts',(11.9628843555245,38.7976904718133,9.09403133467541));
#27005=CARTESIAN_POINT('Ctrl Pts',(12.4721834264259,41.292803575407,11.1176436806954));
#27006=CARTESIAN_POINT('Ctrl Pts',(12.9814824973274,43.7879166790007,13.1412560267153));
#27007=CARTESIAN_POINT('Ctrl Pts',(13.6673484497322,46.884361357741,13.8634749112255));
#27008=CARTESIAN_POINT('Ctrl Pts',(14.353214402137,49.9808060364812,14.5856937957357));
#27009=CARTESIAN_POINT('Ctrl Pts',(15.0390803545419,53.0772507152215,13.8634749112255));
#27010=CARTESIAN_POINT('Ctrl Pts',(12.7462230199163,38.0827145049532,0.));
#27011=CARTESIAN_POINT('Ctrl Pts',(12.5406173827132,38.1430857671335,2.70899372698069));
#27012=CARTESIAN_POINT('Ctrl Pts',(12.6661569043006,39.3312338708266,5.14971273833323));
#27013=CARTESIAN_POINT('Ctrl Pts',(12.791696425888,40.5193819745197,7.59043174968577));
#27014=CARTESIAN_POINT('Ctrl Pts',(13.1827937463386,42.6119368849887,9.27946171175751));
#27015=CARTESIAN_POINT('Ctrl Pts',(13.5738910667892,44.7044917954577,10.9684916738292));
#27016=CARTESIAN_POINT('Ctrl Pts',(14.1123618472582,47.2989546180622,11.5712994880388));
#27017=CARTESIAN_POINT('Ctrl Pts',(14.6508326277272,49.8934174406666,12.1741073022483));
#27018=CARTESIAN_POINT('Ctrl Pts',(15.1893034081961,52.4878802632711,11.5712994880388));
#27019=CARTESIAN_POINT('Ctrl Pts',(14.1108411348348,40.0222531270432,-1.05434036998093E-14));
#27020=CARTESIAN_POINT('Ctrl Pts',(13.9052354976316,40.0826243892235,2.19648874705823));
#27021=CARTESIAN_POINT('Ctrl Pts',(13.9681268331908,41.0574123652206,4.17545672685568));
#27022=CARTESIAN_POINT('Ctrl Pts',(14.0310181687499,42.0322003412176,6.15442470665314));
#27023=CARTESIAN_POINT('Ctrl Pts',(14.3092273587164,43.7402935862748,7.52391304034139));
#27024=CARTESIAN_POINT('Ctrl Pts',(14.5874365486829,45.4483868313321,8.89340137402966));
#27025=CARTESIAN_POINT('Ctrl Pts',(14.9851381329364,47.5634337987569,9.3821661014496));
#27026=CARTESIAN_POINT('Ctrl Pts',(15.38283971719,49.6784807661817,9.87093082886953));
#27027=CARTESIAN_POINT('Ctrl Pts',(15.7805413014435,51.7935277336064,9.3821661014496));
#27028=CARTESIAN_POINT('Ctrl Pts',(15.8276282594351,41.6582954965891,0.));
#27029=CARTESIAN_POINT('Ctrl Pts',(15.622022622232,41.7186667587694,1.72780310113342));
#27030=CARTESIAN_POINT('Ctrl Pts',(15.6276222110082,42.4983369638543,3.28449990511991));
#27031=CARTESIAN_POINT('Ctrl Pts',(15.6332217997845,43.2780071689392,4.84119670910638));
#27032=CARTESIAN_POINT('Ctrl Pts',(15.8081948292727,44.6345103396637,5.91846432228297));
#27033=CARTESIAN_POINT('Ctrl Pts',(15.983167858761,45.9910135103883,6.99573193545955));
#27034=CARTESIAN_POINT('Ctrl Pts',(16.252136056532,47.6676348262506,7.38020429521638));
#27035=CARTESIAN_POINT('Ctrl Pts',(16.521104254303,49.344256142113,7.76467665497321));
#27036=CARTESIAN_POINT('Ctrl Pts',(16.790072452074,51.0208774579754,7.38020429521638));
#27037=CARTESIAN_POINT('',(11.7862169043639,35.9142171164878,1.57948960455104E-9));
#27038=CARTESIAN_POINT('Origin',(28.245428775984,28.6276304970123,0.));
#27039=CARTESIAN_POINT('Ctrl Pts',(11.7862169041098,35.9142171165574,3.13105403642851E-9));
#27040=CARTESIAN_POINT('Ctrl Pts',(11.7706940792791,35.9187750292273,0.24503815333559));
#27041=CARTESIAN_POINT('Ctrl Pts',(11.756819918478,35.9294543009582,0.490791160521951));
#27042=CARTESIAN_POINT('Ctrl Pts',(11.7446485667475,35.9463285033517,0.736766500725725));
#27043=CARTESIAN_POINT('Ctrl Pts',(11.7325171728812,35.9631473086865,0.981934317701356));
#27044=CARTESIAN_POINT('Ctrl Pts',(11.7220774809611,35.9861205266374,1.22732257376599));
#27045=CARTESIAN_POINT('Ctrl Pts',(11.7133702409769,36.0152719968249,1.47243294816374));
#27046=CARTESIAN_POINT('Ctrl Pts',(11.7046761143912,36.0443795639103,1.71717417803052));
#27047=CARTESIAN_POINT('Ctrl Pts',(11.6977092667638,36.079646826587,1.96163791541622));
#27048=CARTESIAN_POINT('Ctrl Pts',(11.6924966907343,36.1210475853283,2.20532408778562));
#27049=CARTESIAN_POINT('Ctrl Pts',(11.6872885852768,36.1624128366599,2.44880126242109));
#27050=CARTESIAN_POINT('Ctrl Pts',(11.6838317679614,36.2099010442177,2.69150175431097));
#27051=CARTESIAN_POINT('Ctrl Pts',(11.6821391062287,36.2634360706164,2.9329295186686));
#27052=CARTESIAN_POINT('Ctrl Pts',(11.6804467986042,36.3169598973807,3.17430677585645));
#27053=CARTESIAN_POINT('Ctrl Pts',(11.6805179152422,36.3765279276399,3.41441139318402));
#27054=CARTESIAN_POINT('Ctrl Pts',(11.6823510237343,36.4420148774081,3.65275710614698));
#27055=CARTESIAN_POINT('Ctrl Pts',(11.6841864598783,36.5075849814588,3.89140546668851));
#27056=CARTESIAN_POINT('Ctrl Pts',(11.6877883562711,36.579088906284,4.12829002081228));
#27057=CARTESIAN_POINT('Ctrl Pts',(11.6931409581037,36.6563532415796,4.36293874377873));
#27058=CARTESIAN_POINT('Ctrl Pts',(11.6984990217246,36.7336964173083,4.59782690201504));
#27059=CARTESIAN_POINT('Ctrl Pts',(11.7056113365131,36.8168115609901,4.83047425895006));
#27060=CARTESIAN_POINT('Ctrl Pts',(11.7144480496049,36.9054796074171,5.0604297595947));
#27061=CARTESIAN_POINT('Ctrl Pts',(11.7233105977818,36.994406884455,5.29105755998342));
#27062=CARTESIAN_POINT('Ctrl Pts',(11.7339075987038,37.0889193314433,5.51897736305724));
#27063=CARTESIAN_POINT('Ctrl Pts',(11.7461953488411,37.1887539873582,5.74376259354366));
#27064=CARTESIAN_POINT('Ctrl Pts',(11.7540303837178,37.2524115326578,5.88709234072642));
#27065=CARTESIAN_POINT('Ctrl Pts',(11.7625525566677,37.3182321008169,6.02914825314204));
#27066=CARTESIAN_POINT('Ctrl Pts',(11.7717478113122,37.3861394252393,6.16982677023484));
#27067=CARTESIAN_POINT('Ctrl Pts',(11.7861662410927,37.4926201075706,6.39041482339101));
#27068=CARTESIAN_POINT('Ctrl Pts',(11.8021412942477,37.6049078439222,6.60890054011826));
#27069=CARTESIAN_POINT('Ctrl Pts',(11.819664541394,37.7228633758097,6.82480412008072));
#27070=CARTESIAN_POINT('Ctrl Pts',(11.8371482288264,37.8405526164633,7.04022028559315));
#27071=CARTESIAN_POINT('Ctrl Pts',(11.8561731288311,37.9638839981998,7.25306552029652));
#27072=CARTESIAN_POINT('Ctrl Pts',(11.8767181155649,38.0926705666683,7.46287566269426));
#27073=CARTESIAN_POINT('Ctrl Pts',(11.8972300575422,38.221249993568,7.67234834441908));
#27074=CARTESIAN_POINT('Ctrl Pts',(11.9192571854562,38.3552669199728,7.87879526533072));
#27075=CARTESIAN_POINT('Ctrl Pts',(11.9427658506832,38.4944885898571,8.08177334612255));
#27076=CARTESIAN_POINT('Ctrl Pts',(11.9662519585,38.6335766715391,8.28455666214149));
#27077=CARTESIAN_POINT('Ctrl Pts',(11.9912167312945,38.7778593027061,8.48387739272872));
#27078=CARTESIAN_POINT('Ctrl Pts',(12.0176143452911,38.9270604659007,8.67931873611092));
#27079=CARTESIAN_POINT('Ctrl Pts',(12.0440132289432,39.0762688052766,8.8747694797048));
#27080=CARTESIAN_POINT('Ctrl Pts',(12.0718450467041,39.2303958882203,9.06634009532807));
#27081=CARTESIAN_POINT('Ctrl Pts',(12.1010522527169,39.3891252359326,9.25364450340952));
#27082=CARTESIAN_POINT('Ctrl Pts',(12.1302701731051,39.5479128119397,9.44101762226463));
#27083=CARTESIAN_POINT('Ctrl Pts',(12.1608644313196,39.7113057183257,9.62412107874999));
#27084=CARTESIAN_POINT('Ctrl Pts',(12.1927664798389,39.878950982619,9.8026043746609));
#27085=CARTESIAN_POINT('Ctrl Pts',(12.2247205672072,40.0468697110625,9.98137881379654));
#27086=CARTESIAN_POINT('Ctrl Pts',(12.2579866432891,40.2190543317699,10.1555177270923));
#27087=CARTESIAN_POINT('Ctrl Pts',(12.2924858372377,40.3951188515069,10.3247095747707));
#27088=CARTESIAN_POINT('Ctrl Pts',(12.302457272062,40.4460074573699,10.3736117457738));
#27089=CARTESIAN_POINT('Ctrl Pts',(12.3125316625314,40.4972200117264,10.4221009095723));
#27090=CARTESIAN_POINT('Ctrl Pts',(12.3227069631098,40.548746775169,10.4701702229062));
#27091=CARTESIAN_POINT('Ctrl Pts',(9.20712674149506,43.602250138795,0.));
#27092=CARTESIAN_POINT('Ctrl Pts',(9.00152110429196,43.6626214009754,1.72780310113343));
#27093=CARTESIAN_POINT('Ctrl Pts',(9.00712069306818,44.4422916060602,3.28449990511991));
#27094=CARTESIAN_POINT('Ctrl Pts',(9.01272028184443,45.2219618111451,4.84119670910638));
#27095=CARTESIAN_POINT('Ctrl Pts',(9.18769331133267,46.5784649818697,5.91846432228298));
#27096=CARTESIAN_POINT('Ctrl Pts',(9.36266634082093,47.9349681525942,6.99573193545957));
#27097=CARTESIAN_POINT('Ctrl Pts',(9.63163453859197,49.6115894684566,7.38020429521639));
#27098=CARTESIAN_POINT('Ctrl Pts',(9.90060273636299,51.2882107843189,7.76467665497321));
#27099=CARTESIAN_POINT('Ctrl Pts',(10.169570934134,52.9648321001813,7.38020429521639));
#27100=CARTESIAN_POINT('Ctrl Pts',(9.76686869112084,41.2977585211119,0.));
#27101=CARTESIAN_POINT('Ctrl Pts',(9.56126305391773,41.3581297832922,2.19648874705823));
#27102=CARTESIAN_POINT('Ctrl Pts',(9.62415438947685,42.3329177592892,4.17545672685568));
#27103=CARTESIAN_POINT('Ctrl Pts',(9.68704572503597,43.3077057352862,6.15442470665314));
#27104=CARTESIAN_POINT('Ctrl Pts',(9.96525491500249,45.0157989803435,7.5239130403414));
#27105=CARTESIAN_POINT('Ctrl Pts',(10.243464104969,46.7238922254008,8.89340137402968));
#27106=CARTESIAN_POINT('Ctrl Pts',(10.6411656892225,48.8389391928255,9.38216610144961));
#27107=CARTESIAN_POINT('Ctrl Pts',(11.038867273476,50.9539861602503,9.87093082886954));
#27108=CARTESIAN_POINT('Ctrl Pts',(11.4365688577295,53.0690331276751,9.3821661014496));
#27109=CARTESIAN_POINT('Ctrl Pts',(9.86626475512792,38.9283465500519,0.));
#27110=CARTESIAN_POINT('Ctrl Pts',(9.66065911792481,38.9887178122322,2.70899372698069));
#27111=CARTESIAN_POINT('Ctrl Pts',(9.78619863951222,40.1768659159253,5.14971273833323));
#27112=CARTESIAN_POINT('Ctrl Pts',(9.91173816109965,41.3650140196184,7.59043174968577));
#27113=CARTESIAN_POINT('Ctrl Pts',(10.3028354815503,43.4575689300874,9.27946171175752));
#27114=CARTESIAN_POINT('Ctrl Pts',(10.6939328020009,45.5501238405564,10.9684916738292));
#27115=CARTESIAN_POINT('Ctrl Pts',(11.2324035824698,48.1445866631609,11.5712994880388));
#27116=CARTESIAN_POINT('Ctrl Pts',(11.7708743629388,50.7390494857653,12.1741073022483));
#27117=CARTESIAN_POINT('Ctrl Pts',(12.3093451434078,53.3335123083698,11.5712994880388));
#27118=CARTESIAN_POINT('Ctrl Pts',(9.50149509066547,36.5850719698904,1.04083408558608E-14));
#27119=CARTESIAN_POINT('Ctrl Pts',(9.29588945346236,36.6454432320708,3.24562220582792));
#27120=CARTESIAN_POINT('Ctrl Pts',(9.48702599768942,38.0569942786768,6.16982677025167));
#27121=CARTESIAN_POINT('Ctrl Pts',(9.67816254191645,39.4685453252828,9.09403133467541));
#27122=CARTESIAN_POINT('Ctrl Pts',(10.1874616128179,41.9636584288765,11.1176436806954));
#27123=CARTESIAN_POINT('Ctrl Pts',(10.6967606837193,44.4587715324702,13.1412560267153));
#27124=CARTESIAN_POINT('Ctrl Pts',(11.3826266361241,47.5552162112105,13.8634749112255));
#27125=CARTESIAN_POINT('Ctrl Pts',(12.068492588529,50.6516608899507,14.5856937957357));
#27126=CARTESIAN_POINT('Ctrl Pts',(12.7543585409338,53.7481055686911,13.8634749112255));
#27127=CARTESIAN_POINT('',(9.50149509066547,36.5850719698904,1.04083408558608E-14));
#27128=CARTESIAN_POINT('Ctrl Pts',(9.50149509066547,36.5850719698904,1.04083408558608E-14));
#27129=CARTESIAN_POINT('Ctrl Pts',(9.29588945346237,36.6454432320708,3.24562220582792));
#27130=CARTESIAN_POINT('Ctrl Pts',(9.48702599768942,38.0569942786767,6.16982677025167));
#27131=CARTESIAN_POINT('Ctrl Pts',(9.64659405380729,39.2354107742189,8.61106394926976));
#27132=CARTESIAN_POINT('Ctrl Pts',(10.033497056841,41.196861549629,10.4489096280657));
#27133=CARTESIAN_POINT('Origin',(-8.28430119040596,39.3537269950292,0.));
#27134=CARTESIAN_POINT('Ctrl Pts',(9.50149509066549,36.5850719698904,1.04083408558608E-14));
#27135=CARTESIAN_POINT('Ctrl Pts',(9.29588945346237,36.6454432320708,3.24562220582792));
#27136=CARTESIAN_POINT('Ctrl Pts',(9.48702599768942,38.0569942786767,6.16982677025167));
#27137=CARTESIAN_POINT('Ctrl Pts',(9.67816254191646,39.4685453252828,9.09403133467541));
#27138=CARTESIAN_POINT('Ctrl Pts',(10.1874616128179,41.9636584288765,11.1176436806954));
#27139=CARTESIAN_POINT('Ctrl Pts',(10.6967606837193,44.4587715324702,13.1412560267153));
#27140=CARTESIAN_POINT('Ctrl Pts',(11.3826266361241,47.5552162112105,13.8634749112255));
#27141=CARTESIAN_POINT('Ctrl Pts',(12.068492588529,50.6516608899507,14.5856937957357));
#27142=CARTESIAN_POINT('Ctrl Pts',(12.7543585409338,53.748105568691,13.8634749112255));
#27143=CARTESIAN_POINT('Ctrl Pts',(10.0094201239378,35.7793349404724,0.));
#27144=CARTESIAN_POINT('Ctrl Pts',(9.80381448673468,35.8397062026528,3.38941559469374));
#27145=CARTESIAN_POINT('Ctrl Pts',(10.012528216215,37.3111196447713,6.44317352589574));
#27146=CARTESIAN_POINT('Ctrl Pts',(10.2212419456952,38.7825330868899,9.49693145709775));
#27147=CARTESIAN_POINT('Ctrl Pts',(10.7622140099937,41.3855144999133,11.6101975146502));
#27148=CARTESIAN_POINT('Ctrl Pts',(11.3031860742922,43.9884959129366,13.7234635722027));
#27149=CARTESIAN_POINT('Ctrl Pts',(12.0285476034518,47.2194501734233,14.4776794959001));
#27150=CARTESIAN_POINT('Ctrl Pts',(12.7539091326114,50.4504044339099,15.2318954195974));
#27151=CARTESIAN_POINT('Ctrl Pts',(13.479270661771,53.6813586943965,14.4776794959001));
#27152=CARTESIAN_POINT('Ctrl Pts',(10.923308849381,35.5109929990846,0.));
#27153=CARTESIAN_POINT('Ctrl Pts',(10.7177032121779,35.571364261265,3.38941559469374));
#27154=CARTESIAN_POINT('Ctrl Pts',(10.9264169416582,37.0427777033835,6.44317352589574));
#27155=CARTESIAN_POINT('Ctrl Pts',(11.1351306711385,38.5141911455021,9.49693145709775));
#27156=CARTESIAN_POINT('Ctrl Pts',(11.6761027354369,41.1171725585255,11.6101975146502));
#27157=CARTESIAN_POINT('Ctrl Pts',(12.2170747997354,43.7201539715489,13.7234635722027));
#27158=CARTESIAN_POINT('Ctrl Pts',(12.942436328895,46.9511082320355,14.4776794959001));
#27159=CARTESIAN_POINT('Ctrl Pts',(13.6677978580546,50.1820624925221,15.2318954195974));
#27160=CARTESIAN_POINT('Ctrl Pts',(14.3931593872142,53.4130167530087,14.4776794959001));
#27161=CARTESIAN_POINT('Ctrl Pts',(11.7862169042735,35.9142171164209,0.));
#27162=CARTESIAN_POINT('Ctrl Pts',(11.5806112670704,35.9745883786013,3.24562220582793));
#27163=CARTESIAN_POINT('Ctrl Pts',(11.7717478112975,37.3861394252072,6.16982677025168));
#27164=CARTESIAN_POINT('Ctrl Pts',(11.9628843555245,38.7976904718133,9.09403133467541));
#27165=CARTESIAN_POINT('Ctrl Pts',(12.472183426426,41.292803575407,11.1176436806954));
#27166=CARTESIAN_POINT('Ctrl Pts',(12.9814824973274,43.7879166790007,13.1412560267153));
#27167=CARTESIAN_POINT('Ctrl Pts',(13.6673484497322,46.884361357741,13.8634749112255));
#27168=CARTESIAN_POINT('Ctrl Pts',(14.353214402137,49.9808060364812,14.5856937957357));
#27169=CARTESIAN_POINT('Ctrl Pts',(15.0390803545419,53.0772507152215,13.8634749112255));
#27170=CARTESIAN_POINT('',(10.5170811194392,35.8178713036897,-1.00239475043615E-29));
#27171=CARTESIAN_POINT('Origin',(11.0241949492054,37.5449600575352,0.));
#27172=CARTESIAN_POINT('Origin',(11.0241949492054,37.5449600575352,0.));
#27173=CARTESIAN_POINT('Ctrl Pts',(16.7773762111445,33.8713086176151,0.));
#27174=CARTESIAN_POINT('Ctrl Pts',(16.5824550692829,33.9603261204012,3.24562220582793));
#27175=CARTESIAN_POINT('Ctrl Pts',(16.972530777998,35.3303080462615,6.16982677025168));
#27176=CARTESIAN_POINT('Ctrl Pts',(17.3626064867132,36.7002899721219,9.09403133467542));
#27177=CARTESIAN_POINT('Ctrl Pts',(18.221813245233,39.0975256070689,11.1176436806954));
#27178=CARTESIAN_POINT('Ctrl Pts',(19.0810200037527,41.4947612420159,13.1412560267153));
#27179=CARTESIAN_POINT('Ctrl Pts',(20.2005748533762,44.4620796765375,13.8634749112255));
#27180=CARTESIAN_POINT('Ctrl Pts',(21.3201297029997,47.4293981110592,14.5856937957357));
#27181=CARTESIAN_POINT('Ctrl Pts',(22.4396845526232,50.3967165455808,13.8634749112255));
#27182=CARTESIAN_POINT('Ctrl Pts',(18.0362202038896,35.8811107143581,0.));
#27183=CARTESIAN_POINT('Ctrl Pts',(17.8412990620279,35.9701282171442,2.7089937269807));
#27184=CARTESIAN_POINT('Ctrl Pts',(18.1346518775204,37.1283165495981,5.14971273833323));
#27185=CARTESIAN_POINT('Ctrl Pts',(18.4280046930129,38.2865048820522,7.59043174968578));
#27186=CARTESIAN_POINT('Ctrl Pts',(19.1129228203184,40.3021016488385,9.27946171175752));
#27187=CARTESIAN_POINT('Ctrl Pts',(19.797840947624,42.317698415625,10.9684916738293));
#27188=CARTESIAN_POINT('Ctrl Pts',(20.7000614289636,44.8091209655645,11.5712994880388));
#27189=CARTESIAN_POINT('Ctrl Pts',(21.6022819103031,47.300543515504,12.1741073022483));
#27190=CARTESIAN_POINT('Ctrl Pts',(22.5045023916426,49.7919660654434,11.5712994880388));
#27191=CARTESIAN_POINT('Ctrl Pts',(19.6629735993426,37.6067022235296,0.));
#27192=CARTESIAN_POINT('Ctrl Pts',(19.4680524574809,37.6957197263157,2.19648874705824));
#27193=CARTESIAN_POINT('Ctrl Pts',(19.6690304430806,38.6516353959964,4.17545672685568));
#27194=CARTESIAN_POINT('Ctrl Pts',(19.8700084286803,39.607551065677,6.15442470665314));
#27195=CARTESIAN_POINT('Ctrl Pts',(20.3884728641635,41.2586650884904,7.5239130403414));
#27196=CARTESIAN_POINT('Ctrl Pts',(20.9069372996467,42.9097791113039,8.89340137402967));
#27197=CARTESIAN_POINT('Ctrl Pts',(21.6015934223203,44.9466991136021,9.3821661014496));
#27198=CARTESIAN_POINT('Ctrl Pts',(22.2962495449939,46.9836191159003,9.87093082886954));
#27199=CARTESIAN_POINT('Ctrl Pts',(22.9909056676675,49.0205391181986,9.3821661014496));
#27200=CARTESIAN_POINT('Ctrl Pts',(21.5951194116472,38.9817677587446,0.));
#27201=CARTESIAN_POINT('Ctrl Pts',(21.4001982697855,39.0707852615307,1.72780310113343));
#27202=CARTESIAN_POINT('Ctrl Pts',(21.5166995019651,39.8417226435484,3.28449990511991));
#27203=CARTESIAN_POINT('Ctrl Pts',(21.6332007341447,40.612660025566,4.84119670910638));
#27204=CARTESIAN_POINT('Ctrl Pts',(21.9994433198419,41.9304546915348,5.91846432228298));
#27205=CARTESIAN_POINT('Ctrl Pts',(22.3656859055391,43.2482493575036,6.99573193545955));
#27206=CARTESIAN_POINT('Ctrl Pts',(22.8705244862895,44.8695269202924,7.38020429521639));
#27207=CARTESIAN_POINT('Ctrl Pts',(23.3753630670398,46.4908044830812,7.76467665497321));
#27208=CARTESIAN_POINT('Ctrl Pts',(23.8802016477901,48.1120820458699,7.38020429521639));
#27209=CARTESIAN_POINT('',(16.7773762109261,33.8713086175738,-1.21941606378243E-9));
#27210=CARTESIAN_POINT('Origin',(32.0320676419193,24.3164988679735,0.));
#27211=CARTESIAN_POINT('Ctrl Pts',(16.7773762111445,33.8713086176151,0.));
#27212=CARTESIAN_POINT('Ctrl Pts',(16.5824550692829,33.9603261204012,3.24562220582793));
#27213=CARTESIAN_POINT('Ctrl Pts',(16.972530777998,35.3303080462615,6.16982677025168));
#27214=CARTESIAN_POINT('Ctrl Pts',(17.3001355482566,36.4808862649313,8.62571762198521));
#27215=CARTESIAN_POINT('Ctrl Pts',(17.9679679135941,38.3823149509185,10.4701702229062));
#27216=CARTESIAN_POINT('Ctrl Pts',(15.3186586437011,41.8481313484577,1.04083408558608E-14));
#27217=CARTESIAN_POINT('Ctrl Pts',(15.1237375018394,41.9371488512438,1.72780310113343));
#27218=CARTESIAN_POINT('Ctrl Pts',(15.240238734019,42.7080862332614,3.28449990511991));
#27219=CARTESIAN_POINT('Ctrl Pts',(15.3567399661986,43.4790236152791,4.84119670910639));
#27220=CARTESIAN_POINT('Ctrl Pts',(15.7229825518958,44.7968182812479,5.91846432228298));
#27221=CARTESIAN_POINT('Ctrl Pts',(16.089225137593,46.1146129472167,6.99573193545957));
#27222=CARTESIAN_POINT('Ctrl Pts',(16.5940637183433,47.7358905100055,7.38020429521639));
#27223=CARTESIAN_POINT('Ctrl Pts',(17.0989022990936,49.3571680727943,7.76467665497322));
#27224=CARTESIAN_POINT('Ctrl Pts',(17.603740879844,50.978445635583,7.38020429521639));
#27225=CARTESIAN_POINT('Ctrl Pts',(15.5447398754882,39.4874365476043,0.));
#27226=CARTESIAN_POINT('Ctrl Pts',(15.3498187336265,39.5764540503904,2.19648874705824));
#27227=CARTESIAN_POINT('Ctrl Pts',(15.5507967192262,40.5323697200711,4.17545672685568));
#27228=CARTESIAN_POINT('Ctrl Pts',(15.7517747048259,41.4882853897517,6.15442470665314));
#27229=CARTESIAN_POINT('Ctrl Pts',(16.2702391403091,43.1393994125652,7.52391304034141));
#27230=CARTESIAN_POINT('Ctrl Pts',(16.7887035757923,44.7905134353786,8.89340137402968));
#27231=CARTESIAN_POINT('Ctrl Pts',(17.4833596984659,46.8274334376768,9.38216610144961));
#27232=CARTESIAN_POINT('Ctrl Pts',(18.1780158211395,48.864353439975,9.87093082886954));
#27233=CARTESIAN_POINT('Ctrl Pts',(18.8726719438131,50.9012734422733,9.38216610144961));
#27234=CARTESIAN_POINT('Ctrl Pts',(15.3059217494168,37.1279962392255,0.));
#27235=CARTESIAN_POINT('Ctrl Pts',(15.1110006075551,37.2170137420116,2.70899372698069));
#27236=CARTESIAN_POINT('Ctrl Pts',(15.4043534230476,38.3752020744656,5.14971273833323));
#27237=CARTESIAN_POINT('Ctrl Pts',(15.6977062385401,39.5333904069196,7.59043174968579));
#27238=CARTESIAN_POINT('Ctrl Pts',(16.3826243658456,41.548987173706,9.27946171175752));
#27239=CARTESIAN_POINT('Ctrl Pts',(17.0675424931512,43.5645839404925,10.9684916738293));
#27240=CARTESIAN_POINT('Ctrl Pts',(17.9697629744908,46.0560064904319,11.5712994880388));
#27241=CARTESIAN_POINT('Ctrl Pts',(18.8719834558303,48.5474290403714,12.1741073022483));
#27242=CARTESIAN_POINT('Ctrl Pts',(19.7742039371699,51.0388515903109,11.5712994880388));
#27243=CARTESIAN_POINT('Ctrl Pts',(14.6113821712786,34.8604849513722,0.));
#27244=CARTESIAN_POINT('Ctrl Pts',(14.4164610294169,34.9495024541583,3.24562220582793));
#27245=CARTESIAN_POINT('Ctrl Pts',(14.8065367381321,36.3194843800186,6.16982677025168));
#27246=CARTESIAN_POINT('Ctrl Pts',(15.1966124468473,37.689466305879,9.09403133467542));
#27247=CARTESIAN_POINT('Ctrl Pts',(16.055819205367,40.086701940826,11.1176436806954));
#27248=CARTESIAN_POINT('Ctrl Pts',(16.9150259638868,42.4839375757731,13.1412560267153));
#27249=CARTESIAN_POINT('Ctrl Pts',(18.0345808135103,45.4512560102947,13.8634749112255));
#27250=CARTESIAN_POINT('Ctrl Pts',(19.1541356631338,48.4185744448163,14.5856937957357));
#27251=CARTESIAN_POINT('Ctrl Pts',(20.2736905127572,51.3858928793379,13.8634749112255));
#27252=CARTESIAN_POINT('',(14.6113821712786,34.8604849513722,0.));
#27253=CARTESIAN_POINT('Ctrl Pts',(14.6113821712786,34.8604849513722,0.));
#27254=CARTESIAN_POINT('Ctrl Pts',(14.4164610294169,34.9495024541583,3.24562220582793));
#27255=CARTESIAN_POINT('Ctrl Pts',(14.8065367381321,36.3194843800186,6.16982677025167));
#27256=CARTESIAN_POINT('Ctrl Pts',(15.1321867744985,37.4631973926724,8.61106394926976));
#27257=CARTESIAN_POINT('Ctrl Pts',(15.7942952127128,39.3496213890631,10.4489096280657));
#27258=CARTESIAN_POINT('Origin',(-2.59935965651494,40.1321417817282,0.));
#27259=CARTESIAN_POINT('Ctrl Pts',(14.6113821712786,34.8604849513722,0.));
#27260=CARTESIAN_POINT('Ctrl Pts',(14.4164610294169,34.9495024541583,3.24562220582793));
#27261=CARTESIAN_POINT('Ctrl Pts',(14.8065367381321,36.3194843800186,6.16982677025167));
#27262=CARTESIAN_POINT('Ctrl Pts',(15.1966124468473,37.689466305879,9.09403133467541));
#27263=CARTESIAN_POINT('Ctrl Pts',(16.055819205367,40.086701940826,11.1176436806954));
#27264=CARTESIAN_POINT('Ctrl Pts',(16.9150259638868,42.483937575773,13.1412560267153));
#27265=CARTESIAN_POINT('Ctrl Pts',(18.0345808135103,45.4512560102947,13.8634749112255));
#27266=CARTESIAN_POINT('Ctrl Pts',(19.1541356631338,48.4185744448163,14.5856937957357));
#27267=CARTESIAN_POINT('Ctrl Pts',(20.2736905127572,51.3858928793379,13.8634749112255));
#27268=CARTESIAN_POINT('Ctrl Pts',(14.9994689250472,33.9906638941717,6.24500451351651E-15));
#27269=CARTESIAN_POINT('Ctrl Pts',(14.8045477831855,34.0796813969578,3.38941559469372));
#27270=CARTESIAN_POINT('Ctrl Pts',(15.2205410738882,35.5064149111822,6.44317352589573));
#27271=CARTESIAN_POINT('Ctrl Pts',(15.636534364591,36.9331484254066,9.49693145709774));
#27272=CARTESIAN_POINT('Ctrl Pts',(16.542442992115,39.4326468889937,11.6101975146502));
#27273=CARTESIAN_POINT('Ctrl Pts',(17.448351619639,41.9321453525807,13.7234635722027));
#27274=CARTESIAN_POINT('Ctrl Pts',(18.6261427473663,45.0269834486349,14.4776794959001));
#27275=CARTESIAN_POINT('Ctrl Pts',(19.8039338750935,48.1218215446891,15.2318954195974));
#27276=CARTESIAN_POINT('Ctrl Pts',(20.9817250028208,51.2166596407433,14.4776794959001));
#27277=CARTESIAN_POINT('Ctrl Pts',(15.8658665409936,33.5949933606688,0.));
#27278=CARTESIAN_POINT('Ctrl Pts',(15.6709453991319,33.684010863455,3.38941559469373));
#27279=CARTESIAN_POINT('Ctrl Pts',(16.0869386898346,35.1107443776793,6.44317352589574));
#27280=CARTESIAN_POINT('Ctrl Pts',(16.5029319805374,36.5374778919037,9.49693145709774));
#27281=CARTESIAN_POINT('Ctrl Pts',(17.4088406080614,39.0369763554908,11.6101975146502));
#27282=CARTESIAN_POINT('Ctrl Pts',(18.3147492355854,41.5364748190779,13.7234635722027));
#27283=CARTESIAN_POINT('Ctrl Pts',(19.4925403633127,44.631312915132,14.4776794959001));
#27284=CARTESIAN_POINT('Ctrl Pts',(20.6703314910399,47.7261510111863,15.2318954195974));
#27285=CARTESIAN_POINT('Ctrl Pts',(21.8481226187672,50.8209891072404,14.4776794959001));
#27286=CARTESIAN_POINT('Ctrl Pts',(16.7773762111446,33.8713086176151,0.));
#27287=CARTESIAN_POINT('Ctrl Pts',(16.5824550692829,33.9603261204012,3.24562220582793));
#27288=CARTESIAN_POINT('Ctrl Pts',(16.972530777998,35.3303080462615,6.16982677025167));
#27289=CARTESIAN_POINT('Ctrl Pts',(17.3626064867132,36.7002899721219,9.09403133467541));
#27290=CARTESIAN_POINT('Ctrl Pts',(18.221813245233,39.0975256070689,11.1176436806954));
#27291=CARTESIAN_POINT('Ctrl Pts',(19.0810200037527,41.4947612420159,13.1412560267153));
#27292=CARTESIAN_POINT('Ctrl Pts',(20.2005748533762,44.4620796765375,13.8634749112255));
#27293=CARTESIAN_POINT('Ctrl Pts',(21.3201297029997,47.4293981110591,14.5856937957357));
#27294=CARTESIAN_POINT('Ctrl Pts',(22.4396845526232,50.3967165455808,13.8634749112255));
#27295=CARTESIAN_POINT('',(15.5074469598942,33.9565603203064,-7.60754902620015E-30));
#27296=CARTESIAN_POINT('Origin',(16.2551894587641,35.5938999782222,0.));
#27297=CARTESIAN_POINT('Origin',(16.2551894587641,35.5938999782222,0.));
#27298=CARTESIAN_POINT('Ctrl Pts',(21.4269965203144,31.1388779521427,1.04083408558608E-14));
#27299=CARTESIAN_POINT('Ctrl Pts',(21.2467279061363,31.2547295558832,3.24562220582793));
#27300=CARTESIAN_POINT('Ctrl Pts',(21.8278019627956,32.5552534796889,6.16982677025168));
#27301=CARTESIAN_POINT('Ctrl Pts',(22.4088760194549,33.8557774034947,9.0940313346754));
#27302=CARTESIAN_POINT('Ctrl Pts',(23.6004994937372,36.1063347653243,11.1176436806954));
#27303=CARTESIAN_POINT('Ctrl Pts',(24.7921229680195,38.3568921271539,13.1412560267153));
#27304=CARTESIAN_POINT('Ctrl Pts',(26.322575806653,41.1346782711697,13.8634749112255));
#27305=CARTESIAN_POINT('Ctrl Pts',(27.8530286452863,43.9124644151855,14.5856937957357));
#27306=CARTESIAN_POINT('Ctrl Pts',(29.3834814839197,46.6902505592013,13.8634749112255));
#27307=CARTESIAN_POINT('Ctrl Pts',(22.9590519566757,32.9490709821973,0.));
#27308=CARTESIAN_POINT('Ctrl Pts',(22.7787833424976,33.0649225859378,2.70899372698069));
#27309=CARTESIAN_POINT('Ctrl Pts',(23.2339776345314,34.1695737726433,5.14971273833323));
#27310=CARTESIAN_POINT('Ctrl Pts',(23.6891719265652,35.2742249593487,7.59043174968578));
#27311=CARTESIAN_POINT('Ctrl Pts',(24.6539679027946,37.1718318447819,9.27946171175752));
#27312=CARTESIAN_POINT('Ctrl Pts',(25.6187638790239,39.069438730215,10.9684916738293));
#27313=CARTESIAN_POINT('Ctrl Pts',(26.866367454023,41.4071028290421,11.5712994880388));
#27314=CARTESIAN_POINT('Ctrl Pts',(28.1139710290221,43.7447669278692,12.1741073022483));
#27315=CARTESIAN_POINT('Ctrl Pts',(29.3615746040211,46.0824310266963,11.5712994880388));
#27316=CARTESIAN_POINT('Ctrl Pts',(24.8148246247012,34.4255873115186,0.));
#27317=CARTESIAN_POINT('Ctrl Pts',(24.6345560105231,34.5414389152591,2.19648874705822));
#27318=CARTESIAN_POINT('Ctrl Pts',(24.9695293139492,35.4590225922219,4.17545672685568));
#27319=CARTESIAN_POINT('Ctrl Pts',(25.3045026173754,36.3766062691846,6.15442470665313));
#27320=CARTESIAN_POINT('Ctrl Pts',(26.0526678575967,37.9371291496694,7.5239130403414));
#27321=CARTESIAN_POINT('Ctrl Pts',(26.8008330978182,39.4976520301542,8.89340137402967));
#27322=CARTESIAN_POINT('Ctrl Pts',(27.7783025634771,41.4149792500713,9.3821661014496));
#27323=CARTESIAN_POINT('Ctrl Pts',(28.755772029136,43.3323064699884,9.87093082886953));
#27324=CARTESIAN_POINT('Ctrl Pts',(29.7332414947948,45.2496336899055,9.3821661014496));
#27325=CARTESIAN_POINT('Ctrl Pts',(26.9229962078201,35.5116836434674,1.04083408558608E-14));
#27326=CARTESIAN_POINT('Ctrl Pts',(26.742727593642,35.6275352472079,1.72780310113343));
#27327=CARTESIAN_POINT('Ctrl Pts',(26.9677588400996,36.3740457442602,3.28449990511991));
#27328=CARTESIAN_POINT('Ctrl Pts',(27.1927900865572,37.1205562413125,4.84119670910639));
#27329=CARTESIAN_POINT('Ctrl Pts',(27.7428465855749,38.3728159033325,5.91846432228298));
#27330=CARTESIAN_POINT('Ctrl Pts',(28.2929030845927,39.6250755653525,6.99573193545956));
#27331=CARTESIAN_POINT('Ctrl Pts',(29.0233349906525,41.1580048392676,7.38020429521639));
#27332=CARTESIAN_POINT('Ctrl Pts',(29.7537668967123,42.6909341131828,7.76467665497322));
#27333=CARTESIAN_POINT('Ctrl Pts',(30.4841988027721,44.223863387098,7.38020429521639));
#27334=CARTESIAN_POINT('',(21.426996519931,31.1388779521943,-2.44187858986325E-9));
#27335=CARTESIAN_POINT('Origin',(35.1666259835204,19.5103534449749,0.));
#27336=CARTESIAN_POINT('Ctrl Pts',(21.4269965203144,31.1388779521427,1.04083408558608E-14));
#27337=CARTESIAN_POINT('Ctrl Pts',(21.2467279061363,31.2547295558832,3.24562220582793));
#27338=CARTESIAN_POINT('Ctrl Pts',(21.8278019627956,32.5552534796889,6.16982677025168));
#27339=CARTESIAN_POINT('Ctrl Pts',(22.3158165419708,33.6474974511925,8.62571762198519));
#27340=CARTESIAN_POINT('Ctrl Pts',(23.2474528526983,35.4345298797235,10.4701702229062));
#27341=CARTESIAN_POINT('Ctrl Pts',(21.118346831285,39.2421052839111,0.));
#27342=CARTESIAN_POINT('Ctrl Pts',(20.9380782171068,39.3579568876516,1.72780310113343));
#27343=CARTESIAN_POINT('Ctrl Pts',(21.1631094635644,40.1044673847039,3.28449990511991));
#27344=CARTESIAN_POINT('Ctrl Pts',(21.388140710022,40.8509778817562,4.84119670910638));
#27345=CARTESIAN_POINT('Ctrl Pts',(21.9381972090398,42.1032375437762,5.91846432228297));
#27346=CARTESIAN_POINT('Ctrl Pts',(22.4882537080575,43.3554972057961,6.99573193545955));
#27347=CARTESIAN_POINT('Ctrl Pts',(23.2186856141173,44.8884264797113,7.38020429521639));
#27348=CARTESIAN_POINT('Ctrl Pts',(23.9491175201772,46.4213557536265,7.76467665497322));
#27349=CARTESIAN_POINT('Ctrl Pts',(24.679549426237,47.9542850275417,7.38020429521639));
#27350=CARTESIAN_POINT('Ctrl Pts',(21.0061649833187,36.8732642383511,0.));
#27351=CARTESIAN_POINT('Ctrl Pts',(20.8258963691406,36.9891158420916,2.19648874705823));
#27352=CARTESIAN_POINT('Ctrl Pts',(21.1608696725667,37.9066995190544,4.17545672685568));
#27353=CARTESIAN_POINT('Ctrl Pts',(21.4958429759929,38.8242831960171,6.15442470665314));
#27354=CARTESIAN_POINT('Ctrl Pts',(22.2440082162142,40.3848060765019,7.5239130403414));
#27355=CARTESIAN_POINT('Ctrl Pts',(22.9921734564357,41.9453289569867,8.89340137402967));
#27356=CARTESIAN_POINT('Ctrl Pts',(23.9696429220946,43.8626561769038,9.38216610144961));
#27357=CARTESIAN_POINT('Ctrl Pts',(24.9471123877534,45.7799833968209,9.87093082886954));
#27358=CARTESIAN_POINT('Ctrl Pts',(25.9245818534123,47.697310616738,9.38216610144961));
#27359=CARTESIAN_POINT('Ctrl Pts',(20.433994315521,34.5718269932683,0.));
#27360=CARTESIAN_POINT('Ctrl Pts',(20.2537257013429,34.6876785970088,2.7089937269807));
#27361=CARTESIAN_POINT('Ctrl Pts',(20.7089199933767,35.7923297837142,5.14971273833323));
#27362=CARTESIAN_POINT('Ctrl Pts',(21.1641142854105,36.8969809704196,7.59043174968577));
#27363=CARTESIAN_POINT('Ctrl Pts',(22.1289102616398,38.7945878558528,9.27946171175751));
#27364=CARTESIAN_POINT('Ctrl Pts',(23.0937062378692,40.6921947412859,10.9684916738293));
#27365=CARTESIAN_POINT('Ctrl Pts',(24.3413098128683,43.029858840113,11.5712994880388));
#27366=CARTESIAN_POINT('Ctrl Pts',(25.5889133878673,45.3675229389401,12.1741073022483));
#27367=CARTESIAN_POINT('Ctrl Pts',(26.8365169628664,47.7051870377672,11.5712994880388));
#27368=CARTESIAN_POINT('Ctrl Pts',(19.4238236466312,32.4262389885811,0.));
#27369=CARTESIAN_POINT('Ctrl Pts',(19.243555032453,32.5420905923216,3.24562220582792));
#27370=CARTESIAN_POINT('Ctrl Pts',(19.8246290891124,33.8426145161273,6.16982677025167));
#27371=CARTESIAN_POINT('Ctrl Pts',(20.4057031457717,35.1431384399331,9.09403133467541));
#27372=CARTESIAN_POINT('Ctrl Pts',(21.597326620054,37.3936958017627,11.1176436806954));
#27373=CARTESIAN_POINT('Ctrl Pts',(22.7889500943363,39.6442531635923,13.1412560267153));
#27374=CARTESIAN_POINT('Ctrl Pts',(24.3194029329697,42.4220393076081,13.8634749112255));
#27375=CARTESIAN_POINT('Ctrl Pts',(25.8498557716031,45.1998254516239,14.5856937957357));
#27376=CARTESIAN_POINT('Ctrl Pts',(27.3803086102365,47.9776115956397,13.8634749112255));
#27377=CARTESIAN_POINT('',(19.4238236466312,32.4262389885811,0.));
#27378=CARTESIAN_POINT('Ctrl Pts',(19.4238236466312,32.4262389885811,0.));
#27379=CARTESIAN_POINT('Ctrl Pts',(19.243555032453,32.5420905923216,3.24562220582792));
#27380=CARTESIAN_POINT('Ctrl Pts',(19.8246290891124,33.8426145161273,6.16982677025167));
#27381=CARTESIAN_POINT('Ctrl Pts',(20.309731810084,34.9283413471511,8.61106394926976));
#27382=CARTESIAN_POINT('Ctrl Pts',(21.2335670650401,36.7013364119535,10.4489096280657));
#27383=CARTESIAN_POINT('Origin',(3.13849734404846,40.0935818932913,0.));
#27384=CARTESIAN_POINT('Ctrl Pts',(19.4238236466311,32.4262389885811,0.));
#27385=CARTESIAN_POINT('Ctrl Pts',(19.243555032453,32.5420905923216,3.24562220582792));
#27386=CARTESIAN_POINT('Ctrl Pts',(19.8246290891124,33.8426145161273,6.16982677025167));
#27387=CARTESIAN_POINT('Ctrl Pts',(20.4057031457717,35.1431384399331,9.09403133467541));
#27388=CARTESIAN_POINT('Ctrl Pts',(21.597326620054,37.3936958017627,11.1176436806954));
#27389=CARTESIAN_POINT('Ctrl Pts',(22.7889500943363,39.6442531635923,13.1412560267153));
#27390=CARTESIAN_POINT('Ctrl Pts',(24.3194029329697,42.4220393076081,13.8634749112255));
#27391=CARTESIAN_POINT('Ctrl Pts',(25.8498557716031,45.1998254516238,14.5856937957357));
#27392=CARTESIAN_POINT('Ctrl Pts',(27.3803086102365,47.9776115956397,13.8634749112255));
#27393=CARTESIAN_POINT('Ctrl Pts',(19.6841717937391,31.5100409519659,0.));
#27394=CARTESIAN_POINT('Ctrl Pts',(19.503903179561,31.6258925557065,3.38941559469373));
#27395=CARTESIAN_POINT('Ctrl Pts',(20.1187076077131,32.9789019620467,6.44317352589574));
#27396=CARTESIAN_POINT('Ctrl Pts',(20.7335120358652,34.331911368387,9.49693145709774));
#27397=CARTESIAN_POINT('Ctrl Pts',(21.9859155393831,36.6770443017775,11.6101975146502));
#27398=CARTESIAN_POINT('Ctrl Pts',(23.238319042901,39.022177235168,13.7234635722027));
#27399=CARTESIAN_POINT('Ctrl Pts',(24.8445633383045,41.9178971879301,14.4776794959001));
#27400=CARTESIAN_POINT('Ctrl Pts',(26.450807633708,44.8136171406923,15.2318954195974));
#27401=CARTESIAN_POINT('Ctrl Pts',(28.0570519291115,47.7093370934545,14.4776794959001));
#27402=CARTESIAN_POINT('Ctrl Pts',(20.4854409432124,30.9950965373906,0.));
#27403=CARTESIAN_POINT('Ctrl Pts',(20.3051723290343,31.1109481411311,3.38941559469372));
#27404=CARTESIAN_POINT('Ctrl Pts',(20.9199767571864,32.4639575474714,6.44317352589573));
#27405=CARTESIAN_POINT('Ctrl Pts',(21.5347811853385,33.8169669538117,9.49693145709774));
#27406=CARTESIAN_POINT('Ctrl Pts',(22.7871846888564,36.1620998872021,11.6101975146502));
#27407=CARTESIAN_POINT('Ctrl Pts',(24.0395881923743,38.5072328205926,13.7234635722027));
#27408=CARTESIAN_POINT('Ctrl Pts',(25.6458324877778,41.4029527733548,14.4776794959001));
#27409=CARTESIAN_POINT('Ctrl Pts',(27.2520767831814,44.298672726117,15.2318954195974));
#27410=CARTESIAN_POINT('Ctrl Pts',(28.8583210785848,47.1943926788791,14.4776794959001));
#27411=CARTESIAN_POINT('Ctrl Pts',(21.4269965203144,31.1388779521427,1.04083408558608E-14));
#27412=CARTESIAN_POINT('Ctrl Pts',(21.2467279061363,31.2547295558832,3.24562220582793));
#27413=CARTESIAN_POINT('Ctrl Pts',(21.8278019627956,32.555253479689,6.16982677025167));
#27414=CARTESIAN_POINT('Ctrl Pts',(22.4088760194549,33.8557774034947,9.0940313346754));
#27415=CARTESIAN_POINT('Ctrl Pts',(23.6004994937372,36.1063347653243,11.1176436806954));
#27416=CARTESIAN_POINT('Ctrl Pts',(24.7921229680195,38.3568921271539,13.1412560267153));
#27417=CARTESIAN_POINT('Ctrl Pts',(26.3225758066529,41.1346782711697,13.8634749112255));
#27418=CARTESIAN_POINT('Ctrl Pts',(27.8530286452863,43.9124644151855,14.5856937957357));
#27419=CARTESIAN_POINT('Ctrl Pts',(29.3834814839197,46.6902505592013,13.8634749112255));
#27420=CARTESIAN_POINT('',(20.182125900029,31.4039916914382,-5.03628278819837E-30));
#27421=CARTESIAN_POINT('Origin',(21.1552751870378,32.918250739684,0.));
#27422=CARTESIAN_POINT('Origin',(21.1552751870378,32.918250739684,0.));
#27423=CARTESIAN_POINT('Ctrl Pts',(25.6404249706861,27.7725495286735,0.));
#27424=CARTESIAN_POINT('Ctrl Pts',(25.4784786333245,27.9128768288047,3.24562220582793));
#27425=CARTESIAN_POINT('Ctrl Pts',(26.2387220458135,29.1174678338684,6.16982677025168));
#27426=CARTESIAN_POINT('Ctrl Pts',(26.9989654583026,30.3220588389322,9.09403133467542));
#27427=CARTESIAN_POINT('Ctrl Pts',(28.4987476307694,32.3801230698289,11.1176436806954));
#27428=CARTESIAN_POINT('Ctrl Pts',(29.9985298032362,34.4381873007258,13.1412560267153));
#27429=CARTESIAN_POINT('Ctrl Pts',(31.9087250245465,36.9698934388173,13.8634749112255));
#27430=CARTESIAN_POINT('Ctrl Pts',(33.8189202458568,39.5015995769089,14.5856937957357));
#27431=CARTESIAN_POINT('Ctrl Pts',(35.729115467167,42.0333057150005,13.8634749112255));
#27432=CARTESIAN_POINT('Ctrl Pts',(27.4145036200624,29.3462831821135,0.));
#27433=CARTESIAN_POINT('Ctrl Pts',(27.2525572827008,29.4866104822447,2.7089937269807));
#27434=CARTESIAN_POINT('Ctrl Pts',(27.860326608162,30.5152370105912,5.14971273833323));
#27435=CARTESIAN_POINT('Ctrl Pts',(28.4680959336233,31.5438635389378,7.59043174968578));
#27436=CARTESIAN_POINT('Ctrl Pts',(29.6931292949422,33.2848507390766,9.27946171175751));
#27437=CARTESIAN_POINT('Ctrl Pts',(30.9181626562612,35.0258379392154,10.9684916738292));
#27438=CARTESIAN_POINT('Ctrl Pts',(32.4857517139244,37.1621554871446,11.5712994880388));
#27439=CARTESIAN_POINT('Ctrl Pts',(34.0533407715877,39.2984730350737,12.1741073022483));
#27440=CARTESIAN_POINT('Ctrl Pts',(35.6209298292509,41.4347905830029,11.5712994880388));
#27441=CARTESIAN_POINT('Ctrl Pts',(29.4615173807458,30.543666717041,-1.05434036998093E-14));
#27442=CARTESIAN_POINT('Ctrl Pts',(29.2995710433842,30.6839940171721,2.19648874705823));
#27443=CARTESIAN_POINT('Ctrl Pts',(29.7617205741622,31.5445663438469,4.17545672685568));
#27444=CARTESIAN_POINT('Ctrl Pts',(30.2238701049403,32.4051386705216,6.15442470665314));
#27445=CARTESIAN_POINT('Ctrl Pts',(31.1865056631394,33.8433026630074,7.52391304034139));
#27446=CARTESIAN_POINT('Ctrl Pts',(32.1491412213385,35.2814666554933,8.89340137402967));
#27447=CARTESIAN_POINT('Ctrl Pts',(33.389525570451,37.0401698399469,9.3821661014496));
#27448=CARTESIAN_POINT('Ctrl Pts',(34.6299099195636,38.7988730244004,9.87093082886954));
#27449=CARTESIAN_POINT('Ctrl Pts',(35.8702942686761,40.557576208854,9.3821661014496));
#27450=CARTESIAN_POINT('Ctrl Pts',(31.7027984407115,31.3186840564482,0.));
#27451=CARTESIAN_POINT('Ctrl Pts',(31.5408521033499,31.4590113565794,1.72780310113342));
#27452=CARTESIAN_POINT('Ctrl Pts',(31.8698323768441,32.1658981677049,3.28449990511991));
#27453=CARTESIAN_POINT('Ctrl Pts',(32.1988126503383,32.8727849788304,4.84119670910639));
#27454=CARTESIAN_POINT('Ctrl Pts',(32.9214854985886,34.0340172414015,5.91846432228298));
#27455=CARTESIAN_POINT('Ctrl Pts',(33.6441583468389,35.1952495039725,6.99573193545956));
#27456=CARTESIAN_POINT('Ctrl Pts',(34.5853140909925,36.6086244696002,7.38020429521639));
#27457=CARTESIAN_POINT('Ctrl Pts',(35.526469835146,38.0219994352279,7.76467665497321));
#27458=CARTESIAN_POINT('Ctrl Pts',(36.4676255792996,39.4353744008555,7.38020429521639));
#27459=CARTESIAN_POINT('',(25.640424970796,27.7725495286968,1.57949969353625E-9));
#27460=CARTESIAN_POINT('Origin',(37.5852932322718,14.3070334890498,0.));
#27461=CARTESIAN_POINT('Ctrl Pts',(25.6404249705938,27.7725495288656,3.13107516801643E-9));
#27462=CARTESIAN_POINT('Ctrl Pts',(25.6281983378206,27.7831439665411,0.245038153335291));
#27463=CARTESIAN_POINT('Ctrl Pts',(25.6200142870521,27.7986217084842,0.490791160521329));
#27464=CARTESIAN_POINT('Ctrl Pts',(25.6159526330981,27.8190271851147,0.736766500724782));
#27465=CARTESIAN_POINT('Ctrl Pts',(25.6119043133259,27.8393656717115,0.98193431770045));
#27466=CARTESIAN_POINT('Ctrl Pts',(25.6119514551675,27.8645996505507,1.22732257376512));
#27467=CARTESIAN_POINT('Ctrl Pts',(25.6161410294536,27.8947338787561,1.47243294816291));
#27468=CARTESIAN_POINT('Ctrl Pts',(25.6203242940988,27.9248227237925,1.71717417802967));
#27469=CARTESIAN_POINT('Ctrl Pts',(25.6286375769735,27.9597970874095,1.96163791541537));
#27470=CARTESIAN_POINT('Ctrl Pts',(25.6410945477697,27.9996219245316,2.20532408778476));
#27471=CARTESIAN_POINT('Ctrl Pts',(25.6535408348301,28.039412605835,2.44880126242025));
#27472=CARTESIAN_POINT('Ctrl Pts',(25.670123717558,28.0840454126417,2.69150175431017));
#27473=CARTESIAN_POINT('Ctrl Pts',(25.690823271976,28.1334457426218,2.93292951866782));
#27474=CARTESIAN_POINT('Ctrl Pts',(25.711518496006,28.1828357379543,3.17430677585562));
#27475=CARTESIAN_POINT('Ctrl Pts',(25.7363286400399,28.2369911812591,3.41441139318315));
#27476=CARTESIAN_POINT('Ctrl Pts',(25.7652003562647,28.2957987052583,3.65275710614606));
#27477=CARTESIAN_POINT('Ctrl Pts',(25.7941087333335,28.3546809021119,3.89140546668757));
#27478=CARTESIAN_POINT('Ctrl Pts',(25.8270889373972,28.4182268780895,4.12829002081133));
#27479=CARTESIAN_POINT('Ctrl Pts',(25.8640546001339,28.4862854384143,4.36293874377776));
#27480=CARTESIAN_POINT('Ctrl Pts',(25.9010579825876,28.5544134456108,4.59782690201416));
#27481=CARTESIAN_POINT('Ctrl Pts',(25.9420548501735,28.6270630772619,4.83047425894926));
#27482=CARTESIAN_POINT('Ctrl Pts',(25.9869270447948,28.7040474659735,5.06042975959398));
#27483=CARTESIAN_POINT('Ctrl Pts',(26.0319304281239,28.7812569268608,5.29105755998273));
#27484=CARTESIAN_POINT('Ctrl Pts',(26.0808316886118,28.8628263193248,5.51897736305657));
#27485=CARTESIAN_POINT('Ctrl Pts',(26.1334818341726,28.9485346007072,5.74376259354302));
#27486=CARTESIAN_POINT('Ctrl Pts',(26.1670531325894,29.0031847495424,5.887092340726));
#27487=CARTESIAN_POINT('Ctrl Pts',(26.2021480259523,29.0595170057056,6.02914825314183));
#27488=CARTESIAN_POINT('Ctrl Pts',(26.2387220458403,29.1174678338915,6.16982677023483));
#27489=CARTESIAN_POINT('Ctrl Pts',(26.2960711849264,29.2083364372324,6.39041482339095));
#27490=CARTESIAN_POINT('Ctrl Pts',(26.3572486158602,29.3038406779897,6.60890054011815));
#27491=CARTESIAN_POINT('Ctrl Pts',(26.4221888209397,29.4038573838824,6.82480412008056));
#27492=CARTESIAN_POINT('Ctrl Pts',(26.4869824198613,29.5036482964479,7.04022028559305));
#27493=CARTESIAN_POINT('Ctrl Pts',(26.5555217851616,29.6079312382239,7.25306552029648));
#27494=CARTESIAN_POINT('Ctrl Pts',(26.6277100364536,29.7165449255437,7.46287566269426));
#27495=CARTESIAN_POINT('Ctrl Pts',(26.6997821794603,29.8249839175527,7.67234834441895));
#27496=CARTESIAN_POINT('Ctrl Pts',(26.7754914030015,29.9377396021008,7.87879526533046));
#27497=CARTESIAN_POINT('Ctrl Pts',(26.8547104088652,30.0546142350032,8.08177334612217));
#27498=CARTESIAN_POINT('Ctrl Pts',(26.9338534012421,30.1713767224897,8.28455666214139));
#27499=CARTESIAN_POINT('Ctrl Pts',(27.016499328435,30.2922500787582,8.48387739272888));
#27500=CARTESIAN_POINT('Ctrl Pts',(27.1024918458758,30.4170022653827,8.67931873611135));
#27501=CARTESIAN_POINT('Ctrl Pts',(27.1884884993292,30.5417604522572,8.87476947970517));
#27502=CARTESIAN_POINT('Ctrl Pts',(27.2778319154184,30.6703976233164,9.06634009532839));
#27503=CARTESIAN_POINT('Ctrl Pts',(27.3703382785463,30.8026498047317,9.25364450340979));
#27504=CARTESIAN_POINT('Ctrl Pts',(27.4628785767206,30.9349505015546,9.44101762226489));
#27505=CARTESIAN_POINT('Ctrl Pts',(27.5585839591973,31.0708686028433,9.62412107875024));
#27506=CARTESIAN_POINT('Ctrl Pts',(27.657245442894,31.2101115092137,9.80260437466114));
#27507=CARTESIAN_POINT('Ctrl Pts',(27.7560678639063,31.3495815496057,9.98137881379688));
#27508=CARTESIAN_POINT('Ctrl Pts',(27.8578558275202,31.4923869622811,10.1555177270927));
#27509=CARTESIAN_POINT('Ctrl Pts',(27.9623772429055,31.638209399578,10.3247095747713));
#27510=CARTESIAN_POINT('Ctrl Pts',(27.9925874699275,31.6803570199426,10.3736117457742));
#27511=CARTESIAN_POINT('Ctrl Pts',(28.0230259217659,31.7227565449012,10.4221009095725));
#27512=CARTESIAN_POINT('Ctrl Pts',(28.0536866918396,31.7653999649233,10.4701702229062));
#27513=CARTESIAN_POINT('Ctrl Pts',(26.4881263776672,35.8372231206707,0.));
#27514=CARTESIAN_POINT('Ctrl Pts',(26.3261800403055,35.9775504208019,1.72780310113343));
#27515=CARTESIAN_POINT('Ctrl Pts',(26.6551603137998,36.6844372319274,3.28449990511992));
#27516=CARTESIAN_POINT('Ctrl Pts',(26.984140587294,37.3913240430529,4.84119670910639));
#27517=CARTESIAN_POINT('Ctrl Pts',(27.7068134355443,38.552556305624,5.91846432228299));
#27518=CARTESIAN_POINT('Ctrl Pts',(28.4294862837945,39.7137885681951,6.99573193545956));
#27519=CARTESIAN_POINT('Ctrl Pts',(29.3706420279481,41.1271635338227,7.3802042952164));
#27520=CARTESIAN_POINT('Ctrl Pts',(30.3117977721017,42.5405384994504,7.76467665497322));
#27521=CARTESIAN_POINT('Ctrl Pts',(31.2529535162552,43.953913465078,7.38020429521639));
#27522=CARTESIAN_POINT('Ctrl Pts',(26.0399651488663,33.5084586029184,0.));
#27523=CARTESIAN_POINT('Ctrl Pts',(25.8780188115047,33.6487859030495,2.19648874705823));
#27524=CARTESIAN_POINT('Ctrl Pts',(26.3401683422827,34.5093582297243,4.17545672685568));
#27525=CARTESIAN_POINT('Ctrl Pts',(26.8023178730608,35.369930556399,6.15442470665314));
#27526=CARTESIAN_POINT('Ctrl Pts',(27.7649534312599,36.8080945488848,7.5239130403414));
#27527=CARTESIAN_POINT('Ctrl Pts',(28.727588989459,38.2462585413707,8.89340137402969));
#27528=CARTESIAN_POINT('Ctrl Pts',(29.9679733385715,40.0049617258242,9.38216610144961));
#27529=CARTESIAN_POINT('Ctrl Pts',(31.208357687684,41.7636649102778,9.87093082886954));
#27530=CARTESIAN_POINT('Ctrl Pts',(32.4487420367966,43.5223680947314,9.3821661014496));
#27531=CARTESIAN_POINT('Ctrl Pts',(25.1460896841347,31.3118750466443,0.));
#27532=CARTESIAN_POINT('Ctrl Pts',(24.9841433467731,31.4522023467755,2.70899372698069));
#27533=CARTESIAN_POINT('Ctrl Pts',(25.5919126722344,32.480828875122,5.14971273833323));
#27534=CARTESIAN_POINT('Ctrl Pts',(26.1996819976956,33.5094554034686,7.59043174968577));
#27535=CARTESIAN_POINT('Ctrl Pts',(27.4247153590146,35.2504426036074,9.27946171175751));
#27536=CARTESIAN_POINT('Ctrl Pts',(28.6497487203335,36.9914298037462,10.9684916738293));
#27537=CARTESIAN_POINT('Ctrl Pts',(30.2173377779967,39.1277473516754,11.5712994880388));
#27538=CARTESIAN_POINT('Ctrl Pts',(31.78492683566,41.2640648996045,12.1741073022483));
#27539=CARTESIAN_POINT('Ctrl Pts',(33.3525158933232,43.4003824475337,11.5712994880388));
#27540=CARTESIAN_POINT('Ctrl Pts',(23.8408520862202,29.3318883095339,0.));
#27541=CARTESIAN_POINT('Ctrl Pts',(23.6789057488586,29.4722156096651,3.24562220582793));
#27542=CARTESIAN_POINT('Ctrl Pts',(24.4391491613477,30.6768066147289,6.16982677025167));
#27543=CARTESIAN_POINT('Ctrl Pts',(25.1993925738368,31.8813976197927,9.09403133467541));
#27544=CARTESIAN_POINT('Ctrl Pts',(26.6991747463036,33.9394618506894,11.1176436806954));
#27545=CARTESIAN_POINT('Ctrl Pts',(28.1989569187704,35.9975260815862,13.1412560267153));
#27546=CARTESIAN_POINT('Ctrl Pts',(30.1091521400807,38.5292322196778,13.8634749112255));
#27547=CARTESIAN_POINT('Ctrl Pts',(32.0193473613909,41.0609383577694,14.5856937957357));
#27548=CARTESIAN_POINT('Ctrl Pts',(33.9295425827012,43.592644495861,13.8634749112255));
#27549=CARTESIAN_POINT('',(23.8408520862202,29.3318883095339,0.));
#27550=CARTESIAN_POINT('Ctrl Pts',(23.8408520862202,29.3318883095339,0.));
#27551=CARTESIAN_POINT('Ctrl Pts',(23.6789057488586,29.4722156096651,3.24562220582793));
#27552=CARTESIAN_POINT('Ctrl Pts',(24.4391491613477,30.6768066147289,6.16982677025167));
#27553=CARTESIAN_POINT('Ctrl Pts',(25.0738292744463,31.6824449968206,8.61106394926976));
#27554=CARTESIAN_POINT('Ctrl Pts',(26.240584724474,33.3059180634109,10.4489096280657));
#27555=CARTESIAN_POINT('Origin',(8.81246358936599,39.2388322978494,0.));
#27556=CARTESIAN_POINT('Ctrl Pts',(23.8408520862202,29.3318883095339,0.));
#27557=CARTESIAN_POINT('Ctrl Pts',(23.6789057488586,29.4722156096651,3.24562220582793));
#27558=CARTESIAN_POINT('Ctrl Pts',(24.4391491613477,30.6768066147289,6.16982677025167));
#27559=CARTESIAN_POINT('Ctrl Pts',(25.1993925738368,31.8813976197927,9.09403133467541));
#27560=CARTESIAN_POINT('Ctrl Pts',(26.6991747463036,33.9394618506894,11.1176436806954));
#27561=CARTESIAN_POINT('Ctrl Pts',(28.1989569187704,35.9975260815862,13.1412560267153));
#27562=CARTESIAN_POINT('Ctrl Pts',(30.1091521400807,38.5292322196778,13.8634749112255));
#27563=CARTESIAN_POINT('Ctrl Pts',(32.0193473613909,41.0609383577694,14.5856937957357));
#27564=CARTESIAN_POINT('Ctrl Pts',(33.9295425827012,43.592644495861,13.8634749112255));
#27565=CARTESIAN_POINT('Ctrl Pts',(23.9681616891744,28.3879644434326,0.));
#27566=CARTESIAN_POINT('Ctrl Pts',(23.8062153518128,28.5282917435638,3.38941559469372));
#27567=CARTESIAN_POINT('Ctrl Pts',(24.6073152722067,29.7800336722638,6.44317352589573));
#27568=CARTESIAN_POINT('Ctrl Pts',(25.4084151926006,31.0317756009639,9.49693145709774));
#27569=CARTESIAN_POINT('Ctrl Pts',(26.9818182484142,33.1748028604388,11.6101975146502));
#27570=CARTESIAN_POINT('Ctrl Pts',(28.5552213042278,35.3178301199138,13.7234635722027));
#27571=CARTESIAN_POINT('Ctrl Pts',(30.5572202654792,37.9554834217125,14.4776794959001));
#27572=CARTESIAN_POINT('Ctrl Pts',(32.5592192267306,40.5931367235112,15.2318954195974));
#27573=CARTESIAN_POINT('Ctrl Pts',(34.5612181879821,43.2307900253099,14.4776794959001));
#27574=CARTESIAN_POINT('Ctrl Pts',(24.6879908429608,27.7642289310884,0.));
#27575=CARTESIAN_POINT('Ctrl Pts',(24.5260445055992,27.9045562312196,3.38941559469372));
#27576=CARTESIAN_POINT('Ctrl Pts',(25.327144425993,29.1562981599196,6.44317352589574));
#27577=CARTESIAN_POINT('Ctrl Pts',(26.1282443463869,30.4080400886197,9.49693145709774));
#27578=CARTESIAN_POINT('Ctrl Pts',(27.7016474022005,32.5510673480946,11.6101975146502));
#27579=CARTESIAN_POINT('Ctrl Pts',(29.2750504580142,34.6940946075696,13.7234635722027));
#27580=CARTESIAN_POINT('Ctrl Pts',(31.2770494192656,37.3317479093683,14.4776794959001));
#27581=CARTESIAN_POINT('Ctrl Pts',(33.279048380517,39.969401211167,15.2318954195974));
#27582=CARTESIAN_POINT('Ctrl Pts',(35.2810473417684,42.6070545129657,14.4776794959001));
#27583=CARTESIAN_POINT('Ctrl Pts',(25.6404249706861,27.7725495286735,0.));
#27584=CARTESIAN_POINT('Ctrl Pts',(25.4784786333245,27.9128768288047,3.24562220582793));
#27585=CARTESIAN_POINT('Ctrl Pts',(26.2387220458135,29.1174678338684,6.16982677025167));
#27586=CARTESIAN_POINT('Ctrl Pts',(26.9989654583026,30.3220588389322,9.09403133467541));
#27587=CARTESIAN_POINT('Ctrl Pts',(28.4987476307694,32.380123069829,11.1176436806954));
#27588=CARTESIAN_POINT('Ctrl Pts',(29.9985298032362,34.4381873007258,13.1412560267153));
#27589=CARTESIAN_POINT('Ctrl Pts',(31.9087250245465,36.9698934388173,13.8634749112255));
#27590=CARTESIAN_POINT('Ctrl Pts',(33.8189202458568,39.5015995769089,14.5856937957357));
#27591=CARTESIAN_POINT('Ctrl Pts',(35.729115467167,42.0333057150005,13.8634749112255));
#27592=CARTESIAN_POINT('',(24.4459549573234,28.2121283533352,-2.36249235658883E-30));
#27593=CARTESIAN_POINT('Origin',(25.6247005192793,29.572480844482,0.));
#27594=CARTESIAN_POINT('Origin',(25.6247005192793,29.572480844482,0.));
#27595=CARTESIAN_POINT('Ctrl Pts',(29.3318883095343,23.8408520862197,0.));
#27596=CARTESIAN_POINT('Ctrl Pts',(29.1915610094032,24.0027984235813,3.24562220582793));
#27597=CARTESIAN_POINT('Ctrl Pts',(30.1154974142047,25.0869345107937,6.16982677025167));
#27598=CARTESIAN_POINT('Ctrl Pts',(31.0394338190063,26.171070598006,9.09403133467541));
#27599=CARTESIAN_POINT('Ctrl Pts',(32.8168434496408,27.994745445196,11.1176436806954));
#27600=CARTESIAN_POINT('Ctrl Pts',(34.5942530802753,29.8184202923861,13.1412560267153));
#27601=CARTESIAN_POINT('Ctrl Pts',(36.8453046181047,32.0525081884195,13.8634749112255));
#27602=CARTESIAN_POINT('Ctrl Pts',(39.0963561559341,34.286596084453,14.5856937957357));
#27603=CARTESIAN_POINT('Ctrl Pts',(41.3474076937634,36.5206839804864,13.8634749112255));
#27604=CARTESIAN_POINT('Ctrl Pts',(31.3118750466448,25.1460896841342,0.));
#27605=CARTESIAN_POINT('Ctrl Pts',(31.1715477465136,25.3080360214958,2.7089937269807));
#27606=CARTESIAN_POINT('Ctrl Pts',(31.9195196745979,26.2396980216803,5.14971273833323));
#27607=CARTESIAN_POINT('Ctrl Pts',(32.6674916026822,27.1713600218648,7.59043174968577));
#27608=CARTESIAN_POINT('Ctrl Pts',(34.1278242025588,28.720286057907,9.27946171175751));
#27609=CARTESIAN_POINT('Ctrl Pts',(35.5881568024354,30.2692120939491,10.9684916738293));
#27610=CARTESIAN_POINT('Ctrl Pts',(37.4438197501023,32.1606938263356,11.5712994880388));
#27611=CARTESIAN_POINT('Ctrl Pts',(39.2994826977692,34.052175558722,12.1741073022483));
#27612=CARTESIAN_POINT('Ctrl Pts',(41.1551456454362,35.9436572911085,11.5712994880388));
#27613=CARTESIAN_POINT('Ctrl Pts',(33.5084586029188,26.0399651488657,-1.05434036998093E-14));
#27614=CARTESIAN_POINT('Ctrl Pts',(33.3681313027877,26.2019114862273,2.19648874705823));
#27615=CARTESIAN_POINT('Ctrl Pts',(33.9480490292002,26.9879536917286,4.17545672685568));
#27616=CARTESIAN_POINT('Ctrl Pts',(34.5279667556127,27.7739958972299,6.15442470665314));
#27617=CARTESIAN_POINT('Ctrl Pts',(35.6854761478363,29.0605241301522,7.5239130403414));
#27618=CARTESIAN_POINT('Ctrl Pts',(36.8429855400598,30.3470523630746,8.89340137402968));
#27619=CARTESIAN_POINT('Ctrl Pts',(38.3210341242512,31.9113293869104,9.38216610144961));
#27620=CARTESIAN_POINT('Ctrl Pts',(39.7990827084425,33.4756064107461,9.87093082886955));
#27621=CARTESIAN_POINT('Ctrl Pts',(41.2771312926339,35.0398834345819,9.38216610144961));
#27622=CARTESIAN_POINT('Ctrl Pts',(35.8372231206712,26.4881263776665,0.));
#27623=CARTESIAN_POINT('Ctrl Pts',(35.6968958205401,26.6500727150282,1.72780310113343));
#27624=CARTESIAN_POINT('Ctrl Pts',(36.1231280314034,27.3029456632456,3.28449990511992));
#27625=CARTESIAN_POINT('Ctrl Pts',(36.5493602422666,27.9558186114631,4.84119670910638));
#27626=CARTESIAN_POINT('Ctrl Pts',(37.4299379045754,29.0023841344366,5.91846432228298));
#27627=CARTESIAN_POINT('Ctrl Pts',(38.3105155668842,30.0489496574101,6.99573193545956));
#27628=CARTESIAN_POINT('Ctrl Pts',(39.4432359322497,31.3139980762869,7.38020429521639));
#27629=CARTESIAN_POINT('Ctrl Pts',(40.5759562976151,32.5790464951637,7.76467665497322));
#27630=CARTESIAN_POINT('Ctrl Pts',(41.7086766629805,33.8440949140405,7.38020429521639));
#27631=CARTESIAN_POINT('',(29.3318883095548,23.8408520862335,1.57950172528022E-9));
#27632=CARTESIAN_POINT('Origin',(39.2388322978496,8.81246358936532,0.));
#27633=CARTESIAN_POINT('Ctrl Pts',(29.3318883094704,23.840852086423,3.1310780077989E-9));
#27634=CARTESIAN_POINT('Ctrl Pts',(29.3212938718738,23.8530787192646,0.245038153335593));
#27635=CARTESIAN_POINT('Ctrl Pts',(29.3153958352832,23.8695636319733,0.490791160521933));
#27636=CARTESIAN_POINT('Ctrl Pts',(29.3142795252166,23.8903394438997,0.736766500725686));
#27637=CARTESIAN_POINT('Ctrl Pts',(29.3131668799332,23.9110470500023,0.981934317701342));
#27638=CARTESIAN_POINT('Ctrl Pts',(29.3168047115563,23.9360174743377,1.227322573766));
#27639=CARTESIAN_POINT('Ctrl Pts',(29.3252401898306,23.965248740963,1.47243294816377));
#27640=CARTESIAN_POINT('Ctrl Pts',(29.3336629639887,23.9944359843101,1.71717417803053));
#27641=CARTESIAN_POINT('Ctrl Pts',(29.3468690005324,24.0278712558265,1.96163791541622));
#27642=CARTESIAN_POINT('Ctrl Pts',(29.3648668425816,24.0655179217451,2.2053240877856));
#27643=CARTESIAN_POINT('Ctrl Pts',(29.3828492487603,24.1031322999562,2.44880126242104));
#27644=CARTESIAN_POINT('Ctrl Pts',(29.4056152523349,24.1449508188713,2.6915017543109));
#27645=CARTESIAN_POINT('Ctrl Pts',(29.4331345151071,24.1909024709822,2.9329295186685));
#27646=CARTESIAN_POINT('Ctrl Pts',(29.4606480207945,24.2368445099158,3.17430677585634));
#27647=CARTESIAN_POINT('Ctrl Pts',(29.492912756491,24.2869178772579,3.41441139318391));
#27648=CARTESIAN_POINT('Ctrl Pts',(29.5298597835414,24.341017951831,3.65275710614686));
#27649=CARTESIAN_POINT('Ctrl Pts',(29.5668537253365,24.3951867218145,3.89140546668843));
#27650=CARTESIAN_POINT('Ctrl Pts',(29.6085417737706,24.4533923189748,4.12829002081224));
#27651=CARTESIAN_POINT('Ctrl Pts',(29.6548169223665,24.5154973789738,4.36293874377873));
#27652=CARTESIAN_POINT('Ctrl Pts',(29.7011392900673,24.5776658109,4.59782690201513));
#27653=CARTESIAN_POINT('Ctrl Pts',(29.7520579892329,24.6437415114729,4.83047425895023));
#27654=CARTESIAN_POINT('Ctrl Pts',(29.8074294704424,24.7135563309893,5.06042975959494));
#27655=CARTESIAN_POINT('Ctrl Pts',(29.862962836158,24.7835752616714,5.29105755998378));
#27656=CARTESIAN_POINT('Ctrl Pts',(29.9229748872206,24.8573550203558,5.51897736305772));
#27657=CARTESIAN_POINT('Ctrl Pts',(29.9872866904184,24.9346980180644,5.74376259354425));
#27658=CARTESIAN_POINT('Ctrl Pts',(30.0282938085162,24.9840142132784,5.88709234072681));
#27659=CARTESIAN_POINT('Ctrl Pts',(30.0710484023926,25.034778564225,6.02914825314223));
#27660=CARTESIAN_POINT('Ctrl Pts',(30.1154974142345,25.0869345108127,6.16982677023484));
#27661=CARTESIAN_POINT('Ctrl Pts',(30.185194772364,25.1687165693392,6.39041482339089));
#27662=CARTESIAN_POINT('Ctrl Pts',(30.2593411758391,25.2545422584419,6.60890054011803));
#27663=CARTESIAN_POINT('Ctrl Pts',(30.3378542445907,25.3442989836975,6.82480412008038));
#27664=CARTESIAN_POINT('Ctrl Pts',(30.4161900656828,25.433853078108,7.04022028559285));
#27665=CARTESIAN_POINT('Ctrl Pts',(30.4988728090635,25.5273204012122,7.25306552029626));
#27666=CARTESIAN_POINT('Ctrl Pts',(30.5857836273893,25.6245550984952,7.46287566269403));
#27667=CARTESIAN_POINT('Ctrl Pts',(30.6725546575099,25.7216334025456,7.67234834441864));
#27668=CARTESIAN_POINT('Ctrl Pts',(30.76354007733,25.8224668509012,7.87879526533008));
#27669=CARTESIAN_POINT('Ctrl Pts',(30.858585742418,25.9268778285522,8.08177334612172));
#27670=CARTESIAN_POINT('Ctrl Pts',(30.9535402077704,26.0311886201132,8.28455666214105));
#27671=CARTESIAN_POINT('Ctrl Pts',(31.052546990739,26.1390699181376,8.48387739272866));
#27672=CARTESIAN_POINT('Ctrl Pts',(31.1554183156071,26.2503142961678,8.67931873611123));
#27673=CARTESIAN_POINT('Ctrl Pts',(31.2582945883135,26.3615640247581,8.87476947970508));
#27674=CARTESIAN_POINT('Ctrl Pts',(31.3650355954447,26.4761769610839,9.06634009532832));
#27675=CARTESIAN_POINT('Ctrl Pts',(31.4754218249885,26.5939179778765,9.25364450340974));
#27676=CARTESIAN_POINT('Ctrl Pts',(31.5858485486312,26.711702186799,9.44101762226468));
#27677=CARTESIAN_POINT('Ctrl Pts',(31.6999229509133,26.8326165417651,9.62412107874988));
#27678=CARTESIAN_POINT('Ctrl Pts',(31.8173965346648,26.9564011630242,9.80260437466064));
#27679=CARTESIAN_POINT('Ctrl Pts',(31.9350617421636,27.08038770264,9.98137881379626));
#27680=CARTESIAN_POINT('Ctrl Pts',(32.0561369802834,27.2072536245427,10.155517727092));
#27681=CARTESIAN_POINT('Ctrl Pts',(32.1803472149479,27.3367168513598,10.3247095747704));
#27682=CARTESIAN_POINT('Ctrl Pts',(32.2162481771956,27.3741361061496,10.3736117457753));
#27683=CARTESIAN_POINT('Ctrl Pts',(32.2524108910217,27.41177222173,10.4221009095756));
#27684=CARTESIAN_POINT('Ctrl Pts',(32.2888283700906,27.4496181106902,10.4701702229111));
#27685=CARTESIAN_POINT('Ctrl Pts',(31.3186840564488,31.702798440711,0.));
#27686=CARTESIAN_POINT('Ctrl Pts',(31.1783567563176,31.8647447780726,1.72780310113343));
#27687=CARTESIAN_POINT('Ctrl Pts',(31.6045889671809,32.51761772629,3.28449990511991));
#27688=CARTESIAN_POINT('Ctrl Pts',(32.0308211780442,33.1704906745075,4.84119670910638));
#27689=CARTESIAN_POINT('Ctrl Pts',(32.911398840353,34.217056197481,5.91846432228298));
#27690=CARTESIAN_POINT('Ctrl Pts',(33.7919765026618,35.2636217204545,6.99573193545956));
#27691=CARTESIAN_POINT('Ctrl Pts',(34.9246968680272,36.5286701393313,7.38020429521639));
#27692=CARTESIAN_POINT('Ctrl Pts',(36.0574172333927,37.7937185582081,7.76467665497322));
#27693=CARTESIAN_POINT('Ctrl Pts',(37.1901375987581,39.0587669770849,7.38020429521639));
#27694=CARTESIAN_POINT('Ctrl Pts',(30.5436667170415,29.4615173807453,0.));
#27695=CARTESIAN_POINT('Ctrl Pts',(30.4033394169104,29.6234637181069,2.19648874705824));
#27696=CARTESIAN_POINT('Ctrl Pts',(30.9832571433228,30.4095059236082,4.17545672685568));
#27697=CARTESIAN_POINT('Ctrl Pts',(31.5631748697354,31.1955481291095,6.15442470665314));
#27698=CARTESIAN_POINT('Ctrl Pts',(32.7206842619589,32.4820763620318,7.5239130403414));
#27699=CARTESIAN_POINT('Ctrl Pts',(33.8781936541825,33.7686045949542,8.89340137402967));
#27700=CARTESIAN_POINT('Ctrl Pts',(35.3562422383739,35.3328816187899,9.3821661014496));
#27701=CARTESIAN_POINT('Ctrl Pts',(36.8342908225652,36.8971586426257,9.87093082886954));
#27702=CARTESIAN_POINT('Ctrl Pts',(38.3123394067565,38.4614356664615,9.3821661014496));
#27703=CARTESIAN_POINT('Ctrl Pts',(29.346283182114,27.4145036200619,0.));
#27704=CARTESIAN_POINT('Ctrl Pts',(29.2059558819829,27.5764499574235,2.7089937269807));
#27705=CARTESIAN_POINT('Ctrl Pts',(29.9539278100672,28.508111957608,5.14971273833323));
#27706=CARTESIAN_POINT('Ctrl Pts',(30.7018997381515,29.4397739577925,7.59043174968578));
#27707=CARTESIAN_POINT('Ctrl Pts',(32.1622323380281,30.9886999938347,9.27946171175752));
#27708=CARTESIAN_POINT('Ctrl Pts',(33.6225649379047,32.5376260298769,10.9684916738293));
#27709=CARTESIAN_POINT('Ctrl Pts',(35.4782278855716,34.4291077622633,11.5712994880388));
#27710=CARTESIAN_POINT('Ctrl Pts',(37.3338908332385,36.3205894946498,12.1741073022483));
#27711=CARTESIAN_POINT('Ctrl Pts',(39.1895537809054,38.2120712270362,11.5712994880388));
#27712=CARTESIAN_POINT('Ctrl Pts',(27.7725495286739,25.6404249706856,0.));
#27713=CARTESIAN_POINT('Ctrl Pts',(27.6322222285428,25.8023713080472,3.24562220582792));
#27714=CARTESIAN_POINT('Ctrl Pts',(28.5561586333444,26.8865073952596,6.16982677025168));
#27715=CARTESIAN_POINT('Ctrl Pts',(29.4800950381459,27.9706434824719,9.09403133467541));
#27716=CARTESIAN_POINT('Ctrl Pts',(31.2575046687804,29.7943183296619,11.1176436806954));
#27717=CARTESIAN_POINT('Ctrl Pts',(33.0349142994149,31.6179931768519,13.1412560267153));
#27718=CARTESIAN_POINT('Ctrl Pts',(35.2859658372443,33.8520810728854,13.8634749112255));
#27719=CARTESIAN_POINT('Ctrl Pts',(37.5370173750737,36.0861689689189,14.5856937957357));
#27720=CARTESIAN_POINT('Ctrl Pts',(39.7880689129031,38.3202568649523,13.8634749112255));
#27721=CARTESIAN_POINT('',(27.7725495286739,25.6404249706856,0.));
#27722=CARTESIAN_POINT('Ctrl Pts',(27.7725495286739,25.6404249706856,0.));
#27723=CARTESIAN_POINT('Ctrl Pts',(27.6322222285428,25.8023713080473,3.24562220582792));
#27724=CARTESIAN_POINT('Ctrl Pts',(28.5561586333444,26.8865073952596,6.16982677025168));
#27725=CARTESIAN_POINT('Ctrl Pts',(29.3274958817336,27.7915854309815,8.61106394926976));
#27726=CARTESIAN_POINT('Ctrl Pts',(30.7134197505153,29.2324872694336,10.4489096280657));
#27727=CARTESIAN_POINT('Origin',(14.3070334890505,37.5852932322716,0.));
#27728=CARTESIAN_POINT('Ctrl Pts',(27.7725495286739,25.6404249706856,0.));
#27729=CARTESIAN_POINT('Ctrl Pts',(27.6322222285428,25.8023713080473,3.24562220582792));
#27730=CARTESIAN_POINT('Ctrl Pts',(28.5561586333444,26.8865073952596,6.16982677025168));
#27731=CARTESIAN_POINT('Ctrl Pts',(29.4800950381459,27.9706434824719,9.09403133467541));
#27732=CARTESIAN_POINT('Ctrl Pts',(31.2575046687804,29.7943183296619,11.1176436806954));
#27733=CARTESIAN_POINT('Ctrl Pts',(33.0349142994149,31.6179931768519,13.1412560267153));
#27734=CARTESIAN_POINT('Ctrl Pts',(35.2859658372443,33.8520810728854,13.8634749112255));
#27735=CARTESIAN_POINT('Ctrl Pts',(37.5370173750737,36.0861689689189,14.5856937957357));
#27736=CARTESIAN_POINT('Ctrl Pts',(39.7880689129031,38.3202568649523,13.8634749112255));
#27737=CARTESIAN_POINT('Ctrl Pts',(27.7642289310889,24.6879908429603,0.));
#27738=CARTESIAN_POINT('Ctrl Pts',(27.6239016309577,24.8499371803219,3.38941559469372));
#27739=CARTESIAN_POINT('Ctrl Pts',(28.5949889593955,25.974929775439,6.44317352589573));
#27740=CARTESIAN_POINT('Ctrl Pts',(29.5660762878334,27.0999223705561,9.49693145709776));
#27741=CARTESIAN_POINT('Ctrl Pts',(31.4284489470461,28.997218101093,11.6101975146502));
#27742=CARTESIAN_POINT('Ctrl Pts',(33.2908216062588,30.8945138316298,13.7234635722027));
#27743=CARTESIAN_POINT('Ctrl Pts',(35.6478203077953,33.2204054676045,14.4776794959001));
#27744=CARTESIAN_POINT('Ctrl Pts',(38.0048190093318,35.5462971035791,15.2318954195974));
#27745=CARTESIAN_POINT('Ctrl Pts',(40.3618177108683,37.8721887395537,14.4776794959001));
#27746=CARTESIAN_POINT('Ctrl Pts',(28.387964443433,23.9681616891739,0.));
#27747=CARTESIAN_POINT('Ctrl Pts',(28.2476371433019,24.1301080265356,3.38941559469372));
#27748=CARTESIAN_POINT('Ctrl Pts',(29.2187244717397,25.2551006216527,6.44317352589573));
#27749=CARTESIAN_POINT('Ctrl Pts',(30.1898118001775,26.3800932167698,9.49693145709775));
#27750=CARTESIAN_POINT('Ctrl Pts',(32.0521844593903,28.2773889473066,11.6101975146502));
#27751=CARTESIAN_POINT('Ctrl Pts',(33.914557118603,30.1746846778435,13.7234635722027));
#27752=CARTESIAN_POINT('Ctrl Pts',(36.2715558201394,32.5005763138181,14.4776794959001));
#27753=CARTESIAN_POINT('Ctrl Pts',(38.6285545216759,34.8264679497928,15.2318954195974));
#27754=CARTESIAN_POINT('Ctrl Pts',(40.9855532232124,37.1523595857673,14.4776794959001));
#27755=CARTESIAN_POINT('Ctrl Pts',(29.3318883095343,23.8408520862197,0.));
#27756=CARTESIAN_POINT('Ctrl Pts',(29.1915610094032,24.0027984235813,3.24562220582793));
#27757=CARTESIAN_POINT('Ctrl Pts',(30.1154974142047,25.0869345107937,6.16982677025167));
#27758=CARTESIAN_POINT('Ctrl Pts',(31.0394338190063,26.171070598006,9.09403133467541));
#27759=CARTESIAN_POINT('Ctrl Pts',(32.8168434496408,27.994745445196,11.1176436806954));
#27760=CARTESIAN_POINT('Ctrl Pts',(34.5942530802753,29.8184202923861,13.1412560267153));
#27761=CARTESIAN_POINT('Ctrl Pts',(36.8453046181047,32.0525081884195,13.8634749112255));
#27762=CARTESIAN_POINT('Ctrl Pts',(39.0963561559341,34.286596084453,14.5856937957357));
#27763=CARTESIAN_POINT('Ctrl Pts',(41.3474076937634,36.5206839804864,13.8634749112255));
#27764=CARTESIAN_POINT('',(28.2121348679648,24.44594743904,3.59391606952161E-31));
#27765=CARTESIAN_POINT('Origin',(29.5724808444824,25.6247005192788,0.));
#27766=CARTESIAN_POINT('Origin',(29.5724808444824,25.6247005192788,0.));
#27767=CARTESIAN_POINT('Ctrl Pts',(32.4262389885814,19.4238236466306,1.04083408558608E-14));
#27768=CARTESIAN_POINT('Ctrl Pts',(32.310387384841,19.6040922608087,3.24562220582793));
#27769=CARTESIAN_POINT('Ctrl Pts',(33.3792081011658,20.5457035458242,6.16982677025168));
#27770=CARTESIAN_POINT('Ctrl Pts',(34.4480288174906,21.4873148308397,9.09403133467541));
#27771=CARTESIAN_POINT('Ctrl Pts',(36.4668829718392,23.0394755334782,11.1176436806954));
#27772=CARTESIAN_POINT('Ctrl Pts',(38.4857371261878,24.5916362361167,13.1412560267153));
#27773=CARTESIAN_POINT('Ctrl Pts',(41.0318200627227,26.4826263031063,13.8634749112255));
#27774=CARTESIAN_POINT('Ctrl Pts',(43.5779029992576,28.3736163700958,14.5856937957357));
#27775=CARTESIAN_POINT('Ctrl Pts',(46.1239859357924,30.2646064370854,13.8634749112255));
#27776=CARTESIAN_POINT('Ctrl Pts',(34.5718269932686,20.4339943155204,0.));
#27777=CARTESIAN_POINT('Ctrl Pts',(34.4559753895281,20.6142629296985,2.70899372698069));
#27778=CARTESIAN_POINT('Ctrl Pts',(35.3289233687526,21.4299944500885,5.14971273833323));
#27779=CARTESIAN_POINT('Ctrl Pts',(36.2018713479771,22.2457259704785,7.59043174968577));
#27780=CARTESIAN_POINT('Ctrl Pts',(37.8677750259293,23.571059175064,9.27946171175751));
#27781=CARTESIAN_POINT('Ctrl Pts',(39.5336787038815,24.8963923796496,10.9684916738292));
#27782=CARTESIAN_POINT('Ctrl Pts',(41.6396395952276,26.5045331830048,11.5712994880388));
#27783=CARTESIAN_POINT('Ctrl Pts',(43.7456004865738,28.1126739863601,12.1741073022483));
#27784=CARTESIAN_POINT('Ctrl Pts',(45.8515613779199,29.7208147897153,11.5712994880388));
#27785=CARTESIAN_POINT('Ctrl Pts',(36.8732642383515,21.006164983318,0.));
#27786=CARTESIAN_POINT('Ctrl Pts',(36.757412634611,21.1864335974961,2.19648874705823));
#27787=CARTESIAN_POINT('Ctrl Pts',(37.4432931040928,21.8819441292785,4.17545672685567));
#27788=CARTESIAN_POINT('Ctrl Pts',(38.1291735735746,22.5774546610608,6.15442470665314));
#27789=CARTESIAN_POINT('Ctrl Pts',(39.4579932465785,23.6861571296384,7.5239130403414));
#27790=CARTESIAN_POINT('Ctrl Pts',(40.7868129195823,24.794859598216,8.89340137402967));
#27791=CARTESIAN_POINT('Ctrl Pts',(42.4724369320184,26.1328662922311,9.3821661014496));
#27792=CARTESIAN_POINT('Ctrl Pts',(44.1580609444546,27.4708729862462,9.87093082886954));
#27793=CARTESIAN_POINT('Ctrl Pts',(45.8436849568907,28.8088796802613,9.3821661014496));
#27794=CARTESIAN_POINT('Ctrl Pts',(39.2421052839114,21.1183468312843,0.));
#27795=CARTESIAN_POINT('Ctrl Pts',(39.126253680171,21.2986154454624,1.72780310113342));
#27796=CARTESIAN_POINT('Ctrl Pts',(39.6410609697423,21.8841839202762,3.28449990511992));
#27797=CARTESIAN_POINT('Ctrl Pts',(40.1558682593137,22.46975239509,4.84119670910638));
#27798=CARTESIAN_POINT('Ctrl Pts',(41.1764247138527,23.3803461224639,5.91846432228298));
#27799=CARTESIAN_POINT('Ctrl Pts',(42.1969811683917,24.2909398498379,6.99573193545956));
#27800=CARTESIAN_POINT('Ctrl Pts',(43.4982072348259,25.3819089842539,7.3802042952164));
#27801=CARTESIAN_POINT('Ctrl Pts',(44.7994333012602,26.4728781186699,7.76467665497322));
#27802=CARTESIAN_POINT('Ctrl Pts',(46.1006593676944,27.5638472530859,7.38020429521639));
#27803=CARTESIAN_POINT('',(32.4262389886935,19.4238236466219,1.57950316568597E-9));
#27804=CARTESIAN_POINT('Origin',(40.0935818932913,3.13849734404774,0.));
#27805=CARTESIAN_POINT('Ctrl Pts',(32.4262389885471,19.4238236468409,3.1310815762065E-9));
#27806=CARTESIAN_POINT('Ctrl Pts',(32.4174924183248,19.4374335758627,0.245038153335351));
#27807=CARTESIAN_POINT('Ctrl Pts',(32.4140004629285,19.4545900740528,0.490791160521444));
#27808=CARTESIAN_POINT('Ctrl Pts',(32.415852221603,19.4753132856566,0.736766500724951));
#27809=CARTESIAN_POINT('Ctrl Pts',(32.4176979010578,19.4959684641205,0.981934317700587));
#27810=CARTESIAN_POINT('Ctrl Pts',(32.4248523667013,19.5201670081214,1.22732257376522));
#27811=CARTESIAN_POINT('Ctrl Pts',(32.4373620269519,19.5479002488741,1.47243294816298));
#27812=CARTESIAN_POINT('Ctrl Pts',(32.4498528472303,19.5755917224263,1.71717417802969));
#27813=CARTESIAN_POINT('Ctrl Pts',(32.467682800622,19.6068072561334,1.96163791541534));
#27814=CARTESIAN_POINT('Ctrl Pts',(32.4908551297617,19.6415093732945,2.20532408778468));
#27815=CARTESIAN_POINT('Ctrl Pts',(32.5140075851258,19.6761817281437,2.4488012624201));
#27816=CARTESIAN_POINT('Ctrl Pts',(32.5424932593661,19.7143346547167,2.69150175430996));
#27817=CARTESIAN_POINT('Ctrl Pts',(32.5762720176612,19.7559021858351,2.93292951866755));
#27818=CARTESIAN_POINT('Ctrl Pts',(32.6100437093728,19.7974610209431,3.17430677585539));
#27819=CARTESIAN_POINT('Ctrl Pts',(32.6491062197569,19.8424329629628,3.41441139318295));
#27820=CARTESIAN_POINT('Ctrl Pts',(32.6933764227085,19.8907242666033,3.6527571061459));
#27821=CARTESIAN_POINT('Ctrl Pts',(32.7377028392566,19.9390768897696,3.89140546668738));
#27822=CARTESIAN_POINT('Ctrl Pts',(32.7872500836133,19.9907572100055,4.12829002081109));
#27823=CARTESIAN_POINT('Ctrl Pts',(32.8418926894894,20.0456444897533,4.36293874377749));
#27824=CARTESIAN_POINT('Ctrl Pts',(32.8965910526136,20.1005877764142,4.5978269020138));
#27825=CARTESIAN_POINT('Ctrl Pts',(32.9563950254811,20.1587444351916,4.83047425894881));
#27826=CARTESIAN_POINT('Ctrl Pts',(33.0211385895995,20.2199684571167,5.06042975959344));
#27827=CARTESIAN_POINT('Ctrl Pts',(33.0860714385207,20.2813714740828,5.29105755998216));
#27828=CARTESIAN_POINT('Ctrl Pts',(33.1559726078587,20.3458596558639,5.51897736305598));
#27829=CARTESIAN_POINT('Ctrl Pts',(33.2306368658403,20.413262889504,5.7437625935424));
#27830=CARTESIAN_POINT('Ctrl Pts',(33.2782450169496,20.4562411955789,5.88709234072559));
#27831=CARTESIAN_POINT('Ctrl Pts',(33.3277889511025,20.5004042255162,6.02914825314163));
#27832=CARTESIAN_POINT('Ctrl Pts',(33.3792081011979,20.5457035458388,6.16982677023484));
#27833=CARTESIAN_POINT('Ctrl Pts',(33.4598348411498,20.6167342126792,6.390414823391));
#27834=CARTESIAN_POINT('Ctrl Pts',(33.5454408102123,20.6911341865983,6.60890054011824));
#27835=CARTESIAN_POINT('Ctrl Pts',(33.6359284429692,20.7688037431276,6.82480412008069));
#27836=CARTESIAN_POINT('Ctrl Pts',(33.7262117948162,20.8462979562736,7.04022028559317));
#27837=CARTESIAN_POINT('Ctrl Pts',(33.8213547340594,20.9270469355452,7.25306552029659));
#27838=CARTESIAN_POINT('Ctrl Pts',(33.9212188657882,21.0109232247564,7.46287566269436));
#27839=CARTESIAN_POINT('Ctrl Pts',(34.0209223750764,21.0946646065286,7.6723483444191));
#27840=CARTESIAN_POINT('Ctrl Pts',(34.1253317904082,21.1815231404629,7.87879526533065));
#27841=CARTESIAN_POINT('Ctrl Pts',(34.2342692590686,21.2713449564541,8.08177334612241));
#27842=CARTESIAN_POINT('Ctrl Pts',(34.3431021983079,21.3610805851808,8.28455666214176));
#27843=CARTESIAN_POINT('Ctrl Pts',(34.456454344463,21.4537736728372,8.48387739272939));
#27844=CARTESIAN_POINT('Ctrl Pts',(34.5741103132403,21.5492456275386,8.67931873611198));
#27845=CARTESIAN_POINT('Ctrl Pts',(34.6917719409582,21.6447221741883,8.87476947970573));
#27846=CARTESIAN_POINT('Ctrl Pts',(34.8137376000418,21.7429776869135,9.06634009532888));
#27847=CARTESIAN_POINT('Ctrl Pts',(34.9397565506955,21.8438106715185,9.25364450341021));
#27848=CARTESIAN_POINT('Ctrl Pts',(35.0658217301578,21.9446806457088,9.44101762226526));
#27849=CARTESIAN_POINT('Ctrl Pts',(35.1959429263784,22.0481297867737,9.62412107875057));
#27850=CARTESIAN_POINT('Ctrl Pts',(35.3298371867854,22.1539362249981,9.80260437466142));
#27851=CARTESIAN_POINT('Ctrl Pts',(35.4639498564645,22.2599152554387,9.98137881379685));
#27852=CARTESIAN_POINT('Ctrl Pts',(35.6018476263942,22.3682590622501,10.1555177270924));
#27853=CARTESIAN_POINT('Ctrl Pts',(35.7432181181529,22.4787275806304,10.3247095747707));
#27854=CARTESIAN_POINT('Ctrl Pts',(35.7840789755634,22.5106567217244,10.3736117457754));
#27855=CARTESIAN_POINT('Ctrl Pts',(35.8252297828071,22.5427632651452,10.4221009095756));
#27856=CARTESIAN_POINT('Ctrl Pts',(35.8666626160154,22.575041189881,10.4701702229111));
#27857=CARTESIAN_POINT('Ctrl Pts',(35.5116836434679,26.9229962078195,0.));
#27858=CARTESIAN_POINT('Ctrl Pts',(35.3958320397274,27.1032648219976,1.72780310113343));
#27859=CARTESIAN_POINT('Ctrl Pts',(35.9106393292987,27.6888332968114,3.28449990511991));
#27860=CARTESIAN_POINT('Ctrl Pts',(36.4254466188701,28.2744017716252,4.84119670910639));
#27861=CARTESIAN_POINT('Ctrl Pts',(37.4460030734091,29.1849954989991,5.91846432228298));
#27862=CARTESIAN_POINT('Ctrl Pts',(38.4665595279481,30.0955892263731,6.99573193545956));
#27863=CARTESIAN_POINT('Ctrl Pts',(39.7677855943823,31.1865583607891,7.38020429521639));
#27864=CARTESIAN_POINT('Ctrl Pts',(41.0690116608166,32.2775274952051,7.76467665497322));
#27865=CARTESIAN_POINT('Ctrl Pts',(42.3702377272508,33.368496629621,7.38020429521639));
#27866=CARTESIAN_POINT('Ctrl Pts',(34.425587311519,24.8148246247006,0.));
#27867=CARTESIAN_POINT('Ctrl Pts',(34.3097357077786,24.9950932388787,2.19648874705823));
#27868=CARTESIAN_POINT('Ctrl Pts',(34.9956161772604,25.690603770661,4.17545672685568));
#27869=CARTESIAN_POINT('Ctrl Pts',(35.6814966467422,26.3861143024433,6.15442470665313));
#27870=CARTESIAN_POINT('Ctrl Pts',(37.010316319746,27.494816771021,7.5239130403414));
#27871=CARTESIAN_POINT('Ctrl Pts',(38.3391359927498,28.6035192395986,8.89340137402967));
#27872=CARTESIAN_POINT('Ctrl Pts',(40.024760005186,29.9415259336137,9.38216610144961));
#27873=CARTESIAN_POINT('Ctrl Pts',(41.7103840176221,31.2795326276287,9.87093082886953));
#27874=CARTESIAN_POINT('Ctrl Pts',(43.3960080300583,32.6175393216438,9.3821661014496));
#27875=CARTESIAN_POINT('Ctrl Pts',(32.9490709821978,22.9590519566751,0.));
#27876=CARTESIAN_POINT('Ctrl Pts',(32.8332193784573,23.1393205708532,2.7089937269807));
#27877=CARTESIAN_POINT('Ctrl Pts',(33.7061673576818,23.9550520912432,5.14971273833323));
#27878=CARTESIAN_POINT('Ctrl Pts',(34.5791153369063,24.7707836116333,7.59043174968577));
#27879=CARTESIAN_POINT('Ctrl Pts',(36.2450190148585,26.0961168162188,9.27946171175751));
#27880=CARTESIAN_POINT('Ctrl Pts',(37.9109226928106,27.4214500208043,10.9684916738292));
#27881=CARTESIAN_POINT('Ctrl Pts',(40.0168835841568,29.0295908241596,11.5712994880388));
#27882=CARTESIAN_POINT('Ctrl Pts',(42.1228444755029,30.6377316275148,12.1741073022483));
#27883=CARTESIAN_POINT('Ctrl Pts',(44.2288053668491,32.2458724308701,11.5712994880388));
#27884=CARTESIAN_POINT('Ctrl Pts',(31.1388779521431,21.4269965203138,0.));
#27885=CARTESIAN_POINT('Ctrl Pts',(31.0230263484026,21.607265134492,3.24562220582793));
#27886=CARTESIAN_POINT('Ctrl Pts',(32.0918470647274,22.5488764195075,6.16982677025167));
#27887=CARTESIAN_POINT('Ctrl Pts',(33.1606677810522,23.490487704523,9.09403133467541));
#27888=CARTESIAN_POINT('Ctrl Pts',(35.1795219354008,25.0426484071615,11.1176436806954));
#27889=CARTESIAN_POINT('Ctrl Pts',(37.1983760897495,26.5948091098,13.1412560267153));
#27890=CARTESIAN_POINT('Ctrl Pts',(39.7444590262843,28.4857991767895,13.8634749112255));
#27891=CARTESIAN_POINT('Ctrl Pts',(42.2905419628192,30.3767892437791,14.5856937957357));
#27892=CARTESIAN_POINT('Ctrl Pts',(44.8366248993541,32.2677793107686,13.8634749112255));
#27893=CARTESIAN_POINT('',(31.1388779521431,21.4269965203138,0.));
#27894=CARTESIAN_POINT('Ctrl Pts',(31.1388779521431,21.4269965203138,0.));
#27895=CARTESIAN_POINT('Ctrl Pts',(31.0230263484026,21.607265134492,3.24562220582793));
#27896=CARTESIAN_POINT('Ctrl Pts',(32.0918470647274,22.5488764195074,6.16982677025168));
#27897=CARTESIAN_POINT('Ctrl Pts',(32.984139246383,23.3349693300819,8.61106394926976));
#27898=CARTESIAN_POINT('Ctrl Pts',(34.5610181206247,24.5639673341826,10.4489096280657));
#27899=CARTESIAN_POINT('Origin',(19.5103534449755,35.16662598352,0.));
#27900=CARTESIAN_POINT('Ctrl Pts',(31.1388779521431,21.4269965203138,0.));
#27901=CARTESIAN_POINT('Ctrl Pts',(31.0230263484026,21.607265134492,3.24562220582793));
#27902=CARTESIAN_POINT('Ctrl Pts',(32.0918470647274,22.5488764195075,6.16982677025167));
#27903=CARTESIAN_POINT('Ctrl Pts',(33.1606677810522,23.490487704523,9.09403133467541));
#27904=CARTESIAN_POINT('Ctrl Pts',(35.1795219354008,25.0426484071615,11.1176436806954));
#27905=CARTESIAN_POINT('Ctrl Pts',(37.1983760897495,26.5948091098,13.1412560267153));
#27906=CARTESIAN_POINT('Ctrl Pts',(39.7444590262843,28.4857991767895,13.8634749112255));
#27907=CARTESIAN_POINT('Ctrl Pts',(42.2905419628192,30.3767892437791,14.5856937957357));
#27908=CARTESIAN_POINT('Ctrl Pts',(44.8366248993541,32.2677793107686,13.8634749112255));
#27909=CARTESIAN_POINT('Ctrl Pts',(30.9950965373909,20.4854409432118,6.24500451351651E-15));
#27910=CARTESIAN_POINT('Ctrl Pts',(30.8792449336505,20.6657095573899,3.38941559469373));
#27911=CARTESIAN_POINT('Ctrl Pts',(32.0005511325098,21.6410512138983,6.44317352589574));
#27912=CARTESIAN_POINT('Ctrl Pts',(33.1218573313691,22.6163928704066,9.49693145709774));
#27913=CARTESIAN_POINT('Ctrl Pts',(35.2352870572787,24.2293336022806,11.6101975146502));
#27914=CARTESIAN_POINT('Ctrl Pts',(37.3487167831882,25.8422743341547,13.7234635722027));
#27915=CARTESIAN_POINT('Ctrl Pts',(40.0127335284694,27.8090558579144,14.4776794959001));
#27916=CARTESIAN_POINT('Ctrl Pts',(42.6767502737507,29.7758373816741,15.2318954195974));
#27917=CARTESIAN_POINT('Ctrl Pts',(45.3407670190319,31.7426189054338,14.4776794959001));
#27918=CARTESIAN_POINT('Ctrl Pts',(31.5100409519663,19.6841717937385,0.));
#27919=CARTESIAN_POINT('Ctrl Pts',(31.3941893482258,19.8644404079166,3.38941559469373));
#27920=CARTESIAN_POINT('Ctrl Pts',(32.5154955470851,20.839782064425,6.44317352589574));
#27921=CARTESIAN_POINT('Ctrl Pts',(33.6368017459444,21.8151237209333,9.49693145709774));
#27922=CARTESIAN_POINT('Ctrl Pts',(35.750231471854,23.4280644528074,11.6101975146502));
#27923=CARTESIAN_POINT('Ctrl Pts',(37.8636611977636,25.0410051846814,13.7234635722027));
#27924=CARTESIAN_POINT('Ctrl Pts',(40.5276779430448,27.0077867084411,14.4776794959001));
#27925=CARTESIAN_POINT('Ctrl Pts',(43.191694688326,28.9745682322008,15.2318954195974));
#27926=CARTESIAN_POINT('Ctrl Pts',(45.8557114336072,30.9413497559605,14.4776794959001));
#27927=CARTESIAN_POINT('Ctrl Pts',(32.4262389885814,19.4238236466306,1.04083408558608E-14));
#27928=CARTESIAN_POINT('Ctrl Pts',(32.310387384841,19.6040922608087,3.24562220582793));
#27929=CARTESIAN_POINT('Ctrl Pts',(33.3792081011658,20.5457035458242,6.16982677025168));
#27930=CARTESIAN_POINT('Ctrl Pts',(34.4480288174906,21.4873148308398,9.09403133467541));
#27931=CARTESIAN_POINT('Ctrl Pts',(36.4668829718392,23.0394755334782,11.1176436806954));
#27932=CARTESIAN_POINT('Ctrl Pts',(38.4857371261878,24.5916362361167,13.1412560267153));
#27933=CARTESIAN_POINT('Ctrl Pts',(41.0318200627227,26.4826263031063,13.8634749112255));
#27934=CARTESIAN_POINT('Ctrl Pts',(43.5779029992576,28.3736163700958,14.5856937957357));
#27935=CARTESIAN_POINT('Ctrl Pts',(46.1239859357924,30.2646064370854,13.8634749112255));
#27936=CARTESIAN_POINT('',(31.4039970697498,20.1821175312128,3.07395939422514E-30));
#27937=CARTESIAN_POINT('Origin',(32.9182507396844,21.1552751870372,0.));
#27938=CARTESIAN_POINT('Origin',(32.9182507396844,21.1552751870372,0.));
#27939=CARTESIAN_POINT('Ctrl Pts',(34.8604849513725,14.611382171278,0.));
#27940=CARTESIAN_POINT('Ctrl Pts',(34.7714674485863,14.8063033131397,3.24562220582793));
#27941=CARTESIAN_POINT('Ctrl Pts',(35.9634143688744,15.5862213055782,6.16982677025167));
#27942=CARTESIAN_POINT('Ctrl Pts',(37.1553612891626,16.3661392980167,9.09403133467541));
#27943=CARTESIAN_POINT('Ctrl Pts',(39.3745619185374,17.6151883402598,11.1176436806954));
#27944=CARTESIAN_POINT('Ctrl Pts',(41.5937625479122,18.8642373825028,13.1412560267153));
#27945=CARTESIAN_POINT('Ctrl Pts',(44.3830459768616,20.3736345158496,13.8634749112255));
#27946=CARTESIAN_POINT('Ctrl Pts',(47.1723294058109,21.8830316491965,14.5856937957357));
#27947=CARTESIAN_POINT('Ctrl Pts',(49.9616128347603,23.3924287825432,13.8634749112255));
#27948=CARTESIAN_POINT('Ctrl Pts',(37.1279962392258,15.3059217494161,0.));
#27949=CARTESIAN_POINT('Ctrl Pts',(37.0389787364397,15.5008428912778,2.70899372698068));
#27950=CARTESIAN_POINT('Ctrl Pts',(38.0191320633214,16.1840379904937,5.14971273833323));
#27951=CARTESIAN_POINT('Ctrl Pts',(38.9992853902032,16.8672330897095,7.59043174968577));
#27952=CARTESIAN_POINT('Ctrl Pts',(40.8368471514174,17.9419935007384,9.2794617117575));
#27953=CARTESIAN_POINT('Ctrl Pts',(42.6744089126316,19.0167539117673,10.9684916738292));
#27954=CARTESIAN_POINT('Ctrl Pts',(44.9877964569989,20.3088166768302,11.5712994880388));
#27955=CARTESIAN_POINT('Ctrl Pts',(47.3011840013661,21.600879441893,12.1741073022483));
#27956=CARTESIAN_POINT('Ctrl Pts',(49.6145715457333,22.8929422069559,11.5712994880388));
#27957=CARTESIAN_POINT('Ctrl Pts',(39.4874365476046,15.5447398754875,-1.05434036998093E-14));
#27958=CARTESIAN_POINT('Ctrl Pts',(39.3984190448184,15.7396610173492,2.19648874705823));
#27959=CARTESIAN_POINT('Ctrl Pts',(40.1762997089269,16.3304812866722,4.17545672685568));
#27960=CARTESIAN_POINT('Ctrl Pts',(40.9541803730353,16.9213015559953,6.15442470665313));
#27961=CARTESIAN_POINT('Ctrl Pts',(42.4272593902765,17.8296082752018,7.5239130403414));
#27962=CARTESIAN_POINT('Ctrl Pts',(43.9003384075178,18.7379149944084,8.89340137402966));
#27963=CARTESIAN_POINT('Ctrl Pts',(45.7592234042437,19.8224134008053,9.3821661014496));
#27964=CARTESIAN_POINT('Ctrl Pts',(47.6181084009697,20.9069118072022,9.87093082886953));
#27965=CARTESIAN_POINT('Ctrl Pts',(49.4769933976957,21.9914102135992,9.38216610144959));
#27966=CARTESIAN_POINT('Ctrl Pts',(41.848131348458,15.3186586437003,1.04083408558608E-14));
#27967=CARTESIAN_POINT('Ctrl Pts',(41.7591138456719,15.513579785562,1.72780310113342));
#27968=CARTESIAN_POINT('Ctrl Pts',(42.3520162221172,16.019923301465,3.28449990511991));
#27969=CARTESIAN_POINT('Ctrl Pts',(42.9449185985626,16.5262668173679,4.84119670910638));
#27970=CARTESIAN_POINT('Ctrl Pts',(44.0846782589592,17.2823516867885,5.91846432228298));
#27971=CARTESIAN_POINT('Ctrl Pts',(45.2244379193558,18.038436556209,6.99573193545956));
#27972=CARTESIAN_POINT('Ctrl Pts',(46.6676804765724,18.9331174206827,7.38020429521639));
#27973=CARTESIAN_POINT('Ctrl Pts',(48.1109230337889,19.8277982851563,7.76467665497322));
#27974=CARTESIAN_POINT('Ctrl Pts',(49.5541655910054,20.72247914963,7.38020429521639));
#27975=CARTESIAN_POINT('',(34.8604849513959,14.6113821712854,1.57949473064594E-9));
#27976=CARTESIAN_POINT('Origin',(40.1321417817281,-2.59935965651565,0.));
#27977=CARTESIAN_POINT('Ctrl Pts',(34.8604849513684,14.6113821714911,3.131065100813E-9));
#27978=CARTESIAN_POINT('Ctrl Pts',(34.8537643034671,14.6260983377859,0.24503815333575));
#27979=CARTESIAN_POINT('Ctrl Pts',(34.852749515407,14.6435771646296,0.490791160522261));
#27980=CARTESIAN_POINT('Ctrl Pts',(34.8575316463562,14.6638259110834,0.736766500726186));
#27981=CARTESIAN_POINT('Ctrl Pts',(34.862298077838,14.6840081820398,0.981934317701831));
#27982=CARTESIAN_POINT('Ctrl Pts',(34.872823533213,14.7069422331332,1.22732257376648));
#27983=CARTESIAN_POINT('Ctrl Pts',(34.8891527148323,14.7326128792076,1.47243294816424));
#27984=CARTESIAN_POINT('Ctrl Pts',(34.9054573041507,14.7582448644191,1.71717417803102));
#27985=CARTESIAN_POINT('Ctrl Pts',(34.9275482079567,14.7866052020688,1.96163791541673));
#27986=CARTESIAN_POINT('Ctrl Pts',(34.955423302389,14.8176563354396,2.20532408778614));
#27987=CARTESIAN_POINT('Ctrl Pts',(34.9832744897135,14.8486808377691,2.44880126242163));
#27988=CARTESIAN_POINT('Ctrl Pts',(35.0168999484379,14.882391488439,2.69150175431155));
#27989=CARTESIAN_POINT('Ctrl Pts',(35.0562505641471,14.9187287035022,2.93292951866921));
#27990=CARTESIAN_POINT('Ctrl Pts',(35.0955929476291,14.9550583167476,3.1743067758571));
#27991=CARTESIAN_POINT('Ctrl Pts',(35.1406580326364,14.9940133343939,3.41441139318471));
#27992=CARTESIAN_POINT('Ctrl Pts',(35.191350197822,15.0355127954202,3.6527571061477));
#27993=CARTESIAN_POINT('Ctrl Pts',(35.2421067311091,15.0770649517992,3.89140546668922));
#27994=CARTESIAN_POINT('Ctrl Pts',(35.2985045323757,15.1211679328245,4.12829002081298));
#27995=CARTESIAN_POINT('Ctrl Pts',(35.3604022296527,15.1677200855873,4.36293874377942));
#27996=CARTESIAN_POINT('Ctrl Pts',(35.4223630872643,15.2143197401098,4.59782690201577));
#27997=CARTESIAN_POINT('Ctrl Pts',(35.4898348974067,15.2633734552292,4.83047425895083));
#27998=CARTESIAN_POINT('Ctrl Pts',(35.5626325521737,15.3147603350321,5.06042975959551));
#27999=CARTESIAN_POINT('Ctrl Pts',(35.6356430387473,15.3662974499285,5.2910575599842));
#28000=CARTESIAN_POINT('Ctrl Pts',(35.7140103401313,15.4201812613939,5.51897736305799));
#28001=CARTESIAN_POINT('Ctrl Pts',(35.7975071039183,15.4762725955035,5.74376259354438));
#28002=CARTESIAN_POINT('Ctrl Pts',(35.8507471233726,15.5120380980664,5.8870923407269));
#28003=CARTESIAN_POINT('Ctrl Pts',(35.9060718261753,15.5487007750603,6.02914825314227));
#28004=CARTESIAN_POINT('Ctrl Pts',(35.9634143689083,15.586221305588,6.16982677023484));
#28005=CARTESIAN_POINT('Ctrl Pts',(36.0533291627655,15.645054601201,6.39041482339096));
#28006=CARTESIAN_POINT('Ctrl Pts',(36.1486520067523,15.7065142910191,6.60890054011815));
#28007=CARTESIAN_POINT('Ctrl Pts',(36.2492721362563,15.7705155506317,6.82480412008057));
#28008=CARTESIAN_POINT('Ctrl Pts',(36.3496651101704,15.8343723238084,7.0402202855931));
#28009=CARTESIAN_POINT('Ctrl Pts',(36.4553314094028,15.9007591428902,7.25306552029658));
#28010=CARTESIAN_POINT('Ctrl Pts',(36.5661159087968,15.9695695446607,7.46287566269441));
#28011=CARTESIAN_POINT('Ctrl Pts',(36.6767222213247,16.0382692711118,7.67234834441893));
#28012=CARTESIAN_POINT('Ctrl Pts',(36.7924301575637,16.1093847013531,7.87879526533028));
#28013=CARTESIAN_POINT('Ctrl Pts',(36.9130417770841,16.1827888425355,8.08177334612183));
#28014=CARTESIAN_POINT('Ctrl Pts',(37.0335376654153,16.2561225498029,8.28455666214065));
#28015=CARTESIAN_POINT('Ctrl Pts',(37.1589276519414,16.3317404631312,8.48387739272776));
#28016=CARTESIAN_POINT('Ctrl Pts',(37.288973128395,16.4094964608243,8.67931873610986));
#28017=CARTESIAN_POINT('Ctrl Pts',(37.4190248596921,16.4872561983753,8.87476947970367));
#28018=CARTESIAN_POINT('Ctrl Pts',(37.5537323016291,16.5671540886063,9.06634009532686));
#28019=CARTESIAN_POINT('Ctrl Pts',(37.6928185909662,16.6490263722355,9.25364450340825));
#28020=CARTESIAN_POINT('Ctrl Pts',(37.8319559027359,16.730928689904,9.44101762226329));
#28021=CARTESIAN_POINT('Ctrl Pts',(37.9754750005784,16.814806690878,9.62412107874858));
#28022=CARTESIAN_POINT('Ctrl Pts',(38.1230642366182,16.900481032106,9.80260437465942));
#28023=CARTESIAN_POINT('Ctrl Pts',(38.270894221272,16.9862951259302,9.98137881379502));
#28024=CARTESIAN_POINT('Ctrl Pts',(38.4228073220804,17.0739112501813,10.1555177270907));
#28025=CARTESIAN_POINT('Ctrl Pts',(38.5784601754,17.1631362396558,10.3247095747691));
#28026=CARTESIAN_POINT('Ctrl Pts',(38.6234491187501,17.1889252818176,10.3736117457744));
#28027=CARTESIAN_POINT('Ctrl Pts',(38.6687503076455,17.2148486564428,10.4221009095751));
#28028=CARTESIAN_POINT('Ctrl Pts',(38.714355041992,17.2409015314888,10.4701702229111));
#28029=CARTESIAN_POINT('Ctrl Pts',(38.981767758745,21.5951194116466,0.));
#28030=CARTESIAN_POINT('Ctrl Pts',(38.8927502559589,21.7900405535082,1.72780310113343));
#28031=CARTESIAN_POINT('Ctrl Pts',(39.4856526324043,22.2963840694112,3.28449990511992));
#28032=CARTESIAN_POINT('Ctrl Pts',(40.0785550088497,22.8027275853141,4.84119670910638));
#28033=CARTESIAN_POINT('Ctrl Pts',(41.2183146692462,23.5588124547347,5.91846432228298));
#28034=CARTESIAN_POINT('Ctrl Pts',(42.3580743296429,24.3148973241552,6.99573193545956));
#28035=CARTESIAN_POINT('Ctrl Pts',(43.8013168868594,25.2095781886289,7.3802042952164));
#28036=CARTESIAN_POINT('Ctrl Pts',(45.2445594440759,26.1042590531026,7.76467665497323));
#28037=CARTESIAN_POINT('Ctrl Pts',(46.6878020012925,26.9989399175762,7.38020429521639));
#28038=CARTESIAN_POINT('Ctrl Pts',(37.6067022235299,19.6629735993419,0.));
#28039=CARTESIAN_POINT('Ctrl Pts',(37.5176847207438,19.8578947412036,2.19648874705823));
#28040=CARTESIAN_POINT('Ctrl Pts',(38.2955653848522,20.4487150105266,4.17545672685568));
#28041=CARTESIAN_POINT('Ctrl Pts',(39.0734460489607,21.0395352798497,6.15442470665314));
#28042=CARTESIAN_POINT('Ctrl Pts',(40.5465250662019,21.9478419990562,7.5239130403414));
#28043=CARTESIAN_POINT('Ctrl Pts',(42.0196040834431,22.8561487182628,8.89340137402969));
#28044=CARTESIAN_POINT('Ctrl Pts',(43.8784890801691,23.9406471246597,9.38216610144961));
#28045=CARTESIAN_POINT('Ctrl Pts',(45.7373740768951,25.0251455310566,9.87093082886954));
#28046=CARTESIAN_POINT('Ctrl Pts',(47.5962590736211,26.1096439374536,9.38216610144961));
#28047=CARTESIAN_POINT('Ctrl Pts',(35.8811107143584,18.036220203889,0.));
#28048=CARTESIAN_POINT('Ctrl Pts',(35.7920932115723,18.2311413457506,2.70899372698069));
#28049=CARTESIAN_POINT('Ctrl Pts',(36.772246538454,18.9143364449665,5.14971273833323));
#28050=CARTESIAN_POINT('Ctrl Pts',(37.7523998653357,19.5975315441823,7.59043174968578));
#28051=CARTESIAN_POINT('Ctrl Pts',(39.5899616265499,20.6722919552112,9.27946171175751));
#28052=CARTESIAN_POINT('Ctrl Pts',(41.4275233877641,21.7470523662401,10.9684916738292));
#28053=CARTESIAN_POINT('Ctrl Pts',(43.7409109321314,23.039115131303,11.5712994880388));
#28054=CARTESIAN_POINT('Ctrl Pts',(46.0542984764987,24.3311778963658,12.1741073022483));
#28055=CARTESIAN_POINT('Ctrl Pts',(48.367686020866,25.6232406614287,11.5712994880388));
#28056=CARTESIAN_POINT('Ctrl Pts',(33.8713086176154,16.777376211144,0.));
#28057=CARTESIAN_POINT('Ctrl Pts',(33.7822911148293,16.9722973530056,3.24562220582793));
#28058=CARTESIAN_POINT('Ctrl Pts',(34.9742380351174,17.7522153454442,6.16982677025167));
#28059=CARTESIAN_POINT('Ctrl Pts',(36.1661849554055,18.5321333378827,9.09403133467541));
#28060=CARTESIAN_POINT('Ctrl Pts',(38.3853855847803,19.7811823801258,11.1176436806954));
#28061=CARTESIAN_POINT('Ctrl Pts',(40.6045862141551,21.0302314223688,13.1412560267153));
#28062=CARTESIAN_POINT('Ctrl Pts',(43.3938696431045,22.5396285557156,13.8634749112255));
#28063=CARTESIAN_POINT('Ctrl Pts',(46.1831530720539,24.0490256890624,14.5856937957357));
#28064=CARTESIAN_POINT('Ctrl Pts',(48.9724365010033,25.5584228224092,13.8634749112255));
#28065=CARTESIAN_POINT('',(33.8713086176154,16.777376211144,0.));
#28066=CARTESIAN_POINT('Ctrl Pts',(33.8713086176154,16.777376211144,0.));
#28067=CARTESIAN_POINT('Ctrl Pts',(33.7822911148293,16.9722973530056,3.24562220582793));
#28068=CARTESIAN_POINT('Ctrl Pts',(34.9742380351174,17.7522153454441,6.16982677025168));
#28069=CARTESIAN_POINT('Ctrl Pts',(35.969320654379,18.4033205461165,8.61106394926976));
#28070=CARTESIAN_POINT('Ctrl Pts',(37.7050538275442,19.39539586064,10.4489096280657));
#28071=CARTESIAN_POINT('Origin',(24.316498867974,32.0320676419189,0.));
#28072=CARTESIAN_POINT('Ctrl Pts',(33.8713086176154,16.7773762111439,0.));
#28073=CARTESIAN_POINT('Ctrl Pts',(33.7822911148293,16.9722973530056,3.24562220582793));
#28074=CARTESIAN_POINT('Ctrl Pts',(34.9742380351174,17.7522153454441,6.16982677025168));
#28075=CARTESIAN_POINT('Ctrl Pts',(36.1661849554055,18.5321333378827,9.09403133467541));
#28076=CARTESIAN_POINT('Ctrl Pts',(38.3853855847803,19.7811823801258,11.1176436806954));
#28077=CARTESIAN_POINT('Ctrl Pts',(40.6045862141551,21.0302314223688,13.1412560267153));
#28078=CARTESIAN_POINT('Ctrl Pts',(43.3938696431045,22.5396285557156,13.8634749112255));
#28079=CARTESIAN_POINT('Ctrl Pts',(46.1831530720539,24.0490256890624,14.5856937957357));
#28080=CARTESIAN_POINT('Ctrl Pts',(48.9724365010033,25.5584228224092,13.8634749112255));
#28081=CARTESIAN_POINT('Ctrl Pts',(33.5949933606691,15.865866540993,0.));
#28082=CARTESIAN_POINT('Ctrl Pts',(33.505975857883,16.0607876828547,3.38941559469372));
#28083=CARTESIAN_POINT('Ctrl Pts',(34.7546743665352,16.8666232572808,6.44317352589574));
#28084=CARTESIAN_POINT('Ctrl Pts',(36.0033728751873,17.6724588317069,9.49693145709774));
#28085=CARTESIAN_POINT('Ctrl Pts',(38.3248363332022,18.9682097429542,11.6101975146502));
#28086=CARTESIAN_POINT('Ctrl Pts',(40.646299791217,20.2639606542015,13.7234635722027));
#28087=CARTESIAN_POINT('Ctrl Pts',(43.563102881699,21.8315940656521,14.4776794959001));
#28088=CARTESIAN_POINT('Ctrl Pts',(46.479905972181,23.3992274771026,15.2318954195974));
#28089=CARTESIAN_POINT('Ctrl Pts',(49.3967090626629,24.9668608885532,14.4776794959001));
#28090=CARTESIAN_POINT('Ctrl Pts',(33.990663894172,14.9994689250466,0.));
#28091=CARTESIAN_POINT('Ctrl Pts',(33.9016463913858,15.1943900669083,3.38941559469372));
#28092=CARTESIAN_POINT('Ctrl Pts',(35.150344900038,16.0002256413344,6.44317352589574));
#28093=CARTESIAN_POINT('Ctrl Pts',(36.3990434086901,16.8060612157605,9.49693145709774));
#28094=CARTESIAN_POINT('Ctrl Pts',(38.720506866705,18.1018121270078,11.6101975146502));
#28095=CARTESIAN_POINT('Ctrl Pts',(41.0419703247199,19.3975630382551,13.7234635722027));
#28096=CARTESIAN_POINT('Ctrl Pts',(43.9587734152018,20.9651964497057,14.4776794959001));
#28097=CARTESIAN_POINT('Ctrl Pts',(46.8755765056838,22.5328298611562,15.2318954195974));
#28098=CARTESIAN_POINT('Ctrl Pts',(49.7923795961658,24.1004632726068,14.4776794959001));
#28099=CARTESIAN_POINT('Ctrl Pts',(34.8604849513725,14.611382171278,0.));
#28100=CARTESIAN_POINT('Ctrl Pts',(34.7714674485863,14.8063033131397,3.24562220582793));
#28101=CARTESIAN_POINT('Ctrl Pts',(35.9634143688744,15.5862213055782,6.16982677025167));
#28102=CARTESIAN_POINT('Ctrl Pts',(37.1553612891626,16.3661392980167,9.09403133467541));
#28103=CARTESIAN_POINT('Ctrl Pts',(39.3745619185374,17.6151883402598,11.1176436806954));
#28104=CARTESIAN_POINT('Ctrl Pts',(41.5937625479122,18.8642373825028,13.1412560267153));
#28105=CARTESIAN_POINT('Ctrl Pts',(44.3830459768616,20.3736345158497,13.8634749112255));
#28106=CARTESIAN_POINT('Ctrl Pts',(47.1723294058109,21.8830316491965,14.5856937957357));
#28107=CARTESIAN_POINT('Ctrl Pts',(49.9616128347603,23.3924287825433,13.8634749112255));
#28108=CARTESIAN_POINT('',(33.9565644528671,15.5074379108486,5.72595023245623E-30));
#28109=CARTESIAN_POINT('Origin',(35.5938999782225,16.2551894587635,0.));
#28110=CARTESIAN_POINT('Origin',(35.5938999782225,16.2551894587635,0.));
#28111=CARTESIAN_POINT('Ctrl Pts',(36.5850719698906,9.50149509066482,0.));
#28112=CARTESIAN_POINT('Ctrl Pts',(36.5247007077103,9.70710072786793,3.24562220582793));
#28113=CARTESIAN_POINT('Ctrl Pts',(37.8155092299557,10.3094485465012,6.16982677025168));
#28114=CARTESIAN_POINT('Ctrl Pts',(39.1063177522012,10.9117963651344,9.09403133467541));
#28115=CARTESIAN_POINT('Ctrl Pts',(41.4806883314343,11.832306710442,11.1176436806954));
#28116=CARTESIAN_POINT('Ctrl Pts',(43.8550589106673,12.7528170557496,13.1412560267153));
#28117=CARTESIAN_POINT('Ctrl Pts',(46.830761065047,13.8498942825606,13.8634749112255));
#28118=CARTESIAN_POINT('Ctrl Pts',(49.8064632194267,14.9469715093716,14.5856937957357));
#28119=CARTESIAN_POINT('Ctrl Pts',(52.7821653738064,16.0440487361825,13.8634749112255));
#28120=CARTESIAN_POINT('Ctrl Pts',(38.928346550052,9.86626475512722,0.));
#28121=CARTESIAN_POINT('Ctrl Pts',(38.8679752878718,10.0718703923303,2.70899372698069));
#28122=CARTESIAN_POINT('Ctrl Pts',(39.9353808672042,10.6086211883239,5.14971273833323));
#28123=CARTESIAN_POINT('Ctrl Pts',(41.0027864465367,11.1453719843175,7.59043174968578));
#28124=CARTESIAN_POINT('Ctrl Pts',(42.9745988326451,11.9476805791743,9.27946171175751));
#28125=CARTESIAN_POINT('Ctrl Pts',(44.9464112187536,12.7499891740311,10.9684916738293));
#28126=CARTESIAN_POINT('Ctrl Pts',(47.4201315169974,13.6996712289063,11.5712994880388));
#28127=CARTESIAN_POINT('Ctrl Pts',(49.8938518152413,14.6493532837814,12.1741073022483));
#28128=CARTESIAN_POINT('Ctrl Pts',(52.3675721134852,15.5990353386566,11.5712994880388));
#28129=CARTESIAN_POINT('Ctrl Pts',(41.2977585211121,9.7668686911201,0.));
#28130=CARTESIAN_POINT('Ctrl Pts',(41.2373872589318,9.97247432832318,2.19648874705823));
#28131=CARTESIAN_POINT('Ctrl Pts',(42.0914327105682,10.4465769382885,4.17545672685568));
#28132=CARTESIAN_POINT('Ctrl Pts',(42.9454781622046,10.9206795482538,6.15442470665314));
#28133=CARTESIAN_POINT('Ctrl Pts',(44.5328288829012,11.6101000126265,7.52391304034141));
#28134=CARTESIAN_POINT('Ctrl Pts',(46.1201796035979,12.2995204769992,8.89340137402968));
#28135=CARTESIAN_POINT('Ctrl Pts',(48.1144840466621,13.1084333356589,9.38216610144961));
#28136=CARTESIAN_POINT('Ctrl Pts',(50.1087884897263,13.9173461943186,9.87093082886955));
#28137=CARTESIAN_POINT('Ctrl Pts',(52.1030929327904,14.7262590529783,9.38216610144962));
#28138=CARTESIAN_POINT('Ctrl Pts',(43.6022501387952,9.20712674149426,0.));
#28139=CARTESIAN_POINT('Ctrl Pts',(43.5418788766149,9.41273237869738,1.72780310113342));
#28140=CARTESIAN_POINT('Ctrl Pts',(44.2008065573392,9.82954324187981,3.28449990511991));
#28141=CARTESIAN_POINT('Ctrl Pts',(44.8597342380634,10.2463541050622,4.84119670910639));
#28142=CARTESIAN_POINT('Ctrl Pts',(46.0954948844274,10.8325384089567,5.91846432228298));
#28143=CARTESIAN_POINT('Ctrl Pts',(47.3312555307913,11.4187227128512,6.99573193545957));
#28144=CARTESIAN_POINT('Ctrl Pts',(48.8871343222931,12.0989021850284,7.3802042952164));
#28145=CARTESIAN_POINT('Ctrl Pts',(50.4430131137949,12.7790816572055,7.76467665497322));
#28146=CARTESIAN_POINT('Ctrl Pts',(51.9988919052966,13.4592611293828,7.38020429521639));
#28147=CARTESIAN_POINT('',(36.5850719699957,9.50149509062496,1.57949199304179E-9));
#28148=CARTESIAN_POINT('Origin',(39.3537269950291,-8.28430119040666,1.04083408558608E-14));
#28149=CARTESIAN_POINT('Ctrl Pts',(36.5850719699169,9.50149509087633,3.13105402820441E-9));
#28150=CARTESIAN_POINT('Ctrl Pts',(36.5805140573471,9.51701791573643,0.245038153335483));
#28151=CARTESIAN_POINT('Ctrl Pts',(36.5819970947817,9.53446325272387,0.490791160521737));
#28152=CARTESIAN_POINT('Ctrl Pts',(36.5896122476099,9.5538253279424,0.736766500725404));
#28153=CARTESIAN_POINT('Ctrl Pts',(36.597202400319,9.57312383855536,0.981934317701064));
#28154=CARTESIAN_POINT('Ctrl Pts',(36.6108845775071,9.59432652559737,1.22732257376573));
#28155=CARTESIAN_POINT('Ctrl Pts',(36.6307008654467,9.61741199666751,1.4724329481635));
#28156=CARTESIAN_POINT('Ctrl Pts',(36.650487309385,9.64046270023582,1.71717417803028));
#28157=CARTESIAN_POINT('Ctrl Pts',(36.6763894565088,9.66539050713801,1.96163791541599));
#28158=CARTESIAN_POINT('Ctrl Pts',(36.7083998596961,9.69215854518714,2.20532408778539));
#28159=CARTESIAN_POINT('Ctrl Pts',(36.7403828091233,9.71890362559676,2.44880126242082));
#28160=CARTESIAN_POINT('Ctrl Pts',(36.77846353496,9.74748574872929,2.69150175431068));
#28161=CARTESIAN_POINT('Ctrl Pts',(36.8225849430252,9.7778529268265,2.93292951866827));
#28162=CARTESIAN_POINT('Ctrl Pts',(36.8666971208038,9.8082137520495,3.17430677585629));
#28163=CARTESIAN_POINT('Ctrl Pts',(36.9168473852605,9.84035883350012,3.41441139318404));
#28164=CARTESIAN_POINT('Ctrl Pts',(36.972929566381,9.87422164256039,3.65275710614716));
#28165=CARTESIAN_POINT('Ctrl Pts',(37.0290829597591,9.90812745007459,3.8914054666886));
#28166=CARTESIAN_POINT('Ctrl Pts',(37.0911832213397,9.94375528237804,4.12829002081229));
#28167=CARTESIAN_POINT('Ctrl Pts',(37.1590759513992,9.98102464057091,4.36293874377867));
#28168=CARTESIAN_POINT('Ctrl Pts',(37.2270379591175,10.0183320283713,4.59782690201507));
#28169=CARTESIAN_POINT('Ctrl Pts',(37.3008040750528,10.0572842076519,4.83047425895017));
#28170=CARTESIAN_POINT('Ctrl Pts',(37.3801738701484,10.0977878566474,5.06042975959489));
#28171=CARTESIAN_POINT('Ctrl Pts',(37.4597757114127,10.1384099224355,5.29105755998366));
#28172=CARTESIAN_POINT('Ctrl Pts',(37.5450138125792,10.180592444572,5.51897736305752));
#28173=CARTESIAN_POINT('Ctrl Pts',(37.6356433288455,10.2242300213427,5.74376259354398));
#28174=CARTESIAN_POINT('Ctrl Pts',(37.6934314033807,10.2520546379008,5.88709234072663));
#28175=CARTESIAN_POINT('Ctrl Pts',(37.7534106234275,10.2804706155742,6.02914825314214));
#28176=CARTESIAN_POINT('Ctrl Pts',(37.8155092299907,10.3094485465061,6.16982677023484));
#28177=CARTESIAN_POINT('Ctrl Pts',(37.9128816718431,10.3548867946542,6.39041482339091));
#28178=CARTESIAN_POINT('Ctrl Pts',(38.0159808925391,10.4021550583218,6.60890054011806));
#28179=CARTESIAN_POINT('Ctrl Pts',(38.124685183118,10.4511851399362,6.82480412008043));
#28180=CARTESIAN_POINT('Ctrl Pts',(38.2331440676596,10.5001045333895,7.04022028559285));
#28181=CARTESIAN_POINT('Ctrl Pts',(38.347182665745,10.5507777480887,7.25306552029621));
#28182=CARTESIAN_POINT('Ctrl Pts',(38.4666322798727,10.6031214810711,7.46287566269393));
#28183=CARTESIAN_POINT('Ctrl Pts',(38.5858897700795,10.6553810238844,7.67234834441863));
#28184=CARTESIAN_POINT('Ctrl Pts',(38.7105407473183,10.7093056453531,7.87879526533015));
#28185=CARTESIAN_POINT('Ctrl Pts',(38.8403712129407,10.7647978150924,8.08177334612187));
#28186=CARTESIAN_POINT('Ctrl Pts',(38.9700771015594,10.820236738098,8.28455666214102));
#28187=CARTESIAN_POINT('Ctrl Pts',(39.1049523499261,10.8772401144471,8.48387739272847));
#28188=CARTESIAN_POINT('Ctrl Pts',(39.2447399831763,10.935697267249,8.67931873611088));
#28189=CARTESIAN_POINT('Ctrl Pts',(39.3845343398416,10.9941572316853,8.87476947970464));
#28190=CARTESIAN_POINT('Ctrl Pts',(39.5292413095784,11.0540710087835,9.06634009532779));
#28191=CARTESIAN_POINT('Ctrl Pts',(39.6785635418397,11.1153159078424,9.25364450340913));
#28192=CARTESIAN_POINT('Ctrl Pts',(39.8279405514883,11.1765832739882,9.44101762226425));
#28193=CARTESIAN_POINT('Ctrl Pts',(39.9819359159956,11.2391826206559,9.62412107874963));
#28194=CARTESIAN_POINT('Ctrl Pts',(40.1402156364348,11.3029807823645,9.80260437466055));
#28195=CARTESIAN_POINT('Ctrl Pts',(40.2987535438823,11.3668830120894,9.9813788137962));
#28196=CARTESIAN_POINT('Ctrl Pts',(40.461589462918,11.4319878421545,10.155517727092));
#28197=CARTESIAN_POINT('Ctrl Pts',(40.6283560345709,11.498152939241,10.3247095747704));
#28198=CARTESIAN_POINT('Ctrl Pts',(40.6765572187104,11.5172768919413,10.3736117457753));
#28199=CARTESIAN_POINT('Ctrl Pts',(40.7250865876886,11.5364893726198,10.4221009095756));
#28200=CARTESIAN_POINT('Ctrl Pts',(40.7739348422944,11.5557868365697,10.4701702229111));
#28201=CARTESIAN_POINT('Ctrl Pts',(41.6582954965894,15.8276282594343,0.));
#28202=CARTESIAN_POINT('Ctrl Pts',(41.5979242344091,16.0332338966374,1.72780310113343));
#28203=CARTESIAN_POINT('Ctrl Pts',(42.2568519151334,16.4500447598199,3.28449990511991));
#28204=CARTESIAN_POINT('Ctrl Pts',(42.9157795958577,16.8668556230023,4.84119670910639));
#28205=CARTESIAN_POINT('Ctrl Pts',(44.1515402422216,17.4530399268967,5.91846432228298));
#28206=CARTESIAN_POINT('Ctrl Pts',(45.3873008885855,18.0392242307912,6.99573193545956));
#28207=CARTESIAN_POINT('Ctrl Pts',(46.9431796800873,18.7194037029684,7.38020429521639));
#28208=CARTESIAN_POINT('Ctrl Pts',(48.4990584715891,19.3995831751456,7.76467665497322));
#28209=CARTESIAN_POINT('Ctrl Pts',(50.0549372630908,20.0797626473228,7.3802042952164));
#28210=CARTESIAN_POINT('Ctrl Pts',(40.0222531270435,14.110841134834,0.));
#28211=CARTESIAN_POINT('Ctrl Pts',(39.9618818648632,14.3164467720371,2.19648874705823));
#28212=CARTESIAN_POINT('Ctrl Pts',(40.8159273164996,14.7905493820025,4.17545672685568));
#28213=CARTESIAN_POINT('Ctrl Pts',(41.669972768136,15.2646519919678,6.15442470665315));
#28214=CARTESIAN_POINT('Ctrl Pts',(43.2573234888327,15.9540724563405,7.52391304034141));
#28215=CARTESIAN_POINT('Ctrl Pts',(44.8446742095293,16.6434929207132,8.89340137402968));
#28216=CARTESIAN_POINT('Ctrl Pts',(46.8389786525935,17.4524057793729,9.38216610144961));
#28217=CARTESIAN_POINT('Ctrl Pts',(48.8332830956577,18.2613186380326,9.87093082886955));
#28218=CARTESIAN_POINT('Ctrl Pts',(50.8275875387219,19.0702314966922,9.38216610144961));
#28219=CARTESIAN_POINT('Ctrl Pts',(38.0827145049534,12.7462230199156,0.));
#28220=CARTESIAN_POINT('Ctrl Pts',(38.0223432427731,12.9518286571187,2.7089937269807));
#28221=CARTESIAN_POINT('Ctrl Pts',(39.0897488221056,13.4885794531123,5.14971273833323));
#28222=CARTESIAN_POINT('Ctrl Pts',(40.1571544014381,14.0253302491059,7.59043174968579));
#28223=CARTESIAN_POINT('Ctrl Pts',(42.1289667875465,14.8276388439627,9.27946171175752));
#28224=CARTESIAN_POINT('Ctrl Pts',(44.1007791736549,15.6299474388195,10.9684916738293));
#28225=CARTESIAN_POINT('Ctrl Pts',(46.5744994718988,16.5796294936946,11.5712994880388));
#28226=CARTESIAN_POINT('Ctrl Pts',(49.0482197701427,17.5293115485698,12.1741073022483));
#28227=CARTESIAN_POINT('Ctrl Pts',(51.5219400683865,18.4789936034449,11.5712994880388));
#28228=CARTESIAN_POINT('Ctrl Pts',(35.9142171164211,11.7862169042729,0.));
#28229=CARTESIAN_POINT('Ctrl Pts',(35.8538458542409,11.991822541476,3.24562220582793));
#28230=CARTESIAN_POINT('Ctrl Pts',(37.1446543764862,12.5941703601092,6.16982677025168));
#28231=CARTESIAN_POINT('Ctrl Pts',(38.4354628987317,13.1965181787425,9.09403133467541));
#28232=CARTESIAN_POINT('Ctrl Pts',(40.8098334779648,14.1170285240501,11.1176436806954));
#28233=CARTESIAN_POINT('Ctrl Pts',(43.1842040571978,15.0375388693576,13.1412560267153));
#28234=CARTESIAN_POINT('Ctrl Pts',(46.1599062115776,16.1346160961686,13.8634749112255));
#28235=CARTESIAN_POINT('Ctrl Pts',(49.1356083659572,17.2316933229796,14.5856937957357));
#28236=CARTESIAN_POINT('Ctrl Pts',(52.1113105203369,18.3287705497906,13.8634749112255));
#28237=CARTESIAN_POINT('',(35.9142171164211,11.7862169042729,0.));
#28238=CARTESIAN_POINT('Ctrl Pts',(35.9142171164211,11.7862169042729,0.));
#28239=CARTESIAN_POINT('Ctrl Pts',(35.8538458542409,11.991822541476,3.24562220582793));
#28240=CARTESIAN_POINT('Ctrl Pts',(37.1446543764862,12.5941703601092,6.16982677025168));
#28241=CARTESIAN_POINT('Ctrl Pts',(38.222270420807,13.0970332266261,8.61106394926975));
#28242=CARTESIAN_POINT('Ctrl Pts',(40.0815233709314,13.8319900590777,10.4489096280657));
#28243=CARTESIAN_POINT('Origin',(28.6276304970128,28.2454287759835,0.));
#28244=CARTESIAN_POINT('Ctrl Pts',(35.9142171164211,11.7862169042729,0.));
#28245=CARTESIAN_POINT('Ctrl Pts',(35.8538458542409,11.991822541476,3.24562220582793));
#28246=CARTESIAN_POINT('Ctrl Pts',(37.1446543764862,12.5941703601092,6.16982677025167));
#28247=CARTESIAN_POINT('Ctrl Pts',(38.4354628987317,13.1965181787425,9.0940313346754));
#28248=CARTESIAN_POINT('Ctrl Pts',(40.8098334779648,14.11702852405,11.1176436806954));
#28249=CARTESIAN_POINT('Ctrl Pts',(43.1842040571979,15.0375388693576,13.1412560267153));
#28250=CARTESIAN_POINT('Ctrl Pts',(46.1599062115776,16.1346160961686,13.8634749112255));
#28251=CARTESIAN_POINT('Ctrl Pts',(49.1356083659572,17.2316933229796,14.5856937957357));
#28252=CARTESIAN_POINT('Ctrl Pts',(52.1113105203369,18.3287705497906,13.8634749112255));
#28253=CARTESIAN_POINT('Ctrl Pts',(35.5109929990849,10.9233088493804,6.24500451351651E-15));
#28254=CARTESIAN_POINT('Ctrl Pts',(35.4506217369045,11.1289144865835,3.38941559469373));
#28255=CARTESIAN_POINT('Ctrl Pts',(36.8012926546625,11.74883949047,6.44317352589573));
#28256=CARTESIAN_POINT('Ctrl Pts',(38.1519635724205,12.3687644943564,9.49693145709774));
#28257=CARTESIAN_POINT('Ctrl Pts',(40.6342024610833,13.3209478330611,11.6101975146502));
#28258=CARTESIAN_POINT('Ctrl Pts',(43.116441349746,14.2731311717657,13.7234635722027));
#28259=CARTESIAN_POINT('Ctrl Pts',(46.226653085872,15.4097039753314,14.4776794959001));
#28260=CARTESIAN_POINT('Ctrl Pts',(49.336864821998,16.5462767788972,15.2318954195974));
#28261=CARTESIAN_POINT('Ctrl Pts',(52.4470765581241,17.682849582463,14.4776794959001));
#28262=CARTESIAN_POINT('Ctrl Pts',(35.7793349404726,10.0094201239371,0.));
#28263=CARTESIAN_POINT('Ctrl Pts',(35.7189636782923,10.2150257611402,3.38941559469373));
#28264=CARTESIAN_POINT('Ctrl Pts',(37.0696345960503,10.8349507650267,6.44317352589573));
#28265=CARTESIAN_POINT('Ctrl Pts',(38.4203055138083,11.4548757689132,9.49693145709775));
#28266=CARTESIAN_POINT('Ctrl Pts',(40.902544402471,12.4070591076178,11.6101975146502));
#28267=CARTESIAN_POINT('Ctrl Pts',(43.3847832911339,13.3592424463224,13.7234635722027));
#28268=CARTESIAN_POINT('Ctrl Pts',(46.4949950272598,14.4958152498882,14.4776794959001));
#28269=CARTESIAN_POINT('Ctrl Pts',(49.6052067633858,15.632388053454,15.2318954195974));
#28270=CARTESIAN_POINT('Ctrl Pts',(52.7154184995118,16.7689608570197,14.4776794959001));
#28271=CARTESIAN_POINT('Ctrl Pts',(36.5850719698906,9.50149509066483,0.));
#28272=CARTESIAN_POINT('Ctrl Pts',(36.5247007077103,9.70710072786794,3.24562220582793));
#28273=CARTESIAN_POINT('Ctrl Pts',(37.8155092299557,10.3094485465012,6.16982677025168));
#28274=CARTESIAN_POINT('Ctrl Pts',(39.1063177522012,10.9117963651344,9.09403133467541));
#28275=CARTESIAN_POINT('Ctrl Pts',(41.4806883314343,11.832306710442,11.1176436806954));
#28276=CARTESIAN_POINT('Ctrl Pts',(43.8550589106673,12.7528170557496,13.1412560267153));
#28277=CARTESIAN_POINT('Ctrl Pts',(46.830761065047,13.8498942825606,13.8634749112255));
#28278=CARTESIAN_POINT('Ctrl Pts',(49.8064632194267,14.9469715093716,14.5856937957357));
#28279=CARTESIAN_POINT('Ctrl Pts',(52.7821653738064,16.0440487361826,13.8634749112255));
#28280=CARTESIAN_POINT('',(35.817874106391,10.5170715743152,8.26137723558795E-30));
#28281=CARTESIAN_POINT('Origin',(37.5449600575355,11.0241949492048,0.));
#28282=CARTESIAN_POINT('Origin',(37.5449600575355,11.0241949492048,0.));
#28283=CARTESIAN_POINT('Ctrl Pts',(37.5648924257372,4.19818497005498,0.));
#28284=CARTESIAN_POINT('Ctrl Pts',(37.5343963889644,4.41028956474376,3.24562220582792));
#28285=CARTESIAN_POINT('Ctrl Pts',(38.8977893740385,4.82280514501199,6.16982677025168));
#28286=CARTESIAN_POINT('Ctrl Pts',(40.2611823591128,5.23532072528026,9.09403133467541));
#28287=CARTESIAN_POINT('Ctrl Pts',(42.7423875503303,5.80855343755452,11.1176436806954));
#28288=CARTESIAN_POINT('Ctrl Pts',(45.2235927415478,6.38178614982881,13.1412560267153));
#28289=CARTESIAN_POINT('Ctrl Pts',(48.325136906711,7.04421014147558,13.8634749112255));
#28290=CARTESIAN_POINT('Ctrl Pts',(51.4266810718742,7.70663413312235,14.5856937957357));
#28291=CARTESIAN_POINT('Ctrl Pts',(54.5282252370374,8.36905812476912,13.8634749112255));
#28292=CARTESIAN_POINT('Ctrl Pts',(39.9362279852005,4.225759062382,0.));
#28293=CARTESIAN_POINT('Ctrl Pts',(39.9057319484277,4.43786365707078,2.7089937269807));
#28294=CARTESIAN_POINT('Ctrl Pts',(41.0386604807592,4.8172434514972,5.14971273833323));
#28295=CARTESIAN_POINT('Ctrl Pts',(42.1715890130907,5.19662324592361,7.59043174968578));
#28296=CARTESIAN_POINT('Ctrl Pts',(44.2375116101495,5.71014733528395,9.27946171175752));
#28297=CARTESIAN_POINT('Ctrl Pts',(46.3034342072083,6.22367142464428,10.9684916738293));
#28298=CARTESIAN_POINT('Ctrl Pts',(48.8871294476768,6.81163998135133,11.5712994880388));
#28299=CARTESIAN_POINT('Ctrl Pts',(51.4708246881453,7.39960853805837,12.1741073022483));
#28300=CARTESIAN_POINT('Ctrl Pts',(54.0545199286137,7.98757709476541,11.5712994880388));
#28301=CARTESIAN_POINT('Ctrl Pts',(42.2673772240309,3.79017222552498,0.));
#28302=CARTESIAN_POINT('Ctrl Pts',(42.236881187258,4.00227682021375,2.19648874705823));
#28303=CARTESIAN_POINT('Ctrl Pts',(43.1497055238908,4.35001040888147,4.17545672685568));
#28304=CARTESIAN_POINT('Ctrl Pts',(44.0625298605235,4.69774399754918,6.15442470665315));
#28305=CARTESIAN_POINT('Ctrl Pts',(45.7318384015437,5.15424359455786,7.52391304034141));
#28306=CARTESIAN_POINT('Ctrl Pts',(47.401146942564,5.61074319156655,8.89340137402969));
#28307=CARTESIAN_POINT('Ctrl Pts',(49.4902725446046,6.12760336939874,9.38216610144961));
#28308=CARTESIAN_POINT('Ctrl Pts',(51.5793981466453,6.64446354723092,9.87093082886955));
#28309=CARTESIAN_POINT('Ctrl Pts',(53.668523748686,7.16132372506311,9.38216610144961));
#28310=CARTESIAN_POINT('Ctrl Pts',(44.4687528548128,2.90816428999238,0.));
#28311=CARTESIAN_POINT('Ctrl Pts',(44.4382568180399,3.12026888468116,1.72780310113342));
#28312=CARTESIAN_POINT('Ctrl Pts',(45.149795935654,3.43906202795197,3.28449990511992));
#28313=CARTESIAN_POINT('Ctrl Pts',(45.8613350532681,3.7578551712228,4.84119670910639));
#28314=CARTESIAN_POINT('Ctrl Pts',(47.1679401624789,4.16220588757978,5.91846432228298));
#28315=CARTESIAN_POINT('Ctrl Pts',(48.4745452716896,4.56655660393679,6.99573193545957));
#28316=CARTESIAN_POINT('Ctrl Pts',(50.1113870920656,5.01838819123964,7.3802042952164));
#28317=CARTESIAN_POINT('Ctrl Pts',(51.7482289124415,5.47021977854247,7.76467665497322));
#28318=CARTESIAN_POINT('Ctrl Pts',(53.3850707328175,5.92205136584531,7.38020429521639));
#28319=CARTESIAN_POINT('',(37.5648924257523,4.19818497006209,1.57948606811744E-9));
#28320=CARTESIAN_POINT('Origin',(37.7741838134883,-13.8005982420128,0.));
#28321=CARTESIAN_POINT('Ctrl Pts',(37.5648924257933,4.19818497026059,3.13104703599162E-9));
#28322=CARTESIAN_POINT('Ctrl Pts',(37.562590034511,4.21419845373592,0.24503815333554));
#28323=CARTESIAN_POINT('Ctrl Pts',(37.5665407070749,4.23125516411427,0.490791160521858));
#28324=CARTESIAN_POINT('Ctrl Pts',(37.5768338592308,4.24933641208172,0.736766500725589));
#28325=CARTESIAN_POINT('Ctrl Pts',(37.5870932195462,4.26735830032753,0.981934317701222));
#28326=CARTESIAN_POINT('Ctrl Pts',(37.6036535888759,4.28639799775346,1.22732257376586));
#28327=CARTESIAN_POINT('Ctrl Pts',(37.6265535806588,4.3064283402013,1.47243294816361));
#28328=CARTESIAN_POINT('Ctrl Pts',(37.649419084278,4.32642851627456,1.71717417803036));
#28329=CARTESIAN_POINT('Ctrl Pts',(37.6786051816996,4.34741633416657,1.96163791541604));
#28330=CARTESIAN_POINT('Ctrl Pts',(37.7140992541436,4.369356356832,2.20532408778542));
#28331=CARTESIAN_POINT('Ctrl Pts',(37.7495628850543,4.39127756261105,2.44880126242083));
#28332=CARTESIAN_POINT('Ctrl Pts',(37.7913236642409,4.41414930860333,2.69150175431066));
#28333=CARTESIAN_POINT('Ctrl Pts',(37.8393176800295,4.43792826156017,2.93292951866823));
#28334=CARTESIAN_POINT('Ctrl Pts',(37.8873016553744,4.46170223991264,3.17430677585613));
#28335=CARTESIAN_POINT('Ctrl Pts',(37.9415161845175,4.48638300400794,3.41441139318375));
#28336=CARTESIAN_POINT('Ctrl Pts',(38.0018467100928,4.51191981196192,3.65275710614676));
#28337=CARTESIAN_POINT('Ctrl Pts',(38.0622538424058,4.53748904614668,3.89140546668832));
#28338=CARTESIAN_POINT('Ctrl Pts',(38.128792382057,4.5639164498048,4.12829002081211));
#28339=CARTESIAN_POINT('Ctrl Pts',(38.2012980447015,4.5911443167709,4.36293874377859));
#28340=CARTESIAN_POINT('Ctrl Pts',(38.2738776920355,4.61839996701916,4.59782690201494));
#28341=CARTESIAN_POINT('Ctrl Pts',(38.3524364483673,4.6464576564197,4.83047425894999));
#28342=CARTESIAN_POINT('Ctrl Pts',(38.4367626436468,4.675253537117,5.06042975959466));
#28343=CARTESIAN_POINT('Ctrl Pts',(38.5213353756664,4.70413360568181,5.29105755998335));
#28344=CARTESIAN_POINT('Ctrl Pts',(38.6117090746819,4.73375612398284,5.51897736305714));
#28345=CARTESIAN_POINT('Ctrl Pts',(38.7076263878304,4.76405160819197,5.74376259354354));
#28346=CARTESIAN_POINT('Ctrl Pts',(38.7687861188958,4.78336890979173,5.88709234072634));
#28347=CARTESIAN_POINT('Ctrl Pts',(38.8321988522325,4.80295972078415,6.029148253142));
#28348=CARTESIAN_POINT('Ctrl Pts',(38.8977893740739,4.8228051450119,6.16982677023485));
#28349=CARTESIAN_POINT('Ctrl Pts',(39.0006372418043,4.85392335399592,6.39041482339099));
#28350=CARTESIAN_POINT('Ctrl Pts',(39.1094140363897,4.88603794597511,6.60890054011821));
#28351=CARTESIAN_POINT('Ctrl Pts',(39.2239895821647,4.91909873852093,6.82480412008064));
#28352=CARTESIAN_POINT('Ctrl Pts',(39.3383064672143,4.95208489447194,7.04022028559313));
#28353=CARTESIAN_POINT('Ctrl Pts',(39.458395867156,4.98601294426688,7.25306552029656));
#28354=CARTESIAN_POINT('Ctrl Pts',(39.584078946338,5.02082444100455,7.46287566269435));
#28355=CARTESIAN_POINT('Ctrl Pts',(39.7095598756334,5.05557994659237,7.67234834441894));
#28356=CARTESIAN_POINT('Ctrl Pts',(39.8406163594389,5.091216009501,7.87879526533036));
#28357=CARTESIAN_POINT('Ctrl Pts',(39.9770226972832,5.12766654724745,8.08177334612198));
#28358=CARTESIAN_POINT('Ctrl Pts',(40.1132981483379,5.16408210939131,8.28455666214124));
#28359=CARTESIAN_POINT('Ctrl Pts',(40.2549129874365,5.20131052440296,8.48387739272877));
#28360=CARTESIAN_POINT('Ctrl Pts',(40.4015971043843,5.23927881325903,8.67931873611127));
#28361=CARTESIAN_POINT('Ctrl Pts',(40.5482882764499,5.27724892828933,8.87476947970516));
#28362=CARTESIAN_POINT('Ctrl Pts',(40.7000489573831,5.31595892053015,9.06634009532842));
#28363=CARTESIAN_POINT('Ctrl Pts',(40.8565673625296,5.35532966548965,9.25364450340988));
#28364=CARTESIAN_POINT('Ctrl Pts',(41.0131431849084,5.3947148532184,9.44101762226502));
#28365=CARTESIAN_POINT('Ctrl Pts',(41.1744799145451,5.43476120340312,9.62412107875041));
#28366=CARTESIAN_POINT('Ctrl Pts',(41.3402280007164,5.47538443899869,9.80260437466134));
#28367=CARTESIAN_POINT('Ctrl Pts',(41.5062464563474,5.51607393950573,9.98137881379686));
#28368=CARTESIAN_POINT('Ctrl Pts',(41.6766903238787,5.55734212879157,10.1555177270925));
#28369=CARTESIAN_POINT('Ctrl Pts',(41.8511757273808,5.59910040291772,10.3247095747708));
#28370=CARTESIAN_POINT('Ctrl Pts',(41.9016079152,5.61116995762813,10.3736117457739));
#28371=CARTESIAN_POINT('Ctrl Pts',(41.9523775462543,5.62328043365736,10.4221009095724));
#28372=CARTESIAN_POINT('Ctrl Pts',(42.0034749115207,5.63542964579433,10.4701702229062));
#28373=CARTESIAN_POINT('Ctrl Pts',(43.4867804707272,9.73793223897082,1.04083408558608E-14));
#28374=CARTESIAN_POINT('Ctrl Pts',(43.4562844339543,9.9500368336596,1.72780310113343));
#28375=CARTESIAN_POINT('Ctrl Pts',(44.1678235515684,10.2688299769304,3.28449990511991));
#28376=CARTESIAN_POINT('Ctrl Pts',(44.8793626691825,10.5876231202012,4.84119670910638));
#28377=CARTESIAN_POINT('Ctrl Pts',(46.1859677783933,10.9919738365582,5.91846432228298));
#28378=CARTESIAN_POINT('Ctrl Pts',(47.492572887604,11.3963245529152,6.99573193545956));
#28379=CARTESIAN_POINT('Ctrl Pts',(49.12941470798,11.8481561402181,7.3802042952164));
#28380=CARTESIAN_POINT('Ctrl Pts',(50.7662565283559,12.2999877275209,7.76467665497321));
#28381=CARTESIAN_POINT('Ctrl Pts',(52.4030983487318,12.7518193148238,7.3802042952164));
#28382=CARTESIAN_POINT('Ctrl Pts',(41.6230663715378,8.27145263712653,0.));
#28383=CARTESIAN_POINT('Ctrl Pts',(41.5925703347649,8.48355723181529,2.19648874705823));
#28384=CARTESIAN_POINT('Ctrl Pts',(42.5053946713977,8.83129082048301,4.17545672685568));
#28385=CARTESIAN_POINT('Ctrl Pts',(43.4182190080304,9.17902440915073,6.15442470665315));
#28386=CARTESIAN_POINT('Ctrl Pts',(45.0875275490506,9.63552400615941,7.52391304034141));
#28387=CARTESIAN_POINT('Ctrl Pts',(46.7568360900709,10.0920236031681,8.89340137402968));
#28388=CARTESIAN_POINT('Ctrl Pts',(48.8459616921115,10.6088837810003,9.38216610144961));
#28389=CARTESIAN_POINT('Ctrl Pts',(50.9350872941522,11.1257439588325,9.87093082886954));
#28390=CARTESIAN_POINT('Ctrl Pts',(53.0242128961929,11.6426041366647,9.38216610144961));
#28391=CARTESIAN_POINT('Ctrl Pts',(39.5090640497074,7.19674949232866,0.));
#28392=CARTESIAN_POINT('Ctrl Pts',(39.4785680129346,7.40885408701741,2.70899372698069));
#28393=CARTESIAN_POINT('Ctrl Pts',(40.6114965452661,7.78823388144385,5.14971273833323));
#28394=CARTESIAN_POINT('Ctrl Pts',(41.7444250775976,8.16761367587025,7.59043174968578));
#28395=CARTESIAN_POINT('Ctrl Pts',(43.8103476746564,8.6811377652306,9.27946171175751));
#28396=CARTESIAN_POINT('Ctrl Pts',(45.8762702717153,9.19466185459093,10.9684916738292));
#28397=CARTESIAN_POINT('Ctrl Pts',(48.4599655121837,9.78263041129798,11.5712994880388));
#28398=CARTESIAN_POINT('Ctrl Pts',(51.0436607526522,10.370598968005,12.1741073022483));
#28399=CARTESIAN_POINT('Ctrl Pts',(53.6273559931206,10.9585675247121,11.5712994880388));
#28400=CARTESIAN_POINT('Ctrl Pts',(37.2260157227863,6.55512420987368,0.));
#28401=CARTESIAN_POINT('Ctrl Pts',(37.1955196860134,6.76722880456246,3.24562220582792));
#28402=CARTESIAN_POINT('Ctrl Pts',(38.5589126710877,7.17974438483072,6.16982677025168));
#28403=CARTESIAN_POINT('Ctrl Pts',(39.9223056561619,7.59225996509896,9.0940313346754));
#28404=CARTESIAN_POINT('Ctrl Pts',(42.4035108473794,8.16549267737322,11.1176436806954));
#28405=CARTESIAN_POINT('Ctrl Pts',(44.8847160385968,8.7387253896475,13.1412560267153));
#28406=CARTESIAN_POINT('Ctrl Pts',(47.9862602037601,9.40114938129427,13.8634749112255));
#28407=CARTESIAN_POINT('Ctrl Pts',(51.0878043689233,10.0635733729411,14.5856937957357));
#28408=CARTESIAN_POINT('Ctrl Pts',(54.1893485340865,10.7259973645878,13.8634749112255));
#28409=CARTESIAN_POINT('',(37.2260157227863,6.55512420987368,0.));
#28410=CARTESIAN_POINT('Ctrl Pts',(37.2260157227863,6.55512420987368,0.));
#28411=CARTESIAN_POINT('Ctrl Pts',(37.1955196860134,6.76722880456246,3.24562220582792));
#28412=CARTESIAN_POINT('Ctrl Pts',(38.5589126710877,7.17974438483072,6.16982677025168));
#28413=CARTESIAN_POINT('Ctrl Pts',(39.6971249853933,7.52412807936664,8.61106394926976));
#28414=CARTESIAN_POINT('Ctrl Pts',(41.6420486840549,7.98700482807798,10.4489096280657));
#28415=CARTESIAN_POINT('Origin',(32.3559861244014,23.8837944332594,0.));
#28416=CARTESIAN_POINT('Ctrl Pts',(37.2260157227863,6.55512420987368,0.));
#28417=CARTESIAN_POINT('Ctrl Pts',(37.1955196860134,6.76722880456246,3.24562220582792));
#28418=CARTESIAN_POINT('Ctrl Pts',(38.5589126710877,7.17974438483072,6.16982677025168));
#28419=CARTESIAN_POINT('Ctrl Pts',(39.9223056561619,7.59225996509896,9.0940313346754));
#28420=CARTESIAN_POINT('Ctrl Pts',(42.4035108473794,8.16549267737322,11.1176436806954));
#28421=CARTESIAN_POINT('Ctrl Pts',(44.8847160385968,8.7387253896475,13.1412560267153));
#28422=CARTESIAN_POINT('Ctrl Pts',(47.9862602037601,9.40114938129427,13.8634749112255));
#28423=CARTESIAN_POINT('Ctrl Pts',(51.0878043689233,10.0635733729411,14.5856937957357));
#28424=CARTESIAN_POINT('Ctrl Pts',(54.1893485340865,10.7259973645878,13.8634749112255));
#28425=CARTESIAN_POINT('Ctrl Pts',(36.7040912252866,5.75838408981591,0.));
#28426=CARTESIAN_POINT('Ctrl Pts',(36.6735951885137,5.97048868450468,3.38941559469373));
#28427=CARTESIAN_POINT('Ctrl Pts',(38.0987427505052,6.39188323248848,6.44317352589574));
#28428=CARTESIAN_POINT('Ctrl Pts',(39.5238903124967,6.81327778047227,9.49693145709775));
#28429=CARTESIAN_POINT('Ctrl Pts',(42.1163734062201,7.40250983972819,11.6101975146502));
#28430=CARTESIAN_POINT('Ctrl Pts',(44.7088564999435,7.99174189898409,13.7234635722027));
#28431=CARTESIAN_POINT('Ctrl Pts',(47.949161939876,8.67411674998977,14.4776794959001));
#28432=CARTESIAN_POINT('Ctrl Pts',(51.1894673798085,9.35649160099544,15.2318954195974));
#28433=CARTESIAN_POINT('Ctrl Pts',(54.4297728197411,10.0388664520011,14.4776794959001));
#28434=CARTESIAN_POINT('Ctrl Pts',(36.8396419064669,4.81560839388842,6.24500451351652E-15));
#28435=CARTESIAN_POINT('Ctrl Pts',(36.8091458696941,5.0277129885772,3.38941559469373));
#28436=CARTESIAN_POINT('Ctrl Pts',(38.2342934316856,5.44910753656099,6.44317352589574));
#28437=CARTESIAN_POINT('Ctrl Pts',(39.6594409936771,5.87050208454479,9.49693145709774));
#28438=CARTESIAN_POINT('Ctrl Pts',(42.2519240874005,6.45973414380071,11.6101975146502));
#28439=CARTESIAN_POINT('Ctrl Pts',(44.8444071811239,7.04896620305661,13.7234635722027));
#28440=CARTESIAN_POINT('Ctrl Pts',(48.0847126210564,7.73134105406228,14.4776794959001));
#28441=CARTESIAN_POINT('Ctrl Pts',(51.3250180609889,8.41371590506795,15.2318954195974));
#28442=CARTESIAN_POINT('Ctrl Pts',(54.5653235009214,9.09609075607363,14.4776794959001));
#28443=CARTESIAN_POINT('Ctrl Pts',(37.5648924257372,4.19818497005498,0.));
#28444=CARTESIAN_POINT('Ctrl Pts',(37.5343963889644,4.41028956474376,3.24562220582792));
#28445=CARTESIAN_POINT('Ctrl Pts',(38.8977893740386,4.822805145012,6.16982677025168));
#28446=CARTESIAN_POINT('Ctrl Pts',(40.2611823591128,5.23532072528026,9.09403133467541));
#28447=CARTESIAN_POINT('Ctrl Pts',(42.7423875503303,5.80855343755452,11.1176436806954));
#28448=CARTESIAN_POINT('Ctrl Pts',(45.2235927415478,6.38178614982881,13.1412560267153));
#28449=CARTESIAN_POINT('Ctrl Pts',(48.325136906711,7.04421014147557,13.8634749112255));
#28450=CARTESIAN_POINT('Ctrl Pts',(51.4266810718742,7.70663413312235,14.5856937957357));
#28451=CARTESIAN_POINT('Ctrl Pts',(54.5282252370374,8.36905812476912,13.8634749112255));
#28452=CARTESIAN_POINT('',(36.9500351333054,5.31260798930611,1.06286264225831E-29));
#28453=CARTESIAN_POINT('Origin',(38.731713020801,5.56877962163325,0.));
#28454=CARTESIAN_POINT('Origin',(38.731713020801,5.56877962163325,0.));
#28455=CARTESIAN_POINT('Ctrl Pts',(37.78,-1.19058808997946,0.));
#28456=CARTESIAN_POINT('Ctrl Pts',(37.78,-0.976302375693734,3.24562220582793));
#28457=CARTESIAN_POINT('Ctrl Pts',(39.1882226984276,-0.762016661408056,
6.16982677025167));
#28458=CARTESIAN_POINT('Ctrl Pts',(40.5964453968552,-0.547730947122339,
9.09403133467541));
#28459=CARTESIAN_POINT('Ctrl Pts',(43.1339750175689,-0.33344523283667,11.1176436806954));
#28460=CARTESIAN_POINT('Ctrl Pts',(45.6715046382825,-0.119159518550966,
13.1412560267153));
#28461=CARTESIAN_POINT('Ctrl Pts',(48.8357523191413,0.0951261957347176,
13.8634749112255));
#28462=CARTESIAN_POINT('Ctrl Pts',(52.0000000000001,0.309411910020398,14.5856937957357));
#28463=CARTESIAN_POINT('Ctrl Pts',(55.1642476808588,0.523697624306074,13.8634749112255));
#28464=CARTESIAN_POINT('Ctrl Pts',(40.1311229851415,-1.50077089879047,0.));
#28465=CARTESIAN_POINT('Ctrl Pts',(40.1311229851416,-1.28648518450476,2.70899372698069));
#28466=CARTESIAN_POINT('Ctrl Pts',(41.30651131265,-1.07219947021906,5.14971273833323));
#28467=CARTESIAN_POINT('Ctrl Pts',(42.4818996401583,-0.857913755933361,
7.59043174968578));
#28468=CARTESIAN_POINT('Ctrl Pts',(44.5998762217203,-0.643628041647661,
9.27946171175752));
#28469=CARTESIAN_POINT('Ctrl Pts',(46.7178528032822,-0.429342327361976,
10.9684916738293));
#28470=CARTESIAN_POINT('Ctrl Pts',(49.3589264016411,-0.21505661307629,11.5712994880388));
#28471=CARTESIAN_POINT('Ctrl Pts',(52.0000000000001,-0.000770898790611535,
12.1741073022483));
#28472=CARTESIAN_POINT('Ctrl Pts',(54.641073598359,0.213514815495078,11.5712994880388));
#28473=CARTESIAN_POINT('Ctrl Pts',(42.376554015719,-2.2636812166277,0.));
#28474=CARTESIAN_POINT('Ctrl Pts',(42.3765540157191,-2.04939550234198,2.19648874705824));
#28475=CARTESIAN_POINT('Ctrl Pts',(43.3295747662223,-1.83510978805626,4.17545672685568));
#28476=CARTESIAN_POINT('Ctrl Pts',(44.2825955167256,-1.62082407377057,6.15442470665314));
#28477=CARTESIAN_POINT('Ctrl Pts',(45.9998795700625,-1.40653835948487,7.5239130403414));
#28478=CARTESIAN_POINT('Ctrl Pts',(47.7171636233994,-1.19225264519917,8.89340137402968));
#28479=CARTESIAN_POINT('Ctrl Pts',(49.8585818116997,-0.977966930913482,
9.38216610144961));
#28480=CARTESIAN_POINT('Ctrl Pts',(52.0000000000001,-0.763681216627804,
9.87093082886955));
#28481=CARTESIAN_POINT('Ctrl Pts',(54.1414181883005,-0.549395502342091,
9.38216610144961));
#28482=CARTESIAN_POINT('Ctrl Pts',(44.43,-3.45000000000046,0.));
#28483=CARTESIAN_POINT('Ctrl Pts',(44.43,-3.23571428571475,1.72780310113343));
#28484=CARTESIAN_POINT('Ctrl Pts',(45.1796656699787,-3.02142857142903,3.28449990511992));
#28485=CARTESIAN_POINT('Ctrl Pts',(45.9293313399574,-2.80714285714333,4.84119670910639));
#28486=CARTESIAN_POINT('Ctrl Pts',(47.2801821999294,-2.59285714285764,5.91846432228298));
#28487=CARTESIAN_POINT('Ctrl Pts',(48.6310330599014,-2.37857142857193,6.99573193545956));
#28488=CARTESIAN_POINT('Ctrl Pts',(50.3155165299507,-2.16428571428624,7.38020429521639));
#28489=CARTESIAN_POINT('Ctrl Pts',(52.,-1.95000000000054,7.76467665497322));
#28490=CARTESIAN_POINT('Ctrl Pts',(53.6844834700493,-1.73571428571485,7.38020429521639));
#28491=CARTESIAN_POINT('',(37.7799999998362,-1.19058808962906,-2.44188901215463E-9));
#28492=CARTESIAN_POINT('Origin',(35.4256671812558,-19.0359549110505,1.04083408558608E-14));
#28493=CARTESIAN_POINT('Ctrl Pts',(37.78,-1.19058808997946,0.));
#28494=CARTESIAN_POINT('Ctrl Pts',(37.78,-0.976302375693734,3.24562220582793));
#28495=CARTESIAN_POINT('Ctrl Pts',(39.1882226984276,-0.762016661408056,
6.16982677025167));
#28496=CARTESIAN_POINT('Ctrl Pts',(40.3709173991841,-0.582048976597612,
8.62571762198518));
#28497=CARTESIAN_POINT('Ctrl Pts',(42.3779453595727,-0.399648641330362,
10.4701702229062));
#28498=CARTESIAN_POINT('Ctrl Pts',(44.4300000000001,3.44999999999955,0.));
#28499=CARTESIAN_POINT('Ctrl Pts',(44.43,3.66428571428526,1.72780310113343));
#28500=CARTESIAN_POINT('Ctrl Pts',(45.1796656699788,3.87857142857096,3.28449990511991));
#28501=CARTESIAN_POINT('Ctrl Pts',(45.9293313399575,4.09285714285668,4.84119670910639));
#28502=CARTESIAN_POINT('Ctrl Pts',(47.2801821999295,4.30714285714236,5.91846432228298));
#28503=CARTESIAN_POINT('Ctrl Pts',(48.6310330599015,4.52142857142807,6.99573193545957));
#28504=CARTESIAN_POINT('Ctrl Pts',(50.3155165299508,4.73571428571376,7.38020429521639));
#28505=CARTESIAN_POINT('Ctrl Pts',(52.0000000000001,4.94999999999945,7.76467665497322));
#28506=CARTESIAN_POINT('Ctrl Pts',(53.6844834700494,5.16428571428516,7.38020429521639));
#28507=CARTESIAN_POINT('Ctrl Pts',(42.3765540157191,2.26368121662681,0.));
#28508=CARTESIAN_POINT('Ctrl Pts',(42.3765540157191,2.47796693091252,2.19648874705823));
#28509=CARTESIAN_POINT('Ctrl Pts',(43.3295747662223,2.69225264519823,4.17545672685568));
#28510=CARTESIAN_POINT('Ctrl Pts',(44.2825955167256,2.90653835948393,6.15442470665313));
#28511=CARTESIAN_POINT('Ctrl Pts',(45.9998795700625,3.12082407376963,7.5239130403414));
#28512=CARTESIAN_POINT('Ctrl Pts',(47.7171636233994,3.33510978805533,8.89340137402968));
#28513=CARTESIAN_POINT('Ctrl Pts',(49.8585818116998,3.54939550234102,9.3821661014496));
#28514=CARTESIAN_POINT('Ctrl Pts',(52.0000000000001,3.7636812166267,9.87093082886954));
#28515=CARTESIAN_POINT('Ctrl Pts',(54.1414181883005,3.97796693091241,9.3821661014496));
#28516=CARTESIAN_POINT('Ctrl Pts',(40.1311229851416,1.50077089878964,-1.05434036998093E-14));
#28517=CARTESIAN_POINT('Ctrl Pts',(40.1311229851416,1.71505661307536,2.70899372698069));
#28518=CARTESIAN_POINT('Ctrl Pts',(41.30651131265,1.92934232736107,5.14971273833323));
#28519=CARTESIAN_POINT('Ctrl Pts',(42.4818996401584,2.14362804164676,7.59043174968578));
#28520=CARTESIAN_POINT('Ctrl Pts',(44.5998762217203,2.35791375593245,9.2794617117575));
#28521=CARTESIAN_POINT('Ctrl Pts',(46.7178528032822,2.57219947021815,10.9684916738292));
#28522=CARTESIAN_POINT('Ctrl Pts',(49.3589264016411,2.78648518450383,11.5712994880388));
#28523=CARTESIAN_POINT('Ctrl Pts',(52.0000000000001,3.00077089878951,12.1741073022483));
#28524=CARTESIAN_POINT('Ctrl Pts',(54.641073598359,3.2150566130752,11.5712994880388));
#28525=CARTESIAN_POINT('Ctrl Pts',(37.78,1.19058808997868,0.));
#28526=CARTESIAN_POINT('Ctrl Pts',(37.7800000000001,1.4048738042644,3.24562220582793));
#28527=CARTESIAN_POINT('Ctrl Pts',(39.1882226984277,1.6191595185501,6.16982677025167));
#28528=CARTESIAN_POINT('Ctrl Pts',(40.5964453968553,1.8334452328358,9.09403133467541));
#28529=CARTESIAN_POINT('Ctrl Pts',(43.1339750175689,2.04773094712147,11.1176436806954));
#28530=CARTESIAN_POINT('Ctrl Pts',(45.6715046382825,2.26201666140717,13.1412560267153));
#28531=CARTESIAN_POINT('Ctrl Pts',(48.8357523191413,2.47630237569286,13.8634749112255));
#28532=CARTESIAN_POINT('Ctrl Pts',(52.0000000000001,2.69058808997853,14.5856937957357));
#28533=CARTESIAN_POINT('Ctrl Pts',(55.1642476808589,2.90487380426421,13.8634749112255));
#28534=CARTESIAN_POINT('',(37.78,1.19058808997869,0.));
#28535=CARTESIAN_POINT('Ctrl Pts',(37.78,1.19058808997869,0.));
#28536=CARTESIAN_POINT('Ctrl Pts',(37.7800000000001,1.4048738042644,3.24562220582793));
#28537=CARTESIAN_POINT('Ctrl Pts',(39.1882226984277,1.6191595185501,6.16982677025167));
#28538=CARTESIAN_POINT('Ctrl Pts',(40.3638605623321,1.79805338220488,8.61106394926975));
#28539=CARTESIAN_POINT('Ctrl Pts',(42.3548619717231,1.97942721139859,10.4489096280657));
#28540=CARTESIAN_POINT('Origin',(35.4256671812562,19.0359549110498,0.));
#28541=CARTESIAN_POINT('Ctrl Pts',(37.78,1.19058808997868,0.));
#28542=CARTESIAN_POINT('Ctrl Pts',(37.7800000000001,1.4048738042644,3.24562220582793));
#28543=CARTESIAN_POINT('Ctrl Pts',(39.1882226984277,1.6191595185501,6.16982677025167));
#28544=CARTESIAN_POINT('Ctrl Pts',(40.5964453968553,1.8334452328358,9.09403133467541));
#28545=CARTESIAN_POINT('Ctrl Pts',(43.1339750175689,2.04773094712147,11.1176436806954));
#28546=CARTESIAN_POINT('Ctrl Pts',(45.6715046382825,2.26201666140717,13.1412560267153));
#28547=CARTESIAN_POINT('Ctrl Pts',(48.8357523191413,2.47630237569286,13.8634749112255));
#28548=CARTESIAN_POINT('Ctrl Pts',(52.0000000000001,2.69058808997853,14.5856937957357));
#28549=CARTESIAN_POINT('Ctrl Pts',(55.1642476808589,2.90487380426421,13.8634749112255));
#28550=CARTESIAN_POINT('Ctrl Pts',(37.15,0.476235235991243,0.));
#28551=CARTESIAN_POINT('Ctrl Pts',(37.1500000000001,0.69052095027696,3.38941559469373));
#28552=CARTESIAN_POINT('Ctrl Pts',(38.6206123116491,0.904806664562659,6.44317352589573));
#28553=CARTESIAN_POINT('Ctrl Pts',(40.0912246232982,1.11909237884837,9.49693145709774));
#28554=CARTESIAN_POINT('Ctrl Pts',(42.7411764423978,1.33337809313404,11.6101975146502));
#28555=CARTESIAN_POINT('Ctrl Pts',(45.3911282614975,1.54766380741972,13.7234635722027));
#28556=CARTESIAN_POINT('Ctrl Pts',(48.6955641307488,1.76194952170541,14.4776794959001));
#28557=CARTESIAN_POINT('Ctrl Pts',(52.,1.97623523599108,15.2318954195974));
#28558=CARTESIAN_POINT('Ctrl Pts',(55.3044358692513,2.19052095027676,14.4776794959001));
#28559=CARTESIAN_POINT('Ctrl Pts',(37.15,-0.476235235992009,0.));
#28560=CARTESIAN_POINT('Ctrl Pts',(37.15,-0.261949521706298,3.38941559469373));
#28561=CARTESIAN_POINT('Ctrl Pts',(38.6206123116491,-0.0476638074206039,
6.44317352589573));
#28562=CARTESIAN_POINT('Ctrl Pts',(40.0912246232982,0.166621906865105,9.49693145709774));
#28563=CARTESIAN_POINT('Ctrl Pts',(42.7411764423978,0.380907621150789,11.6101975146502));
#28564=CARTESIAN_POINT('Ctrl Pts',(45.3911282614975,0.595193335436467,13.7234635722027));
#28565=CARTESIAN_POINT('Ctrl Pts',(48.6955641307488,0.80947904972215,14.4776794959001));
#28566=CARTESIAN_POINT('Ctrl Pts',(52.,1.02376476400783,15.2318954195974));
#28567=CARTESIAN_POINT('Ctrl Pts',(55.3044358692513,1.23805047829351,14.4776794959001));
#28568=CARTESIAN_POINT('Ctrl Pts',(37.7800000000001,-1.19058808997946,0.));
#28569=CARTESIAN_POINT('Ctrl Pts',(37.7800000000001,-0.976302375693737,
3.24562220582793));
#28570=CARTESIAN_POINT('Ctrl Pts',(39.1882226984276,-0.762016661408056,
6.16982677025167));
#28571=CARTESIAN_POINT('Ctrl Pts',(40.5964453968553,-0.547730947122335,
9.09403133467541));
#28572=CARTESIAN_POINT('Ctrl Pts',(43.1339750175689,-0.333445232836653,
11.1176436806954));
#28573=CARTESIAN_POINT('Ctrl Pts',(45.6715046382825,-0.11915951855097,13.1412560267153));
#28574=CARTESIAN_POINT('Ctrl Pts',(48.8357523191413,0.095126195734721,13.8634749112255));
#28575=CARTESIAN_POINT('Ctrl Pts',(52.0000000000001,0.309411910020398,14.5856937957357));
#28576=CARTESIAN_POINT('Ctrl Pts',(55.1642476808589,0.523697624306077,13.8634749112255));
#28577=CARTESIAN_POINT('',(37.3300000000069,-4.97400852990502E-6,1.27795074265261E-29));
#28578=CARTESIAN_POINT('Origin',(39.13,-4.02455846426619E-13,0.));
#28579=CARTESIAN_POINT('Origin',(39.13,-4.02455846426619E-13,0.));
#28580=CARTESIAN_POINT('Ctrl Pts',(37.2260157227862,-6.55512420987448,0.));
#28581=CARTESIAN_POINT('Ctrl Pts',(37.256511759559,-6.34301961518571,3.24562220582792));
#28582=CARTESIAN_POINT('Ctrl Pts',(38.6808968181789,-6.33132600607645,6.16982677025168));
#28583=CARTESIAN_POINT('Ctrl Pts',(40.1052818767988,-6.31963239696717,9.09403133467541));
#28584=CARTESIAN_POINT('Ctrl Pts',(42.647479141562,-6.46865591986398,11.1176436806954));
#28585=CARTESIAN_POINT('Ctrl Pts',(45.1896764063252,-6.61767944276075,13.1412560267153));
#28586=CARTESIAN_POINT('Ctrl Pts',(48.3522126450341,-6.85589424503005,13.8634749112255));
#28587=CARTESIAN_POINT('Ctrl Pts',(51.5147488837429,-7.09410904729936,14.5856937957357));
#28588=CARTESIAN_POINT('Ctrl Pts',(54.6772851224518,-7.33232384956867,13.8634749112255));
#28589=CARTESIAN_POINT('Ctrl Pts',(39.5090640497072,-7.1967494923295,-1.05434036998093E-14));
#28590=CARTESIAN_POINT('Ctrl Pts',(39.5395600864801,-6.98464489764072,2.70899372698069));
#28591=CARTESIAN_POINT('Ctrl Pts',(40.7334806923573,-6.93981550268964,5.14971273833323));
#28592=CARTESIAN_POINT('Ctrl Pts',(41.9274012982345,-6.89498610773854,7.59043174968577));
#28593=CARTESIAN_POINT('Ctrl Pts',(44.054315968839,-6.98430100772137,9.27946171175751));
#28594=CARTESIAN_POINT('Ctrl Pts',(46.1812306394436,-7.07361590770423,10.9684916738293));
#28595=CARTESIAN_POINT('Ctrl Pts',(48.8259179534577,-7.23737527503378,11.5712994880388));
#28596=CARTESIAN_POINT('Ctrl Pts',(51.4706052674719,-7.40113464236333,12.1741073022483));
#28597=CARTESIAN_POINT('Ctrl Pts',(54.115292581486,-7.56489400969289,11.5712994880388));
#28598=CARTESIAN_POINT('Ctrl Pts',(41.6230663715376,-8.27145263712742,0.));
#28599=CARTESIAN_POINT('Ctrl Pts',(41.6535624083104,-8.05934804243867,2.19648874705824));
#28600=CARTESIAN_POINT('Ctrl Pts',(42.6273788184889,-7.98287244172884,4.17545672685568));
#28601=CARTESIAN_POINT('Ctrl Pts',(43.6011952286674,-7.90639684101905,6.15442470665314));
#28602=CARTESIAN_POINT('Ctrl Pts',(45.3314958432332,-7.93868724865023,7.5239130403414));
#28603=CARTESIAN_POINT('Ctrl Pts',(47.0617964577991,-7.97097765628139,8.89340137402967));
#28604=CARTESIAN_POINT('Ctrl Pts',(49.2119141333854,-8.06362864473609,9.38216610144961));
#28605=CARTESIAN_POINT('Ctrl Pts',(51.3620318089718,-8.15627963319078,9.87093082886954));
#28606=CARTESIAN_POINT('Ctrl Pts',(53.5121494845582,-8.24893062164547,9.3821661014496));
#28607=CARTESIAN_POINT('Ctrl Pts',(43.4867804707269,-9.73793223897177,0.));
#28608=CARTESIAN_POINT('Ctrl Pts',(43.5172765074998,-9.525827644283,1.72780310113342));
#28609=CARTESIAN_POINT('Ctrl Pts',(44.2898076986596,-9.42041159817628,3.28449990511991));
#28610=CARTESIAN_POINT('Ctrl Pts',(45.0623388898194,-9.31499555206956,4.84119670910639));
#28611=CARTESIAN_POINT('Ctrl Pts',(46.4299360725758,-9.29513707904906,5.91846432228298));
#28612=CARTESIAN_POINT('Ctrl Pts',(47.7975332553323,-9.27527860602855,6.99573193545956));
#28613=CARTESIAN_POINT('Ctrl Pts',(49.4953671492539,-9.30290100395389,7.38020429521639));
#28614=CARTESIAN_POINT('Ctrl Pts',(51.1932010431756,-9.33052340187922,7.76467665497322));
#28615=CARTESIAN_POINT('Ctrl Pts',(52.8910349370971,-9.35814579980457,7.38020429521639));
#28616=CARTESIAN_POINT('',(37.226015722685,-6.55512420967655,-1.21941697785192E-9));
#28617=CARTESIAN_POINT('Origin',(32.3559861244009,-23.8837944332601,0.));
#28618=CARTESIAN_POINT('Ctrl Pts',(37.2260157227862,-6.55512420987448,0.));
#28619=CARTESIAN_POINT('Ctrl Pts',(37.256511759559,-6.34301961518571,3.24562220582792));
#28620=CARTESIAN_POINT('Ctrl Pts',(38.6808968181789,-6.33132600607645,6.16982677025168));
#28621=CARTESIAN_POINT('Ctrl Pts',(39.8771654641448,-6.32150513787023,8.62571762198518));
#28622=CARTESIAN_POINT('Ctrl Pts',(41.8897230480066,-6.42659123460911,10.4701702229062));
#28623=CARTESIAN_POINT('Ctrl Pts',(44.4687528548127,-2.90816428999336,0.));
#28624=CARTESIAN_POINT('Ctrl Pts',(44.4992488915855,-2.69605969530457,1.72780310113343));
#28625=CARTESIAN_POINT('Ctrl Pts',(45.2717800827454,-2.59064364919786,3.28449990511992));
#28626=CARTESIAN_POINT('Ctrl Pts',(46.0443112739052,-2.48522760309115,4.84119670910639));
#28627=CARTESIAN_POINT('Ctrl Pts',(47.4119084566616,-2.46536913007065,5.91846432228298));
#28628=CARTESIAN_POINT('Ctrl Pts',(48.779505639418,-2.44551065705014,6.99573193545957));
#28629=CARTESIAN_POINT('Ctrl Pts',(50.4773395333396,-2.47313305497548,7.3802042952164));
#28630=CARTESIAN_POINT('Ctrl Pts',(52.1751734272613,-2.50075545290081,7.76467665497322));
#28631=CARTESIAN_POINT('Ctrl Pts',(53.8730073211829,-2.52837785082615,7.3802042952164));
#28632=CARTESIAN_POINT('Ctrl Pts',(42.2673772240308,-3.7901722255259,0.));
#28633=CARTESIAN_POINT('Ctrl Pts',(42.2978732608037,-3.57806763083714,2.19648874705823));
#28634=CARTESIAN_POINT('Ctrl Pts',(43.2716896709821,-3.50159203012731,4.17545672685568));
#28635=CARTESIAN_POINT('Ctrl Pts',(44.2455060811606,-3.42511642941753,6.15442470665314));
#28636=CARTESIAN_POINT('Ctrl Pts',(45.9758066957264,-3.4574068370487,7.5239130403414));
#28637=CARTESIAN_POINT('Ctrl Pts',(47.7061073102923,-3.48969724467988,8.89340137402967));
#28638=CARTESIAN_POINT('Ctrl Pts',(49.8562249858787,-3.58234823313457,9.3821661014496));
#28639=CARTESIAN_POINT('Ctrl Pts',(52.006342661465,-3.67499922158926,9.87093082886954));
#28640=CARTESIAN_POINT('Ctrl Pts',(54.1564603370514,-3.76765021004393,9.38216610144961));
#28641=CARTESIAN_POINT('Ctrl Pts',(39.9362279852004,-4.22575906238287,-1.05434036998093E-14));
#28642=CARTESIAN_POINT('Ctrl Pts',(39.9667240219732,-4.01365446769409,2.70899372698069));
#28643=CARTESIAN_POINT('Ctrl Pts',(41.1606446278505,-3.968825072743,5.14971273833323));
#28644=CARTESIAN_POINT('Ctrl Pts',(42.3545652337277,-3.92399567779192,7.59043174968577));
#28645=CARTESIAN_POINT('Ctrl Pts',(44.4814799043322,-4.01331057777475,9.27946171175751));
#28646=CARTESIAN_POINT('Ctrl Pts',(46.6083945749367,-4.1026254777576,10.9684916738292));
#28647=CARTESIAN_POINT('Ctrl Pts',(49.2530818889508,-4.26638484508716,11.5712994880388));
#28648=CARTESIAN_POINT('Ctrl Pts',(51.897769202965,-4.43014421241671,12.1741073022483));
#28649=CARTESIAN_POINT('Ctrl Pts',(54.5424565169792,-4.59390357974626,11.5712994880388));
#28650=CARTESIAN_POINT('Ctrl Pts',(37.5648924257371,-4.19818497005578,0.));
#28651=CARTESIAN_POINT('Ctrl Pts',(37.59538846251,-3.98608037536701,3.24562220582793));
#28652=CARTESIAN_POINT('Ctrl Pts',(39.0197735211298,-3.97438676625777,6.16982677025168));
#28653=CARTESIAN_POINT('Ctrl Pts',(40.4441585797498,-3.96269315714849,9.09403133467541));
#28654=CARTESIAN_POINT('Ctrl Pts',(42.986355844513,-4.11171668004528,11.1176436806954));
#28655=CARTESIAN_POINT('Ctrl Pts',(45.5285531092761,-4.26074020294207,13.1412560267153));
#28656=CARTESIAN_POINT('Ctrl Pts',(48.691089347985,-4.49895500521137,13.8634749112255));
#28657=CARTESIAN_POINT('Ctrl Pts',(51.8536255866939,-4.73716980748066,14.5856937957357));
#28658=CARTESIAN_POINT('Ctrl Pts',(55.0161618254028,-4.97538460974997,13.8634749112255));
#28659=CARTESIAN_POINT('',(37.5648924257371,-4.19818497005578,0.));
#28660=CARTESIAN_POINT('Ctrl Pts',(37.5648924257371,-4.19818497005578,0.));
#28661=CARTESIAN_POINT('Ctrl Pts',(37.59538846251,-3.98608037536701,3.24562220582793));
#28662=CARTESIAN_POINT('Ctrl Pts',(39.0197735211299,-3.97438676625775,6.16982677025168));
#28663=CARTESIAN_POINT('Ctrl Pts',(40.2089043379837,-3.96462449666083,8.61106394926976));
#28664=CARTESIAN_POINT('Ctrl Pts',(42.2054524109828,-4.06844583510822,10.4489096280657));
#28665=CARTESIAN_POINT('Origin',(37.7741838134886,13.800598242012,0.));
#28666=CARTESIAN_POINT('Ctrl Pts',(37.5648924257371,-4.19818497005578,0.));
#28667=CARTESIAN_POINT('Ctrl Pts',(37.59538846251,-3.98608037536701,3.24562220582793));
#28668=CARTESIAN_POINT('Ctrl Pts',(39.0197735211298,-3.97438676625777,6.16982677025168));
#28669=CARTESIAN_POINT('Ctrl Pts',(40.4441585797498,-3.96269315714849,9.09403133467541));
#28670=CARTESIAN_POINT('Ctrl Pts',(42.986355844513,-4.11171668004528,11.1176436806954));
#28671=CARTESIAN_POINT('Ctrl Pts',(45.5285531092761,-4.26074020294207,13.1412560267153));
#28672=CARTESIAN_POINT('Ctrl Pts',(48.691089347985,-4.49895500521137,13.8634749112255));
#28673=CARTESIAN_POINT('Ctrl Pts',(51.8536255866939,-4.73716980748066,14.5856937957357));
#28674=CARTESIAN_POINT('Ctrl Pts',(55.0161618254028,-4.97538460974997,13.8634749112255));
#28675=CARTESIAN_POINT('Ctrl Pts',(36.8396419064668,-4.81560839388922,6.24500451351651E-15));
#28676=CARTESIAN_POINT('Ctrl Pts',(36.8701379432397,-4.60350379920046,3.38941559469372));
#28677=CARTESIAN_POINT('Ctrl Pts',(38.3562775787769,-4.60068915780673,6.44317352589573));
#28678=CARTESIAN_POINT('Ctrl Pts',(39.8424172143141,-4.59787451641302,9.49693145709773));
#28679=CARTESIAN_POINT('Ctrl Pts',(42.4958923815831,-4.76289738629144,11.6101975146502));
#28680=CARTESIAN_POINT('Ctrl Pts',(45.1493675488522,-4.92792025616987,13.7234635722027));
#28681=CARTESIAN_POINT('Ctrl Pts',(48.4506650623304,-5.18608591779808,14.4776794959001));
#28682=CARTESIAN_POINT('Ctrl Pts',(51.7519625758086,-5.44425157942627,15.2318954195974));
#28683=CARTESIAN_POINT('Ctrl Pts',(55.0532600892868,-5.70241724105448,14.4776794959001));
#28684=CARTESIAN_POINT('Ctrl Pts',(36.7040912252864,-5.7583840898167,0.));
#28685=CARTESIAN_POINT('Ctrl Pts',(36.7345872620593,-5.54627949512793,3.38941559469372));
#28686=CARTESIAN_POINT('Ctrl Pts',(38.2207268975965,-5.54346485373421,6.44317352589573));
#28687=CARTESIAN_POINT('Ctrl Pts',(39.7068665331337,-5.5406502123405,9.49693145709774));
#28688=CARTESIAN_POINT('Ctrl Pts',(42.3603417004027,-5.70567308221891,11.6101975146502));
#28689=CARTESIAN_POINT('Ctrl Pts',(45.0138168676718,-5.87069595209734,13.7234635722027));
#28690=CARTESIAN_POINT('Ctrl Pts',(48.31511438115,-6.12886161372555,14.4776794959001));
#28691=CARTESIAN_POINT('Ctrl Pts',(51.6164118946282,-6.38702727535376,15.2318954195974));
#28692=CARTESIAN_POINT('Ctrl Pts',(54.9177094081065,-6.64519293698195,14.4776794959001));
#28693=CARTESIAN_POINT('Ctrl Pts',(37.2260157227862,-6.55512420987448,0.));
#28694=CARTESIAN_POINT('Ctrl Pts',(37.256511759559,-6.34301961518571,3.24562220582792));
#28695=CARTESIAN_POINT('Ctrl Pts',(38.6808968181789,-6.33132600607645,6.16982677025168));
#28696=CARTESIAN_POINT('Ctrl Pts',(40.1052818767988,-6.31963239696717,9.09403133467541));
#28697=CARTESIAN_POINT('Ctrl Pts',(42.647479141562,-6.46865591986398,11.1176436806954));
#28698=CARTESIAN_POINT('Ctrl Pts',(45.1896764063252,-6.61767944276075,13.1412560267153));
#28699=CARTESIAN_POINT('Ctrl Pts',(48.3522126450341,-6.85589424503005,13.8634749112255));
#28700=CARTESIAN_POINT('Ctrl Pts',(51.5147488837429,-7.09410904729936,14.5856937957357));
#28701=CARTESIAN_POINT('Ctrl Pts',(54.6772851224518,-7.33232384956867,13.8634749112255));
#28702=CARTESIAN_POINT('',(36.9500337175455,-5.31261783613237,1.46702345117554E-29));
#28703=CARTESIAN_POINT('Origin',(38.7317130208009,-5.56877962163409,0.));
#28704=CARTESIAN_POINT('Origin',(38.7317130208009,-5.56877962163409,0.));
#28705=CARTESIAN_POINT('Ctrl Pts',(35.9142171164209,-11.7862169042736,0.));
#28706=CARTESIAN_POINT('Ctrl Pts',(35.9745883786012,-11.5806112670705,3.24562220582793));
#28707=CARTESIAN_POINT('Ctrl Pts',(37.3861394252072,-11.7717478112976,6.16982677025167));
#28708=CARTESIAN_POINT('Ctrl Pts',(38.7976904718132,-11.9628843555247,9.09403133467541));
#28709=CARTESIAN_POINT('Ctrl Pts',(41.2928035754069,-12.4721834264261,11.1176436806954));
#28710=CARTESIAN_POINT('Ctrl Pts',(43.7879166790006,-12.9814824973275,13.1412560267153));
#28711=CARTESIAN_POINT('Ctrl Pts',(46.8843613577409,-13.6673484497324,13.8634749112255));
#28712=CARTESIAN_POINT('Ctrl Pts',(49.9808060364812,-14.3532144021372,14.5856937957357));
#28713=CARTESIAN_POINT('Ctrl Pts',(53.0772507152214,-15.039080354542,13.8634749112255));
#28714=CARTESIAN_POINT('Ctrl Pts',(38.0827145049531,-12.7462230199164,0.));
#28715=CARTESIAN_POINT('Ctrl Pts',(38.1430857671334,-12.5406173827133,2.70899372698069));
#28716=CARTESIAN_POINT('Ctrl Pts',(39.3312338708265,-12.6661569043007,5.14971273833323));
#28717=CARTESIAN_POINT('Ctrl Pts',(40.5193819745196,-12.7916964258881,7.59043174968578));
#28718=CARTESIAN_POINT('Ctrl Pts',(42.6119368849886,-13.1827937463388,9.27946171175752));
#28719=CARTESIAN_POINT('Ctrl Pts',(44.7044917954577,-13.5738910667894,10.9684916738293));
#28720=CARTESIAN_POINT('Ctrl Pts',(47.2989546180621,-14.1123618472584,11.5712994880388));
#28721=CARTESIAN_POINT('Ctrl Pts',(49.8934174406666,-14.6508326277274,12.1741073022483));
#28722=CARTESIAN_POINT('Ctrl Pts',(52.487880263271,-15.1893034081963,11.5712994880388));
#28723=CARTESIAN_POINT('Ctrl Pts',(40.0222531270432,-14.1108411348349,0.));
#28724=CARTESIAN_POINT('Ctrl Pts',(40.0826243892235,-13.9052354976318,2.19648874705824));
#28725=CARTESIAN_POINT('Ctrl Pts',(41.0574123652205,-13.9681268331909,4.17545672685568));
#28726=CARTESIAN_POINT('Ctrl Pts',(42.0322003412175,-14.03101816875,6.15442470665314));
#28727=CARTESIAN_POINT('Ctrl Pts',(43.7402935862748,-14.3092273587166,7.5239130403414));
#28728=CARTESIAN_POINT('Ctrl Pts',(45.4483868313321,-14.5874365486831,8.89340137402968));
#28729=CARTESIAN_POINT('Ctrl Pts',(47.5634337987568,-14.9851381329366,9.38216610144961));
#28730=CARTESIAN_POINT('Ctrl Pts',(49.6784807661816,-15.3828397171901,9.87093082886955));
#28731=CARTESIAN_POINT('Ctrl Pts',(51.7935277336064,-15.7805413014436,9.38216610144961));
#28732=CARTESIAN_POINT('Ctrl Pts',(41.6582954965891,-15.8276282594352,0.));
#28733=CARTESIAN_POINT('Ctrl Pts',(41.7186667587694,-15.6220226222321,1.72780310113343));
#28734=CARTESIAN_POINT('Ctrl Pts',(42.4983369638542,-15.6276222110084,3.28449990511991));
#28735=CARTESIAN_POINT('Ctrl Pts',(43.2780071689391,-15.6332217997846,4.84119670910639));
#28736=CARTESIAN_POINT('Ctrl Pts',(44.6345103396636,-15.8081948292729,5.91846432228298));
#28737=CARTESIAN_POINT('Ctrl Pts',(45.9910135103882,-15.9831678587611,6.99573193545957));
#28738=CARTESIAN_POINT('Ctrl Pts',(47.6676348262506,-16.2521360565322,7.38020429521639));
#28739=CARTESIAN_POINT('Ctrl Pts',(49.344256142113,-16.5211042543032,7.76467665497321));
#28740=CARTESIAN_POINT('Ctrl Pts',(51.0208774579753,-16.7900724520742,7.38020429521639));
#28741=CARTESIAN_POINT('',(35.9142171164435,-11.7862169042834,1.57948957610185E-9));
#28742=CARTESIAN_POINT('Origin',(28.6276304970122,-28.2454287759841,0.));
#28743=CARTESIAN_POINT('Ctrl Pts',(35.9142171165573,-11.7862169041099,3.13105350628993E-9));
#28744=CARTESIAN_POINT('Ctrl Pts',(35.9187750292272,-11.7706940792792,0.245038153335639));
#28745=CARTESIAN_POINT('Ctrl Pts',(35.9294543009581,-11.7568199184781,0.490791160522051));
#28746=CARTESIAN_POINT('Ctrl Pts',(35.9463285033517,-11.7446485667476,0.736766500725875));
#28747=CARTESIAN_POINT('Ctrl Pts',(35.9631473086864,-11.7325171728813,0.981934317701509));
#28748=CARTESIAN_POINT('Ctrl Pts',(35.9861205266374,-11.7220774809613,1.22732257376614));
#28749=CARTESIAN_POINT('Ctrl Pts',(36.0152719968248,-11.713370240977,1.47243294816389));
#28750=CARTESIAN_POINT('Ctrl Pts',(36.0443795639103,-11.7046761143913,1.71717417803068));
#28751=CARTESIAN_POINT('Ctrl Pts',(36.079646826587,-11.6977092667639,1.96163791541639));
#28752=CARTESIAN_POINT('Ctrl Pts',(36.1210475853283,-11.6924966907345,2.2053240877858));
#28753=CARTESIAN_POINT('Ctrl Pts',(36.1624128366599,-11.687288585277,2.4488012624212));
#28754=CARTESIAN_POINT('Ctrl Pts',(36.2099010442177,-11.6838317679615,2.69150175431102));
#28755=CARTESIAN_POINT('Ctrl Pts',(36.2634360706163,-11.6821391062288,2.93292951866858));
#28756=CARTESIAN_POINT('Ctrl Pts',(36.3169598973807,-11.6804467986043,3.17430677585647));
#28757=CARTESIAN_POINT('Ctrl Pts',(36.3765279276399,-11.6805179152423,3.41441139318408));
#28758=CARTESIAN_POINT('Ctrl Pts',(36.442014877408,-11.6823510237344,3.65275710614708));
#28759=CARTESIAN_POINT('Ctrl Pts',(36.5075849814588,-11.6841864598785,3.89140546668862));
#28760=CARTESIAN_POINT('Ctrl Pts',(36.579088906284,-11.6877883562712,4.1282900208124));
#28761=CARTESIAN_POINT('Ctrl Pts',(36.6563532415796,-11.6931409581038,4.36293874377886));
#28762=CARTESIAN_POINT('Ctrl Pts',(36.7336964173084,-11.6984990217247,4.59782690201532));
#28763=CARTESIAN_POINT('Ctrl Pts',(36.8168115609902,-11.7056113365133,4.83047425895048));
#28764=CARTESIAN_POINT('Ctrl Pts',(36.9054796074173,-11.714448049605,5.06042975959526));
#28765=CARTESIAN_POINT('Ctrl Pts',(36.9944068844552,-11.723310597782,5.291057559984));
#28766=CARTESIAN_POINT('Ctrl Pts',(37.0889193314435,-11.7339075987039,5.51897736305783));
#28767=CARTESIAN_POINT('Ctrl Pts',(37.1887539873585,-11.7461953488412,5.74376259354426));
#28768=CARTESIAN_POINT('Ctrl Pts',(37.252411532658,-11.7540303837179,5.88709234072682));
#28769=CARTESIAN_POINT('Ctrl Pts',(37.318232100817,-11.7625525566678,6.02914825314224));
#28770=CARTESIAN_POINT('Ctrl Pts',(37.3861394252393,-11.7717478113124,6.16982677023484));
#28771=CARTESIAN_POINT('Ctrl Pts',(37.4926201075705,-11.7861662410928,6.39041482339093));
#28772=CARTESIAN_POINT('Ctrl Pts',(37.6049078439221,-11.8021412942478,6.60890054011811));
#28773=CARTESIAN_POINT('Ctrl Pts',(37.7228633758095,-11.8196645413942,6.8248041200805));
#28774=CARTESIAN_POINT('Ctrl Pts',(37.8405526164631,-11.8371482288266,7.04022028559291));
#28775=CARTESIAN_POINT('Ctrl Pts',(37.9638839981996,-11.8561731288313,7.25306552029626));
#28776=CARTESIAN_POINT('Ctrl Pts',(38.0926705666681,-11.876718115565,7.46287566269397));
#28777=CARTESIAN_POINT('Ctrl Pts',(38.2212499935677,-11.8972300575423,7.67234834441866));
#28778=CARTESIAN_POINT('Ctrl Pts',(38.3552669199725,-11.9192571854562,7.87879526533018));
#28779=CARTESIAN_POINT('Ctrl Pts',(38.4944885898566,-11.9427658506833,8.08177334612189));
#28780=CARTESIAN_POINT('Ctrl Pts',(38.6335766715385,-11.9662519585001,8.28455666214066));
#28781=CARTESIAN_POINT('Ctrl Pts',(38.7778593027053,-11.9912167312945,8.48387739272773));
#28782=CARTESIAN_POINT('Ctrl Pts',(38.9270604658997,-12.0176143452911,8.67931873610978));
#28783=CARTESIAN_POINT('Ctrl Pts',(39.0762688052756,-12.0440132289432,8.87476947970365));
#28784=CARTESIAN_POINT('Ctrl Pts',(39.2303958882193,-12.071845046704,9.06634009532691));
#28785=CARTESIAN_POINT('Ctrl Pts',(39.3891252359316,-12.1010522527169,9.25364450340837));
#28786=CARTESIAN_POINT('Ctrl Pts',(39.5479128119385,-12.130270173105,9.44101762226336));
#28787=CARTESIAN_POINT('Ctrl Pts',(39.7113057183244,-12.1608644313195,9.62412107874861));
#28788=CARTESIAN_POINT('Ctrl Pts',(39.8789509826175,-12.1927664798388,9.80260437465941));
#28789=CARTESIAN_POINT('Ctrl Pts',(40.0468697110609,-12.2247205672071,9.9813788137949));
#28790=CARTESIAN_POINT('Ctrl Pts',(40.219054331768,-12.2579866432889,10.1555177270905));
#28791=CARTESIAN_POINT('Ctrl Pts',(40.3951188515048,-12.2924858372374,10.3247095747688));
#28792=CARTESIAN_POINT('Ctrl Pts',(40.4460074573685,-12.3024572720619,10.3736117457726));
#28793=CARTESIAN_POINT('Ctrl Pts',(40.4972200117257,-12.3125316625314,10.4221009095717));
#28794=CARTESIAN_POINT('Ctrl Pts',(40.5487467751689,-12.3227069631099,10.4701702229062));
#28795=CARTESIAN_POINT('Ctrl Pts',(43.602250138795,-9.2071267414952,0.));
#28796=CARTESIAN_POINT('Ctrl Pts',(43.6626214009753,-9.00152110429209,1.72780310113343));
#28797=CARTESIAN_POINT('Ctrl Pts',(44.4422916060602,-9.00712069306833,3.28449990511991));
#28798=CARTESIAN_POINT('Ctrl Pts',(45.2219618111451,-9.01272028184456,4.84119670910638));
#28799=CARTESIAN_POINT('Ctrl Pts',(46.5784649818696,-9.18769331133286,5.91846432228298));
#28800=CARTESIAN_POINT('Ctrl Pts',(47.9349681525942,-9.36266634082112,6.99573193545957));
#28801=CARTESIAN_POINT('Ctrl Pts',(49.6115894684565,-9.63163453859214,7.38020429521639));
#28802=CARTESIAN_POINT('Ctrl Pts',(51.2882107843189,-9.90060273636318,7.76467665497322));
#28803=CARTESIAN_POINT('Ctrl Pts',(52.9648321001812,-10.1695709341342,7.38020429521639));
#28804=CARTESIAN_POINT('Ctrl Pts',(41.2977585211119,-9.76686869112097,0.));
#28805=CARTESIAN_POINT('Ctrl Pts',(41.3581297832922,-9.56126305391789,2.19648874705823));
#28806=CARTESIAN_POINT('Ctrl Pts',(42.3329177592892,-9.624154389477,4.17545672685569));
#28807=CARTESIAN_POINT('Ctrl Pts',(43.3077057352862,-9.68704572503613,6.15442470665315));
#28808=CARTESIAN_POINT('Ctrl Pts',(45.0157989803434,-9.96525491500266,7.52391304034141));
#28809=CARTESIAN_POINT('Ctrl Pts',(46.7238922254007,-10.2434641049692,8.89340137402968));
#28810=CARTESIAN_POINT('Ctrl Pts',(48.8389391928255,-10.6411656892227,9.38216610144961));
#28811=CARTESIAN_POINT('Ctrl Pts',(50.9539861602503,-11.0388672734762,9.87093082886955));
#28812=CARTESIAN_POINT('Ctrl Pts',(53.0690331276751,-11.4365688577297,9.38216610144962));
#28813=CARTESIAN_POINT('Ctrl Pts',(38.9283465500518,-9.86626475512805,0.));
#28814=CARTESIAN_POINT('Ctrl Pts',(38.9887178122321,-9.66065911792495,2.70899372698069));
#28815=CARTESIAN_POINT('Ctrl Pts',(40.1768659159253,-9.78619863951237,5.14971273833323));
#28816=CARTESIAN_POINT('Ctrl Pts',(41.3650140196183,-9.91173816109979,7.59043174968577));
#28817=CARTESIAN_POINT('Ctrl Pts',(43.4575689300874,-10.3028354815504,9.27946171175751));
#28818=CARTESIAN_POINT('Ctrl Pts',(45.5501238405564,-10.693932802001,10.9684916738293));
#28819=CARTESIAN_POINT('Ctrl Pts',(48.1445866631608,-11.23240358247,11.5712994880388));
#28820=CARTESIAN_POINT('Ctrl Pts',(50.7390494857653,-11.770874362939,12.1741073022483));
#28821=CARTESIAN_POINT('Ctrl Pts',(53.3335123083697,-12.309345143408,11.5712994880388));
#28822=CARTESIAN_POINT('Ctrl Pts',(36.5850719698904,-9.50149509066561,0.));
#28823=CARTESIAN_POINT('Ctrl Pts',(36.6454432320707,-9.2958894534625,3.24562220582793));
#28824=CARTESIAN_POINT('Ctrl Pts',(38.0569942786767,-9.48702599768955,6.16982677025167));
#28825=CARTESIAN_POINT('Ctrl Pts',(39.4685453252828,-9.6781625419166,9.09403133467541));
#28826=CARTESIAN_POINT('Ctrl Pts',(41.9636584288764,-10.1874616128181,11.1176436806954));
#28827=CARTESIAN_POINT('Ctrl Pts',(44.4587715324701,-10.6967606837195,13.1412560267153));
#28828=CARTESIAN_POINT('Ctrl Pts',(47.5552162112104,-11.3826266361243,13.8634749112255));
#28829=CARTESIAN_POINT('Ctrl Pts',(50.6516608899507,-12.0684925885292,14.5856937957357));
#28830=CARTESIAN_POINT('Ctrl Pts',(53.748105568691,-12.754358540934,13.8634749112255));
#28831=CARTESIAN_POINT('',(36.5850719698904,-9.50149509066561,0.));
#28832=CARTESIAN_POINT('Ctrl Pts',(36.5850719698904,-9.50149509066561,0.));
#28833=CARTESIAN_POINT('Ctrl Pts',(36.6454432320707,-9.2958894534625,3.24562220582793));
#28834=CARTESIAN_POINT('Ctrl Pts',(38.0569942786767,-9.48702599768957,6.16982677025167));
#28835=CARTESIAN_POINT('Ctrl Pts',(39.2354107742189,-9.64659405380744,8.61106394926976));
#28836=CARTESIAN_POINT('Ctrl Pts',(41.196861549629,-10.0334970568411,10.4489096280657));
#28837=CARTESIAN_POINT('Origin',(39.3537269950292,8.28430119040582,0.));
#28838=CARTESIAN_POINT('Ctrl Pts',(36.5850719698904,-9.50149509066561,0.));
#28839=CARTESIAN_POINT('Ctrl Pts',(36.6454432320707,-9.2958894534625,3.24562220582793));
#28840=CARTESIAN_POINT('Ctrl Pts',(38.0569942786767,-9.48702599768957,6.16982677025167));
#28841=CARTESIAN_POINT('Ctrl Pts',(39.4685453252828,-9.67816254191661,9.09403133467541));
#28842=CARTESIAN_POINT('Ctrl Pts',(41.9636584288765,-10.187461612818,11.1176436806954));
#28843=CARTESIAN_POINT('Ctrl Pts',(44.4587715324701,-10.6967606837195,13.1412560267153));
#28844=CARTESIAN_POINT('Ctrl Pts',(47.5552162112104,-11.3826266361243,13.8634749112255));
#28845=CARTESIAN_POINT('Ctrl Pts',(50.6516608899507,-12.0684925885292,14.5856937957357));
#28846=CARTESIAN_POINT('Ctrl Pts',(53.748105568691,-12.754358540934,13.8634749112255));
#28847=CARTESIAN_POINT('Ctrl Pts',(35.7793349404724,-10.0094201239379,0.));
#28848=CARTESIAN_POINT('Ctrl Pts',(35.8397062026527,-9.80381448673481,3.38941559469373));
#28849=CARTESIAN_POINT('Ctrl Pts',(37.3111196447713,-10.0125282162151,6.44317352589573));
#28850=CARTESIAN_POINT('Ctrl Pts',(38.7825330868899,-10.2212419456954,9.49693145709775));
#28851=CARTESIAN_POINT('Ctrl Pts',(41.3855144999132,-10.7622140099939,11.6101975146502));
#28852=CARTESIAN_POINT('Ctrl Pts',(43.9884959129366,-11.3031860742923,13.7234635722027));
#28853=CARTESIAN_POINT('Ctrl Pts',(47.2194501734232,-12.028547603452,14.4776794959001));
#28854=CARTESIAN_POINT('Ctrl Pts',(50.4504044339098,-12.7539091326116,15.2318954195974));
#28855=CARTESIAN_POINT('Ctrl Pts',(53.6813586943964,-13.4792706617712,14.4776794959001));
#28856=CARTESIAN_POINT('Ctrl Pts',(35.5109929990846,-10.9233088493811,0.));
#28857=CARTESIAN_POINT('Ctrl Pts',(35.5713642612649,-10.717703212178,3.38941559469372));
#28858=CARTESIAN_POINT('Ctrl Pts',(37.0427777033835,-10.9264169416583,6.44317352589573));
#28859=CARTESIAN_POINT('Ctrl Pts',(38.514191145502,-11.1351306711386,9.49693145709775));
#28860=CARTESIAN_POINT('Ctrl Pts',(41.1171725585254,-11.6761027354371,11.6101975146502));
#28861=CARTESIAN_POINT('Ctrl Pts',(43.7201539715488,-12.2170747997355,13.7234635722027));
#28862=CARTESIAN_POINT('Ctrl Pts',(46.9511082320354,-12.9424363288952,14.4776794959001));
#28863=CARTESIAN_POINT('Ctrl Pts',(50.182062492522,-13.6677978580548,15.2318954195974));
#28864=CARTESIAN_POINT('Ctrl Pts',(53.4130167530086,-14.3931593872144,14.4776794959001));
#28865=CARTESIAN_POINT('Ctrl Pts',(35.9142171164209,-11.7862169042736,0.));
#28866=CARTESIAN_POINT('Ctrl Pts',(35.9745883786012,-11.5806112670705,3.24562220582793));
#28867=CARTESIAN_POINT('Ctrl Pts',(37.3861394252072,-11.7717478112976,6.16982677025167));
#28868=CARTESIAN_POINT('Ctrl Pts',(38.7976904718132,-11.9628843555247,9.09403133467541));
#28869=CARTESIAN_POINT('Ctrl Pts',(41.2928035754069,-12.4721834264261,11.1176436806954));
#28870=CARTESIAN_POINT('Ctrl Pts',(43.7879166790006,-12.9814824973275,13.1412560267153));
#28871=CARTESIAN_POINT('Ctrl Pts',(46.8843613577409,-13.6673484497324,13.8634749112255));
#28872=CARTESIAN_POINT('Ctrl Pts',(49.9808060364812,-14.3532144021372,14.5856937957357));
#28873=CARTESIAN_POINT('Ctrl Pts',(53.0772507152214,-15.039080354542,13.8634749112255));
#28874=CARTESIAN_POINT('',(35.8178713036688,-10.5170811195104,1.62623179273832E-29));
#28875=CARTESIAN_POINT('Origin',(37.5449600575352,-11.0241949492056,0.));
#28876=CARTESIAN_POINT('Origin',(37.5449600575352,-11.0241949492056,0.));
#28877=CARTESIAN_POINT('Ctrl Pts',(33.871308617615,-16.7773762111447,0.));
#28878=CARTESIAN_POINT('Ctrl Pts',(33.9603261204011,-16.582455069283,3.24562220582793));
#28879=CARTESIAN_POINT('Ctrl Pts',(35.3303080462614,-16.9725307779982,6.16982677025168));
#28880=CARTESIAN_POINT('Ctrl Pts',(36.7002899721218,-17.3626064867134,9.09403133467541));
#28881=CARTESIAN_POINT('Ctrl Pts',(39.0975256070688,-18.2218132452332,11.1176436806954));
#28882=CARTESIAN_POINT('Ctrl Pts',(41.4947612420158,-19.0810200037529,13.1412560267153));
#28883=CARTESIAN_POINT('Ctrl Pts',(44.4620796765374,-20.2005748533764,13.8634749112255));
#28884=CARTESIAN_POINT('Ctrl Pts',(47.4293981110591,-21.3201297029999,14.5856937957357));
#28885=CARTESIAN_POINT('Ctrl Pts',(50.3967165455806,-22.4396845526234,13.8634749112255));
#28886=CARTESIAN_POINT('Ctrl Pts',(35.881110714358,-18.0362202038897,0.));
#28887=CARTESIAN_POINT('Ctrl Pts',(35.9701282171441,-17.841299062028,2.70899372698069));
#28888=CARTESIAN_POINT('Ctrl Pts',(37.1283165495981,-18.1346518775205,5.14971273833323));
#28889=CARTESIAN_POINT('Ctrl Pts',(38.2865048820521,-18.428004693013,7.59043174968578));
#28890=CARTESIAN_POINT('Ctrl Pts',(40.3021016488385,-19.1129228203186,9.27946171175752));
#28891=CARTESIAN_POINT('Ctrl Pts',(42.3176984156249,-19.7978409476242,10.9684916738293));
#28892=CARTESIAN_POINT('Ctrl Pts',(44.8091209655643,-20.7000614289637,11.5712994880388));
#28893=CARTESIAN_POINT('Ctrl Pts',(47.3005435155039,-21.6022819103033,12.1741073022483));
#28894=CARTESIAN_POINT('Ctrl Pts',(49.7919660654433,-22.5045023916429,11.5712994880388));
#28895=CARTESIAN_POINT('Ctrl Pts',(37.6067022235295,-19.6629735993427,0.));
#28896=CARTESIAN_POINT('Ctrl Pts',(37.6957197263156,-19.468052457481,2.19648874705823));
#28897=CARTESIAN_POINT('Ctrl Pts',(38.6516353959963,-19.6690304430807,4.17545672685568));
#28898=CARTESIAN_POINT('Ctrl Pts',(39.607551065677,-19.8700084286804,6.15442470665314));
#28899=CARTESIAN_POINT('Ctrl Pts',(41.2586650884904,-20.3884728641637,7.5239130403414));
#28900=CARTESIAN_POINT('Ctrl Pts',(42.9097791113038,-20.9069372996469,8.89340137402966));
#28901=CARTESIAN_POINT('Ctrl Pts',(44.946699113602,-21.6015934223205,9.38216610144959));
#28902=CARTESIAN_POINT('Ctrl Pts',(46.9836191159003,-22.2962495449941,9.87093082886953));
#28903=CARTESIAN_POINT('Ctrl Pts',(49.0205391181984,-22.9909056676677,9.3821661014496));
#28904=CARTESIAN_POINT('Ctrl Pts',(38.9817677587446,-21.5951194116474,0.));
#28905=CARTESIAN_POINT('Ctrl Pts',(39.0707852615307,-21.4001982697857,1.72780310113343));
#28906=CARTESIAN_POINT('Ctrl Pts',(39.8417226435483,-21.5166995019653,3.28449990511991));
#28907=CARTESIAN_POINT('Ctrl Pts',(40.6126600255659,-21.6332007341449,4.84119670910639));
#28908=CARTESIAN_POINT('Ctrl Pts',(41.9304546915347,-21.9994433198421,5.91846432228298));
#28909=CARTESIAN_POINT('Ctrl Pts',(43.2482493575035,-22.3656859055393,6.99573193545955));
#28910=CARTESIAN_POINT('Ctrl Pts',(44.8695269202923,-22.8705244862897,7.38020429521639));
#28911=CARTESIAN_POINT('Ctrl Pts',(46.4908044830811,-23.37536306704,7.76467665497322));
#28912=CARTESIAN_POINT('Ctrl Pts',(48.1120820458698,-23.8802016477904,7.38020429521639));
#28913=CARTESIAN_POINT('',(33.871308617636,-16.7773762111576,1.57949292205503E-9));
#28914=CARTESIAN_POINT('Origin',(24.3164988679733,-32.0320676419195,0.));
#28915=CARTESIAN_POINT('Ctrl Pts',(33.8713086177734,-16.777376211002,3.13106037980953E-9));
#28916=CARTESIAN_POINT('Ctrl Pts',(33.8780292657696,-16.7626600447505,0.245038153335595));
#28917=CARTESIAN_POINT('Ctrl Pts',(33.8905743368631,-16.7504469217307,0.490791160521955));
#28918=CARTESIAN_POINT('Ctrl Pts',(33.90900894816,-16.7408009061958,0.736766500725727));
#28919=CARTESIAN_POINT('Ctrl Pts',(33.9273830396632,-16.7311865579883,0.981934317701375));
#28920=CARTESIAN_POINT('Ctrl Pts',(33.9516081464472,-16.7241225568764,1.22732257376602));
#28921=CARTESIAN_POINT('Ctrl Pts',(33.9817020661513,-16.7196526308056,1.47243294816379));
#28922=CARTESIAN_POINT('Ctrl Pts',(34.0117506633924,-16.7151894365949,1.71717417803055));
#28923=CARTESIAN_POINT('Ctrl Pts',(34.0476504419797,-16.7133125562152,1.96163791541624));
#28924=CARTESIAN_POINT('Ctrl Pts',(34.0893716276066,-16.7140449789785,2.20532408778562));
#28925=CARTESIAN_POINT('Ctrl Pts',(34.1310570310093,-16.7147767735785,2.44880126242103));
#28926=CARTESIAN_POINT('Ctrl Pts',(34.1785538334837,-16.7181134182575,2.69150175431087));
#28927=CARTESIAN_POINT('Ctrl Pts',(34.2317848413854,-16.7240568140044,2.93292951866844));
#28928=CARTESIAN_POINT('Ctrl Pts',(34.2850047132542,-16.7299989663812,3.17430677585624));
#28929=CARTESIAN_POINT('Ctrl Pts',(34.3439563059025,-16.7385467737469,3.41441139318376));
#28930=CARTESIAN_POINT('Ctrl Pts',(34.4085158144078,-16.749680988503,3.65275710614667));
#28931=CARTESIAN_POINT('Ctrl Pts',(34.4731572995456,-16.7608293413071,3.89140546668821));
#28932=CARTESIAN_POINT('Ctrl Pts',(34.5434208142135,-16.7745706450855,4.12829002081199));
#28933=CARTESIAN_POINT('Ctrl Pts',(34.6191369553176,-16.7908646265311,4.36293874377845));
#28934=CARTESIAN_POINT('Ctrl Pts',(34.6949303570795,-16.8071752343354,4.59782690201486));
#28935=CARTESIAN_POINT('Ctrl Pts',(34.7761873205119,-16.8260436742457,4.83047425894996));
#28936=CARTESIAN_POINT('Ctrl Pts',(34.8626952586805,-16.8474092210269,5.06042975959468));
#28937=CARTESIAN_POINT('Ctrl Pts',(34.9494561121503,-16.8688372322919,5.29105755998348));
#28938=CARTESIAN_POINT('Ctrl Pts',(35.0414984482316,-16.8927768946321,5.51897736305738));
#28939=CARTESIAN_POINT('Ctrl Pts',(35.1385682021255,-16.9191475261011,5.74376259354388));
#28940=CARTESIAN_POINT('Ctrl Pts',(35.2004627636792,-16.9359622248841,5.88709234072657));
#28941=CARTESIAN_POINT('Ctrl Pts',(35.2644005416947,-16.9537648979139,6.02914825314211));
#28942=CARTESIAN_POINT('Ctrl Pts',(35.3303080462911,-16.9725307780174,6.16982677023484));
#28943=CARTESIAN_POINT('Ctrl Pts',(35.4336529523063,-17.0019562300575,6.39041482339096));
#28944=CARTESIAN_POINT('Ctrl Pts',(35.5425242743013,-17.0337488912445,6.60890054011815));
#28945=CARTESIAN_POINT('Ctrl Pts',(35.6567853708682,-17.0678805994453,6.82480412008056));
#28946=CARTESIAN_POINT('Ctrl Pts',(35.7707885165964,-17.1019352533992,7.04022028559298));
#28947=CARTESIAN_POINT('Ctrl Pts',(35.8901570371288,-17.1383183929993,7.25306552029635));
#28948=CARTESIAN_POINT('Ctrl Pts',(36.0147088875608,-17.1769825010549,7.46287566269407));
#28949=CARTESIAN_POINT('Ctrl Pts',(36.1390604075855,-17.2155844213831,7.6723483444187));
#28950=CARTESIAN_POINT('Ctrl Pts',(36.2685784477692,-17.2564599421026,7.87879526533015));
#28951=CARTESIAN_POINT('Ctrl Pts',(36.4030374099052,-17.299542632448,8.0817733461218));
#28952=CARTESIAN_POINT('Ctrl Pts',(36.5373673538287,-17.3425839834018,8.28455666214107));
#28953=CARTESIAN_POINT('Ctrl Pts',(36.6766285382462,-17.3878282101257,8.48387739272861));
#28954=CARTESIAN_POINT('Ctrl Pts',(36.8205542765633,-17.4351906738843,8.67931873611112));
#28955=CARTESIAN_POINT('Ctrl Pts',(36.9644869373274,-17.4825554156522,8.87476947970492));
#28956=CARTESIAN_POINT('Ctrl Pts',(37.1130843481561,-17.532038516521,9.06634009532812));
#28957=CARTESIAN_POINT('Ctrl Pts',(37.2660414411774,-17.5835379767389,9.2536445034095));
#28958=CARTESIAN_POINT('Ctrl Pts',(37.4190546449988,-17.6350563290255,9.4410176222646));
#28959=CARTESIAN_POINT('Ctrl Pts',(37.576430430281,-17.6885924168519,9.62412107874996));
#28960=CARTESIAN_POINT('Ctrl Pts',(37.7378291726326,-17.7440281571915,9.80260437466087));
#28961=CARTESIAN_POINT('Ctrl Pts',(37.8994911897635,-17.7995543247059,9.98137881379659));
#28962=CARTESIAN_POINT('Ctrl Pts',(38.0651889630643,-17.8569862265482,10.1555177270924));
#28963=CARTESIAN_POINT('Ctrl Pts',(38.2345516526472,-17.9161908620981,10.3247095747709));
#28964=CARTESIAN_POINT('Ctrl Pts',(38.2835032027451,-17.9333030058075,10.3736117457756));
#28965=CARTESIAN_POINT('Ctrl Pts',(38.3327607518919,-17.9505631598993,10.4221009095757));
#28966=CARTESIAN_POINT('Ctrl Pts',(38.3823149509235,-17.9679679135961,10.4701702229111));
#28967=CARTESIAN_POINT('Ctrl Pts',(41.8481313484576,-15.3186586437012,0.));
#28968=CARTESIAN_POINT('Ctrl Pts',(41.9371488512437,-15.1237375018396,1.72780310113343));
#28969=CARTESIAN_POINT('Ctrl Pts',(42.7080862332614,-15.2402387340191,3.28449990511991));
#28970=CARTESIAN_POINT('Ctrl Pts',(43.479023615279,-15.3567399661987,4.84119670910638));
#28971=CARTESIAN_POINT('Ctrl Pts',(44.7968182812478,-15.722982551896,5.91846432228297));
#28972=CARTESIAN_POINT('Ctrl Pts',(46.1146129472166,-16.0892251375932,6.99573193545956));
#28973=CARTESIAN_POINT('Ctrl Pts',(47.7358905100054,-16.5940637183435,7.38020429521639));
#28974=CARTESIAN_POINT('Ctrl Pts',(49.3571680727942,-17.0989022990938,7.76467665497322));
#28975=CARTESIAN_POINT('Ctrl Pts',(50.9784456355829,-17.6037408798442,7.38020429521639));
#28976=CARTESIAN_POINT('Ctrl Pts',(39.4874365476042,-15.5447398754884,0.));
#28977=CARTESIAN_POINT('Ctrl Pts',(39.5764540503904,-15.3498187336267,2.19648874705824));
#28978=CARTESIAN_POINT('Ctrl Pts',(40.532369720071,-15.5507967192264,4.17545672685568));
#28979=CARTESIAN_POINT('Ctrl Pts',(41.4882853897517,-15.7517747048261,6.15442470665313));
#28980=CARTESIAN_POINT('Ctrl Pts',(43.1393994125651,-16.2702391403093,7.5239130403414));
#28981=CARTESIAN_POINT('Ctrl Pts',(44.7905134353786,-16.7887035757925,8.89340137402968));
#28982=CARTESIAN_POINT('Ctrl Pts',(46.8274334376768,-17.4833596984661,9.3821661014496));
#28983=CARTESIAN_POINT('Ctrl Pts',(48.864353439975,-18.1780158211397,9.87093082886952));
#28984=CARTESIAN_POINT('Ctrl Pts',(50.9012734422732,-18.8726719438133,9.3821661014496));
#28985=CARTESIAN_POINT('Ctrl Pts',(37.1279962392254,-15.3059217494169,0.));
#28986=CARTESIAN_POINT('Ctrl Pts',(37.2170137420116,-15.1110006075553,2.70899372698069));
#28987=CARTESIAN_POINT('Ctrl Pts',(38.3752020744656,-15.4043534230478,5.14971273833323));
#28988=CARTESIAN_POINT('Ctrl Pts',(39.5333904069196,-15.6977062385402,7.59043174968578));
#28989=CARTESIAN_POINT('Ctrl Pts',(41.548987173706,-16.3826243658458,9.27946171175751));
#28990=CARTESIAN_POINT('Ctrl Pts',(43.5645839404924,-17.0675424931514,10.9684916738293));
#28991=CARTESIAN_POINT('Ctrl Pts',(46.0560064904318,-17.969762974491,11.5712994880388));
#28992=CARTESIAN_POINT('Ctrl Pts',(48.5474290403713,-18.8719834558305,12.1741073022483));
#28993=CARTESIAN_POINT('Ctrl Pts',(51.0388515903108,-19.7742039371701,11.5712994880388));
#28994=CARTESIAN_POINT('Ctrl Pts',(34.8604849513721,-14.6113821712787,0.));
#28995=CARTESIAN_POINT('Ctrl Pts',(34.9495024541582,-14.416461029417,3.24562220582792));
#28996=CARTESIAN_POINT('Ctrl Pts',(36.3194843800186,-14.8065367381322,6.16982677025167));
#28997=CARTESIAN_POINT('Ctrl Pts',(37.6894663058789,-15.1966124468474,9.09403133467541));
#28998=CARTESIAN_POINT('Ctrl Pts',(40.086701940826,-16.0558192053672,11.1176436806954));
#28999=CARTESIAN_POINT('Ctrl Pts',(42.483937575773,-16.9150259638869,13.1412560267153));
#29000=CARTESIAN_POINT('Ctrl Pts',(45.4512560102946,-18.0345808135104,13.8634749112255));
#29001=CARTESIAN_POINT('Ctrl Pts',(48.4185744448162,-19.1541356631339,14.5856937957357));
#29002=CARTESIAN_POINT('Ctrl Pts',(51.3858928793377,-20.2736905127574,13.8634749112255));
#29003=CARTESIAN_POINT('',(34.8604849513721,-14.6113821712787,0.));
#29004=CARTESIAN_POINT('Ctrl Pts',(34.8604849513721,-14.6113821712787,0.));
#29005=CARTESIAN_POINT('Ctrl Pts',(34.9495024541582,-14.416461029417,3.24562220582792));
#29006=CARTESIAN_POINT('Ctrl Pts',(36.3194843800186,-14.8065367381322,6.16982677025167));
#29007=CARTESIAN_POINT('Ctrl Pts',(37.4631973926724,-15.1321867744986,8.61106394926975));
#29008=CARTESIAN_POINT('Ctrl Pts',(39.3496213890631,-15.794295212713,10.4489096280657));
#29009=CARTESIAN_POINT('Origin',(40.1321417817282,2.59935965651478,0.));
#29010=CARTESIAN_POINT('Ctrl Pts',(34.8604849513721,-14.6113821712787,0.));
#29011=CARTESIAN_POINT('Ctrl Pts',(34.9495024541582,-14.416461029417,3.24562220582792));
#29012=CARTESIAN_POINT('Ctrl Pts',(36.3194843800186,-14.8065367381322,6.16982677025167));
#29013=CARTESIAN_POINT('Ctrl Pts',(37.6894663058789,-15.1966124468474,9.09403133467541));
#29014=CARTESIAN_POINT('Ctrl Pts',(40.086701940826,-16.0558192053672,11.1176436806954));
#29015=CARTESIAN_POINT('Ctrl Pts',(42.483937575773,-16.9150259638869,13.1412560267153));
#29016=CARTESIAN_POINT('Ctrl Pts',(45.4512560102946,-18.0345808135104,13.8634749112255));
#29017=CARTESIAN_POINT('Ctrl Pts',(48.4185744448162,-19.1541356631339,14.5856937957357));
#29018=CARTESIAN_POINT('Ctrl Pts',(51.3858928793377,-20.2736905127574,13.8634749112255));
#29019=CARTESIAN_POINT('Ctrl Pts',(33.9906638941716,-14.9994689250473,6.24500451351652E-15));
#29020=CARTESIAN_POINT('Ctrl Pts',(34.0796813969578,-14.8045477831856,3.38941559469372));
#29021=CARTESIAN_POINT('Ctrl Pts',(35.5064149111821,-15.2205410738884,6.44317352589573));
#29022=CARTESIAN_POINT('Ctrl Pts',(36.9331484254065,-15.6365343645912,9.49693145709774));
#29023=CARTESIAN_POINT('Ctrl Pts',(39.4326468889936,-16.5424429921152,11.6101975146502));
#29024=CARTESIAN_POINT('Ctrl Pts',(41.9321453525807,-17.4483516196392,13.7234635722027));
#29025=CARTESIAN_POINT('Ctrl Pts',(45.0269834486349,-18.6261427473665,14.4776794959001));
#29026=CARTESIAN_POINT('Ctrl Pts',(48.121821544689,-19.8039338750937,15.2318954195974));
#29027=CARTESIAN_POINT('Ctrl Pts',(51.2166596407432,-20.981725002821,14.4776794959001));
#29028=CARTESIAN_POINT('Ctrl Pts',(33.5949933606688,-15.8658665409937,6.24500451351652E-15));
#29029=CARTESIAN_POINT('Ctrl Pts',(33.6840108634549,-15.670945399132,3.38941559469373));
#29030=CARTESIAN_POINT('Ctrl Pts',(35.1107443776793,-16.0869386898348,6.44317352589574));
#29031=CARTESIAN_POINT('Ctrl Pts',(36.5374778919037,-16.5029319805376,9.49693145709775));
#29032=CARTESIAN_POINT('Ctrl Pts',(39.0369763554907,-17.4088406080616,11.6101975146502));
#29033=CARTESIAN_POINT('Ctrl Pts',(41.5364748190778,-18.3147492355856,13.7234635722027));
#29034=CARTESIAN_POINT('Ctrl Pts',(44.631312915132,-19.4925403633128,14.4776794959001));
#29035=CARTESIAN_POINT('Ctrl Pts',(47.7261510111862,-20.6703314910401,15.2318954195974));
#29036=CARTESIAN_POINT('Ctrl Pts',(50.8209891072403,-21.8481226187674,14.4776794959001));
#29037=CARTESIAN_POINT('Ctrl Pts',(33.871308617615,-16.7773762111447,0.));
#29038=CARTESIAN_POINT('Ctrl Pts',(33.9603261204011,-16.582455069283,3.24562220582793));
#29039=CARTESIAN_POINT('Ctrl Pts',(35.3303080462614,-16.9725307779982,6.16982677025168));
#29040=CARTESIAN_POINT('Ctrl Pts',(36.7002899721218,-17.3626064867134,9.09403133467541));
#29041=CARTESIAN_POINT('Ctrl Pts',(39.0975256070688,-18.2218132452332,11.1176436806954));
#29042=CARTESIAN_POINT('Ctrl Pts',(41.4947612420158,-19.0810200037529,13.1412560267153));
#29043=CARTESIAN_POINT('Ctrl Pts',(44.4620796765374,-20.2005748533764,13.8634749112255));
#29044=CARTESIAN_POINT('Ctrl Pts',(47.4293981110591,-21.3201297029999,14.5856937957357));
#29045=CARTESIAN_POINT('Ctrl Pts',(50.3967165455806,-22.4396845526234,13.8634749112255));
#29046=CARTESIAN_POINT('',(33.9565603202809,-15.5074469599502,1.75233474473275E-29));
#29047=CARTESIAN_POINT('Origin',(35.5938999782222,-16.2551894587643,0.));
#29048=CARTESIAN_POINT('Origin',(35.5938999782222,-16.2551894587643,0.));
#29049=CARTESIAN_POINT('Ctrl Pts',(39.242105283911,-21.1183468312851,0.));
#29050=CARTESIAN_POINT('Ctrl Pts',(39.3579568876515,-20.938078217107,1.72780310113343));
#29051=CARTESIAN_POINT('Ctrl Pts',(40.1044673847038,-21.1631094635646,3.28449990511991));
#29052=CARTESIAN_POINT('Ctrl Pts',(40.8509778817561,-21.3881407100222,4.84119670910638));
#29053=CARTESIAN_POINT('Ctrl Pts',(42.1032375437761,-21.9381972090399,5.91846432228298));
#29054=CARTESIAN_POINT('Ctrl Pts',(43.355497205796,-22.4882537080577,6.99573193545956));
#29055=CARTESIAN_POINT('Ctrl Pts',(44.8884264797112,-23.2186856141175,7.38020429521639));
#29056=CARTESIAN_POINT('Ctrl Pts',(45.6451607014122,-23.5792650807266,7.56999999999999));
#29057=CARTESIAN_POINT('Ctrl Pts',(46.4213557536264,-23.9491175201773,7.56999999999998));
#29058=CARTESIAN_POINT('Ctrl Pts',(36.873264238351,-21.0061649833188,0.));
#29059=CARTESIAN_POINT('Ctrl Pts',(36.9891158420916,-20.8258963691407,2.19648874705823));
#29060=CARTESIAN_POINT('Ctrl Pts',(37.9066995190543,-21.1608696725668,4.17545672685568));
#29061=CARTESIAN_POINT('Ctrl Pts',(38.8242831960171,-21.495842975993,6.15442470665313));
#29062=CARTESIAN_POINT('Ctrl Pts',(40.3848060765019,-22.2440082162144,7.5239130403414));
#29063=CARTESIAN_POINT('Ctrl Pts',(41.9453289569866,-22.9921734564358,8.89340137402968));
#29064=CARTESIAN_POINT('Ctrl Pts',(43.8626561769037,-23.9696429220947,9.3821661014496));
#29065=CARTESIAN_POINT('Ctrl Pts',(44.8091493688593,-24.4521730739541,9.62344598428096));
#29066=CARTESIAN_POINT('Ctrl Pts',(45.7799833968209,-24.9471123877536,9.62344598428097));
#29067=CARTESIAN_POINT('Ctrl Pts',(34.5718269932681,-20.4339943155211,0.));
#29068=CARTESIAN_POINT('Ctrl Pts',(34.6876785970087,-20.253725701343,2.70899372698069));
#29069=CARTESIAN_POINT('Ctrl Pts',(35.7923297837141,-20.7089199933768,5.14971273833323));
#29070=CARTESIAN_POINT('Ctrl Pts',(36.8969809704195,-21.1641142854106,7.59043174968577));
#29071=CARTESIAN_POINT('Ctrl Pts',(38.7945878558527,-22.12891026164,9.27946171175751));
#29072=CARTESIAN_POINT('Ctrl Pts',(40.6921947412858,-23.0937062378693,10.9684916738293));
#29073=CARTESIAN_POINT('Ctrl Pts',(43.0298588401129,-24.3413098128684,11.5712994880388));
#29074=CARTESIAN_POINT('Ctrl Pts',(44.1838523429614,-24.9571923172889,11.8688770148584));
#29075=CARTESIAN_POINT('Ctrl Pts',(45.36752293894,-25.5889133878675,11.8688770148585));
#29076=CARTESIAN_POINT('Ctrl Pts',(32.426238988581,-19.4238236466313,0.));
#29077=CARTESIAN_POINT('Ctrl Pts',(32.5420905923215,-19.2435550324532,3.24562220582792));
#29078=CARTESIAN_POINT('Ctrl Pts',(33.8426145161273,-19.8246290891125,6.16982677025168));
#29079=CARTESIAN_POINT('Ctrl Pts',(35.143138439933,-20.4057031457718,9.09403133467541));
#29080=CARTESIAN_POINT('Ctrl Pts',(37.3936958017626,-21.5973266200541,11.1176436806954));
#29081=CARTESIAN_POINT('Ctrl Pts',(39.6442531635922,-22.7889500943365,13.1412560267153));
#29082=CARTESIAN_POINT('Ctrl Pts',(42.4220393076079,-24.3194029329699,13.8634749112255));
#29083=CARTESIAN_POINT('Ctrl Pts',(43.7933001162524,-25.0749146564399,14.22));
#29084=CARTESIAN_POINT('Ctrl Pts',(45.1998254516238,-25.8498557716033,14.22));
#29085=CARTESIAN_POINT('',(32.426238988581,-19.4238236466313,0.));
#29086=CARTESIAN_POINT('Ctrl Pts',(32.426238988581,-19.4238236466313,0.));
#29087=CARTESIAN_POINT('Ctrl Pts',(32.5420905923215,-19.2435550324532,3.24562220582792));
#29088=CARTESIAN_POINT('Ctrl Pts',(33.8426145161273,-19.8246290891125,6.16982677025168));
#29089=CARTESIAN_POINT('Ctrl Pts',(34.9283413471525,-20.3097318100848,8.61106394927298));
#29090=CARTESIAN_POINT('Ctrl Pts',(36.7013364119534,-21.2335670650402,10.4489096280657));
#29091=CARTESIAN_POINT('Origin',(40.0935818932912,-3.1384973440487,0.));
#29092=CARTESIAN_POINT('Ctrl Pts',(31.1388779521426,-21.4269965203145,1.04083408558608E-14));
#29093=CARTESIAN_POINT('Ctrl Pts',(31.2547295558831,-21.2467279061364,3.24562220582792));
#29094=CARTESIAN_POINT('Ctrl Pts',(32.5552534796889,-21.8278019627957,6.16982677025168));
#29095=CARTESIAN_POINT('Ctrl Pts',(33.8557774034946,-22.4088760194551,9.09403133467541));
#29096=CARTESIAN_POINT('Ctrl Pts',(36.1063347653242,-23.6004994937374,11.1176436806954));
#29097=CARTESIAN_POINT('Ctrl Pts',(38.3568921271538,-24.7921229680197,13.1412560267153));
#29098=CARTESIAN_POINT('Ctrl Pts',(41.1346782711696,-26.3225758066531,13.8634749112255));
#29099=CARTESIAN_POINT('Ctrl Pts',(42.505939079814,-27.0780875301231,14.22));
#29100=CARTESIAN_POINT('Ctrl Pts',(43.9124644151854,-27.8530286452865,14.22));
#29101=CARTESIAN_POINT('Ctrl Pts',(32.9490709821973,-22.9590519566758,0.));
#29102=CARTESIAN_POINT('Ctrl Pts',(33.0649225859378,-22.7787833424977,2.70899372698069));
#29103=CARTESIAN_POINT('Ctrl Pts',(34.1695737726432,-23.2339776345315,5.14971273833323));
#29104=CARTESIAN_POINT('Ctrl Pts',(35.2742249593487,-23.6891719265653,7.59043174968577));
#29105=CARTESIAN_POINT('Ctrl Pts',(37.1718318447818,-24.6539679027947,9.27946171175751));
#29106=CARTESIAN_POINT('Ctrl Pts',(39.0694387302149,-25.618763879024,10.9684916738293));
#29107=CARTESIAN_POINT('Ctrl Pts',(41.407102829042,-26.8663674540231,11.5712994880388));
#29108=CARTESIAN_POINT('Ctrl Pts',(42.5610963318905,-27.4822499584436,11.8688770148584));
#29109=CARTESIAN_POINT('Ctrl Pts',(43.7447669278692,-28.1139710290222,11.8688770148585));
#29110=CARTESIAN_POINT('Ctrl Pts',(34.4255873115185,-24.8148246247013,0.));
#29111=CARTESIAN_POINT('Ctrl Pts',(34.541438915259,-24.6345560105232,2.19648874705824));
#29112=CARTESIAN_POINT('Ctrl Pts',(35.4590225922217,-24.9695293139493,4.17545672685568));
#29113=CARTESIAN_POINT('Ctrl Pts',(36.3766062691845,-25.3045026173755,6.15442470665314));
#29114=CARTESIAN_POINT('Ctrl Pts',(37.9371291496693,-26.0526678575969,7.5239130403414));
#29115=CARTESIAN_POINT('Ctrl Pts',(39.4976520301541,-26.8008330978183,8.89340137402967));
#29116=CARTESIAN_POINT('Ctrl Pts',(41.4149792500712,-27.7783025634772,9.38216610144961));
#29117=CARTESIAN_POINT('Ctrl Pts',(42.3614724420268,-28.2608327153365,9.62344598428098));
#29118=CARTESIAN_POINT('Ctrl Pts',(43.3323064699883,-28.7557720291361,9.62344598428099));
#29119=CARTESIAN_POINT('Ctrl Pts',(35.5116836434673,-26.9229962078202,0.));
#29120=CARTESIAN_POINT('Ctrl Pts',(35.6275352472078,-26.7427275936421,1.72780310113343));
#29121=CARTESIAN_POINT('Ctrl Pts',(36.3740457442601,-26.9677588400997,3.28449990511991));
#29122=CARTESIAN_POINT('Ctrl Pts',(37.1205562413124,-27.1927900865573,4.84119670910639));
#29123=CARTESIAN_POINT('Ctrl Pts',(38.3728159033324,-27.742846585575,5.91846432228298));
#29124=CARTESIAN_POINT('Ctrl Pts',(39.6250755653524,-28.2929030845928,6.99573193545956));
#29125=CARTESIAN_POINT('Ctrl Pts',(41.1580048392676,-29.0233349906526,7.38020429521641));
#29126=CARTESIAN_POINT('Ctrl Pts',(41.9147390609686,-29.3839144572617,7.57));
#29127=CARTESIAN_POINT('Ctrl Pts',(42.6909341131827,-29.7537668967124,7.57));
#29128=CARTESIAN_POINT('',(31.1388779521917,-21.4269965202912,2.36595504102218E-9));
#29129=CARTESIAN_POINT('Origin',(19.5103534449748,-35.1666259835204,1.04083408558608E-14));
#29130=CARTESIAN_POINT('Ctrl Pts',(31.1388779521426,-21.4269965203145,1.04083408558608E-14));
#29131=CARTESIAN_POINT('Ctrl Pts',(31.2547295558831,-21.2467279061364,3.24562220582792));
#29132=CARTESIAN_POINT('Ctrl Pts',(32.5552534796889,-21.8278019627957,6.16982677025168));
#29133=CARTESIAN_POINT('Ctrl Pts',(33.6474974511925,-22.3158165419709,8.62571762198519));
#29134=CARTESIAN_POINT('Ctrl Pts',(35.4345298797234,-23.2474528526984,10.4701702229062));
#29135=CARTESIAN_POINT('Ctrl Pts',(32.426238988581,-19.4238236466313,0.));
#29136=CARTESIAN_POINT('Ctrl Pts',(32.5420905923215,-19.2435550324532,3.24562220582792));
#29137=CARTESIAN_POINT('Ctrl Pts',(33.8426145161273,-19.8246290891125,6.16982677025168));
#29138=CARTESIAN_POINT('Ctrl Pts',(35.143138439933,-20.4057031457718,9.09403133467541));
#29139=CARTESIAN_POINT('Ctrl Pts',(37.3936958017626,-21.5973266200541,11.1176436806954));
#29140=CARTESIAN_POINT('Ctrl Pts',(39.6442531635922,-22.7889500943365,13.1412560267153));
#29141=CARTESIAN_POINT('Ctrl Pts',(42.4220393076079,-24.3194029329699,13.8634749112255));
#29142=CARTESIAN_POINT('Ctrl Pts',(43.7933001162524,-25.0749146564399,14.22));
#29143=CARTESIAN_POINT('Ctrl Pts',(45.1998254516238,-25.8498557716033,14.22));
#29144=CARTESIAN_POINT('Ctrl Pts',(31.5100409519659,-19.6841717937392,0.));
#29145=CARTESIAN_POINT('Ctrl Pts',(31.6258925557063,-19.5039031795611,3.38941559469373));
#29146=CARTESIAN_POINT('Ctrl Pts',(32.9789019620466,-20.1187076077132,6.44317352589574));
#29147=CARTESIAN_POINT('Ctrl Pts',(34.3319113683869,-20.7335120358653,9.49693145709774));
#29148=CARTESIAN_POINT('Ctrl Pts',(36.6770443017774,-21.9859155393833,11.6101975146502));
#29149=CARTESIAN_POINT('Ctrl Pts',(39.0221772351679,-23.2383190429012,13.7234635722027));
#29150=CARTESIAN_POINT('Ctrl Pts',(41.9178971879301,-24.8445633383047,14.4776794959001));
#29151=CARTESIAN_POINT('Ctrl Pts',(43.3473763048113,-25.6374896966353,14.85));
#29152=CARTESIAN_POINT('Ctrl Pts',(44.8136171406923,-26.4508076337082,14.85));
#29153=CARTESIAN_POINT('Ctrl Pts',(30.9950965373905,-20.4854409432125,0.));
#29154=CARTESIAN_POINT('Ctrl Pts',(31.110948141131,-20.3051723290344,3.38941559469373));
#29155=CARTESIAN_POINT('Ctrl Pts',(32.4639575474713,-20.9199767571865,6.44317352589574));
#29156=CARTESIAN_POINT('Ctrl Pts',(33.8169669538116,-21.5347811853386,9.49693145709775));
#29157=CARTESIAN_POINT('Ctrl Pts',(36.1620998872021,-22.7871846888565,11.6101975146502));
#29158=CARTESIAN_POINT('Ctrl Pts',(38.5072328205925,-24.0395881923744,13.7234635722027));
#29159=CARTESIAN_POINT('Ctrl Pts',(41.4029527733547,-25.645832487778,14.4776794959001));
#29160=CARTESIAN_POINT('Ctrl Pts',(42.8324318902359,-26.4387588461085,14.85));
#29161=CARTESIAN_POINT('Ctrl Pts',(44.2986727261169,-27.2520767831815,14.85));
#29162=CARTESIAN_POINT('Ctrl Pts',(31.1388779521426,-21.4269965203145,1.04083408558608E-14));
#29163=CARTESIAN_POINT('Ctrl Pts',(31.2547295558831,-21.2467279061364,3.24562220582792));
#29164=CARTESIAN_POINT('Ctrl Pts',(32.5552534796889,-21.8278019627957,6.16982677025168));
#29165=CARTESIAN_POINT('Ctrl Pts',(33.8557774034946,-22.4088760194551,9.09403133467541));
#29166=CARTESIAN_POINT('Ctrl Pts',(36.1063347653242,-23.6004994937374,11.1176436806954));
#29167=CARTESIAN_POINT('Ctrl Pts',(38.3568921271537,-24.7921229680197,13.1412560267153));
#29168=CARTESIAN_POINT('Ctrl Pts',(41.1346782711696,-26.3225758066531,13.8634749112255));
#29169=CARTESIAN_POINT('Ctrl Pts',(42.505939079814,-27.0780875301231,14.22));
#29170=CARTESIAN_POINT('Ctrl Pts',(43.9124644151854,-27.8530286452865,14.22));
#29171=CARTESIAN_POINT('',(31.4039916914005,-20.1821259000877,1.90249220280833E-29));
#29172=CARTESIAN_POINT('Origin',(32.9182507396839,-21.1552751870379,0.));
#29173=CARTESIAN_POINT('Origin',(32.9182507396839,-21.1552751870379,0.));
#29174=CARTESIAN_POINT('Ctrl Pts',(27.7725495286734,-25.6404249706862,0.));
#29175=CARTESIAN_POINT('Ctrl Pts',(27.9128768288045,-25.4784786333246,3.24562220582792));
#29176=CARTESIAN_POINT('Ctrl Pts',(29.1174678338683,-26.2387220458137,6.16982677025168));
#29177=CARTESIAN_POINT('Ctrl Pts',(30.3220588389321,-26.9989654583028,9.09403133467541));
#29178=CARTESIAN_POINT('Ctrl Pts',(32.3801230698288,-28.4987476307696,11.1176436806954));
#29179=CARTESIAN_POINT('Ctrl Pts',(34.4381873007256,-29.9985298032364,13.1412560267153));
#29180=CARTESIAN_POINT('Ctrl Pts',(36.9698934388172,-31.9087250245467,13.8634749112255));
#29181=CARTESIAN_POINT('Ctrl Pts',(39.5015995769088,-33.8189202458569,14.5856937957357));
#29182=CARTESIAN_POINT('Ctrl Pts',(42.0333057150004,-35.7291154671672,13.8634749112255));
#29183=CARTESIAN_POINT('Ctrl Pts',(29.3462831821134,-27.4145036200625,0.));
#29184=CARTESIAN_POINT('Ctrl Pts',(29.4866104822446,-27.2525572827009,2.70899372698069));
#29185=CARTESIAN_POINT('Ctrl Pts',(30.5152370105911,-27.8603266081622,5.14971273833323));
#29186=CARTESIAN_POINT('Ctrl Pts',(31.5438635389376,-28.4680959336234,7.59043174968578));
#29187=CARTESIAN_POINT('Ctrl Pts',(33.2848507390765,-29.6931292949424,9.27946171175751));
#29188=CARTESIAN_POINT('Ctrl Pts',(35.0258379392153,-30.9181626562613,10.9684916738293));
#29189=CARTESIAN_POINT('Ctrl Pts',(37.1621554871444,-32.4857517139246,11.5712994880388));
#29190=CARTESIAN_POINT('Ctrl Pts',(39.2984730350736,-34.0533407715878,12.1741073022483));
#29191=CARTESIAN_POINT('Ctrl Pts',(41.4347905830027,-35.6209298292511,11.5712994880388));
#29192=CARTESIAN_POINT('Ctrl Pts',(30.5436667170408,-29.461517380746,0.));
#29193=CARTESIAN_POINT('Ctrl Pts',(30.683994017172,-29.2995710433843,2.19648874705823));
#29194=CARTESIAN_POINT('Ctrl Pts',(31.5445663438467,-29.7617205741624,4.17545672685568));
#29195=CARTESIAN_POINT('Ctrl Pts',(32.4051386705215,-30.2238701049404,6.15442470665314));
#29196=CARTESIAN_POINT('Ctrl Pts',(33.8433026630073,-31.1865056631395,7.5239130403414));
#29197=CARTESIAN_POINT('Ctrl Pts',(35.2814666554931,-32.1491412213386,8.89340137402967));
#29198=CARTESIAN_POINT('Ctrl Pts',(37.0401698399467,-33.3895255704512,9.3821661014496));
#29199=CARTESIAN_POINT('Ctrl Pts',(38.7988730244003,-34.6299099195637,9.87093082886953));
#29200=CARTESIAN_POINT('Ctrl Pts',(40.5575762088539,-35.8702942686763,9.3821661014496));
#29201=CARTESIAN_POINT('Ctrl Pts',(31.3186840564481,-31.7027984407116,0.));
#29202=CARTESIAN_POINT('Ctrl Pts',(31.4590113565792,-31.54085210335,1.72780310113342));
#29203=CARTESIAN_POINT('Ctrl Pts',(32.1658981677048,-31.8698323768442,3.28449990511991));
#29204=CARTESIAN_POINT('Ctrl Pts',(32.8727849788303,-32.1988126503384,4.84119670910639));
#29205=CARTESIAN_POINT('Ctrl Pts',(34.0340172414013,-32.9214854985887,5.91846432228298));
#29206=CARTESIAN_POINT('Ctrl Pts',(35.1952495039724,-33.644158346839,6.99573193545957));
#29207=CARTESIAN_POINT('Ctrl Pts',(36.6086244696001,-34.5853140909926,7.38020429521639));
#29208=CARTESIAN_POINT('Ctrl Pts',(38.0219994352277,-35.5264698351462,7.76467665497322));
#29209=CARTESIAN_POINT('Ctrl Pts',(39.4353744008554,-36.4676255792997,7.38020429521639));
#29210=CARTESIAN_POINT('',(27.7725495286886,-25.6404249706929,1.57949994983948E-9));
#29211=CARTESIAN_POINT('Origin',(14.3070334890497,-37.5852932322719,0.));
#29212=CARTESIAN_POINT('Ctrl Pts',(27.7725495288655,-25.640424970594,3.13107432308264E-9));
#29213=CARTESIAN_POINT('Ctrl Pts',(27.783143966541,-25.6281983378207,0.245038153335697));
#29214=CARTESIAN_POINT('Ctrl Pts',(27.7986217084841,-25.6200142870522,0.490791160522144));
#29215=CARTESIAN_POINT('Ctrl Pts',(27.8190271851147,-25.6159526330982,0.736766500726005));
#29216=CARTESIAN_POINT('Ctrl Pts',(27.8393656717115,-25.611904313326,0.981934317701654));
#29217=CARTESIAN_POINT('Ctrl Pts',(27.8645996505507,-25.6119514551676,1.2273225737663));
#29218=CARTESIAN_POINT('Ctrl Pts',(27.8947338787561,-25.6161410294537,1.47243294816407));
#29219=CARTESIAN_POINT('Ctrl Pts',(27.9248227237926,-25.6203242940989,1.71717417803081));
#29220=CARTESIAN_POINT('Ctrl Pts',(27.9597970874096,-25.6286375769737,1.96163791541648));
#29221=CARTESIAN_POINT('Ctrl Pts',(27.9996219245317,-25.6410945477699,2.20532408778584));
#29222=CARTESIAN_POINT('Ctrl Pts',(28.0394126058351,-25.6535408348303,2.44880126242126));
#29223=CARTESIAN_POINT('Ctrl Pts',(28.0840454126418,-25.6701237175581,2.6915017543111));
#29224=CARTESIAN_POINT('Ctrl Pts',(28.1334457426218,-25.6908232719762,2.93292951866868));
#29225=CARTESIAN_POINT('Ctrl Pts',(28.1828357379543,-25.7115184960062,3.17430677585651));
#29226=CARTESIAN_POINT('Ctrl Pts',(28.2369911812592,-25.7363286400401,3.41441139318407));
#29227=CARTESIAN_POINT('Ctrl Pts',(28.2957987052584,-25.7652003562649,3.65275710614702));
#29228=CARTESIAN_POINT('Ctrl Pts',(28.3546809021121,-25.7941087333337,3.8914054666885));
#29229=CARTESIAN_POINT('Ctrl Pts',(28.4182268780896,-25.8270889373975,4.12829002081223));
#29230=CARTESIAN_POINT('Ctrl Pts',(28.4862854384144,-25.8640546001341,4.36293874377863));
#29231=CARTESIAN_POINT('Ctrl Pts',(28.5544134456109,-25.9010579825879,4.59782690201503));
#29232=CARTESIAN_POINT('Ctrl Pts',(28.627063077262,-25.9420548501738,4.83047425895014));
#29233=CARTESIAN_POINT('Ctrl Pts',(28.7040474659737,-25.9869270447951,5.06042975959485));
#29234=CARTESIAN_POINT('Ctrl Pts',(28.781256926861,-26.0319304281242,5.29105755998367));
#29235=CARTESIAN_POINT('Ctrl Pts',(28.8628263193251,-26.0808316886121,5.51897736305757));
#29236=CARTESIAN_POINT('Ctrl Pts',(28.9485346007075,-26.1334818341729,5.74376259354408));
#29237=CARTESIAN_POINT('Ctrl Pts',(29.0031847495425,-26.1670531325897,5.8870923407267));
#29238=CARTESIAN_POINT('Ctrl Pts',(29.0595170057056,-26.2021480259525,6.02914825314218));
#29239=CARTESIAN_POINT('Ctrl Pts',(29.1174678338914,-26.2387220458404,6.16982677023484));
#29240=CARTESIAN_POINT('Ctrl Pts',(29.2083364372323,-26.2960711849266,6.39041482339096));
#29241=CARTESIAN_POINT('Ctrl Pts',(29.3038406779896,-26.3572486158603,6.60890054011817));
#29242=CARTESIAN_POINT('Ctrl Pts',(29.4038573838823,-26.4221888209398,6.82480412008059));
#29243=CARTESIAN_POINT('Ctrl Pts',(29.5036482964477,-26.4869824198614,7.04022028559291));
#29244=CARTESIAN_POINT('Ctrl Pts',(29.6079312382237,-26.5555217851617,7.25306552029617));
#29245=CARTESIAN_POINT('Ctrl Pts',(29.7165449255433,-26.6277100364536,7.4628756626938));
#29246=CARTESIAN_POINT('Ctrl Pts',(29.8249839175523,-26.6997821794602,7.67234834441843));
#29247=CARTESIAN_POINT('Ctrl Pts',(29.9377396021004,-26.7754914030014,7.87879526532988));
#29248=CARTESIAN_POINT('Ctrl Pts',(30.0546142350027,-26.8547104088651,8.08177334612154));
#29249=CARTESIAN_POINT('Ctrl Pts',(30.1713767224891,-26.933853401242,8.28455666214074));
#29250=CARTESIAN_POINT('Ctrl Pts',(30.2922500787577,-27.0164993284348,8.48387739272822));
#29251=CARTESIAN_POINT('Ctrl Pts',(30.4170022653821,-27.1024918458757,8.67931873611067));
#29252=CARTESIAN_POINT('Ctrl Pts',(30.5417604522566,-27.1884884993291,8.87476947970451));
#29253=CARTESIAN_POINT('Ctrl Pts',(30.6703976233158,-27.2778319154182,9.06634009532774));
#29254=CARTESIAN_POINT('Ctrl Pts',(30.8026498047311,-27.3703382785461,9.25364450340917));
#29255=CARTESIAN_POINT('Ctrl Pts',(30.9349505015539,-27.4628785767203,9.44101762226418));
#29256=CARTESIAN_POINT('Ctrl Pts',(31.0708686028425,-27.558583959197,9.62412107874945));
#29257=CARTESIAN_POINT('Ctrl Pts',(31.2101115092128,-27.6572454428936,9.80260437466027));
#29258=CARTESIAN_POINT('Ctrl Pts',(31.3495815496048,-27.7560678639059,9.98137881379597));
#29259=CARTESIAN_POINT('Ctrl Pts',(31.4923869622801,-27.8578558275198,10.1555177270918));
#29260=CARTESIAN_POINT('Ctrl Pts',(31.638209399577,-27.962377242905,10.3247095747703));
#29261=CARTESIAN_POINT('Ctrl Pts',(31.6803570199419,-27.9925874699272,10.3736117457735));
#29262=CARTESIAN_POINT('Ctrl Pts',(31.7227565449007,-28.0230259217658,10.4221009095722));
#29263=CARTESIAN_POINT('Ctrl Pts',(31.7653999649232,-28.0536866918398,10.4701702229062));
#29264=CARTESIAN_POINT('Ctrl Pts',(35.8372231206706,-26.4881263776673,0.));
#29265=CARTESIAN_POINT('Ctrl Pts',(35.9775504208018,-26.3261800403057,1.72780310113343));
#29266=CARTESIAN_POINT('Ctrl Pts',(36.6844372319273,-26.6551603137999,3.28449990511991));
#29267=CARTESIAN_POINT('Ctrl Pts',(37.3913240430528,-26.9841405872941,4.84119670910638));
#29268=CARTESIAN_POINT('Ctrl Pts',(38.5525563056238,-27.7068134355444,5.91846432228298));
#29269=CARTESIAN_POINT('Ctrl Pts',(39.7137885681949,-28.4294862837947,6.99573193545956));
#29270=CARTESIAN_POINT('Ctrl Pts',(41.1271635338226,-29.3706420279483,7.38020429521639));
#29271=CARTESIAN_POINT('Ctrl Pts',(42.5405384994503,-30.3117977721018,7.76467665497322));
#29272=CARTESIAN_POINT('Ctrl Pts',(43.953913465078,-31.2529535162554,7.38020429521639));
#29273=CARTESIAN_POINT('Ctrl Pts',(33.5084586029183,-26.0399651488665,0.));
#29274=CARTESIAN_POINT('Ctrl Pts',(33.6487859030494,-25.8780188115048,2.19648874705823));
#29275=CARTESIAN_POINT('Ctrl Pts',(34.5093582297241,-26.3401683422829,4.17545672685568));
#29276=CARTESIAN_POINT('Ctrl Pts',(35.3699305563989,-26.8023178730609,6.15442470665314));
#29277=CARTESIAN_POINT('Ctrl Pts',(36.8080945488847,-27.76495343126,7.5239130403414));
#29278=CARTESIAN_POINT('Ctrl Pts',(38.2462585413705,-28.7275889894591,8.89340137402967));
#29279=CARTESIAN_POINT('Ctrl Pts',(40.0049617258241,-29.9679733385717,9.3821661014496));
#29280=CARTESIAN_POINT('Ctrl Pts',(41.7636649102777,-31.2083576876842,9.87093082886953));
#29281=CARTESIAN_POINT('Ctrl Pts',(43.5223680947313,-32.4487420367968,9.3821661014496));
#29282=CARTESIAN_POINT('Ctrl Pts',(31.3118750466442,-25.1460896841349,0.));
#29283=CARTESIAN_POINT('Ctrl Pts',(31.4522023467754,-24.9841433467732,2.70899372698069));
#29284=CARTESIAN_POINT('Ctrl Pts',(32.4808288751219,-25.5919126722345,5.14971273833323));
#29285=CARTESIAN_POINT('Ctrl Pts',(33.5094554034684,-26.1996819976958,7.59043174968578));
#29286=CARTESIAN_POINT('Ctrl Pts',(35.2504426036073,-27.4247153590147,9.27946171175752));
#29287=CARTESIAN_POINT('Ctrl Pts',(36.9914298037461,-28.6497487203337,10.9684916738293));
#29288=CARTESIAN_POINT('Ctrl Pts',(39.1277473516752,-30.2173377779969,11.5712994880388));
#29289=CARTESIAN_POINT('Ctrl Pts',(41.2640648996044,-31.7849268356602,12.1741073022483));
#29290=CARTESIAN_POINT('Ctrl Pts',(43.4003824475335,-33.3525158933234,11.5712994880388));
#29291=CARTESIAN_POINT('Ctrl Pts',(29.3318883095338,-23.8408520862203,0.));
#29292=CARTESIAN_POINT('Ctrl Pts',(29.4722156096649,-23.6789057488587,3.24562220582793));
#29293=CARTESIAN_POINT('Ctrl Pts',(30.6768066147287,-24.4391491613478,6.16982677025167));
#29294=CARTESIAN_POINT('Ctrl Pts',(31.8813976197925,-25.1993925738369,9.09403133467541));
#29295=CARTESIAN_POINT('Ctrl Pts',(33.9394618506893,-26.6991747463037,11.1176436806954));
#29296=CARTESIAN_POINT('Ctrl Pts',(35.997526081586,-28.1989569187706,13.1412560267153));
#29297=CARTESIAN_POINT('Ctrl Pts',(38.5292322196776,-30.1091521400808,13.8634749112255));
#29298=CARTESIAN_POINT('Ctrl Pts',(41.0609383577692,-32.0193473613911,14.5856937957357));
#29299=CARTESIAN_POINT('Ctrl Pts',(43.5926444958608,-33.9295425827013,13.8634749112255));
#29300=CARTESIAN_POINT('',(29.3318883095338,-23.8408520862203,0.));
#29301=CARTESIAN_POINT('Ctrl Pts',(29.3318883095338,-23.8408520862203,0.));
#29302=CARTESIAN_POINT('Ctrl Pts',(29.472215609665,-23.6789057488587,3.24562220582793));
#29303=CARTESIAN_POINT('Ctrl Pts',(30.6768066147287,-24.4391491613478,6.16982677025167));
#29304=CARTESIAN_POINT('Ctrl Pts',(31.6824449968205,-25.0738292744465,8.61106394926976));
#29305=CARTESIAN_POINT('Ctrl Pts',(33.3059180634108,-26.2405847244742,10.4489096280657));
#29306=CARTESIAN_POINT('Origin',(39.2388322978494,-8.81246358936616,0.));
#29307=CARTESIAN_POINT('Ctrl Pts',(29.3318883095338,-23.8408520862204,0.));
#29308=CARTESIAN_POINT('Ctrl Pts',(29.472215609665,-23.6789057488587,3.24562220582793));
#29309=CARTESIAN_POINT('Ctrl Pts',(30.6768066147287,-24.4391491613478,6.16982677025167));
#29310=CARTESIAN_POINT('Ctrl Pts',(31.8813976197925,-25.1993925738369,9.09403133467541));
#29311=CARTESIAN_POINT('Ctrl Pts',(33.9394618506893,-26.6991747463037,11.1176436806954));
#29312=CARTESIAN_POINT('Ctrl Pts',(35.997526081586,-28.1989569187706,13.1412560267153));
#29313=CARTESIAN_POINT('Ctrl Pts',(38.5292322196776,-30.1091521400808,13.8634749112255));
#29314=CARTESIAN_POINT('Ctrl Pts',(41.0609383577692,-32.0193473613911,14.5856937957357));
#29315=CARTESIAN_POINT('Ctrl Pts',(43.5926444958608,-33.9295425827013,13.8634749112255));
#29316=CARTESIAN_POINT('Ctrl Pts',(28.3879644434325,-23.9681616891746,0.));
#29317=CARTESIAN_POINT('Ctrl Pts',(28.5282917435636,-23.8062153518129,3.38941559469372));
#29318=CARTESIAN_POINT('Ctrl Pts',(29.7800336722637,-24.6073152722068,6.44317352589573));
#29319=CARTESIAN_POINT('Ctrl Pts',(31.0317756009638,-25.4084151926007,9.49693145709773));
#29320=CARTESIAN_POINT('Ctrl Pts',(33.1748028604387,-26.9818182484143,11.6101975146502));
#29321=CARTESIAN_POINT('Ctrl Pts',(35.3178301199137,-28.555221304228,13.7234635722027));
#29322=CARTESIAN_POINT('Ctrl Pts',(37.9554834217124,-30.5572202654794,14.4776794959001));
#29323=CARTESIAN_POINT('Ctrl Pts',(40.5931367235111,-32.5592192267308,15.2318954195974));
#29324=CARTESIAN_POINT('Ctrl Pts',(43.2307900253098,-34.5612181879822,14.4776794959001));
#29325=CARTESIAN_POINT('Ctrl Pts',(27.7642289310883,-24.6879908429609,0.));
#29326=CARTESIAN_POINT('Ctrl Pts',(27.9045562312195,-24.5260445055993,3.38941559469372));
#29327=CARTESIAN_POINT('Ctrl Pts',(29.1562981599195,-25.3271444259932,6.44317352589573));
#29328=CARTESIAN_POINT('Ctrl Pts',(30.4080400886196,-26.128244346387,9.49693145709774));
#29329=CARTESIAN_POINT('Ctrl Pts',(32.5510673480945,-27.7016474022007,11.6101975146502));
#29330=CARTESIAN_POINT('Ctrl Pts',(34.6940946075695,-29.2750504580143,13.7234635722027));
#29331=CARTESIAN_POINT('Ctrl Pts',(37.3317479093682,-31.2770494192658,14.4776794959001));
#29332=CARTESIAN_POINT('Ctrl Pts',(39.9694012111669,-33.2790483805172,15.2318954195974));
#29333=CARTESIAN_POINT('Ctrl Pts',(42.6070545129656,-35.2810473417686,14.4776794959001));
#29334=CARTESIAN_POINT('Ctrl Pts',(27.7725495286734,-25.6404249706862,0.));
#29335=CARTESIAN_POINT('Ctrl Pts',(27.9128768288045,-25.4784786333246,3.24562220582792));
#29336=CARTESIAN_POINT('Ctrl Pts',(29.1174678338683,-26.2387220458137,6.16982677025167));
#29337=CARTESIAN_POINT('Ctrl Pts',(30.3220588389321,-26.9989654583028,9.09403133467541));
#29338=CARTESIAN_POINT('Ctrl Pts',(32.3801230698288,-28.4987476307696,11.1176436806954));
#29339=CARTESIAN_POINT('Ctrl Pts',(34.4381873007256,-29.9985298032364,13.1412560267153));
#29340=CARTESIAN_POINT('Ctrl Pts',(36.9698934388172,-31.9087250245467,13.8634749112255));
#29341=CARTESIAN_POINT('Ctrl Pts',(39.5015995769088,-33.8189202458569,14.5856937957357));
#29342=CARTESIAN_POINT('Ctrl Pts',(42.0333057150004,-35.7291154671672,13.8634749112255));
#29343=CARTESIAN_POINT('',(28.2121283533189,-24.4459549573422,1.89568229885369E-29));
#29344=CARTESIAN_POINT('Origin',(29.5724808444819,-25.6247005192794,0.));
#29345=CARTESIAN_POINT('Origin',(29.5724808444819,-25.6247005192794,0.));
#29346=CARTESIAN_POINT('Ctrl Pts',(23.8408520862196,-29.3318883095344,0.));
#29347=CARTESIAN_POINT('Ctrl Pts',(24.0027984235812,-29.1915610094033,3.24562220582793));
#29348=CARTESIAN_POINT('Ctrl Pts',(25.0869345107936,-30.1154974142048,6.16982677025167));
#29349=CARTESIAN_POINT('Ctrl Pts',(26.1710705980059,-31.0394338190064,9.09403133467541));
#29350=CARTESIAN_POINT('Ctrl Pts',(27.9947454451959,-32.8168434496409,11.1176436806954));
#29351=CARTESIAN_POINT('Ctrl Pts',(29.8184202923859,-34.5942530802755,13.1412560267153));
#29352=CARTESIAN_POINT('Ctrl Pts',(32.0525081884194,-36.8453046181048,13.8634749112255));
#29353=CARTESIAN_POINT('Ctrl Pts',(34.2865960844529,-39.0963561559342,14.5856937957357));
#29354=CARTESIAN_POINT('Ctrl Pts',(36.5206839804863,-41.3474076937636,13.8634749112255));
#29355=CARTESIAN_POINT('Ctrl Pts',(25.1460896841341,-31.3118750466448,0.));
#29356=CARTESIAN_POINT('Ctrl Pts',(25.3080360214957,-31.1715477465137,2.70899372698069));
#29357=CARTESIAN_POINT('Ctrl Pts',(26.2396980216802,-31.919519674598,5.14971273833323));
#29358=CARTESIAN_POINT('Ctrl Pts',(27.1713600218647,-32.6674916026823,7.59043174968577));
#29359=CARTESIAN_POINT('Ctrl Pts',(28.7202860579068,-34.1278242025589,9.27946171175751));
#29360=CARTESIAN_POINT('Ctrl Pts',(30.269212093949,-35.5881568024355,10.9684916738293));
#29361=CARTESIAN_POINT('Ctrl Pts',(32.1606938263354,-37.4438197501024,11.5712994880388));
#29362=CARTESIAN_POINT('Ctrl Pts',(34.0521755587219,-39.2994826977694,12.1741073022483));
#29363=CARTESIAN_POINT('Ctrl Pts',(35.9436572911084,-41.1551456454363,11.5712994880388));
#29364=CARTESIAN_POINT('Ctrl Pts',(26.0399651488656,-33.5084586029189,0.));
#29365=CARTESIAN_POINT('Ctrl Pts',(26.2019114862272,-33.3681313027878,2.19648874705823));
#29366=CARTESIAN_POINT('Ctrl Pts',(26.9879536917285,-33.9480490292003,4.17545672685567));
#29367=CARTESIAN_POINT('Ctrl Pts',(27.7739958972298,-34.5279667556128,6.15442470665314));
#29368=CARTESIAN_POINT('Ctrl Pts',(29.0605241301521,-35.6854761478364,7.5239130403414));
#29369=CARTESIAN_POINT('Ctrl Pts',(30.3470523630745,-36.84298554006,8.89340137402967));
#29370=CARTESIAN_POINT('Ctrl Pts',(31.9113293869102,-38.3210341242513,9.3821661014496));
#29371=CARTESIAN_POINT('Ctrl Pts',(33.475606410746,-39.7990827084427,9.87093082886954));
#29372=CARTESIAN_POINT('Ctrl Pts',(35.0398834345817,-41.277131292634,9.3821661014496));
#29373=CARTESIAN_POINT('Ctrl Pts',(26.4881263776664,-35.8372231206713,0.));
#29374=CARTESIAN_POINT('Ctrl Pts',(26.650072715028,-35.6968958205402,1.72780310113342));
#29375=CARTESIAN_POINT('Ctrl Pts',(27.3029456632455,-36.1231280314035,3.28449990511991));
#29376=CARTESIAN_POINT('Ctrl Pts',(27.955818611463,-36.5493602422667,4.84119670910638));
#29377=CARTESIAN_POINT('Ctrl Pts',(29.0023841344365,-37.4299379045755,5.91846432228297));
#29378=CARTESIAN_POINT('Ctrl Pts',(30.0489496574099,-38.3105155668843,6.99573193545956));
#29379=CARTESIAN_POINT('Ctrl Pts',(31.3139980762868,-39.4432359322498,7.38020429521639));
#29380=CARTESIAN_POINT('Ctrl Pts',(32.5790464951636,-40.5759562976152,7.76467665497321));
#29381=CARTESIAN_POINT('Ctrl Pts',(33.8440949140404,-41.7086766629806,7.38020429521638));
#29382=CARTESIAN_POINT('',(23.8408520862337,-29.3318883095433,1.57949914646235E-9));
#29383=CARTESIAN_POINT('Origin',(8.81246358936518,-39.2388322978496,0.));
#29384=CARTESIAN_POINT('Ctrl Pts',(23.8408520864229,-29.3318883094705,3.13107447079983E-9));
#29385=CARTESIAN_POINT('Ctrl Pts',(23.8530787192645,-29.3212938718739,0.245038153335542));
#29386=CARTESIAN_POINT('Ctrl Pts',(23.8695636319732,-29.3153958352833,0.490791160521833));
#29387=CARTESIAN_POINT('Ctrl Pts',(23.8903394438996,-29.3142795252166,0.736766500725538));
#29388=CARTESIAN_POINT('Ctrl Pts',(23.9110470500022,-29.3131668799333,0.98193431770121));
#29389=CARTESIAN_POINT('Ctrl Pts',(23.9360174743375,-29.3168047115564,1.22732257376588));
#29390=CARTESIAN_POINT('Ctrl Pts',(23.9652487409628,-29.3252401898307,1.47243294816367));
#29391=CARTESIAN_POINT('Ctrl Pts',(23.9944359843099,-29.3336629639887,1.71717417803045));
#29392=CARTESIAN_POINT('Ctrl Pts',(24.0278712558264,-29.3468690005325,1.96163791541615));
#29393=CARTESIAN_POINT('Ctrl Pts',(24.065517921745,-29.3648668425817,2.20532408778555));
#29394=CARTESIAN_POINT('Ctrl Pts',(24.1031322999561,-29.3828492487604,2.44880126242098));
#29395=CARTESIAN_POINT('Ctrl Pts',(24.1449508188711,-29.405615252335,2.69150175431084));
#29396=CARTESIAN_POINT('Ctrl Pts',(24.190902470982,-29.4331345151071,2.93292951866843));
#29397=CARTESIAN_POINT('Ctrl Pts',(24.2368445099157,-29.4606480207946,3.1743067758563));
#29398=CARTESIAN_POINT('Ctrl Pts',(24.2869178772577,-29.4929127564911,3.41441139318389));
#29399=CARTESIAN_POINT('Ctrl Pts',(24.3410179518308,-29.5298597835415,3.65275710614686));
#29400=CARTESIAN_POINT('Ctrl Pts',(24.3951867218144,-29.5668537253366,3.8914054666884));
#29401=CARTESIAN_POINT('Ctrl Pts',(24.4533923189747,-29.6085417737707,4.12829002081218));
#29402=CARTESIAN_POINT('Ctrl Pts',(24.5154973789737,-29.6548169223665,4.36293874377864));
#29403=CARTESIAN_POINT('Ctrl Pts',(24.5776658108999,-29.7011392900673,4.59782690201484));
#29404=CARTESIAN_POINT('Ctrl Pts',(24.6437415114726,-29.7520579892328,4.83047425894975));
#29405=CARTESIAN_POINT('Ctrl Pts',(24.713556330989,-29.8074294704423,5.06042975959428));
#29406=CARTESIAN_POINT('Ctrl Pts',(24.7835752616711,-29.8629628361579,5.29105755998308));
#29407=CARTESIAN_POINT('Ctrl Pts',(24.8573550203555,-29.9229748872205,5.51897736305697));
#29408=CARTESIAN_POINT('Ctrl Pts',(24.934698018064,-29.9872866904183,5.74376259354346));
#29409=CARTESIAN_POINT('Ctrl Pts',(24.9840142132782,-30.0282938085162,5.88709234072629));
#29410=CARTESIAN_POINT('Ctrl Pts',(25.0347785642248,-30.0710484023926,6.02914825314197));
#29411=CARTESIAN_POINT('Ctrl Pts',(25.0869345108126,-30.1154974142346,6.16982677023484));
#29412=CARTESIAN_POINT('Ctrl Pts',(25.1687165693391,-30.1851947723641,6.39041482339095));
#29413=CARTESIAN_POINT('Ctrl Pts',(25.2545422584419,-30.2593411758393,6.60890054011814));
#29414=CARTESIAN_POINT('Ctrl Pts',(25.3442989836975,-30.3378542445908,6.82480412008055));
#29415=CARTESIAN_POINT('Ctrl Pts',(25.4338530781079,-30.4161900656829,7.04022028559292));
#29416=CARTESIAN_POINT('Ctrl Pts',(25.5273204012121,-30.4988728090636,7.25306552029623));
#29417=CARTESIAN_POINT('Ctrl Pts',(25.6245550984951,-30.5857836273894,7.4628756626939));
#29418=CARTESIAN_POINT('Ctrl Pts',(25.7216334025455,-30.67255465751,7.67234834441854));
#29419=CARTESIAN_POINT('Ctrl Pts',(25.8224668509011,-30.76354007733,7.87879526533001));
#29420=CARTESIAN_POINT('Ctrl Pts',(25.9268778285521,-30.8585857424181,8.08177334612168));
#29421=CARTESIAN_POINT('Ctrl Pts',(26.031188620113,-30.9535402077705,8.28455666214093));
#29422=CARTESIAN_POINT('Ctrl Pts',(26.1390699181374,-31.052546990739,8.48387739272847));
#29423=CARTESIAN_POINT('Ctrl Pts',(26.2503142961675,-31.155418315607,8.67931873611097));
#29424=CARTESIAN_POINT('Ctrl Pts',(26.3615640247578,-31.2582945883135,8.87476947970483));
#29425=CARTESIAN_POINT('Ctrl Pts',(26.4761769610836,-31.3650355954447,9.06634009532807));
#29426=CARTESIAN_POINT('Ctrl Pts',(26.5939179778762,-31.4754218249885,9.2536445034095));
#29427=CARTESIAN_POINT('Ctrl Pts',(26.711702186799,-31.5858485486314,9.44101762226479));
#29428=CARTESIAN_POINT('Ctrl Pts',(26.8326165417653,-31.6999229509137,9.62412107875033));
#29429=CARTESIAN_POINT('Ctrl Pts',(26.9564011630246,-31.8173965346654,9.8026043746614));
#29430=CARTESIAN_POINT('Ctrl Pts',(27.0803877026405,-31.9350617421642,9.98137881379707));
#29431=CARTESIAN_POINT('Ctrl Pts',(27.2072536245433,-32.0561369802841,10.1555177270928));
#29432=CARTESIAN_POINT('Ctrl Pts',(27.3367168513604,-32.1803472149487,10.3247095747713));
#29433=CARTESIAN_POINT('Ctrl Pts',(27.3741361061487,-32.2162481771949,10.3736117457742));
#29434=CARTESIAN_POINT('Ctrl Pts',(27.4117722217276,-32.2524108910196,10.4221009095725));
#29435=CARTESIAN_POINT('Ctrl Pts',(27.4496181106863,-32.288828370087,10.4701702229062));
#29436=CARTESIAN_POINT('Ctrl Pts',(31.7027984407109,-31.3186840564489,1.04083408558608E-14));
#29437=CARTESIAN_POINT('Ctrl Pts',(31.8647447780725,-31.1783567563178,1.72780310113343));
#29438=CARTESIAN_POINT('Ctrl Pts',(32.5176177262899,-31.604588967181,3.28449990511991));
#29439=CARTESIAN_POINT('Ctrl Pts',(33.1704906745074,-32.0308211780443,4.84119670910639));
#29440=CARTESIAN_POINT('Ctrl Pts',(34.2170561974809,-32.9113988403531,5.91846432228298));
#29441=CARTESIAN_POINT('Ctrl Pts',(35.2636217204544,-33.791976502662,6.99573193545957));
#29442=CARTESIAN_POINT('Ctrl Pts',(36.5286701393312,-34.9246968680274,7.3802042952164));
#29443=CARTESIAN_POINT('Ctrl Pts',(37.793718558208,-36.0574172333928,7.76467665497322));
#29444=CARTESIAN_POINT('Ctrl Pts',(39.0587669770848,-37.1901375987582,7.38020429521639));
#29445=CARTESIAN_POINT('Ctrl Pts',(29.4615173807452,-30.5436667170416,0.));
#29446=CARTESIAN_POINT('Ctrl Pts',(29.6234637181068,-30.4033394169105,2.19648874705823));
#29447=CARTESIAN_POINT('Ctrl Pts',(30.4095059236081,-30.983257143323,4.17545672685568));
#29448=CARTESIAN_POINT('Ctrl Pts',(31.1955481291094,-31.5631748697354,6.15442470665313));
#29449=CARTESIAN_POINT('Ctrl Pts',(32.4820763620317,-32.720684261959,7.5239130403414));
#29450=CARTESIAN_POINT('Ctrl Pts',(33.7686045949541,-33.8781936541826,8.89340137402968));
#29451=CARTESIAN_POINT('Ctrl Pts',(35.3328816187898,-35.356242238374,9.3821661014496));
#29452=CARTESIAN_POINT('Ctrl Pts',(36.8971586426256,-36.8342908225653,9.87093082886953));
#29453=CARTESIAN_POINT('Ctrl Pts',(38.4614356664613,-38.3123394067567,9.3821661014496));
#29454=CARTESIAN_POINT('Ctrl Pts',(27.4145036200618,-29.3462831821141,-1.05434036998093E-14));
#29455=CARTESIAN_POINT('Ctrl Pts',(27.5764499574234,-29.205955881983,2.7089937269807));
#29456=CARTESIAN_POINT('Ctrl Pts',(28.5081119576079,-29.9539278100673,5.14971273833323));
#29457=CARTESIAN_POINT('Ctrl Pts',(29.4397739577924,-30.7018997381516,7.59043174968578));
#29458=CARTESIAN_POINT('Ctrl Pts',(30.9886999938346,-32.1622323380282,9.27946171175751));
#29459=CARTESIAN_POINT('Ctrl Pts',(32.5376260298767,-33.6225649379048,10.9684916738293));
#29460=CARTESIAN_POINT('Ctrl Pts',(34.4291077622632,-35.4782278855717,11.5712994880388));
#29461=CARTESIAN_POINT('Ctrl Pts',(36.3205894946496,-37.3338908332386,12.1741073022483));
#29462=CARTESIAN_POINT('Ctrl Pts',(38.2120712270361,-39.1895537809055,11.5712994880388));
#29463=CARTESIAN_POINT('Ctrl Pts',(25.6404249706855,-27.772549528674,0.));
#29464=CARTESIAN_POINT('Ctrl Pts',(25.8023713080471,-27.6322222285429,3.24562220582793));
#29465=CARTESIAN_POINT('Ctrl Pts',(26.8865073952594,-28.5561586333444,6.16982677025167));
#29466=CARTESIAN_POINT('Ctrl Pts',(27.9706434824718,-29.480095038146,9.09403133467541));
#29467=CARTESIAN_POINT('Ctrl Pts',(29.7943183296618,-31.2575046687805,11.1176436806954));
#29468=CARTESIAN_POINT('Ctrl Pts',(31.6179931768518,-33.034914299415,13.1412560267153));
#29469=CARTESIAN_POINT('Ctrl Pts',(33.8520810728853,-35.2859658372444,13.8634749112255));
#29470=CARTESIAN_POINT('Ctrl Pts',(36.0861689689187,-37.5370173750738,14.5856937957357));
#29471=CARTESIAN_POINT('Ctrl Pts',(38.3202568649522,-39.7880689129032,13.8634749112255));
#29472=CARTESIAN_POINT('',(25.6404249706855,-27.772549528674,0.));
#29473=CARTESIAN_POINT('Ctrl Pts',(25.6404249706855,-27.772549528674,0.));
#29474=CARTESIAN_POINT('Ctrl Pts',(25.8023713080471,-27.6322222285429,3.24562220582793));
#29475=CARTESIAN_POINT('Ctrl Pts',(26.8865073952594,-28.5561586333444,6.16982677025168));
#29476=CARTESIAN_POINT('Ctrl Pts',(27.7915854309814,-29.3274958817337,8.61106394926977));
#29477=CARTESIAN_POINT('Ctrl Pts',(29.2324872694335,-30.7134197505154,10.4489096280657));
#29478=CARTESIAN_POINT('Origin',(37.5852932322715,-14.3070334890506,0.));
#29479=CARTESIAN_POINT('Ctrl Pts',(25.6404249706855,-27.772549528674,0.));
#29480=CARTESIAN_POINT('Ctrl Pts',(25.8023713080471,-27.6322222285429,3.24562220582793));
#29481=CARTESIAN_POINT('Ctrl Pts',(26.8865073952594,-28.5561586333444,6.16982677025168));
#29482=CARTESIAN_POINT('Ctrl Pts',(27.9706434824718,-29.480095038146,9.09403133467541));
#29483=CARTESIAN_POINT('Ctrl Pts',(29.7943183296618,-31.2575046687805,11.1176436806954));
#29484=CARTESIAN_POINT('Ctrl Pts',(31.6179931768518,-33.0349142994151,13.1412560267153));
#29485=CARTESIAN_POINT('Ctrl Pts',(33.8520810728853,-35.2859658372444,13.8634749112255));
#29486=CARTESIAN_POINT('Ctrl Pts',(36.0861689689187,-37.5370173750738,14.5856937957357));
#29487=CARTESIAN_POINT('Ctrl Pts',(38.3202568649522,-39.7880689129032,13.8634749112255));
#29488=CARTESIAN_POINT('Ctrl Pts',(24.6879908429602,-27.764228931089,6.24500451351652E-15));
#29489=CARTESIAN_POINT('Ctrl Pts',(24.8499371803218,-27.6239016309578,3.38941559469372));
#29490=CARTESIAN_POINT('Ctrl Pts',(25.9749297754389,-28.5949889593956,6.44317352589574));
#29491=CARTESIAN_POINT('Ctrl Pts',(27.0999223705561,-29.5660762878334,9.49693145709774));
#29492=CARTESIAN_POINT('Ctrl Pts',(28.9972181010929,-31.4284489470462,11.6101975146502));
#29493=CARTESIAN_POINT('Ctrl Pts',(30.8945138316298,-33.2908216062589,13.7234635722027));
#29494=CARTESIAN_POINT('Ctrl Pts',(33.2204054676043,-35.6478203077954,14.4776794959001));
#29495=CARTESIAN_POINT('Ctrl Pts',(35.5462971035789,-38.0048190093319,15.2318954195974));
#29496=CARTESIAN_POINT('Ctrl Pts',(37.8721887395536,-40.3618177108684,14.4776794959001));
#29497=CARTESIAN_POINT('Ctrl Pts',(23.9681616891738,-28.3879644434331,0.));
#29498=CARTESIAN_POINT('Ctrl Pts',(24.1301080265355,-28.247637143302,3.38941559469374));
#29499=CARTESIAN_POINT('Ctrl Pts',(25.2551006216526,-29.2187244717398,6.44317352589574));
#29500=CARTESIAN_POINT('Ctrl Pts',(26.3800932167697,-30.1898118001776,9.49693145709774));
#29501=CARTESIAN_POINT('Ctrl Pts',(28.2773889473065,-32.0521844593903,11.6101975146502));
#29502=CARTESIAN_POINT('Ctrl Pts',(30.1746846778434,-33.9145571186031,13.7234635722027));
#29503=CARTESIAN_POINT('Ctrl Pts',(32.500576313818,-36.2715558201396,14.4776794959001));
#29504=CARTESIAN_POINT('Ctrl Pts',(34.8264679497926,-38.6285545216761,15.2318954195974));
#29505=CARTESIAN_POINT('Ctrl Pts',(37.1523595857672,-40.9855532232126,14.4776794959001));
#29506=CARTESIAN_POINT('Ctrl Pts',(23.8408520862196,-29.3318883095344,0.));
#29507=CARTESIAN_POINT('Ctrl Pts',(24.0027984235812,-29.1915610094033,3.24562220582793));
#29508=CARTESIAN_POINT('Ctrl Pts',(25.0869345107935,-30.1154974142048,6.16982677025168));
#29509=CARTESIAN_POINT('Ctrl Pts',(26.1710705980059,-31.0394338190064,9.09403133467541));
#29510=CARTESIAN_POINT('Ctrl Pts',(27.9947454451959,-32.8168434496409,11.1176436806954));
#29511=CARTESIAN_POINT('Ctrl Pts',(29.8184202923859,-34.5942530802755,13.1412560267153));
#29512=CARTESIAN_POINT('Ctrl Pts',(32.0525081884194,-36.8453046181048,13.8634749112255));
#29513=CARTESIAN_POINT('Ctrl Pts',(34.2865960844529,-39.0963561559342,14.5856937957357));
#29514=CARTESIAN_POINT('Ctrl Pts',(36.5206839804863,-41.3474076937636,13.8634749112255));
#29515=CARTESIAN_POINT('',(24.4459474390596,-28.2121348679478,1.9100087581672E-29));
#29516=CARTESIAN_POINT('Origin',(25.6247005192787,-29.5724808444825,0.));
#29517=CARTESIAN_POINT('Origin',(25.6247005192787,-29.5724808444825,0.));
#29518=CARTESIAN_POINT('Ctrl Pts',(19.4238236466305,-32.4262389885815,0.));
#29519=CARTESIAN_POINT('Ctrl Pts',(19.6040922608086,-32.3103873848411,3.24562220582793));
#29520=CARTESIAN_POINT('Ctrl Pts',(20.5457035458241,-33.3792081011658,6.16982677025167));
#29521=CARTESIAN_POINT('Ctrl Pts',(21.4873148308396,-34.4480288174907,9.09403133467541));
#29522=CARTESIAN_POINT('Ctrl Pts',(23.0394755334781,-36.4668829718393,11.1176436806954));
#29523=CARTESIAN_POINT('Ctrl Pts',(24.5916362361166,-38.4857371261879,13.1412560267153));
#29524=CARTESIAN_POINT('Ctrl Pts',(26.4826263031061,-41.0318200627228,13.8634749112255));
#29525=CARTESIAN_POINT('Ctrl Pts',(28.3736163700957,-43.5779029992577,14.5856937957357));
#29526=CARTESIAN_POINT('Ctrl Pts',(30.2646064370852,-46.1239859357925,13.8634749112255));
#29527=CARTESIAN_POINT('Ctrl Pts',(20.4339943155202,-34.5718269932687,-1.05434036998093E-14));
#29528=CARTESIAN_POINT('Ctrl Pts',(20.6142629296984,-34.4559753895282,2.7089937269807));
#29529=CARTESIAN_POINT('Ctrl Pts',(21.4299944500884,-35.3289233687527,5.14971273833323));
#29530=CARTESIAN_POINT('Ctrl Pts',(22.2457259704784,-36.2018713479772,7.59043174968578));
#29531=CARTESIAN_POINT('Ctrl Pts',(23.5710591750639,-37.8677750259294,9.27946171175752));
#29532=CARTESIAN_POINT('Ctrl Pts',(24.8963923796494,-39.5336787038816,10.9684916738293));
#29533=CARTESIAN_POINT('Ctrl Pts',(26.5045331830047,-41.6396395952277,11.5712994880388));
#29534=CARTESIAN_POINT('Ctrl Pts',(28.1126739863599,-43.7456004865739,12.1741073022483));
#29535=CARTESIAN_POINT('Ctrl Pts',(29.7208147897152,-45.8515613779201,11.5712994880388));
#29536=CARTESIAN_POINT('Ctrl Pts',(21.0061649833179,-36.8732642383516,-1.05434036998093E-14));
#29537=CARTESIAN_POINT('Ctrl Pts',(21.186433597496,-36.7574126346111,2.19648874705824));
#29538=CARTESIAN_POINT('Ctrl Pts',(21.8819441292783,-37.4432931040929,4.17545672685568));
#29539=CARTESIAN_POINT('Ctrl Pts',(22.5774546610607,-38.1291735735747,6.15442470665314));
#29540=CARTESIAN_POINT('Ctrl Pts',(23.6861571296383,-39.4579932465786,7.5239130403414));
#29541=CARTESIAN_POINT('Ctrl Pts',(24.7948595982159,-40.7868129195824,8.89340137402968));
#29542=CARTESIAN_POINT('Ctrl Pts',(26.1328662922309,-42.4724369320186,9.38216610144961));
#29543=CARTESIAN_POINT('Ctrl Pts',(27.470872986246,-44.1580609444547,9.87093082886954));
#29544=CARTESIAN_POINT('Ctrl Pts',(28.8088796802611,-45.8436849568909,9.3821661014496));
#29545=CARTESIAN_POINT('Ctrl Pts',(21.1183468312841,-39.2421052839115,0.));
#29546=CARTESIAN_POINT('Ctrl Pts',(21.2986154454622,-39.1262536801711,1.72780310113343));
#29547=CARTESIAN_POINT('Ctrl Pts',(21.884183920276,-39.6410609697424,3.28449990511991));
#29548=CARTESIAN_POINT('Ctrl Pts',(22.4697523950898,-40.1558682593138,4.84119670910639));
#29549=CARTESIAN_POINT('Ctrl Pts',(23.3803461224637,-41.1764247138528,5.91846432228298));
#29550=CARTESIAN_POINT('Ctrl Pts',(24.2909398498377,-42.1969811683918,6.99573193545956));
#29551=CARTESIAN_POINT('Ctrl Pts',(25.3819089842537,-43.4982072348261,7.38020429521639));
#29552=CARTESIAN_POINT('Ctrl Pts',(26.4728781186697,-44.7994333012603,7.76467665497321));
#29553=CARTESIAN_POINT('Ctrl Pts',(27.5638472530857,-46.1006593676945,7.38020429521639));
#29554=CARTESIAN_POINT('',(19.4238236466412,-32.4262389886037,1.57949788822268E-9));
#29555=CARTESIAN_POINT('Origin',(3.1384973440476,-40.0935818932913,0.));
#29556=CARTESIAN_POINT('Ctrl Pts',(19.4238236468408,-32.4262389885472,3.13107065661919E-9));
#29557=CARTESIAN_POINT('Ctrl Pts',(19.4374335758626,-32.4174924183249,0.245038153335379));
#29558=CARTESIAN_POINT('Ctrl Pts',(19.4545900740527,-32.4140004629286,0.490791160521511));
#29559=CARTESIAN_POINT('Ctrl Pts',(19.4753132856565,-32.4158522216031,0.736766500725056));
#29560=CARTESIAN_POINT('Ctrl Pts',(19.4959684641204,-32.4176979010579,0.981934317700683));
#29561=CARTESIAN_POINT('Ctrl Pts',(19.5201670081213,-32.4248523667014,1.22732257376531));
#29562=CARTESIAN_POINT('Ctrl Pts',(19.547900248874,-32.437362026952,1.47243294816306));
#29563=CARTESIAN_POINT('Ctrl Pts',(19.5755917224262,-32.4498528472304,1.71717417802983));
#29564=CARTESIAN_POINT('Ctrl Pts',(19.6068072561333,-32.4676828006221,1.96163791541552));
#29565=CARTESIAN_POINT('Ctrl Pts',(19.6415093732944,-32.4908551297618,2.20532408778492));
#29566=CARTESIAN_POINT('Ctrl Pts',(19.6761817281436,-32.5140075851259,2.44880126242038));
#29567=CARTESIAN_POINT('Ctrl Pts',(19.7143346547166,-32.5424932593662,2.69150175431026));
#29568=CARTESIAN_POINT('Ctrl Pts',(19.755902185835,-32.5762720176614,2.93292951866789));
#29569=CARTESIAN_POINT('Ctrl Pts',(19.797461020943,-32.6100437093729,3.17430677585578));
#29570=CARTESIAN_POINT('Ctrl Pts',(19.8424329629628,-32.649106219757,3.4144113931834));
#29571=CARTESIAN_POINT('Ctrl Pts',(19.8907242666033,-32.6933764227087,3.6527571061464));
#29572=CARTESIAN_POINT('Ctrl Pts',(19.9390768897696,-32.7377028392568,3.89140546668789));
#29573=CARTESIAN_POINT('Ctrl Pts',(19.9907572100055,-32.7872500836135,4.12829002081164));
#29574=CARTESIAN_POINT('Ctrl Pts',(20.0456444897533,-32.8418926894896,4.36293874377806));
#29575=CARTESIAN_POINT('Ctrl Pts',(20.1005877764142,-32.8965910526139,4.59782690201453));
#29576=CARTESIAN_POINT('Ctrl Pts',(20.1587444351917,-32.9563950254815,4.83047425894971));
#29577=CARTESIAN_POINT('Ctrl Pts',(20.2199684571168,-33.0211385895999,5.0604297595945));
#29578=CARTESIAN_POINT('Ctrl Pts',(20.281371474083,-33.0860714385212,5.29105755998329));
#29579=CARTESIAN_POINT('Ctrl Pts',(20.3458596558642,-33.1559726078591,5.51897736305717));
#29580=CARTESIAN_POINT('Ctrl Pts',(20.4132628895043,-33.2306368658408,5.74376259354365));
#29581=CARTESIAN_POINT('Ctrl Pts',(20.456241195579,-33.27824501695,5.88709234072642));
#29582=CARTESIAN_POINT('Ctrl Pts',(20.5004042255162,-33.3277889511028,6.02914825314203));
#29583=CARTESIAN_POINT('Ctrl Pts',(20.5457035458387,-33.379208101198,6.16982677023483));
#29584=CARTESIAN_POINT('Ctrl Pts',(20.6167342126791,-33.4598348411499,6.39041482339093));
#29585=CARTESIAN_POINT('Ctrl Pts',(20.6911341865981,-33.5454408102123,6.6089005401181));
#29586=CARTESIAN_POINT('Ctrl Pts',(20.7688037431274,-33.6359284429692,6.8248041200805));
#29587=CARTESIAN_POINT('Ctrl Pts',(20.8462979562734,-33.7262117948162,7.04022028559294));
#29588=CARTESIAN_POINT('Ctrl Pts',(20.927046935545,-33.8213547340594,7.25306552029632));
#29589=CARTESIAN_POINT('Ctrl Pts',(21.0109232247562,-33.9212188657881,7.46287566269406));
#29590=CARTESIAN_POINT('Ctrl Pts',(21.0946646065284,-34.0209223750764,7.67234834441878));
#29591=CARTESIAN_POINT('Ctrl Pts',(21.1815231404626,-34.1253317904081,7.87879526533031));
#29592=CARTESIAN_POINT('Ctrl Pts',(21.2713449564538,-34.2342692590686,8.08177334612205));
#29593=CARTESIAN_POINT('Ctrl Pts',(21.3610805851804,-34.3431021983077,8.28455666214114));
#29594=CARTESIAN_POINT('Ctrl Pts',(21.4537736728366,-34.4564543444626,8.48387739272852));
#29595=CARTESIAN_POINT('Ctrl Pts',(21.5492456275379,-34.5741103132398,8.67931873611087));
#29596=CARTESIAN_POINT('Ctrl Pts',(21.6447221741876,-34.6917719409576,8.87476947970466));
#29597=CARTESIAN_POINT('Ctrl Pts',(21.7429776869128,-34.8137376000412,9.06634009532782));
#29598=CARTESIAN_POINT('Ctrl Pts',(21.8438106715178,-34.939756550695,9.25364450340919));
#29599=CARTESIAN_POINT('Ctrl Pts',(21.9446806457081,-35.0658217301572,9.44101762226418));
#29600=CARTESIAN_POINT('Ctrl Pts',(22.0481297867729,-35.1959429263777,9.62412107874944));
#29601=CARTESIAN_POINT('Ctrl Pts',(22.1539362249972,-35.3298371867847,9.80260437466024));
#29602=CARTESIAN_POINT('Ctrl Pts',(22.259915255438,-35.4639498564639,9.98137881379584));
#29603=CARTESIAN_POINT('Ctrl Pts',(22.3682590622494,-35.6018476263936,10.1555177270916));
#29604=CARTESIAN_POINT('Ctrl Pts',(22.4787275806298,-35.7432181181524,10.32470957477));
#29605=CARTESIAN_POINT('Ctrl Pts',(22.510656721724,-35.7840789755632,10.373611745775));
#29606=CARTESIAN_POINT('Ctrl Pts',(22.5427632651449,-35.825229782807,10.4221009095754));
#29607=CARTESIAN_POINT('Ctrl Pts',(22.5750411898809,-35.8666626160155,10.4701702229111));
#29608=CARTESIAN_POINT('Ctrl Pts',(26.9229962078193,-35.511683643468,0.));
#29609=CARTESIAN_POINT('Ctrl Pts',(27.1032648219974,-35.3958320397275,1.72780310113343));
#29610=CARTESIAN_POINT('Ctrl Pts',(27.6888332968112,-35.9106393292988,3.28449990511992));
#29611=CARTESIAN_POINT('Ctrl Pts',(28.274401771625,-36.4254466188702,4.84119670910639));
#29612=CARTESIAN_POINT('Ctrl Pts',(29.184995498999,-37.4460030734092,5.91846432228298));
#29613=CARTESIAN_POINT('Ctrl Pts',(30.0955892263729,-38.4665595279482,6.99573193545956));
#29614=CARTESIAN_POINT('Ctrl Pts',(31.1865583607889,-39.7677855943825,7.3802042952164));
#29615=CARTESIAN_POINT('Ctrl Pts',(32.2775274952049,-41.0690116608167,7.76467665497323));
#29616=CARTESIAN_POINT('Ctrl Pts',(33.3684966296209,-42.3702377272509,7.3802042952164));
#29617=CARTESIAN_POINT('Ctrl Pts',(24.8148246247004,-34.4255873115191,0.));
#29618=CARTESIAN_POINT('Ctrl Pts',(24.9950932388786,-34.3097357077786,2.19648874705823));
#29619=CARTESIAN_POINT('Ctrl Pts',(25.6906037706609,-34.9956161772605,4.17545672685568));
#29620=CARTESIAN_POINT('Ctrl Pts',(26.3861143024432,-35.6814966467423,6.15442470665315));
#29621=CARTESIAN_POINT('Ctrl Pts',(27.4948167710208,-37.0103163197461,7.52391304034141));
#29622=CARTESIAN_POINT('Ctrl Pts',(28.6035192395985,-38.33913599275,8.89340137402968));
#29623=CARTESIAN_POINT('Ctrl Pts',(29.9415259336135,-40.0247600051861,9.38216610144961));
#29624=CARTESIAN_POINT('Ctrl Pts',(31.2795326276286,-41.7103840176223,9.87093082886955));
#29625=CARTESIAN_POINT('Ctrl Pts',(32.6175393216436,-43.3960080300584,9.38216610144961));
#29626=CARTESIAN_POINT('Ctrl Pts',(22.959051956675,-32.9490709821979,0.));
#29627=CARTESIAN_POINT('Ctrl Pts',(23.1393205708531,-32.8332193784574,2.7089937269807));
#29628=CARTESIAN_POINT('Ctrl Pts',(23.9550520912431,-33.7061673576819,5.14971273833323));
#29629=CARTESIAN_POINT('Ctrl Pts',(24.7707836116331,-34.5791153369064,7.59043174968579));
#29630=CARTESIAN_POINT('Ctrl Pts',(26.0961168162186,-36.2450190148586,9.27946171175752));
#29631=CARTESIAN_POINT('Ctrl Pts',(27.4214500208042,-37.9109226928107,10.9684916738293));
#29632=CARTESIAN_POINT('Ctrl Pts',(29.0295908241594,-40.0168835841569,11.5712994880388));
#29633=CARTESIAN_POINT('Ctrl Pts',(30.6377316275147,-42.1228444755031,12.1741073022483));
#29634=CARTESIAN_POINT('Ctrl Pts',(32.2458724308699,-44.2288053668492,11.5712994880388));
#29635=CARTESIAN_POINT('Ctrl Pts',(21.4269965203137,-31.1388779521432,0.));
#29636=CARTESIAN_POINT('Ctrl Pts',(21.6072651344918,-31.0230263484027,3.24562220582792));
#29637=CARTESIAN_POINT('Ctrl Pts',(22.5488764195073,-32.0918470647275,6.16982677025168));
#29638=CARTESIAN_POINT('Ctrl Pts',(23.4904877045229,-33.1606677810523,9.09403133467541));
#29639=CARTESIAN_POINT('Ctrl Pts',(25.0426484071614,-35.1795219354009,11.1176436806954));
#29640=CARTESIAN_POINT('Ctrl Pts',(26.5948091097998,-37.1983760897496,13.1412560267153));
#29641=CARTESIAN_POINT('Ctrl Pts',(28.4857991767894,-39.7444590262845,13.8634749112255));
#29642=CARTESIAN_POINT('Ctrl Pts',(30.3767892437789,-42.2905419628193,14.5856937957357));
#29643=CARTESIAN_POINT('Ctrl Pts',(32.2677793107685,-44.8366248993542,13.8634749112255));
#29644=CARTESIAN_POINT('',(21.4269965203137,-31.1388779521432,0.));
#29645=CARTESIAN_POINT('Ctrl Pts',(21.4269965203137,-31.1388779521432,0.));
#29646=CARTESIAN_POINT('Ctrl Pts',(21.6072651344918,-31.0230263484027,3.24562220582792));
#29647=CARTESIAN_POINT('Ctrl Pts',(22.5488764195073,-32.0918470647275,6.16982677025168));
#29648=CARTESIAN_POINT('Ctrl Pts',(23.3349693300818,-32.9841392463831,8.61106394926976));
#29649=CARTESIAN_POINT('Ctrl Pts',(24.5639673341825,-34.5610181206248,10.4489096280657));
#29650=CARTESIAN_POINT('Origin',(35.1666259835199,-19.5103534449756,1.04083408558608E-14));
#29651=CARTESIAN_POINT('Ctrl Pts',(21.4269965203137,-31.1388779521432,0.));
#29652=CARTESIAN_POINT('Ctrl Pts',(21.6072651344918,-31.0230263484027,3.24562220582792));
#29653=CARTESIAN_POINT('Ctrl Pts',(22.5488764195073,-32.0918470647275,6.16982677025167));
#29654=CARTESIAN_POINT('Ctrl Pts',(23.4904877045229,-33.1606677810523,9.09403133467541));
#29655=CARTESIAN_POINT('Ctrl Pts',(25.0426484071614,-35.1795219354009,11.1176436806954));
#29656=CARTESIAN_POINT('Ctrl Pts',(26.5948091097998,-37.1983760897496,13.1412560267153));
#29657=CARTESIAN_POINT('Ctrl Pts',(28.4857991767894,-39.7444590262845,13.8634749112255));
#29658=CARTESIAN_POINT('Ctrl Pts',(30.3767892437789,-42.2905419628193,14.5856937957357));
#29659=CARTESIAN_POINT('Ctrl Pts',(32.2677793107685,-44.8366248993542,13.8634749112255));
#29660=CARTESIAN_POINT('Ctrl Pts',(20.4854409432117,-30.995096537391,0.));
#29661=CARTESIAN_POINT('Ctrl Pts',(20.6657095573898,-30.8792449336506,3.38941559469372));
#29662=CARTESIAN_POINT('Ctrl Pts',(21.6410512138981,-32.0005511325099,6.44317352589574));
#29663=CARTESIAN_POINT('Ctrl Pts',(22.6163928704065,-33.1218573313692,9.49693145709775));
#29664=CARTESIAN_POINT('Ctrl Pts',(24.2293336022805,-35.2352870572788,11.6101975146502));
#29665=CARTESIAN_POINT('Ctrl Pts',(25.8422743341546,-37.3487167831883,13.7234635722027));
#29666=CARTESIAN_POINT('Ctrl Pts',(27.8090558579143,-40.0127335284696,14.4776794959001));
#29667=CARTESIAN_POINT('Ctrl Pts',(29.775837381674,-42.6767502737508,15.2318954195974));
#29668=CARTESIAN_POINT('Ctrl Pts',(31.7426189054336,-45.3407670190321,14.4776794959001));
#29669=CARTESIAN_POINT('Ctrl Pts',(19.6841717937384,-31.5100409519664,0.));
#29670=CARTESIAN_POINT('Ctrl Pts',(19.8644404079165,-31.3941893482259,3.38941559469373));
#29671=CARTESIAN_POINT('Ctrl Pts',(20.8397820644248,-32.5154955470852,6.44317352589574));
#29672=CARTESIAN_POINT('Ctrl Pts',(21.8151237209332,-33.6368017459446,9.49693145709774));
#29673=CARTESIAN_POINT('Ctrl Pts',(23.4280644528072,-35.7502314718541,11.6101975146502));
#29674=CARTESIAN_POINT('Ctrl Pts',(25.0410051846813,-37.8636611977637,13.7234635722027));
#29675=CARTESIAN_POINT('Ctrl Pts',(27.007786708441,-40.5276779430449,14.4776794959001));
#29676=CARTESIAN_POINT('Ctrl Pts',(28.9745682322006,-43.1916946883262,15.2318954195974));
#29677=CARTESIAN_POINT('Ctrl Pts',(30.9413497559604,-45.8557114336074,14.4776794959001));
#29678=CARTESIAN_POINT('Ctrl Pts',(19.4238236466305,-32.4262389885815,0.));
#29679=CARTESIAN_POINT('Ctrl Pts',(19.6040922608086,-32.3103873848411,3.24562220582793));
#29680=CARTESIAN_POINT('Ctrl Pts',(20.5457035458241,-33.3792081011658,6.16982677025167));
#29681=CARTESIAN_POINT('Ctrl Pts',(21.4873148308396,-34.4480288174907,9.09403133467541));
#29682=CARTESIAN_POINT('Ctrl Pts',(23.0394755334781,-36.4668829718393,11.1176436806954));
#29683=CARTESIAN_POINT('Ctrl Pts',(24.5916362361166,-38.4857371261879,13.1412560267153));
#29684=CARTESIAN_POINT('Ctrl Pts',(26.4826263031061,-41.0318200627228,13.8634749112255));
#29685=CARTESIAN_POINT('Ctrl Pts',(28.3736163700957,-43.5779029992577,14.5856937957357));
#29686=CARTESIAN_POINT('Ctrl Pts',(30.2646064370852,-46.1239859357925,13.8634749112255));
#29687=CARTESIAN_POINT('',(20.182117531154,-31.4039970697876,1.88545294717751E-29));
#29688=CARTESIAN_POINT('Origin',(21.1552751870371,-32.9182507396845,0.));
#29689=CARTESIAN_POINT('Origin',(21.1552751870371,-32.9182507396845,0.));
#29690=CARTESIAN_POINT('Ctrl Pts',(14.6113821712778,-34.8604849513725,0.));
#29691=CARTESIAN_POINT('Ctrl Pts',(14.8063033131395,-34.7714674485864,3.24562220582793));
#29692=CARTESIAN_POINT('Ctrl Pts',(15.586221305578,-35.9634143688745,6.16982677025167));
#29693=CARTESIAN_POINT('Ctrl Pts',(16.3661392980166,-37.1553612891626,9.09403133467541));
#29694=CARTESIAN_POINT('Ctrl Pts',(17.6151883402596,-39.3745619185374,11.1176436806954));
#29695=CARTESIAN_POINT('Ctrl Pts',(18.8642373825027,-41.5937625479123,13.1412560267153));
#29696=CARTESIAN_POINT('Ctrl Pts',(20.3736345158495,-44.3830459768616,13.8634749112255));
#29697=CARTESIAN_POINT('Ctrl Pts',(21.8830316491963,-47.172329405811,14.5856937957357));
#29698=CARTESIAN_POINT('Ctrl Pts',(23.3924287825431,-49.9616128347604,13.8634749112255));
#29699=CARTESIAN_POINT('Ctrl Pts',(15.305921749416,-37.1279962392258,0.));
#29700=CARTESIAN_POINT('Ctrl Pts',(15.5008428912777,-37.0389787364397,2.70899372698069));
#29701=CARTESIAN_POINT('Ctrl Pts',(16.1840379904935,-38.0191320633215,5.14971273833323));
#29702=CARTESIAN_POINT('Ctrl Pts',(16.8672330897094,-38.9992853902033,7.59043174968577));
#29703=CARTESIAN_POINT('Ctrl Pts',(17.9419935007382,-40.8368471514174,9.27946171175751));
#29704=CARTESIAN_POINT('Ctrl Pts',(19.0167539117671,-42.6744089126316,10.9684916738292));
#29705=CARTESIAN_POINT('Ctrl Pts',(20.30881667683,-44.9877964569989,11.5712994880388));
#29706=CARTESIAN_POINT('Ctrl Pts',(21.6008794418929,-47.3011840013662,12.1741073022483));
#29707=CARTESIAN_POINT('Ctrl Pts',(22.8929422069557,-49.6145715457335,11.5712994880388));
#29708=CARTESIAN_POINT('Ctrl Pts',(15.5447398754874,-39.4874365476046,0.));
#29709=CARTESIAN_POINT('Ctrl Pts',(15.739661017349,-39.3984190448185,2.19648874705823));
#29710=CARTESIAN_POINT('Ctrl Pts',(16.3304812866721,-40.1762997089269,4.17545672685568));
#29711=CARTESIAN_POINT('Ctrl Pts',(16.9213015559951,-40.9541803730353,6.15442470665314));
#29712=CARTESIAN_POINT('Ctrl Pts',(17.8296082752017,-42.4272593902766,7.5239130403414));
#29713=CARTESIAN_POINT('Ctrl Pts',(18.7379149944082,-43.9003384075178,8.89340137402966));
#29714=CARTESIAN_POINT('Ctrl Pts',(19.8224134008051,-45.7592234042438,9.3821661014496));
#29715=CARTESIAN_POINT('Ctrl Pts',(20.9069118072021,-47.6181084009698,9.87093082886953));
#29716=CARTESIAN_POINT('Ctrl Pts',(21.991410213599,-49.4769933976958,9.3821661014496));
#29717=CARTESIAN_POINT('Ctrl Pts',(15.3186586437002,-41.848131348458,0.));
#29718=CARTESIAN_POINT('Ctrl Pts',(15.5135797855619,-41.7591138456719,1.72780310113342));
#29719=CARTESIAN_POINT('Ctrl Pts',(16.0199233014648,-42.3520162221173,3.28449990511991));
#29720=CARTESIAN_POINT('Ctrl Pts',(16.5262668173678,-42.9449185985627,4.84119670910638));
#29721=CARTESIAN_POINT('Ctrl Pts',(17.2823516867883,-44.0846782589593,5.91846432228297));
#29722=CARTESIAN_POINT('Ctrl Pts',(18.0384365562089,-45.2244379193559,6.99573193545956));
#29723=CARTESIAN_POINT('Ctrl Pts',(18.9331174206825,-46.6676804765724,7.38020429521639));
#29724=CARTESIAN_POINT('Ctrl Pts',(19.8277982851562,-48.1109230337889,7.76467665497321));
#29725=CARTESIAN_POINT('Ctrl Pts',(20.7224791496298,-49.5541655910055,7.38020429521638));
#29726=CARTESIAN_POINT('',(14.6113821712889,-34.8604849513849,1.57949468734771E-9));
#29727=CARTESIAN_POINT('Origin',(-2.59935965651579,-40.1321417817281,0.));
#29728=CARTESIAN_POINT('Ctrl Pts',(14.6113821714909,-34.8604849513684,3.13106366345279E-9));
#29729=CARTESIAN_POINT('Ctrl Pts',(14.6260983377858,-34.8537643034671,0.245038153335408));
#29730=CARTESIAN_POINT('Ctrl Pts',(14.6435771646294,-34.852749515407,0.490791160521576));
#29731=CARTESIAN_POINT('Ctrl Pts',(14.6638259110832,-34.8575316463562,0.736766500725157));
#29732=CARTESIAN_POINT('Ctrl Pts',(14.6840081820396,-34.862298077838,0.981934317700836));
#29733=CARTESIAN_POINT('Ctrl Pts',(14.706942233133,-34.872823533213,1.22732257376552));
#29734=CARTESIAN_POINT('Ctrl Pts',(14.7326128792074,-34.8891527148323,1.47243294816331));
#29735=CARTESIAN_POINT('Ctrl Pts',(14.7582448644189,-34.9054573041506,1.71717417803004));
#29736=CARTESIAN_POINT('Ctrl Pts',(14.7866052020686,-34.9275482079566,1.96163791541569));
#29737=CARTESIAN_POINT('Ctrl Pts',(14.8176563354393,-34.9554233023889,2.20532408778503));
#29738=CARTESIAN_POINT('Ctrl Pts',(14.8486808377688,-34.9832744897134,2.4488012624205));
#29739=CARTESIAN_POINT('Ctrl Pts',(14.8823914884387,-35.0168999484378,2.69150175431039));
#29740=CARTESIAN_POINT('Ctrl Pts',(14.9187287035019,-35.056250564147,2.93292951866801));
#29741=CARTESIAN_POINT('Ctrl Pts',(14.9550583167473,-35.0955929476289,3.17430677585596));
#29742=CARTESIAN_POINT('Ctrl Pts',(14.9940133343936,-35.1406580326362,3.41441139318363));
#29743=CARTESIAN_POINT('Ctrl Pts',(15.0355127954199,-35.1913501978218,3.65275710614669));
#29744=CARTESIAN_POINT('Ctrl Pts',(15.0770649517989,-35.2421067311089,3.89140546668819));
#29745=CARTESIAN_POINT('Ctrl Pts',(15.1211679328242,-35.2985045323755,4.12829002081193));
#29746=CARTESIAN_POINT('Ctrl Pts',(15.167720085587,-35.3604022296525,4.36293874377836));
#29747=CARTESIAN_POINT('Ctrl Pts',(15.2143197401095,-35.4223630872641,4.5978269020147));
#29748=CARTESIAN_POINT('Ctrl Pts',(15.2633734552288,-35.4898348974064,4.83047425894974));
#29749=CARTESIAN_POINT('Ctrl Pts',(15.3147603350317,-35.5626325521734,5.0604297595944));
#29750=CARTESIAN_POINT('Ctrl Pts',(15.3662974499281,-35.635643038747,5.29105755998315));
#29751=CARTESIAN_POINT('Ctrl Pts',(15.4201812613936,-35.714010340131,5.51897736305698));
#29752=CARTESIAN_POINT('Ctrl Pts',(15.4762725955032,-35.797507103918,5.74376259354342));
#29753=CARTESIAN_POINT('Ctrl Pts',(15.5120380980662,-35.8507471233724,5.88709234072627));
#29754=CARTESIAN_POINT('Ctrl Pts',(15.5487007750601,-35.9060718261752,6.02914825314196));
#29755=CARTESIAN_POINT('Ctrl Pts',(15.5862213055879,-35.9634143689084,6.16982677023484));
#29756=CARTESIAN_POINT('Ctrl Pts',(15.6450546012009,-36.0533291627655,6.39041482339095));
#29757=CARTESIAN_POINT('Ctrl Pts',(15.706514291019,-36.1486520067524,6.60890054011813));
#29758=CARTESIAN_POINT('Ctrl Pts',(15.7705155506315,-36.2492721362564,6.82480412008053));
#29759=CARTESIAN_POINT('Ctrl Pts',(15.8343723238082,-36.3496651101704,7.04022028559287));
#29760=CARTESIAN_POINT('Ctrl Pts',(15.9007591428899,-36.4553314094026,7.25306552029615));
#29761=CARTESIAN_POINT('Ctrl Pts',(15.9695695446603,-36.5661159087965,7.4628756626938));
#29762=CARTESIAN_POINT('Ctrl Pts',(16.0382692711115,-36.6767222213245,7.67234834441846));
#29763=CARTESIAN_POINT('Ctrl Pts',(16.1093847013528,-36.7924301575636,7.87879526532994));
#29764=CARTESIAN_POINT('Ctrl Pts',(16.1827888425353,-36.913041777084,8.08177334612163));
#29765=CARTESIAN_POINT('Ctrl Pts',(16.2561225498028,-37.0335376654154,8.28455666214069));
#29766=CARTESIAN_POINT('Ctrl Pts',(16.3317404631311,-37.1589276519416,8.48387739272803));
#29767=CARTESIAN_POINT('Ctrl Pts',(16.4094964608244,-37.2889731283954,8.67931873611035));
#29768=CARTESIAN_POINT('Ctrl Pts',(16.4872561983753,-37.4190248596925,8.87476947970416));
#29769=CARTESIAN_POINT('Ctrl Pts',(16.5671540886063,-37.5537323016295,9.06634009532735));
#29770=CARTESIAN_POINT('Ctrl Pts',(16.6490263722356,-37.6928185909666,9.25364450340874));
#29771=CARTESIAN_POINT('Ctrl Pts',(16.7309286899041,-37.8319559027364,9.44101762226376));
#29772=CARTESIAN_POINT('Ctrl Pts',(16.8148066908781,-37.9754750005788,9.62412107874904));
#29773=CARTESIAN_POINT('Ctrl Pts',(16.9004810321061,-38.1230642366186,9.80260437465986));
#29774=CARTESIAN_POINT('Ctrl Pts',(16.9862951259303,-38.2708942212726,9.9813788137956));
#29775=CARTESIAN_POINT('Ctrl Pts',(17.0739112501815,-38.4228073220811,10.1555177270914));
#29776=CARTESIAN_POINT('Ctrl Pts',(17.1631362396561,-38.5784601754009,10.32470957477));
#29777=CARTESIAN_POINT('Ctrl Pts',(17.1889252818169,-38.6234491187491,10.3736117457733));
#29778=CARTESIAN_POINT('Ctrl Pts',(17.2148486564411,-38.6687503076427,10.4221009095721));
#29779=CARTESIAN_POINT('Ctrl Pts',(17.240901531486,-38.7143550419874,10.4701702229062));
#29780=CARTESIAN_POINT('Ctrl Pts',(21.5951194116464,-38.9817677587451,0.));
#29781=CARTESIAN_POINT('Ctrl Pts',(21.7900405535081,-38.892750255959,1.72780310113343));
#29782=CARTESIAN_POINT('Ctrl Pts',(22.296384069411,-39.4856526324043,3.28449990511992));
#29783=CARTESIAN_POINT('Ctrl Pts',(22.802727585314,-40.0785550088497,4.84119670910638));
#29784=CARTESIAN_POINT('Ctrl Pts',(23.5588124547345,-41.2183146692463,5.91846432228299));
#29785=CARTESIAN_POINT('Ctrl Pts',(24.3148973241551,-42.3580743296429,6.99573193545957));
#29786=CARTESIAN_POINT('Ctrl Pts',(25.2095781886287,-43.8013168868595,7.3802042952164));
#29787=CARTESIAN_POINT('Ctrl Pts',(26.1042590531024,-45.244559444076,7.76467665497323));
#29788=CARTESIAN_POINT('Ctrl Pts',(26.9989399175761,-46.6878020012926,7.3802042952164));
#29789=CARTESIAN_POINT('Ctrl Pts',(19.6629735993418,-37.60670222353,0.));
#29790=CARTESIAN_POINT('Ctrl Pts',(19.8578947412035,-37.5176847207439,2.19648874705824));
#29791=CARTESIAN_POINT('Ctrl Pts',(20.4487150105265,-38.2955653848523,4.17545672685568));
#29792=CARTESIAN_POINT('Ctrl Pts',(21.0395352798495,-39.0734460489607,6.15442470665314));
#29793=CARTESIAN_POINT('Ctrl Pts',(21.9478419990561,-40.5465250662019,7.5239130403414));
#29794=CARTESIAN_POINT('Ctrl Pts',(22.8561487182626,-42.0196040834432,8.89340137402968));
#29795=CARTESIAN_POINT('Ctrl Pts',(23.9406471246595,-43.8784890801692,9.38216610144961));
#29796=CARTESIAN_POINT('Ctrl Pts',(25.0251455310565,-45.7373740768952,9.87093082886955));
#29797=CARTESIAN_POINT('Ctrl Pts',(26.1096439374534,-47.5962590736212,9.3821661014496));
#29798=CARTESIAN_POINT('Ctrl Pts',(18.0362202038888,-35.8811107143584,0.));
#29799=CARTESIAN_POINT('Ctrl Pts',(18.2311413457505,-35.7920932115723,2.70899372698068));
#29800=CARTESIAN_POINT('Ctrl Pts',(18.9143364449663,-36.7722465384541,5.14971273833322));
#29801=CARTESIAN_POINT('Ctrl Pts',(19.5975315441822,-37.7523998653359,7.59043174968576));
#29802=CARTESIAN_POINT('Ctrl Pts',(20.672291955211,-39.58996162655,9.2794617117575));
#29803=CARTESIAN_POINT('Ctrl Pts',(21.7470523662399,-41.4275233877642,10.9684916738292));
#29804=CARTESIAN_POINT('Ctrl Pts',(23.0391151313028,-43.7409109321315,11.5712994880388));
#29805=CARTESIAN_POINT('Ctrl Pts',(24.3311778963657,-46.0542984764988,12.1741073022483));
#29806=CARTESIAN_POINT('Ctrl Pts',(25.6232406614285,-48.367686020866,11.5712994880388));
#29807=CARTESIAN_POINT('Ctrl Pts',(16.7773762111438,-33.8713086176154,0.));
#29808=CARTESIAN_POINT('Ctrl Pts',(16.9722973530055,-33.7822911148293,3.24562220582793));
#29809=CARTESIAN_POINT('Ctrl Pts',(17.752215345444,-34.9742380351174,6.16982677025167));
#29810=CARTESIAN_POINT('Ctrl Pts',(18.5321333378825,-36.1661849554056,9.0940313346754));
#29811=CARTESIAN_POINT('Ctrl Pts',(19.7811823801256,-38.3853855847804,11.1176436806954));
#29812=CARTESIAN_POINT('Ctrl Pts',(21.0302314223687,-40.6045862141552,13.1412560267153));
#29813=CARTESIAN_POINT('Ctrl Pts',(22.5396285557155,-43.3938696431046,13.8634749112255));
#29814=CARTESIAN_POINT('Ctrl Pts',(24.0490256890623,-46.183153072054,14.5856937957357));
#29815=CARTESIAN_POINT('Ctrl Pts',(25.558422822409,-48.9724365010033,13.8634749112255));
#29816=CARTESIAN_POINT('',(16.7773762111438,-33.8713086176154,0.));
#29817=CARTESIAN_POINT('Ctrl Pts',(16.7773762111438,-33.8713086176154,0.));
#29818=CARTESIAN_POINT('Ctrl Pts',(16.9722973530055,-33.7822911148293,3.24562220582793));
#29819=CARTESIAN_POINT('Ctrl Pts',(17.752215345444,-34.9742380351174,6.16982677025167));
#29820=CARTESIAN_POINT('Ctrl Pts',(18.4033205461164,-35.969320654379,8.61106394926976));
#29821=CARTESIAN_POINT('Ctrl Pts',(19.3953958606399,-37.7050538275443,10.4489096280657));
#29822=CARTESIAN_POINT('Origin',(32.0320676419188,-24.3164988679741,0.));
#29823=CARTESIAN_POINT('Ctrl Pts',(16.7773762111438,-33.8713086176154,0.));
#29824=CARTESIAN_POINT('Ctrl Pts',(16.9722973530055,-33.7822911148293,3.24562220582793));
#29825=CARTESIAN_POINT('Ctrl Pts',(17.752215345444,-34.9742380351174,6.16982677025167));
#29826=CARTESIAN_POINT('Ctrl Pts',(18.5321333378825,-36.1661849554056,9.0940313346754));
#29827=CARTESIAN_POINT('Ctrl Pts',(19.7811823801256,-38.3853855847804,11.1176436806954));
#29828=CARTESIAN_POINT('Ctrl Pts',(21.0302314223687,-40.6045862141552,13.1412560267153));
#29829=CARTESIAN_POINT('Ctrl Pts',(22.5396285557155,-43.3938696431046,13.8634749112255));
#29830=CARTESIAN_POINT('Ctrl Pts',(24.0490256890623,-46.183153072054,14.5856937957357));
#29831=CARTESIAN_POINT('Ctrl Pts',(25.5584228224091,-48.9724365010033,13.8634749112255));
#29832=CARTESIAN_POINT('Ctrl Pts',(15.8658665409928,-33.5949933606692,0.));
#29833=CARTESIAN_POINT('Ctrl Pts',(16.0607876828545,-33.5059758578831,3.38941559469373));
#29834=CARTESIAN_POINT('Ctrl Pts',(16.8666232572806,-34.7546743665352,6.44317352589574));
#29835=CARTESIAN_POINT('Ctrl Pts',(17.6724588317067,-36.0033728751874,9.49693145709775));
#29836=CARTESIAN_POINT('Ctrl Pts',(18.968209742954,-38.3248363332023,11.6101975146502));
#29837=CARTESIAN_POINT('Ctrl Pts',(20.2639606542014,-40.6462997912171,13.7234635722027));
#29838=CARTESIAN_POINT('Ctrl Pts',(21.8315940656519,-43.5631028816991,14.4776794959001));
#29839=CARTESIAN_POINT('Ctrl Pts',(23.3992274771025,-46.4799059721811,15.2318954195974));
#29840=CARTESIAN_POINT('Ctrl Pts',(24.966860888553,-49.3967090626631,14.4776794959001));
#29841=CARTESIAN_POINT('Ctrl Pts',(14.9994689250464,-33.990663894172,0.));
#29842=CARTESIAN_POINT('Ctrl Pts',(15.1943900669081,-33.9016463913859,3.38941559469372));
#29843=CARTESIAN_POINT('Ctrl Pts',(16.0002256413342,-35.150344900038,6.44317352589574));
#29844=CARTESIAN_POINT('Ctrl Pts',(16.8060612157603,-36.3990434086902,9.49693145709774));
#29845=CARTESIAN_POINT('Ctrl Pts',(18.1018121270076,-38.7205068667051,11.6101975146502));
#29846=CARTESIAN_POINT('Ctrl Pts',(19.397563038255,-41.04197032472,13.7234635722027));
#29847=CARTESIAN_POINT('Ctrl Pts',(20.9651964497055,-43.9587734152019,14.4776794959001));
#29848=CARTESIAN_POINT('Ctrl Pts',(22.5328298611561,-46.8755765056839,15.2318954195974));
#29849=CARTESIAN_POINT('Ctrl Pts',(24.1004632726066,-49.7923795961659,14.4776794959001));
#29850=CARTESIAN_POINT('Ctrl Pts',(14.6113821712778,-34.8604849513725,0.));
#29851=CARTESIAN_POINT('Ctrl Pts',(14.8063033131395,-34.7714674485864,3.24562220582793));
#29852=CARTESIAN_POINT('Ctrl Pts',(15.586221305578,-35.9634143688745,6.16982677025167));
#29853=CARTESIAN_POINT('Ctrl Pts',(16.3661392980166,-37.1553612891626,9.0940313346754));
#29854=CARTESIAN_POINT('Ctrl Pts',(17.6151883402596,-39.3745619185374,11.1176436806954));
#29855=CARTESIAN_POINT('Ctrl Pts',(18.8642373825027,-41.5937625479123,13.1412560267153));
#29856=CARTESIAN_POINT('Ctrl Pts',(20.3736345158495,-44.3830459768616,13.8634749112255));
#29857=CARTESIAN_POINT('Ctrl Pts',(21.8830316491963,-47.172329405811,14.5856937957357));
#29858=CARTESIAN_POINT('Ctrl Pts',(23.3924287825431,-49.9616128347604,13.8634749112255));
#29859=CARTESIAN_POINT('',(15.5074379107559,-33.9565644529094,1.82251475138647E-29));
#29860=CARTESIAN_POINT('Origin',(16.2551894587634,-35.5938999782226,0.));
#29861=CARTESIAN_POINT('Origin',(16.2551894587634,-35.5938999782226,0.));
#29862=CARTESIAN_POINT('Ctrl Pts',(9.50149509066468,-36.5850719698906,0.));
#29863=CARTESIAN_POINT('Ctrl Pts',(9.7071007278678,-36.5247007077103,3.24562220582793));
#29864=CARTESIAN_POINT('Ctrl Pts',(10.309448546501,-37.8155092299558,6.16982677025168));
#29865=CARTESIAN_POINT('Ctrl Pts',(10.9117963651343,-39.1063177522012,9.09403133467541));
#29866=CARTESIAN_POINT('Ctrl Pts',(11.8323067104418,-41.4806883314343,11.1176436806954));
#29867=CARTESIAN_POINT('Ctrl Pts',(12.7528170557494,-43.8550589106674,13.1412560267153));
#29868=CARTESIAN_POINT('Ctrl Pts',(13.8498942825604,-46.8307610650471,13.8634749112255));
#29869=CARTESIAN_POINT('Ctrl Pts',(14.9469715093714,-49.8064632194268,14.5856937957357));
#29870=CARTESIAN_POINT('Ctrl Pts',(16.0440487361823,-52.7821653738064,13.8634749112255));
#29871=CARTESIAN_POINT('Ctrl Pts',(9.86626475512707,-38.9283465500521,0.));
#29872=CARTESIAN_POINT('Ctrl Pts',(10.0718703923302,-38.8679752878718,2.70899372698069));
#29873=CARTESIAN_POINT('Ctrl Pts',(10.6086211883238,-39.9353808672043,5.14971273833323));
#29874=CARTESIAN_POINT('Ctrl Pts',(11.1453719843174,-41.0027864465368,7.59043174968577));
#29875=CARTESIAN_POINT('Ctrl Pts',(11.9476805791742,-42.9745988326452,9.27946171175751));
#29876=CARTESIAN_POINT('Ctrl Pts',(12.7499891740309,-44.9464112187536,10.9684916738293));
#29877=CARTESIAN_POINT('Ctrl Pts',(13.6996712289061,-47.4201315169975,11.5712994880388));
#29878=CARTESIAN_POINT('Ctrl Pts',(14.6493532837812,-49.8938518152413,12.1741073022483));
#29879=CARTESIAN_POINT('Ctrl Pts',(15.5990353386564,-52.3675721134852,11.5712994880388));
#29880=CARTESIAN_POINT('Ctrl Pts',(9.76686869111994,-41.2977585211121,-1.05434036998093E-14));
#29881=CARTESIAN_POINT('Ctrl Pts',(9.97247432832304,-41.2373872589318,2.19648874705824));
#29882=CARTESIAN_POINT('Ctrl Pts',(10.4465769382884,-42.0914327105682,4.17545672685568));
#29883=CARTESIAN_POINT('Ctrl Pts',(10.9206795482537,-42.9454781622046,6.15442470665314));
#29884=CARTESIAN_POINT('Ctrl Pts',(11.6101000126264,-44.5328288829013,7.5239130403414));
#29885=CARTESIAN_POINT('Ctrl Pts',(12.2995204769991,-46.120179603598,8.89340137402967));
#29886=CARTESIAN_POINT('Ctrl Pts',(13.1084333356587,-48.1144840466621,9.3821661014496));
#29887=CARTESIAN_POINT('Ctrl Pts',(13.9173461943184,-50.1087884897263,9.87093082886953));
#29888=CARTESIAN_POINT('Ctrl Pts',(14.7262590529781,-52.1030929327905,9.3821661014496));
#29889=CARTESIAN_POINT('Ctrl Pts',(9.20712674149411,-43.6022501387952,0.));
#29890=CARTESIAN_POINT('Ctrl Pts',(9.41273237869722,-43.541878876615,1.72780310113342));
#29891=CARTESIAN_POINT('Ctrl Pts',(9.82954324187965,-44.2008065573392,3.28449990511991));
#29892=CARTESIAN_POINT('Ctrl Pts',(10.2463541050621,-44.8597342380635,4.84119670910639));
#29893=CARTESIAN_POINT('Ctrl Pts',(10.8325384089565,-46.0954948844274,5.91846432228298));
#29894=CARTESIAN_POINT('Ctrl Pts',(11.418722712851,-47.3312555307914,6.99573193545957));
#29895=CARTESIAN_POINT('Ctrl Pts',(12.0989021850282,-48.8871343222931,7.38020429521639));
#29896=CARTESIAN_POINT('Ctrl Pts',(12.7790816572054,-50.4430131137949,7.76467665497322));
#29897=CARTESIAN_POINT('Ctrl Pts',(13.4592611293826,-51.9988919052966,7.38020429521639));
#29898=CARTESIAN_POINT('',(9.50149509067387,-36.5850719699046,1.57948920827305E-9));
#29899=CARTESIAN_POINT('Origin',(-8.28430119040681,-39.353726995029,0.));
#29900=CARTESIAN_POINT('Ctrl Pts',(9.50149509087619,-36.5850719699169,3.13105453121543E-9));
#29901=CARTESIAN_POINT('Ctrl Pts',(9.5170179157363,-36.5805140573471,0.245038153335614));
#29902=CARTESIAN_POINT('Ctrl Pts',(9.53446325272375,-36.5819970947818,0.490791160521999));
#29903=CARTESIAN_POINT('Ctrl Pts',(9.5538253279423,-36.58961224761,0.736766500725797));
#29904=CARTESIAN_POINT('Ctrl Pts',(9.57312383855526,-36.5972024003191,0.981934317701467));
#29905=CARTESIAN_POINT('Ctrl Pts',(9.59432652559727,-36.6108845775071,1.22732257376614));
#29906=CARTESIAN_POINT('Ctrl Pts',(9.61741199666741,-36.6307008654467,1.47243294816393));
#29907=CARTESIAN_POINT('Ctrl Pts',(9.64046270023572,-36.6504873093851,1.7171741780307));
#29908=CARTESIAN_POINT('Ctrl Pts',(9.66539050713792,-36.6763894565088,1.9616379154164));
#29909=CARTESIAN_POINT('Ctrl Pts',(9.69215854518704,-36.7083998596962,2.2053240877858));
#29910=CARTESIAN_POINT('Ctrl Pts',(9.71890362559667,-36.7403828091234,2.44880126242122));
#29911=CARTESIAN_POINT('Ctrl Pts',(9.7474857487292,-36.7784635349601,2.69150175431106));
#29912=CARTESIAN_POINT('Ctrl Pts',(9.7778529268264,-36.8225849430253,2.93292951866864));
#29913=CARTESIAN_POINT('Ctrl Pts',(9.80821375204938,-36.8666971208039,3.17430677585648));
#29914=CARTESIAN_POINT('Ctrl Pts',(9.84035883349998,-36.9168473852606,3.41441139318403));
#29915=CARTESIAN_POINT('Ctrl Pts',(9.87422164256022,-36.972929566381,3.65275710614698));
#29916=CARTESIAN_POINT('Ctrl Pts',(9.90812745007443,-37.0290829597591,3.89140546668847));
#29917=CARTESIAN_POINT('Ctrl Pts',(9.94375528237788,-37.0911832213397,4.12829002081221));
#29918=CARTESIAN_POINT('Ctrl Pts',(9.98102464057076,-37.1590759513993,4.36293874377864));
#29919=CARTESIAN_POINT('Ctrl Pts',(10.0183320283712,-37.2270379591175,4.59782690201516));
#29920=CARTESIAN_POINT('Ctrl Pts',(10.0572842076518,-37.3008040750529,4.83047425895038));
#29921=CARTESIAN_POINT('Ctrl Pts',(10.0977878566473,-37.3801738701485,5.06042975959522));
#29922=CARTESIAN_POINT('Ctrl Pts',(10.1384099224354,-37.4597757114128,5.29105755998397));
#29923=CARTESIAN_POINT('Ctrl Pts',(10.1805924445719,-37.5450138125793,5.51897736305782));
#29924=CARTESIAN_POINT('Ctrl Pts',(10.2242300213426,-37.6356433288457,5.74376259354427));
#29925=CARTESIAN_POINT('Ctrl Pts',(10.2520546379007,-37.6934314033808,5.88709234072682));
#29926=CARTESIAN_POINT('Ctrl Pts',(10.280470615574,-37.7534106234276,6.02914825314224));
#29927=CARTESIAN_POINT('Ctrl Pts',(10.3094485465059,-37.8155092299908,6.16982677023484));
#29928=CARTESIAN_POINT('Ctrl Pts',(10.3548867946541,-37.9128816718431,6.39041482339091));
#29929=CARTESIAN_POINT('Ctrl Pts',(10.4021550583216,-38.0159808925391,6.60890054011806));
#29930=CARTESIAN_POINT('Ctrl Pts',(10.4511851399361,-38.124685183118,6.82480412008043));
#29931=CARTESIAN_POINT('Ctrl Pts',(10.5001045333893,-38.2331440676597,7.04022028559294));
#29932=CARTESIAN_POINT('Ctrl Pts',(10.5507777480886,-38.3471826657451,7.25306552029639));
#29933=CARTESIAN_POINT('Ctrl Pts',(10.603121481071,-38.4666322798728,7.4628756626942));
#29934=CARTESIAN_POINT('Ctrl Pts',(10.6553810238844,-38.5858897700798,7.67234834441904));
#29935=CARTESIAN_POINT('Ctrl Pts',(10.7093056453531,-38.7105407473187,7.87879526533069));
#29936=CARTESIAN_POINT('Ctrl Pts',(10.7647978150924,-38.8403712129412,8.08177334612254));
#29937=CARTESIAN_POINT('Ctrl Pts',(10.820236738098,-38.9700771015598,8.28455666214159));
#29938=CARTESIAN_POINT('Ctrl Pts',(10.8772401144471,-39.1049523499265,8.48387739272893));
#29939=CARTESIAN_POINT('Ctrl Pts',(10.935697267249,-39.2447399831766,8.67931873611124));
#29940=CARTESIAN_POINT('Ctrl Pts',(10.9941572316853,-39.384534339842,8.87476947970509));
#29941=CARTESIAN_POINT('Ctrl Pts',(11.0540710087835,-39.5292413095788,9.06634009532832));
#29942=CARTESIAN_POINT('Ctrl Pts',(11.1153159078425,-39.6785635418402,9.25364450340974));
#29943=CARTESIAN_POINT('Ctrl Pts',(11.1765832739882,-39.8279405514888,9.44101762226473));
#29944=CARTESIAN_POINT('Ctrl Pts',(11.2391826206558,-39.9819359159959,9.62412107874997));
#29945=CARTESIAN_POINT('Ctrl Pts',(11.3029807823644,-40.140215636435,9.80260437466077));
#29946=CARTESIAN_POINT('Ctrl Pts',(11.3668830120892,-40.2987535438825,9.98137881379633));
#29947=CARTESIAN_POINT('Ctrl Pts',(11.4319878421544,-40.4615894629181,10.155517727092));
#29948=CARTESIAN_POINT('Ctrl Pts',(11.4981529392408,-40.6283560345708,10.3247095747704));
#29949=CARTESIAN_POINT('Ctrl Pts',(11.5172768919405,-40.6765572187088,10.3736117457736));
#29950=CARTESIAN_POINT('Ctrl Pts',(11.5364893726183,-40.7250865876853,10.4221009095722));
#29951=CARTESIAN_POINT('Ctrl Pts',(11.5557868365676,-40.7739348422894,10.4701702229062));
#29952=CARTESIAN_POINT('Ctrl Pts',(15.8276282594342,-41.6582954965895,0.));
#29953=CARTESIAN_POINT('Ctrl Pts',(16.0332338966373,-41.5979242344092,1.72780310113342));
#29954=CARTESIAN_POINT('Ctrl Pts',(16.4500447598197,-42.2568519151334,3.28449990511991));
#29955=CARTESIAN_POINT('Ctrl Pts',(16.8668556230022,-42.9157795958577,4.84119670910639));
#29956=CARTESIAN_POINT('Ctrl Pts',(17.4530399268966,-44.1515402422216,5.91846432228298));
#29957=CARTESIAN_POINT('Ctrl Pts',(18.039224230791,-45.3873008885856,6.99573193545957));
#29958=CARTESIAN_POINT('Ctrl Pts',(18.7194037029683,-46.9431796800874,7.38020429521639));
#29959=CARTESIAN_POINT('Ctrl Pts',(19.3995831751455,-48.4990584715891,7.76467665497321));
#29960=CARTESIAN_POINT('Ctrl Pts',(20.0797626473227,-50.0549372630909,7.38020429521639));
#29961=CARTESIAN_POINT('Ctrl Pts',(14.1108411348339,-40.0222531270435,-1.05434036998093E-14));
#29962=CARTESIAN_POINT('Ctrl Pts',(14.316446772037,-39.9618818648632,2.19648874705824));
#29963=CARTESIAN_POINT('Ctrl Pts',(14.7905493820023,-40.8159273164997,4.17545672685568));
#29964=CARTESIAN_POINT('Ctrl Pts',(15.2646519919676,-41.669972768136,6.15442470665314));
#29965=CARTESIAN_POINT('Ctrl Pts',(15.9540724563403,-43.2573234888327,7.5239130403414));
#29966=CARTESIAN_POINT('Ctrl Pts',(16.643492920713,-44.8446742095294,8.89340137402968));
#29967=CARTESIAN_POINT('Ctrl Pts',(17.4524057793727,-46.8389786525935,9.38216610144961));
#29968=CARTESIAN_POINT('Ctrl Pts',(18.2613186380324,-48.8332830956577,9.87093082886954));
#29969=CARTESIAN_POINT('Ctrl Pts',(19.070231496692,-50.8275875387219,9.38216610144961));
#29970=CARTESIAN_POINT('Ctrl Pts',(12.7462230199154,-38.0827145049534,0.));
#29971=CARTESIAN_POINT('Ctrl Pts',(12.9518286571185,-38.0223432427732,2.70899372698069));
#29972=CARTESIAN_POINT('Ctrl Pts',(13.4885794531121,-39.0897488221056,5.14971273833323));
#29973=CARTESIAN_POINT('Ctrl Pts',(14.0253302491058,-40.1571544014381,7.59043174968578));
#29974=CARTESIAN_POINT('Ctrl Pts',(14.8276388439625,-42.1289667875466,9.27946171175751));
#29975=CARTESIAN_POINT('Ctrl Pts',(15.6299474388193,-44.1007791736549,10.9684916738292));
#29976=CARTESIAN_POINT('Ctrl Pts',(16.5796294936944,-46.5744994718988,11.5712994880388));
#29977=CARTESIAN_POINT('Ctrl Pts',(17.5293115485696,-49.0482197701427,12.1741073022483));
#29978=CARTESIAN_POINT('Ctrl Pts',(18.4789936034447,-51.5219400683866,11.5712994880388));
#29979=CARTESIAN_POINT('Ctrl Pts',(11.7862169042728,-35.9142171164212,0.));
#29980=CARTESIAN_POINT('Ctrl Pts',(11.9918225414759,-35.8538458542409,3.24562220582792));
#29981=CARTESIAN_POINT('Ctrl Pts',(12.5941703601091,-37.1446543764863,6.16982677025168));
#29982=CARTESIAN_POINT('Ctrl Pts',(13.1965181787423,-38.4354628987318,9.0940313346754));
#29983=CARTESIAN_POINT('Ctrl Pts',(14.1170285240499,-40.8098334779648,11.1176436806954));
#29984=CARTESIAN_POINT('Ctrl Pts',(15.0375388693575,-43.1842040571979,13.1412560267153));
#29985=CARTESIAN_POINT('Ctrl Pts',(16.1346160961685,-46.1599062115776,13.8634749112255));
#29986=CARTESIAN_POINT('Ctrl Pts',(17.2316933229794,-49.1356083659573,14.5856937957357));
#29987=CARTESIAN_POINT('Ctrl Pts',(18.3287705497904,-52.111310520337,13.8634749112255));
#29988=CARTESIAN_POINT('',(11.7862169042728,-35.9142171164212,0.));
#29989=CARTESIAN_POINT('Ctrl Pts',(11.7862169042728,-35.9142171164212,0.));
#29990=CARTESIAN_POINT('Ctrl Pts',(11.9918225414759,-35.8538458542409,3.24562220582792));
#29991=CARTESIAN_POINT('Ctrl Pts',(12.5941703601091,-37.1446543764863,6.16982677025168));
#29992=CARTESIAN_POINT('Ctrl Pts',(13.097033226626,-38.222270420807,8.61106394926975));
#29993=CARTESIAN_POINT('Ctrl Pts',(13.8319900590775,-40.0815233709314,10.4489096280657));
#29994=CARTESIAN_POINT('Origin',(28.2454287759834,-28.6276304970129,0.));
#29995=CARTESIAN_POINT('Ctrl Pts',(11.7862169042728,-35.9142171164212,0.));
#29996=CARTESIAN_POINT('Ctrl Pts',(11.9918225414759,-35.8538458542409,3.24562220582792));
#29997=CARTESIAN_POINT('Ctrl Pts',(12.5941703601091,-37.1446543764863,6.16982677025168));
#29998=CARTESIAN_POINT('Ctrl Pts',(13.1965181787423,-38.4354628987318,9.0940313346754));
#29999=CARTESIAN_POINT('Ctrl Pts',(14.1170285240499,-40.8098334779648,11.1176436806954));
#30000=CARTESIAN_POINT('Ctrl Pts',(15.0375388693575,-43.1842040571979,13.1412560267153));
#30001=CARTESIAN_POINT('Ctrl Pts',(16.1346160961685,-46.1599062115776,13.8634749112255));
#30002=CARTESIAN_POINT('Ctrl Pts',(17.2316933229794,-49.1356083659573,14.5856937957357));
#30003=CARTESIAN_POINT('Ctrl Pts',(18.3287705497904,-52.1113105203369,13.8634749112255));
#30004=CARTESIAN_POINT('Ctrl Pts',(10.9233088493802,-35.5109929990849,0.));
#30005=CARTESIAN_POINT('Ctrl Pts',(11.1289144865834,-35.4506217369046,3.38941559469371));
#30006=CARTESIAN_POINT('Ctrl Pts',(11.7488394904698,-36.8012926546625,6.44317352589574));
#30007=CARTESIAN_POINT('Ctrl Pts',(12.3687644943563,-38.1519635724205,9.49693145709774));
#30008=CARTESIAN_POINT('Ctrl Pts',(13.3209478330609,-40.6342024610833,11.6101975146502));
#30009=CARTESIAN_POINT('Ctrl Pts',(14.2731311717655,-43.1164413497461,13.7234635722027));
#30010=CARTESIAN_POINT('Ctrl Pts',(15.4097039753313,-46.2266530858721,14.4776794959001));
#30011=CARTESIAN_POINT('Ctrl Pts',(16.546276778897,-49.3368648219981,15.2318954195974));
#30012=CARTESIAN_POINT('Ctrl Pts',(17.6828495824628,-52.4470765581242,14.4776794959001));
#30013=CARTESIAN_POINT('Ctrl Pts',(10.009420123937,-35.7793349404727,0.));
#30014=CARTESIAN_POINT('Ctrl Pts',(10.2150257611401,-35.7189636782924,3.38941559469371));
#30015=CARTESIAN_POINT('Ctrl Pts',(10.8349507650266,-37.0696345960503,6.44317352589574));
#30016=CARTESIAN_POINT('Ctrl Pts',(11.4548757689131,-38.4203055138083,9.49693145709774));
#30017=CARTESIAN_POINT('Ctrl Pts',(12.4070591076177,-40.9025444024711,11.6101975146502));
#30018=CARTESIAN_POINT('Ctrl Pts',(13.3592424463223,-43.3847832911339,13.7234635722027));
#30019=CARTESIAN_POINT('Ctrl Pts',(14.4958152498881,-46.4949950272599,14.4776794959001));
#30020=CARTESIAN_POINT('Ctrl Pts',(15.6323880534538,-49.6052067633859,15.2318954195974));
#30021=CARTESIAN_POINT('Ctrl Pts',(16.7689608570196,-52.7154184995119,14.4776794959001));
#30022=CARTESIAN_POINT('Ctrl Pts',(9.50149509066469,-36.5850719698907,0.));
#30023=CARTESIAN_POINT('Ctrl Pts',(9.70710072786781,-36.5247007077104,3.24562220582793));
#30024=CARTESIAN_POINT('Ctrl Pts',(10.309448546501,-37.8155092299558,6.16982677025168));
#30025=CARTESIAN_POINT('Ctrl Pts',(10.9117963651343,-39.1063177522012,9.09403133467541));
#30026=CARTESIAN_POINT('Ctrl Pts',(11.8323067104419,-41.4806883314343,11.1176436806954));
#30027=CARTESIAN_POINT('Ctrl Pts',(12.7528170557494,-43.8550589106674,13.1412560267153));
#30028=CARTESIAN_POINT('Ctrl Pts',(13.8498942825604,-46.8307610650471,13.8634749112255));
#30029=CARTESIAN_POINT('Ctrl Pts',(14.9469715093714,-49.8064632194267,14.5856937957357));
#30030=CARTESIAN_POINT('Ctrl Pts',(16.0440487361824,-52.7821653738064,13.8634749112255));
#30031=CARTESIAN_POINT('',(10.5170715743482,-35.8178741063813,1.72247541091518E-29));
#30032=CARTESIAN_POINT('Origin',(11.0241949492046,-37.5449600575355,0.));
#30033=CARTESIAN_POINT('Origin',(11.0241949492046,-37.5449600575355,0.));
#30034=CARTESIAN_POINT('Ctrl Pts',(4.19818497005484,-37.5648924257372,0.));
#30035=CARTESIAN_POINT('Ctrl Pts',(4.41028956474361,-37.5343963889644,3.24562220582792));
#30036=CARTESIAN_POINT('Ctrl Pts',(4.82280514501186,-38.8977893740386,6.16982677025168));
#30037=CARTESIAN_POINT('Ctrl Pts',(5.23532072528011,-40.2611823591128,9.09403133467541));
#30038=CARTESIAN_POINT('Ctrl Pts',(5.80855343755438,-42.7423875503303,11.1176436806954));
#30039=CARTESIAN_POINT('Ctrl Pts',(6.38178614982864,-45.2235927415478,13.1412560267153));
#30040=CARTESIAN_POINT('Ctrl Pts',(7.0442101414754,-48.325136906711,13.8634749112255));
#30041=CARTESIAN_POINT('Ctrl Pts',(7.70663413312217,-51.4266810718742,14.5856937957357));
#30042=CARTESIAN_POINT('Ctrl Pts',(8.36905812476893,-54.5282252370374,13.8634749112255));
#30043=CARTESIAN_POINT('Ctrl Pts',(4.22575906238186,-39.9362279852005,0.));
#30044=CARTESIAN_POINT('Ctrl Pts',(4.43786365707062,-39.9057319484277,2.7089937269807));
#30045=CARTESIAN_POINT('Ctrl Pts',(4.81724345149705,-41.0386604807592,5.14971273833324));
#30046=CARTESIAN_POINT('Ctrl Pts',(5.19662324592347,-42.1715890130908,7.59043174968579));
#30047=CARTESIAN_POINT('Ctrl Pts',(5.71014733528379,-44.2375116101495,9.27946171175752));
#30048=CARTESIAN_POINT('Ctrl Pts',(6.22367142464412,-46.3034342072083,10.9684916738293));
#30049=CARTESIAN_POINT('Ctrl Pts',(6.81163998135116,-48.8871294476768,11.5712994880388));
#30050=CARTESIAN_POINT('Ctrl Pts',(7.39960853805819,-51.4708246881453,12.1741073022483));
#30051=CARTESIAN_POINT('Ctrl Pts',(7.98757709476522,-54.0545199286138,11.5712994880388));
#30052=CARTESIAN_POINT('Ctrl Pts',(3.79017222552483,-42.2673772240309,0.));
#30053=CARTESIAN_POINT('Ctrl Pts',(4.00227682021359,-42.2368811872581,2.19648874705823));
#30054=CARTESIAN_POINT('Ctrl Pts',(4.35001040888132,-43.1497055238908,4.17545672685568));
#30055=CARTESIAN_POINT('Ctrl Pts',(4.69774399754902,-44.0625298605236,6.15442470665315));
#30056=CARTESIAN_POINT('Ctrl Pts',(5.1542435945577,-45.7318384015438,7.5239130403414));
#30057=CARTESIAN_POINT('Ctrl Pts',(5.61074319156639,-47.401146942564,8.89340137402968));
#30058=CARTESIAN_POINT('Ctrl Pts',(6.12760336939855,-49.4902725446046,9.38216610144961));
#30059=CARTESIAN_POINT('Ctrl Pts',(6.64446354723073,-51.5793981466453,9.87093082886954));
#30060=CARTESIAN_POINT('Ctrl Pts',(7.16132372506291,-53.668523748686,9.38216610144961));
#30061=CARTESIAN_POINT('Ctrl Pts',(2.90816428999222,-44.4687528548128,0.));
#30062=CARTESIAN_POINT('Ctrl Pts',(3.120268884681,-44.43825681804,1.72780310113342));
#30063=CARTESIAN_POINT('Ctrl Pts',(3.43906202795181,-45.149795935654,3.28449990511991));
#30064=CARTESIAN_POINT('Ctrl Pts',(3.75785517122262,-45.8613350532681,4.84119670910638));
#30065=CARTESIAN_POINT('Ctrl Pts',(4.16220588757961,-47.1679401624789,5.91846432228298));
#30066=CARTESIAN_POINT('Ctrl Pts',(4.56655660393661,-48.4745452716896,6.99573193545956));
#30067=CARTESIAN_POINT('Ctrl Pts',(5.01838819123945,-50.1113870920656,7.38020429521639));
#30068=CARTESIAN_POINT('Ctrl Pts',(5.47021977854229,-51.7482289124416,7.76467665497321));
#30069=CARTESIAN_POINT('Ctrl Pts',(5.92205136584512,-53.3850707328175,7.38020429521638));
#30070=CARTESIAN_POINT('',(4.19818497029635,-37.5648924255374,-1.21941740813109E-9));
#30071=CARTESIAN_POINT('Origin',(-13.800598242013,-37.7741838134883,0.));
#30072=CARTESIAN_POINT('Ctrl Pts',(4.19818497005484,-37.5648924257372,0.));
#30073=CARTESIAN_POINT('Ctrl Pts',(4.41028956474361,-37.5343963889644,3.24562220582792));
#30074=CARTESIAN_POINT('Ctrl Pts',(4.82280514501186,-38.8977893740386,6.16982677025168));
#30075=CARTESIAN_POINT('Ctrl Pts',(5.16925602334772,-40.0428338760881,8.6257176219852));
#30076=CARTESIAN_POINT('Ctrl Pts',(5.63542964579419,-42.0034749115208,10.4701702229062));
#30077=CARTESIAN_POINT('Ctrl Pts',(9.73793223897069,-43.4867804707272,0.));
#30078=CARTESIAN_POINT('Ctrl Pts',(9.95003683365946,-43.4562844339544,1.72780310113343));
#30079=CARTESIAN_POINT('Ctrl Pts',(10.2688299769303,-44.1678235515685,3.28449990511991));
#30080=CARTESIAN_POINT('Ctrl Pts',(10.5876231202011,-44.8793626691825,4.84119670910638));
#30081=CARTESIAN_POINT('Ctrl Pts',(10.9919738365581,-46.1859677783933,5.91846432228297));
#30082=CARTESIAN_POINT('Ctrl Pts',(11.3963245529151,-47.4925728876041,6.99573193545955));
#30083=CARTESIAN_POINT('Ctrl Pts',(11.8481561402179,-49.12941470798,7.38020429521639));
#30084=CARTESIAN_POINT('Ctrl Pts',(12.2999877275208,-50.766256528356,7.76467665497321));
#30085=CARTESIAN_POINT('Ctrl Pts',(12.7518193148236,-52.4030983487319,7.38020429521638));
#30086=CARTESIAN_POINT('Ctrl Pts',(8.27145263712638,-41.6230663715378,0.));
#30087=CARTESIAN_POINT('Ctrl Pts',(8.48355723181515,-41.592570334765,2.19648874705824));
#30088=CARTESIAN_POINT('Ctrl Pts',(8.83129082048287,-42.5053946713977,4.17545672685568));
#30089=CARTESIAN_POINT('Ctrl Pts',(9.17902440915059,-43.4182190080305,6.15442470665314));
#30090=CARTESIAN_POINT('Ctrl Pts',(9.63552400615925,-45.0875275490507,7.5239130403414));
#30091=CARTESIAN_POINT('Ctrl Pts',(10.0920236031679,-46.7568360900709,8.89340137402966));
#30092=CARTESIAN_POINT('Ctrl Pts',(10.6088837810001,-48.8459616921115,9.3821661014496));
#30093=CARTESIAN_POINT('Ctrl Pts',(11.1257439588323,-50.9350872941522,9.87093082886954));
#30094=CARTESIAN_POINT('Ctrl Pts',(11.6426041366645,-53.0242128961929,9.3821661014496));
#30095=CARTESIAN_POINT('Ctrl Pts',(7.19674949232852,-39.5090640497074,0.));
#30096=CARTESIAN_POINT('Ctrl Pts',(7.40885408701727,-39.4785680129346,2.7089937269807));
#30097=CARTESIAN_POINT('Ctrl Pts',(7.7882338814437,-40.6114965452661,5.14971273833323));
#30098=CARTESIAN_POINT('Ctrl Pts',(8.16761367587013,-41.7444250775977,7.59043174968578));
#30099=CARTESIAN_POINT('Ctrl Pts',(8.68113776523044,-43.8103476746565,9.27946171175752));
#30100=CARTESIAN_POINT('Ctrl Pts',(9.19466185459077,-45.8762702717153,10.9684916738293));
#30101=CARTESIAN_POINT('Ctrl Pts',(9.78263041129781,-48.4599655121837,11.5712994880388));
#30102=CARTESIAN_POINT('Ctrl Pts',(10.3705989680048,-51.0436607526522,12.1741073022483));
#30103=CARTESIAN_POINT('Ctrl Pts',(10.9585675247119,-53.6273559931207,11.5712994880388));
#30104=CARTESIAN_POINT('Ctrl Pts',(6.55512420987355,-37.2260157227863,0.));
#30105=CARTESIAN_POINT('Ctrl Pts',(6.76722880456232,-37.1955196860135,3.24562220582793));
#30106=CARTESIAN_POINT('Ctrl Pts',(7.17974438483057,-38.5589126710877,6.16982677025168));
#30107=CARTESIAN_POINT('Ctrl Pts',(7.59225996509882,-39.922305656162,9.09403133467541));
#30108=CARTESIAN_POINT('Ctrl Pts',(8.16549267737308,-42.4035108473794,11.1176436806954));
#30109=CARTESIAN_POINT('Ctrl Pts',(8.73872538964735,-44.8847160385969,13.1412560267153));
#30110=CARTESIAN_POINT('Ctrl Pts',(9.4011493812941,-47.9862602037601,13.8634749112255));
#30111=CARTESIAN_POINT('Ctrl Pts',(10.0635733729409,-51.0878043689233,14.5856937957357));
#30112=CARTESIAN_POINT('Ctrl Pts',(10.7259973645876,-54.1893485340865,13.8634749112255));
#30113=CARTESIAN_POINT('',(6.55512420987355,-37.2260157227863,0.));
#30114=CARTESIAN_POINT('Ctrl Pts',(6.55512420987355,-37.2260157227863,0.));
#30115=CARTESIAN_POINT('Ctrl Pts',(6.76722880456232,-37.1955196860135,3.24562220582793));
#30116=CARTESIAN_POINT('Ctrl Pts',(7.17974438483056,-38.5589126710877,6.16982677025168));
#30117=CARTESIAN_POINT('Ctrl Pts',(7.52412807936649,-39.6971249853933,8.61106394926976));
#30118=CARTESIAN_POINT('Ctrl Pts',(7.98700482807783,-41.6420486840549,10.4489096280657));
#30119=CARTESIAN_POINT('Origin',(23.8837944332593,-32.3559861244015,0.));
#30120=CARTESIAN_POINT('Ctrl Pts',(6.55512420987355,-37.2260157227863,0.));
#30121=CARTESIAN_POINT('Ctrl Pts',(6.76722880456232,-37.1955196860135,3.24562220582793));
#30122=CARTESIAN_POINT('Ctrl Pts',(7.17974438483056,-38.5589126710877,6.16982677025168));
#30123=CARTESIAN_POINT('Ctrl Pts',(7.59225996509882,-39.922305656162,9.09403133467541));
#30124=CARTESIAN_POINT('Ctrl Pts',(8.16549267737308,-42.4035108473794,11.1176436806954));
#30125=CARTESIAN_POINT('Ctrl Pts',(8.73872538964735,-44.8847160385969,13.1412560267153));
#30126=CARTESIAN_POINT('Ctrl Pts',(9.4011493812941,-47.9862602037601,13.8634749112255));
#30127=CARTESIAN_POINT('Ctrl Pts',(10.0635733729409,-51.0878043689233,14.5856937957357));
#30128=CARTESIAN_POINT('Ctrl Pts',(10.7259973645876,-54.1893485340865,13.8634749112255));
#30129=CARTESIAN_POINT('Ctrl Pts',(5.75838408981577,-36.7040912252866,0.));
#30130=CARTESIAN_POINT('Ctrl Pts',(5.97048868450455,-36.6735951885137,3.38941559469373));
#30131=CARTESIAN_POINT('Ctrl Pts',(6.39188323248834,-38.0987427505053,6.44317352589574));
#30132=CARTESIAN_POINT('Ctrl Pts',(6.81327778047213,-39.5238903124967,9.49693145709775));
#30133=CARTESIAN_POINT('Ctrl Pts',(7.40250983972804,-42.1163734062201,11.6101975146502));
#30134=CARTESIAN_POINT('Ctrl Pts',(7.99174189898394,-44.7088564999435,13.7234635722027));
#30135=CARTESIAN_POINT('Ctrl Pts',(8.6741167499896,-47.9491619398761,14.4776794959001));
#30136=CARTESIAN_POINT('Ctrl Pts',(9.35649160099525,-51.1894673798086,15.2318954195974));
#30137=CARTESIAN_POINT('Ctrl Pts',(10.0388664520009,-54.4297728197412,14.4776794959001));
#30138=CARTESIAN_POINT('Ctrl Pts',(4.81560839388829,-36.839641906467,0.));
#30139=CARTESIAN_POINT('Ctrl Pts',(5.02771298857707,-36.8091458696941,3.38941559469373));
#30140=CARTESIAN_POINT('Ctrl Pts',(5.44910753656085,-38.2342934316856,6.44317352589574));
#30141=CARTESIAN_POINT('Ctrl Pts',(5.87050208454464,-39.6594409936771,9.49693145709774));
#30142=CARTESIAN_POINT('Ctrl Pts',(6.45973414380055,-42.2519240874005,11.6101975146502));
#30143=CARTESIAN_POINT('Ctrl Pts',(7.04896620305647,-44.8444071811239,13.7234635722027));
#30144=CARTESIAN_POINT('Ctrl Pts',(7.73134105406212,-48.0847126210564,14.4776794959001));
#30145=CARTESIAN_POINT('Ctrl Pts',(8.41371590506776,-51.3250180609889,15.2318954195974));
#30146=CARTESIAN_POINT('Ctrl Pts',(9.09609075607344,-54.5653235009215,14.4776794959001));
#30147=CARTESIAN_POINT('Ctrl Pts',(4.19818497005484,-37.5648924257372,0.));
#30148=CARTESIAN_POINT('Ctrl Pts',(4.41028956474361,-37.5343963889644,3.24562220582792));
#30149=CARTESIAN_POINT('Ctrl Pts',(4.82280514501185,-38.8977893740386,6.16982677025168));
#30150=CARTESIAN_POINT('Ctrl Pts',(5.23532072528011,-40.2611823591128,9.09403133467541));
#30151=CARTESIAN_POINT('Ctrl Pts',(5.80855343755438,-42.7423875503303,11.1176436806954));
#30152=CARTESIAN_POINT('Ctrl Pts',(6.38178614982865,-45.2235927415478,13.1412560267153));
#30153=CARTESIAN_POINT('Ctrl Pts',(7.0442101414754,-48.325136906711,13.8634749112255));
#30154=CARTESIAN_POINT('Ctrl Pts',(7.70663413312217,-51.4266810718742,14.5856937957357));
#30155=CARTESIAN_POINT('Ctrl Pts',(8.36905812476893,-54.5282252370374,13.8634749112255));
#30156=CARTESIAN_POINT('',(5.31260798926534,-36.9500351333113,1.04083408558609E-14));
#30157=CARTESIAN_POINT('Origin',(5.56877962163311,-38.731713020801,1.04083408558608E-14));
#30158=CARTESIAN_POINT('Origin',(5.56877962163311,-38.731713020801,1.04083408558608E-14));
#30159=CARTESIAN_POINT('Ctrl Pts',(-4.33370633274479,-37.6057474666452,
1.59647061166203));
#30160=CARTESIAN_POINT('Ctrl Pts',(-4.29042532205908,-37.58837141962,1.1525915890158));
#30161=CARTESIAN_POINT('Ctrl Pts',(-4.24082283094062,-37.5585354835099,
0.635572970286848));
#30162=CARTESIAN_POINT('Ctrl Pts',(-4.0728295363398,-37.5835818541808,-1.86858636184043));
#30163=CARTESIAN_POINT('Ctrl Pts',(-4.00528018448063,-37.9619119569937,
-3.71029995868706));
#30164=CARTESIAN_POINT('Ctrl Pts',(-3.95610755721523,-39.4161093304728,
-7.16936247494803));
#30165=CARTESIAN_POINT('Ctrl Pts',(-3.98510500544276,-40.4714275735321,
-8.73699595771102));
#30166=CARTESIAN_POINT('Ctrl Pts',(-4.11161181537858,-43.1170704486883,
-11.3730256982087));
#30167=CARTESIAN_POINT('Ctrl Pts',(-4.21430601439535,-44.6849606627836,
-12.423580519233));
#30168=CARTESIAN_POINT('Ctrl Pts',(-4.45373622019712,-48.1464351665928,
-13.8529470821493));
#30169=CARTESIAN_POINT('Ctrl Pts',(-4.59667050421776,-49.9934079386698,
-14.2204718556168));
#30170=CARTESIAN_POINT('Ctrl Pts',(-4.73676521641172,-51.8536466863969,
-14.2198708430667));
#30171=CARTESIAN_POINT('Ctrl Pts',(-4.95142919224136,-36.8815114147053,
1.62964605326969));
#30172=CARTESIAN_POINT('Ctrl Pts',(-4.90850926387041,-36.8642803315616,
1.18947019887277));
#30173=CARTESIAN_POINT('Ctrl Pts',(-4.85838298962999,-36.8334013785574,
0.664243925048727));
#30174=CARTESIAN_POINT('Ctrl Pts',(-4.6898509593033,-36.8579890764814,-1.95287905135618));
#30175=CARTESIAN_POINT('Ctrl Pts',(-4.62539547708617,-37.2526110659569,
-3.87337387077168));
#30176=CARTESIAN_POINT('Ctrl Pts',(-4.58435548150261,-38.7695270469137,
-7.48792130215392));
#30177=CARTESIAN_POINT('Ctrl Pts',(-4.62052713520802,-39.8706950784986,
-9.12360836232429));
#30178=CARTESIAN_POINT('Ctrl Pts',(-4.76347923308091,-42.6325290552054,
-11.8774049927068));
#30179=CARTESIAN_POINT('Ctrl Pts',(-4.87652118893798,-44.2683416970719,
-12.9732563608828));
#30180=CARTESIAN_POINT('Ctrl Pts',(-5.13710478159844,-47.8830959478653,
-14.467685804552));
#30181=CARTESIAN_POINT('Ctrl Pts',(-5.29206142837077,-49.8087293766692,
-14.8501851004961));
#30182=CARTESIAN_POINT('Ctrl Pts',(-5.44377846349937,-51.7519872491302,
-14.8499483202528));
#30183=CARTESIAN_POINT('Ctrl Pts',(-5.89423842867615,-36.7461942621623,
1.62975523620947));
#30184=CARTESIAN_POINT('Ctrl Pts',(-5.85132433672737,-36.7289655221682,
1.18963923865732));
#30185=CARTESIAN_POINT('Ctrl Pts',(-5.8011842412917,-36.6980284414522,0.664246367120141));
#30186=CARTESIAN_POINT('Ctrl Pts',(-5.63255152129859,-36.7219158272082,
-1.95288623105315));
#30187=CARTESIAN_POINT('Ctrl Pts',(-5.56825045708737,-37.1176115175603,
-3.8731703451746));
#30188=CARTESIAN_POINT('Ctrl Pts',(-5.52703808205162,-38.6333292122955,
-7.48823335805512));
#30189=CARTESIAN_POINT('Ctrl Pts',(-5.56331547728646,-39.7352322893832,
-9.12349227714319));
#30190=CARTESIAN_POINT('Ctrl Pts',(-5.706229372011,-42.4968007058835,-11.877576477626));
#30191=CARTESIAN_POINT('Ctrl Pts',(-5.81933389107478,-44.1330482236679,
-12.9726927515199));
#30192=CARTESIAN_POINT('Ctrl Pts',(-6.0798476762211,-47.7473173225431,-14.4683433355162));
#30193=CARTESIAN_POINT('Ctrl Pts',(-6.23484434202101,-49.6732762742138,
-14.8498038985338));
#30194=CARTESIAN_POINT('Ctrl Pts',(-6.38655415380882,-51.6164365682428,
-14.8500516281495));
#30195=CARTESIAN_POINT('Ctrl Pts',(-6.69072942383177,-37.2674545852877,
1.59674356901149));
#30196=CARTESIAN_POINT('Ctrl Pts',(-6.64746300420088,-37.2500843961327,
1.1530141884774));
#30197=CARTESIAN_POINT('Ctrl Pts',(-6.5978259600943,-37.2201031407487,0.635579075465374));
#30198=CARTESIAN_POINT('Ctrl Pts',(-6.42958094132981,-37.2433987309931,
-1.86860431108287));
#30199=CARTESIAN_POINT('Ctrl Pts',(-6.36241763448362,-37.6244130859999,
-3.70979114469557));
#30200=CARTESIAN_POINT('Ctrl Pts',(-6.31281405858778,-39.0756147439297,
-7.17014261469985));
#30201=CARTESIAN_POINT('Ctrl Pts',(-6.34207586063706,-40.1327706007388,
-8.73670574475346));
#30202=CARTESIAN_POINT('Ctrl Pts',(-6.4684871627056,-42.7777495753881,-11.3734544105114));
#30203=CARTESIAN_POINT('Ctrl Pts',(-6.57133776973947,-44.3467269792784,
-12.4221714958233));
#30204=CARTESIAN_POINT('Ctrl Pts',(-6.81059345675164,-47.8069886032824,
-13.8545909095622));
#30205=CARTESIAN_POINT('Ctrl Pts',(-6.95362708074765,-49.6547753637202,
-14.2195188100007));
#30206=CARTESIAN_POINT('Ctrl Pts',(-7.09370444218534,-51.5147699841784,
-14.2201291128083));
#30207=CARTESIAN_POINT('Ctrl Pts',(-4.19818497005538,-37.5648924257372,
0.));
#30208=CARTESIAN_POINT('Ctrl Pts',(-4.0728295363398,-37.5835818541808,-1.86858636184043));
#30209=CARTESIAN_POINT('Ctrl Pts',(-4.00528018448063,-37.9619119569937,
-3.71029995868706));
#30210=CARTESIAN_POINT('Ctrl Pts',(-3.95610755721523,-39.4161093304728,
-7.16936247494803));
#30211=CARTESIAN_POINT('Ctrl Pts',(-3.98510500544276,-40.4714275735321,
-8.73699595771102));
#30212=CARTESIAN_POINT('Ctrl Pts',(-4.05479285274714,-41.9288128067802,
-10.1890856763498));
#30213=CARTESIAN_POINT('Ctrl Pts',(-4.06163542615445,-42.0659125600699,
-10.3203928635166));
#30214=CARTESIAN_POINT('Ctrl Pts',(-4.06886253049728,-42.2054617208604,
-10.4488603765996));
#30215=CARTESIAN_POINT('Ctrl Pts',(-6.55512420987408,-37.2260157227862,
1.16573417585641E-15));
#30216=CARTESIAN_POINT('Ctrl Pts',(-6.42958094132981,-37.2433987309931,
-1.86860431108287));
#30217=CARTESIAN_POINT('Ctrl Pts',(-6.36241763448362,-37.6244130859999,
-3.70979114469557));
#30218=CARTESIAN_POINT('Ctrl Pts',(-6.31281405858778,-39.0756147439297,
-7.17014261469985));
#30219=CARTESIAN_POINT('Ctrl Pts',(-6.34207586063706,-40.1327706007388,
-8.73670574475346));
#30220=CARTESIAN_POINT('Ctrl Pts',(-6.41206653251623,-41.5972271209447,
-10.1966053555719));
#30221=CARTESIAN_POINT('Ctrl Pts',(-6.4193084084792,-41.7420345975441,-10.3350231942278));
#30222=CARTESIAN_POINT('Ctrl Pts',(-6.4269788511404,-41.8895769551535,-10.4702558451001));
#30223=CARTESIAN_POINT('Ctrl Pts',(-3.0407109084869,-44.5001944306519,1.24689076028081));
#30224=CARTESIAN_POINT('Ctrl Pts',(-2.99365083345024,-44.4813012009514,
0.764254616149155));
#30225=CARTESIAN_POINT('Ctrl Pts',(-2.94950053245697,-44.4621525981,0.332948654549386));
#30226=CARTESIAN_POINT('Ctrl Pts',(-2.78663561818149,-44.4881576285441,
-0.978870002610901));
#30227=CARTESIAN_POINT('Ctrl Pts',(-2.68728492515961,-44.7004709588365,
-1.98783577089445));
#30228=CARTESIAN_POINT('Ctrl Pts',(-2.55131209325869,-45.4859946801644,
-3.80852727283077));
#30229=CARTESIAN_POINT('Ctrl Pts',(-2.50516810165338,-46.0614183982294,
-4.65544360721816));
#30230=CARTESIAN_POINT('Ctrl Pts',(-2.45787394353332,-47.4791272455671,
-6.04997283343549));
#30231=CARTESIAN_POINT('Ctrl Pts',(-2.45168870249929,-48.3324696724382,
-6.61832169902995));
#30232=CARTESIAN_POINT('Ctrl Pts',(-2.46744610983318,-50.1733013631149,
-7.36768403078693));
#30233=CARTESIAN_POINT('Ctrl Pts',(-2.4837595942785,-51.1917533012822,-7.5713864867327));
#30234=CARTESIAN_POINT('Ctrl Pts',(-2.50107414862773,-52.1751568070597,
-7.56962581969452));
#30235=CARTESIAN_POINT('Ctrl Pts',(-3.92365461890846,-42.3018453782487,
1.354893140661));
#30236=CARTESIAN_POINT('Ctrl Pts',(-3.8777644710901,-42.2834218397599,0.884255472099668));
#30237=CARTESIAN_POINT('Ctrl Pts',(-3.83192350390373,-42.2609432865998,
0.426396927819385));
#30238=CARTESIAN_POINT('Ctrl Pts',(-3.66742334693191,-42.2862930185953,
-1.25360819497148));
#30239=CARTESIAN_POINT('Ctrl Pts',(-3.57797177381454,-42.5504213117472,
-2.51960912779949));
#30240=CARTESIAN_POINT('Ctrl Pts',(-3.46871344469187,-43.5418092681725,
-4.84647586782144));
#30241=CARTESIAN_POINT('Ctrl Pts',(-3.44582654101365,-44.2657961681601,
-5.91572199046669));
#30242=CARTESIAN_POINT('Ctrl Pts',(-3.4521805883684,-46.0625411381476,-7.69376028692055));
#30243=CARTESIAN_POINT('Ctrl Pts',(-3.47964820282461,-47.136751069223,-8.41063186557174));
#30244=CARTESIAN_POINT('Ctrl Pts',(-3.56443746807183,-49.4777703293325,
-9.37059840619463));
#30245=CARTESIAN_POINT('Ctrl Pts',(-3.61985039974772,-50.7522326212068,
-9.62435378618528));
#30246=CARTESIAN_POINT('Ctrl Pts',(-3.67509457152176,-52.0063376889004,
-9.62320046360557));
#30247=CARTESIAN_POINT('Ctrl Pts',(-4.36024590432551,-39.9738746787523,
1.4729318543386));
#30248=CARTESIAN_POINT('Ctrl Pts',(-4.31563179084644,-39.9559634303431,
1.01538086897134));
#30249=CARTESIAN_POINT('Ctrl Pts',(-4.26794984367694,-39.9298762050481,
0.528580691603471));
#30250=CARTESIAN_POINT('Ctrl Pts',(-4.10171804395032,-39.9549022371289,
-1.55402875458448));
#30251=CARTESIAN_POINT('Ctrl Pts',(-4.0230044735796,-40.2750875547349,-3.10121432123278));
#30252=CARTESIAN_POINT('Ctrl Pts',(-3.9430549975307,-41.4922590552058,-5.98129145451134));
#30253=CARTESIAN_POINT('Ctrl Pts',(-3.94554026237701,-42.3782865653845,
-7.29389406576502));
#30254=CARTESIAN_POINT('Ctrl Pts',(-4.01057973632053,-44.5896542676493,
-9.49113593804167));
#30255=CARTESIAN_POINT('Ctrl Pts',(-4.0748114520217,-45.9051375482353,-10.3708286017178));
#30256=CARTESIAN_POINT('Ctrl Pts',(-4.23512580634915,-48.7933811184272,
-11.5604045561244));
#30257=CARTESIAN_POINT('Ctrl Pts',(-4.3332969012096,-50.3476002080508,-11.8694761541095));
#30258=CARTESIAN_POINT('Ctrl Pts',(-4.42999533819651,-51.8977769668582,
-11.8687142284813));
#30259=CARTESIAN_POINT('Ctrl Pts',(-4.33370633274479,-37.6057474666452,
1.59647061166203));
#30260=CARTESIAN_POINT('Ctrl Pts',(-4.29042532205909,-37.58837141962,1.15259158901579));
#30261=CARTESIAN_POINT('Ctrl Pts',(-4.24082283094062,-37.5585354835099,
0.635572970286848));
#30262=CARTESIAN_POINT('Ctrl Pts',(-4.0728295363398,-37.5835818541808,-1.86858636184043));
#30263=CARTESIAN_POINT('Ctrl Pts',(-4.00528018448063,-37.9619119569937,
-3.71029995868706));
#30264=CARTESIAN_POINT('Ctrl Pts',(-3.95610755721523,-39.4161093304728,
-7.16936247494803));
#30265=CARTESIAN_POINT('Ctrl Pts',(-3.98510500544276,-40.4714275735321,
-8.73699595771102));
#30266=CARTESIAN_POINT('Ctrl Pts',(-4.11161181537858,-43.1170704486883,
-11.3730256982087));
#30267=CARTESIAN_POINT('Ctrl Pts',(-4.21430601439535,-44.6849606627836,
-12.423580519233));
#30268=CARTESIAN_POINT('Ctrl Pts',(-4.45373622019711,-48.1464351665928,
-13.8529470821493));
#30269=CARTESIAN_POINT('Ctrl Pts',(-4.59667050421633,-49.9934079386698,
-14.2204718556168));
#30270=CARTESIAN_POINT('Ctrl Pts',(-4.73676521641171,-51.8536466863969,
-14.2198708430667));
#30271=CARTESIAN_POINT('Ctrl Pts',(-6.69072942383177,-37.2674545852877,
1.59674356901149));
#30272=CARTESIAN_POINT('Ctrl Pts',(-6.64746300420088,-37.2500843961327,
1.1530141884774));
#30273=CARTESIAN_POINT('Ctrl Pts',(-6.5978259600943,-37.2201031407487,0.635579075465374));
#30274=CARTESIAN_POINT('Ctrl Pts',(-6.42958094132981,-37.2433987309931,
-1.86860431108287));
#30275=CARTESIAN_POINT('Ctrl Pts',(-6.36241763448362,-37.6244130859999,
-3.70979114469557));
#30276=CARTESIAN_POINT('Ctrl Pts',(-6.31281405858778,-39.0756147439297,
-7.17014261469985));
#30277=CARTESIAN_POINT('Ctrl Pts',(-6.34207586063706,-40.1327706007388,
-8.73670574475346));
#30278=CARTESIAN_POINT('Ctrl Pts',(-6.4684871627056,-42.7777495753881,-11.3734544105114));
#30279=CARTESIAN_POINT('Ctrl Pts',(-6.57133776973947,-44.3467269792784,
-12.4221714958233));
#30280=CARTESIAN_POINT('Ctrl Pts',(-6.81059345675164,-47.8069886032824,
-13.8545909095622));
#30281=CARTESIAN_POINT('Ctrl Pts',(-6.95362708074765,-49.6547753637202,
-14.2195188100007));
#30282=CARTESIAN_POINT('Ctrl Pts',(-7.09370444218534,-51.5147699841784,
-14.2201291128083));
#30283=CARTESIAN_POINT('Ctrl Pts',(-7.33134203123344,-39.5474466673499,
1.4732759250127));
#30284=CARTESIAN_POINT('Ctrl Pts',(-7.28674631020376,-39.5295428029629,
1.01591356787765));
#30285=CARTESIAN_POINT('Ctrl Pts',(-7.2390208079874,-39.5032723984918,0.528588387358482));
#30286=CARTESIAN_POINT('Ctrl Pts',(-7.07247170263556,-39.5260915209495,
-1.55405138012636));
#30287=CARTESIAN_POINT('Ctrl Pts',(-6.99424475322478,-39.8496604164817,
-3.10057294640376));
#30288=CARTESIAN_POINT('Ctrl Pts',(-6.91375205390094,-41.0630557304083,
-5.98227484334893));
#30289=CARTESIAN_POINT('Ctrl Pts',(-6.91657054442394,-41.9513996061453,
-7.29352824389797));
#30290=CARTESIAN_POINT('Ctrl Pts',(-6.98148962792371,-44.161930442516,-9.4916763423596));
#30291=CARTESIAN_POINT('Ctrl Pts',(-7.04591850047786,-45.4787841574446,
-10.3690524867544));
#30292=CARTESIAN_POINT('Ctrl Pts',(-7.20601286879719,-48.3654988573867,
-11.5624766483598));
#30293=CARTESIAN_POINT('Ctrl Pts',(-7.30430498990994,-49.9207450076481,
-11.8682745705925));
#30294=CARTESIAN_POINT('Ctrl Pts',(-7.40098575043892,-51.4706130322883,
-11.8690397849987));
#30295=CARTESIAN_POINT('Ctrl Pts',(-8.40509445805894,-41.6586445536368,
1.35541211815635));
#30296=CARTESIAN_POINT('Ctrl Pts',(-8.35923205241047,-41.6402321527941,
0.885058966163931));
#30297=CARTESIAN_POINT('Ctrl Pts',(-8.31332538916123,-41.6174773021374,
0.426408535677771));
#30298=CARTESIAN_POINT('Ctrl Pts',(-8.14834662563531,-41.6394982516602,
-1.25364232210855));
#30299=CARTESIAN_POINT('Ctrl Pts',(-8.05962904511716,-41.9087301497685,
-2.51864171288232));
#30300=CARTESIAN_POINT('Ctrl Pts',(-7.94955134754164,-42.8944223117487,
-4.8479591580715));
#30301=CARTESIAN_POINT('Ctrl Pts',(-7.92716706335529,-43.6219030915812,
-5.91517020465636));
#30302=CARTESIAN_POINT('Ctrl Pts',(-7.93333952031304,-45.4173857785723,
-7.69457540340655));
#30303=CARTESIAN_POINT('Ctrl Pts',(-7.96110451544491,-46.4936627982893,
-8.40795287033041));
#30304=CARTESIAN_POINT('Ctrl Pts',(-8.04556196575892,-48.8323759936388,
-9.37372383745879));
#30305=CARTESIAN_POINT('Ctrl Pts',(-8.10114839964434,-50.1083893187776,
-9.62254086009649));
#30306=CARTESIAN_POINT('Ctrl Pts',(-8.15637495641919,-51.3620268377999,
-9.62369151535369));
#30307=CARTESIAN_POINT('Ctrl Pts',(-9.87072183560191,-43.5199138025265,
1.2476817163332));
#30308=CARTESIAN_POINT('Ctrl Pts',(-9.82370404146966,-43.5010375473475,
0.765479194283311));
#30309=CARTESIAN_POINT('Ctrl Pts',(-9.77945361532658,-43.4814678488086,
0.332966345693859));
#30310=CARTESIAN_POINT('Ctrl Pts',(-9.61585927298705,-43.5023995944572,
-0.978922014626564));
#30311=CARTESIAN_POINT('Ctrl Pts',(-9.51762723326553,-43.7224911564908,
-1.98636136653616));
#30312=CARTESIAN_POINT('Ctrl Pts',(-9.38040562961129,-44.4993341100839,
-3.81078790534053));
#30313=CARTESIAN_POINT('Ctrl Pts',(-9.33502766337921,-45.0800827322847,
-4.654602649119));
#30314=CARTESIAN_POINT('Ctrl Pts',(-9.28745674947336,-46.4958677767967,
-6.05121512491338));
#30315=CARTESIAN_POINT('Ctrl Pts',(-9.28172473627183,-47.3523605835685,
-6.61423873297828));
#30316=CARTESIAN_POINT('Ctrl Pts',(-9.29697643568735,-49.1896776789186,
-7.37244739488559));
#30317=CARTESIAN_POINT('Ctrl Pts',(-9.31353425505142,-50.2104967200013,
-7.56862230187139));
#30318=CARTESIAN_POINT('Ctrl Pts',(-9.33084205690732,-51.1931844250964,
-7.57037421505981));
#30319=CARTESIAN_POINT('Ctrl Pts',(-9.64145132693333,-36.6062244663075,
1.59647068126627));
#30320=CARTESIAN_POINT('Ctrl Pts',(-9.59613798295645,-36.5951848118862,
1.15259163659385));
#30321=CARTESIAN_POINT('Ctrl Pts',(-9.54279427444346,-36.5727117312865,
0.635573001860467));
#30322=CARTESIAN_POINT('Ctrl Pts',(-9.38007537753151,-36.6214111051535,
-1.86858636179946));
#30323=CARTESIAN_POINT('Ctrl Pts',(-9.36705556804196,-37.0055036281524,
-3.71029995871102));
#30324=CARTESIAN_POINT('Ctrl Pts',(-9.52533731124922,-38.4518973636108,
-7.1693624749242));
#30325=CARTESIAN_POINT('Ctrl Pts',(-9.70422705227032,-39.4923472214852,
-8.73699595767225));
#30326=CARTESIAN_POINT('Ctrl Pts',(-10.2059604433558,-42.0930574706308,
-11.3730256982475));
#30327=CARTESIAN_POINT('Ctrl Pts',(-10.5307434056497,-43.6303739147856,
-12.4235805192274));
#30328=CARTESIAN_POINT('Ctrl Pts',(-11.2603557414205,-47.0225411281053,
-13.8529470821549));
#30329=CARTESIAN_POINT('Ctrl Pts',(-11.6646867919259,-48.8303727109964,
-14.2204718556692));
#30330=CARTESIAN_POINT('Ctrl Pts',(-12.0680951184148,-50.6517393542017,
-14.2198708430667));
#30331=CARTESIAN_POINT('Ctrl Pts',(-10.1498171217995,-35.8014489642672,
1.62964612287391));
#30332=CARTESIAN_POINT('Ctrl Pts',(-10.1048818153719,-35.7905014108337,
1.18947024664515));
#30333=CARTESIAN_POINT('Ctrl Pts',(-10.0508712182972,-35.7670704718592,
0.664243958044528));
#30334=CARTESIAN_POINT('Ctrl Pts',(-9.88755379327951,-35.8153925117011,
-1.95287905130714));
#30335=CARTESIAN_POINT('Ctrl Pts',(-9.87991493950544,-36.2151707898814,
-3.87337387079805));
#30336=CARTESIAN_POINT('Ctrl Pts',(-10.0551723244117,-37.7224873536628,
-7.48792130212771));
#30337=CARTESIAN_POINT('Ctrl Pts',(-10.2476883530651,-38.8072993194331,
-9.12360836229508));
#30338=CARTESIAN_POINT('Ctrl Pts',(-10.7822353606272,-41.5206776037571,
-11.8774049927361));
#30339=CARTESIAN_POINT('Ctrl Pts',(-11.1269271238186,-43.1237524839686,
-12.9732563608868));
#30340=CARTESIAN_POINT('Ctrl Pts',(-11.8992915178841,-46.6646288366181,
-14.467685804548));
#30341=CARTESIAN_POINT('Ctrl Pts',(-12.3267171394702,-48.5486094635654,
-14.8501851005342));
#30342=CARTESIAN_POINT('Ctrl Pts',(-12.7534443437025,-50.4504961875092,
-14.8499483202528));
#30343=CARTESIAN_POINT('Ctrl Pts',(-11.0637722809463,-35.5333334012202,
1.6297553058137));
#30344=CARTESIAN_POINT('Ctrl Pts',(-11.0188430850024,-35.5223873364666,
1.18963928643661));
#30345=CARTESIAN_POINT('Ctrl Pts',(-10.9648105349745,-35.4989008284127,
0.664246400116173));
#30346=CARTESIAN_POINT('Ctrl Pts',(-10.8012937803563,-35.5465440138953,
-1.95288623100444));
#30347=CARTESIAN_POINT('Ctrl Pts',(-10.7939605763972,-35.9473630882332,
-3.87317034520098));
#30348=CARTESIAN_POINT('Ctrl Pts',(-10.9688768025169,-37.4535180947868,
-7.48823335802893));
#30349=CARTESIAN_POINT('Ctrl Pts',(-11.1616021042806,-38.539042575736,-9.12349227712832));
#30350=CARTESIAN_POINT('Ctrl Pts',(-11.6960735043977,-41.252163439798,-11.8775764776409));
#30351=CARTESIAN_POINT('Ctrl Pts',(-12.0408890832862,-42.8556598658169,
-12.9726927515287));
#30352=CARTESIAN_POINT('Ctrl Pts',(-12.8131153360569,-46.3960659393468,
-14.4683433355075));
#30353=CARTESIAN_POINT('Ctrl Pts',(-13.2406268960767,-48.2803630804993,
-14.8498038985338));
#30354=CARTESIAN_POINT('Ctrl Pts',(-13.6673330636265,-50.1821542472109,
-14.8500516281495));
#30355=CARTESIAN_POINT('Ctrl Pts',(-11.9263392248003,-35.9359355586899,
1.59674363861575));
#30356=CARTESIAN_POINT('Ctrl Pts',(-11.8810411570285,-35.9248996259805,
1.15301423607239));
#30357=CARTESIAN_POINT('Ctrl Pts',(-11.8276425661371,-35.9022876226733,
0.635579107039569));
#30358=CARTESIAN_POINT('Ctrl Pts',(-11.6644253452223,-35.9492898606295,
-1.8686043110427));
#30359=CARTESIAN_POINT('Ctrl Pts',(-11.6521696602714,-36.3359843740415,
-3.70979114471714));
#30360=CARTESIAN_POINT('Ctrl Pts',(-11.8095985065123,-37.7794742164111,
-7.17014261467843));
#30361=CARTESIAN_POINT('Ctrl Pts',(-11.989011430306,-38.8217053622615,-8.73670574475537));
#30362=CARTESIAN_POINT('Ctrl Pts',(-12.490555802785,-41.4217720607139,-11.3734544105096));
#30363=CARTESIAN_POINT('Ctrl Pts',(-12.8156483043172,-42.960142369416,-12.4221714958418));
#30364=CARTESIAN_POINT('Ctrl Pts',(-13.5449152868542,-46.3511338849175,
-13.8545909095439));
#30365=CARTESIAN_POINT('Ctrl Pts',(-13.9494605088193,-48.1597570333837,
-14.2195188100007));
#30366=CARTESIAN_POINT('Ctrl Pts',(-14.352816918225,-49.980884503456,-14.2201291128083));
#30367=CARTESIAN_POINT('Ctrl Pts',(-9.50149509066523,-36.5850719698905,
3.46944695195361E-15));
#30368=CARTESIAN_POINT('Ctrl Pts',(-9.3800753775315,-36.6214111051535,-1.86858636179946));
#30369=CARTESIAN_POINT('Ctrl Pts',(-9.36705556804075,-37.0055036281572,
-3.71029995871102));
#30370=CARTESIAN_POINT('Ctrl Pts',(-9.52533731125042,-38.451897363606,-7.1693624749242));
#30371=CARTESIAN_POINT('Ctrl Pts',(-9.70422705227151,-39.49234722149,-8.73699595767225));
#30372=CARTESIAN_POINT('Ctrl Pts',(-9.98061312163023,-40.9249807596884,
-10.1890856763525));
#30373=CARTESIAN_POINT('Ctrl Pts',(-10.0068973767291,-41.0597112354399,
-10.3203928635211));
#30374=CARTESIAN_POINT('Ctrl Pts',(-10.0339108358238,-41.1968114627984,
-10.4488603766053));
#30375=CARTESIAN_POINT('Ctrl Pts',(-11.7862169042733,-35.914217116421,1.16573417585641E-15));
#30376=CARTESIAN_POINT('Ctrl Pts',(-11.6644253452223,-35.9492898606295,
-1.8686043110427));
#30377=CARTESIAN_POINT('Ctrl Pts',(-11.6521696602714,-36.3359843740415,
-3.70979114471714));
#30378=CARTESIAN_POINT('Ctrl Pts',(-11.8095985065123,-37.7794742164111,
-7.17014261467843));
#30379=CARTESIAN_POINT('Ctrl Pts',(-11.989011430306,-38.8217053622615,-8.73670574475537));
#30380=CARTESIAN_POINT('Ctrl Pts',(-12.2667035909955,-40.2612951155294,
-10.1966053555699));
#30381=CARTESIAN_POINT('Ctrl Pts',(-12.2944800077231,-40.4035980344053,
-10.335023194224));
#30382=CARTESIAN_POINT('Ctrl Pts',(-12.3230698431047,-40.5485470057454,
-10.4702558450949));
#30383=CARTESIAN_POINT('Ctrl Pts',(-9.34279883641492,-43.6145083358836,
1.24689082988532));
#30384=CARTESIAN_POINT('Ctrl Pts',(-9.29352897570114,-43.6025047584042,
0.764254661714488));
#30385=CARTESIAN_POINT('Ctrl Pts',(-9.24710292814764,-43.589834301908,0.332948671112318));
#30386=CARTESIAN_POINT('Ctrl Pts',(-9.08959664352382,-43.638752733162,-0.978870002656774));
#30387=CARTESIAN_POINT('Ctrl Pts',(-9.02147253461304,-43.8630440977154,
-1.98783577088714));
#30388=CARTESIAN_POINT('Ctrl Pts',(-8.99867539144458,-44.6599232717705,
-3.80852727283793));
#30389=CARTESIAN_POINT('Ctrl Pts',(-9.03489241259897,-45.2360569808236,
-4.65544360716999));
#30390=CARTESIAN_POINT('Ctrl Pts',(-9.18984064597521,-46.6460662566439,
-6.04997283348356));
#30391=CARTESIAN_POINT('Ctrl Pts',(-9.30516165135279,-47.491603139623,-6.61832169899598));
#30392=CARTESIAN_POINT('Ctrl Pts',(-9.58273633530685,-49.3114553051195,
-7.36768403082088));
#30393=CARTESIAN_POINT('Ctrl Pts',(-9.74382459483866,-50.3172192201122,
-7.57138648681379));
#30394=CARTESIAN_POINT('Ctrl Pts',(-9.90091582292576,-51.2881489781561,
-7.56962581969457));
#30395=CARTESIAN_POINT('Ctrl Pts',(-9.90389776310323,-41.3128793157233,
1.35489321026542));
#30396=CARTESIAN_POINT('Ctrl Pts',(-9.8558527655289,-41.301174150679,0.884255518290098));
#30397=CARTESIAN_POINT('Ctrl Pts',(-9.80727935893592,-41.2854482448494,
0.426396949017563));
#30398=CARTESIAN_POINT('Ctrl Pts',(-9.648061217345,-41.3339507669544,-1.2536081949907));
#30399=CARTESIAN_POINT('Ctrl Pts',(-9.59710950760655,-41.6081209010958,
-2.51960912779942));
#30400=CARTESIAN_POINT('Ctrl Pts',(-9.63005248742419,-42.6049670390315,
-4.84647586782148));
#30401=CARTESIAN_POINT('Ctrl Pts',(-9.71043261803931,-43.3248419422994,
-5.91572199043044));
#30402=CARTESIAN_POINT('Ctrl Pts',(-9.97242546011253,-45.1023943639113,
-7.69376028695677));
#30403=CARTESIAN_POINT('Ctrl Pts',(-10.1524895065122,-46.161761337687,-8.41063186554247));
#30404=CARTESIAN_POINT('Ctrl Pts',(-10.5695775166737,-48.4668856266306,
-9.37059840622391));
#30405=CARTESIAN_POINT('Ctrl Pts',(-10.8058013195489,-49.7204896475899,
-9.62435378622341));
#30406=CARTESIAN_POINT('Ctrl Pts',(-11.0389609452142,-50.9539676685889,
-9.62320046360561));
#30407=CARTESIAN_POINT('Ctrl Pts',(-10.0047404051437,-38.9464705831155,
1.47293192394294));
#30408=CARTESIAN_POINT('Ctrl Pts',(-9.95803136026999,-38.9350908951825,
1.01538091584094));
#30409=CARTESIAN_POINT('Ctrl Pts',(-9.90712214456661,-38.91605504704,0.52858071787014));
#30410=CARTESIAN_POINT('Ctrl Pts',(-9.74614391855838,-38.9644836024863,
-1.55402875457437));
#30411=CARTESIAN_POINT('Ctrl Pts',(-9.71379866052385,-39.2926120042886,
-3.10121432124472));
#30412=CARTESIAN_POINT('Ctrl Pts',(-9.80788452010917,-40.5087724506344,
-5.98129145449945));
#30413=CARTESIAN_POINT('Ctrl Pts',(-9.93643935033497,-41.3854277882792,
-7.29389406573111));
#30414=CARTESIAN_POINT('Ctrl Pts',(-10.3155272531674,-43.5650308735925,
-9.49113593807561));
#30415=CARTESIAN_POINT('Ctrl Pts',(-10.5663179729168,-44.8579833049588,
-10.3708286017124));
#30416=CARTESIAN_POINT('Ctrl Pts',(-11.1360404748697,-47.6940136086793,
-11.5604045561299));
#30417=CARTESIAN_POINT('Ctrl Pts',(-11.454400767937,-49.2184417854932,-11.8694761541429));
#30418=CARTESIAN_POINT('Ctrl Pts',(-11.770728108961,-50.7390783576438,-11.8687142284813));
#30419=CARTESIAN_POINT('Ctrl Pts',(-9.64145132693333,-36.6062244663075,
1.59647068126627));
#30420=CARTESIAN_POINT('Ctrl Pts',(-9.59613798295645,-36.5951848118862,
1.15259163659386));
#30421=CARTESIAN_POINT('Ctrl Pts',(-9.54279427444346,-36.5727117312865,
0.635573001860467));
#30422=CARTESIAN_POINT('Ctrl Pts',(-9.3800753775315,-36.6214111051535,-1.86858636179946));
#30423=CARTESIAN_POINT('Ctrl Pts',(-9.36705556804075,-37.0055036281572,
-3.71029995871102));
#30424=CARTESIAN_POINT('Ctrl Pts',(-9.52533731125042,-38.451897363606,-7.1693624749242));
#30425=CARTESIAN_POINT('Ctrl Pts',(-9.70422705227151,-39.49234722149,-8.73699595767225));
#30426=CARTESIAN_POINT('Ctrl Pts',(-10.2059604433546,-42.093057470626,-11.3730256982475));
#30427=CARTESIAN_POINT('Ctrl Pts',(-10.5307434056497,-43.6303739147808,
-12.4235805192275));
#30428=CARTESIAN_POINT('Ctrl Pts',(-11.2603557414205,-47.0225411281101,
-13.8529470821549));
#30429=CARTESIAN_POINT('Ctrl Pts',(-11.6646867919251,-48.830372710993,-14.2204718556692));
#30430=CARTESIAN_POINT('Ctrl Pts',(-12.0680951184148,-50.6517393542017,
-14.2198708430668));
#30431=CARTESIAN_POINT('Ctrl Pts',(-11.9263392248003,-35.9359355586899,
1.59674363861575));
#30432=CARTESIAN_POINT('Ctrl Pts',(-11.8810411570285,-35.9248996259805,
1.15301423607239));
#30433=CARTESIAN_POINT('Ctrl Pts',(-11.8276425661371,-35.9022876226733,
0.635579107039569));
#30434=CARTESIAN_POINT('Ctrl Pts',(-11.6644253452223,-35.9492898606295,
-1.8686043110427));
#30435=CARTESIAN_POINT('Ctrl Pts',(-11.6521696602714,-36.3359843740415,
-3.70979114471595));
#30436=CARTESIAN_POINT('Ctrl Pts',(-11.8095985065123,-37.7794742164111,
-7.17014261467964));
#30437=CARTESIAN_POINT('Ctrl Pts',(-11.9890114303072,-38.8217053622615,
-8.73670574475537));
#30438=CARTESIAN_POINT('Ctrl Pts',(-12.4905558027838,-41.4217720607139,
-11.3734544105096));
#30439=CARTESIAN_POINT('Ctrl Pts',(-12.8156483043172,-42.9601423694208,
-12.422171495837));
#30440=CARTESIAN_POINT('Ctrl Pts',(-13.5449152868542,-46.3511338849126,
-13.8545909095487));
#30441=CARTESIAN_POINT('Ctrl Pts',(-13.94946050882,-48.1597570333872,-14.2195188100007));
#30442=CARTESIAN_POINT('Ctrl Pts',(-14.352816918225,-49.980884503456,-14.2201291128083));
#30443=CARTESIAN_POINT('Ctrl Pts',(-12.8849080239687,-38.1015519292156,
1.47327599461705));
#30444=CARTESIAN_POINT('Ctrl Pts',(-12.8382182351927,-38.0901769326068,
1.01591361476925));
#30445=CARTESIAN_POINT('Ctrl Pts',(-12.7872398386582,-38.0709659683553,
0.528588413625886));
#30446=CARTESIAN_POINT('Ctrl Pts',(-12.6256334607596,-38.1172552346473,
-1.55405138011728));
#30447=CARTESIAN_POINT('Ctrl Pts',(-12.5942514039184,-38.4486635210123,
-3.10057294641332));
#30448=CARTESIAN_POINT('Ctrl Pts',(-12.687262162083,-39.6611635256934,-5.98227484333945));
#30449=CARTESIAN_POINT('Ctrl Pts',(-12.8164764794026,-40.5400642286176,
-7.29352824390953));
#30450=CARTESIAN_POINT('Ctrl Pts',(-13.1953261187877,-42.718856099577,-9.49167634234811));
#30451=CARTESIAN_POINT('Ctrl Pts',(-13.4465070217463,-44.0131369578427,
-10.3690524867682));
#30452=CARTESIAN_POINT('Ctrl Pts',(-14.0157941959057,-46.8476852602797,
-11.5624766483461));
#30453=CARTESIAN_POINT('Ctrl Pts',(-14.3344204493215,-48.3731128199053,
-11.8682745705877));
#30454=CARTESIAN_POINT('Ctrl Pts',(-14.6506863563567,-49.8934463159786,
-11.8690397849987));
#30455=CARTESIAN_POINT('Ctrl Pts',(-14.248185985062,-40.038449962147,1.3554121877608));
#30456=CARTESIAN_POINT('Ctrl Pts',(-14.2001700323384,-40.026751873255,0.885059012386578));
#30457=CARTESIAN_POINT('Ctrl Pts',(-14.1514922771424,-40.0107618317946,
0.426408556877058));
#30458=CARTESIAN_POINT('Ctrl Pts',(-13.9913266653939,-40.056037566468,-1.25364232212933));
#30459=CARTESIAN_POINT('Ctrl Pts',(-13.9418277959601,-40.3351549001415,
-2.51864171287987));
#30460=CARTESIAN_POINT('Ctrl Pts',(-13.973149151259,-41.3264798268969,-4.84795915807396));
#30461=CARTESIAN_POINT('Ctrl Pts',(-14.0545240163445,-42.0497415170713,
-5.91517020468713));
#30462=CARTESIAN_POINT('Ctrl Pts',(-14.3161574747883,-43.8260703470498,
-7.69457540337582));
#30463=CARTESIAN_POINT('Ctrl Pts',(-14.4968100523213,-44.8874410477277,
-8.40795287034433));
#30464=CARTESIAN_POINT('Ctrl Pts',(-14.9132414377173,-47.1903299665294,
-9.37372383744494));
#30465=CARTESIAN_POINT('Ctrl Pts',(-15.1498577118458,-48.4454445415184,
-9.62254086005834));
#30466=CARTESIAN_POINT('Ctrl Pts',(-15.382933362694,-49.6784622796992,-9.62369151535366));
#30467=CARTESIAN_POINT('Ctrl Pts',(-15.9637816213004,-41.6721936506077,
1.24768178593774));
#30468=CARTESIAN_POINT('Ctrl Pts',(-15.9145560268668,-41.6602008576382,
0.765479239898045));
#30469=CARTESIAN_POINT('Ctrl Pts',(-15.8679709451303,-41.6471278409701,
0.332966362258481));
#30470=CARTESIAN_POINT('Ctrl Pts',(-15.7090206532774,-41.6911284346186,
-0.978922014674807));
#30471=CARTESIAN_POINT('Ctrl Pts',(-15.6431107691496,-41.9229596586886,
-1.98636136651691));
#30472=CARTESIAN_POINT('Ctrl Pts',(-15.617842162883,-42.7114241414764,-3.81078790535973));
#30473=CARTESIAN_POINT('Ctrl Pts',(-15.6555752252088,-43.2927195379191,
-4.65460264917615));
#30474=CARTESIAN_POINT('Ctrl Pts',(-15.8099757341484,-44.7008639791348,
-6.05121512485625));
#30475=CARTESIAN_POINT('Ctrl Pts',(-15.9261936999267,-45.5494546745318,
-6.61423873299709));
#30476=CARTESIAN_POINT('Ctrl Pts',(-16.2027676442761,-47.3658999879523,
-7.37244739486684));
#30477=CARTESIAN_POINT('Ctrl Pts',(-16.3644346256248,-48.3739721396825,
-7.56862230182844));
#30478=CARTESIAN_POINT('Ctrl Pts',(-16.5214173008833,-49.3441943438431,
-7.57037421505976));
#30479=CARTESIAN_POINT('Ctrl Pts',(-14.7529241788868,-34.861504297702,1.596470776103));
#30480=CARTESIAN_POINT('Ctrl Pts',(-14.7414705295769,-34.8603993451942,
1.48695587718827));
#30481=CARTESIAN_POINT('Ctrl Pts',(-14.7300185573963,-34.8592949433733,
1.37746402257862));
#30482=CARTESIAN_POINT('Ctrl Pts',(-14.6812048800309,-34.8545841497113,
0.910698635110844));
#30483=CARTESIAN_POINT('Ctrl Pts',(-14.641323265537,-34.8466226370302,0.486448413024372));
#30484=CARTESIAN_POINT('Ctrl Pts',(-14.4963699338215,-34.913734033555,-1.86858636180693));
#30485=CARTESIAN_POINT('Ctrl Pts',(-14.5381447125539,-35.2957699605276,
-3.71029995869199));
#30486=CARTESIAN_POINT('Ctrl Pts',(-14.9006586664723,-36.7049156525157,
-7.1693624749433));
#30487=CARTESIAN_POINT('Ctrl Pts',(-15.2257990212174,-37.7093165664316,
-8.73699595772034));
#30488=CARTESIAN_POINT('Ctrl Pts',(-16.092545148042,-40.2121512289274,-11.3730256981995));
#30489=CARTESIAN_POINT('Ctrl Pts',(-16.6328052292483,-41.6875985735071,
-12.423580519199));
#30490=CARTESIAN_POINT('Ctrl Pts',(-17.8377468920061,-44.9414037540446,
-13.8529470821835));
#30491=CARTESIAN_POINT('Ctrl Pts',(-18.4952436947709,-46.6732919100445,
-14.2204718557262));
#30492=CARTESIAN_POINT('Ctrl Pts',(-19.1537534053194,-48.4187086763094,
-14.2198708430667));
#30493=CARTESIAN_POINT('Ctrl Pts',(-15.1415840475452,-33.992572254002,1.62964621771061));
#30494=CARTESIAN_POINT('Ctrl Pts',(-15.1301302752945,-33.9914672896339,
1.52013014329387));
#30495=CARTESIAN_POINT('Ctrl Pts',(-15.1186784705795,-33.9903629797955,
1.41064104114018));
#30496=CARTESIAN_POINT('Ctrl Pts',(-15.069864603448,-33.9856518446506,0.943868932653774));
#30497=CARTESIAN_POINT('Ctrl Pts',(-15.0295355352549,-33.9768575865842,
0.508392298453448));
#30498=CARTESIAN_POINT('Ctrl Pts',(-14.8839745452192,-34.043697838521,-1.95287905130899));
#30499=CARTESIAN_POINT('Ctrl Pts',(-14.9333078250241,-34.4404940724738,
-3.87337387078378));
#30500=CARTESIAN_POINT('Ctrl Pts',(-15.3212948555725,-35.9075266005405,
-7.48792130214209));
#30501=CARTESIAN_POINT('Ctrl Pts',(-15.6662361882241,-36.9538988571314,
-9.12360836231688));
#30502=CARTESIAN_POINT('Ctrl Pts',(-16.5814962693528,-39.5635848921456,
-11.8774049927144));
#30503=CARTESIAN_POINT('Ctrl Pts',(-17.1508209097751,-41.1012880289292,
-12.9732563608727));
#30504=CARTESIAN_POINT('Ctrl Pts',(-18.4192429936803,-44.4962044519299,
-14.4676858045622));
#30505=CARTESIAN_POINT('Ctrl Pts',(-19.110436436978,-46.3001798643399,-14.8501851005532));
#30506=CARTESIAN_POINT('Ctrl Pts',(-19.8034868749641,-48.1219785107276,
-14.8499483202528));
#30507=CARTESIAN_POINT('Ctrl Pts',(-16.0080796379928,-33.5971163401331,
1.62975540065039));
#30508=CARTESIAN_POINT('Ctrl Pts',(-15.9966258648996,-33.5960113756864,
1.52023931818491));
#30509=CARTESIAN_POINT('Ctrl Pts',(-15.9851740659136,-33.5949070766362,
1.41075023429581));
#30510=CARTESIAN_POINT('Ctrl Pts',(-15.9363601779558,-33.5901958958465,
0.94397808226918));
#30511=CARTESIAN_POINT('Ctrl Pts',(-15.8959902453789,-33.5813120719023,
0.508394167540087));
#30512=CARTESIAN_POINT('Ctrl Pts',(-15.7501528462318,-33.6475470722586,
-1.95288623100104));
#30513=CARTESIAN_POINT('Ctrl Pts',(-15.7999367855235,-34.0453300100855,
-3.87317034519272));
#30514=CARTESIAN_POINT('Ctrl Pts',(-16.1874208229716,-35.5112613558745,
-7.48823335803731));
#30515=CARTESIAN_POINT('Ctrl Pts',(-16.5326707001234,-36.5583090926344,
-9.12349227711425));
#30516=CARTESIAN_POINT('Ctrl Pts',(-17.4478193086362,-39.1677510875279,
-11.8775764776552));
#30517=CARTESIAN_POINT('Ctrl Pts',(-18.0173264967234,-40.7058538586162,
-12.9726927515386));
#30518=CARTESIAN_POINT('Ctrl Pts',(-19.2855449177196,-44.1003244488304,
-14.4683433354976));
#30519=CARTESIAN_POINT('Ctrl Pts',(-19.9768684693679,-45.9046009234682,
-14.8498038985385));
#30520=CARTESIAN_POINT('Ctrl Pts',(-20.6698844856026,-47.7263079790887,
-14.8500516281495));
#30521=CARTESIAN_POINT('Ctrl Pts',(-16.9191631550059,-33.8728645130297,
1.59674373345244));
#30522=CARTESIAN_POINT('Ctrl Pts',(-16.9077095035903,-33.8717595603218,
1.48722881441586));
#30523=CARTESIAN_POINT('Ctrl Pts',(-16.8962575457316,-33.8706551854743,
1.37773700546765));
#30524=CARTESIAN_POINT('Ctrl Pts',(-16.8474438163005,-33.8659442777035,
0.910971509149462));
#30525=CARTESIAN_POINT('Ctrl Pts',(-16.8074600408464,-33.8577588503261,
0.486453085740971));
#30526=CARTESIAN_POINT('Ctrl Pts',(-16.6618156863547,-33.9233571178964,
-1.86860431103707));
#30527=CARTESIAN_POINT('Ctrl Pts',(-16.7047171138001,-34.3078598045567,
-3.70979114471372));
#30528=CARTESIAN_POINT('Ctrl Pts',(-17.0659735849724,-35.7142525408506,
-7.17014261468198));
#30529=CARTESIAN_POINT('Ctrl Pts',(-17.3918853009681,-36.7203421551653,
-8.73670574471736));
#30530=CARTESIAN_POINT('Ctrl Pts',(-18.2583527462481,-39.222566717407,-11.3734544105477));
#30531=CARTESIAN_POINT('Ctrl Pts',(-18.7990691966108,-40.699013147727,-12.422171495866));
#30532=CARTESIAN_POINT('Ctrl Pts',(-20.0035017021128,-43.9517037462935,
-13.8545909095196));
#30533=CARTESIAN_POINT('Ctrl Pts',(-20.6613231478877,-45.6843449310519,
-14.2195188099912));
#30534=CARTESIAN_POINT('Ctrl Pts',(-21.3197474319156,-47.429532347212,-14.2201291128083));
#30535=CARTESIAN_POINT('Ctrl Pts',(-14.6113821712783,-34.8604849513723,
1.04083408558608E-14));
#30536=CARTESIAN_POINT('Ctrl Pts',(-14.4963699338215,-34.913734033555,-1.86858636180693));
#30537=CARTESIAN_POINT('Ctrl Pts',(-14.5381447125539,-35.2957699605276,
-3.71029995869199));
#30538=CARTESIAN_POINT('Ctrl Pts',(-14.9006586664723,-36.7049156525157,
-7.1693624749433));
#30539=CARTESIAN_POINT('Ctrl Pts',(-15.2257990212174,-37.7093165664316,
-8.73699595772034));
#30540=CARTESIAN_POINT('Ctrl Pts',(-15.7032568890462,-39.0880341222414,
-10.1890856763482));
#30541=CARTESIAN_POINT('Ctrl Pts',(-15.7484477541819,-39.2176525965103,
-10.3203928635132));
#30542=CARTESIAN_POINT('Ctrl Pts',(-15.7946976518867,-39.3495129251816,
-10.4488603765943));
#30543=CARTESIAN_POINT('Ctrl Pts',(-16.7773762106051,-33.871308617679,-4.87765735985715E-9));
#30544=CARTESIAN_POINT('Ctrl Pts',(-16.6618156862293,-33.923357118505,-1.8686043142631));
#30545=CARTESIAN_POINT('Ctrl Pts',(-16.7047171137966,-34.307859805123,-3.70979114625147));
#30546=CARTESIAN_POINT('Ctrl Pts',(-16.8853453492638,-35.0110561726707,
-5.43996687972834));
#30547=CARTESIAN_POINT('Ctrl Pts',(-17.0659735848888,-35.7142525408324,
-7.17014261471563));
#30548=CARTESIAN_POINT('Ctrl Pts',(-17.3918853009222,-36.7203421551587,
-8.73670574474088));
#30549=CARTESIAN_POINT('Ctrl Pts',(-17.8251190235969,-37.9714544362847,
-10.0550800776385));
#30550=CARTESIAN_POINT('Ctrl Pts',(-17.871625938579,-38.1057592455506,-10.1966053555787));
#30551=CARTESIAN_POINT('Ctrl Pts',(-17.9193714483085,-38.2426607296452,
-10.335023194235));
#30552=CARTESIAN_POINT('Ctrl Pts',(-17.9682986697938,-38.3820655716606,
-10.4702558451073));
#30553=CARTESIAN_POINT('Ctrl Pts',(-15.4546943255721,-41.8409566234848,
1.2468909247223));
#30554=CARTESIAN_POINT('Ctrl Pts',(-15.4432419692989,-41.8398517957208,
1.13738838925849));
#30555=CARTESIAN_POINT('Ctrl Pts',(-15.431788261189,-41.8387464827955,1.02786758221435));
#30556=CARTESIAN_POINT('Ctrl Pts',(-15.3829764714434,-41.8340390406225,
0.561172897424349));
#30557=CARTESIAN_POINT('Ctrl Pts',(-15.3475914064577,-41.8343710194632,
0.254828874437198));
#30558=CARTESIAN_POINT('Ctrl Pts',(-15.2075196936098,-41.9009886759871,
-0.978870002694615));
#30559=CARTESIAN_POINT('Ctrl Pts',(-15.1720089791053,-42.132692149374,-1.98783577086012));
#30560=CARTESIAN_POINT('Ctrl Pts',(-15.2628516086326,-42.9247046141117,
-3.8085272728648));
#30561=CARTESIAN_POINT('Ctrl Pts',(-15.3806923682557,-43.4898198932175,
-4.65544360728965));
#30562=CARTESIAN_POINT('Ctrl Pts',(-15.7347286944236,-44.8634258749694,
-6.04997283336378));
#30563=CARTESIAN_POINT('Ctrl Pts',(-15.969208342928,-45.6839445214029,-6.61832169892421));
#30564=CARTESIAN_POINT('Ctrl Pts',(-16.5029496832502,-47.4457702195624,
-7.36768403089269));
#30565=CARTESIAN_POINT('Ctrl Pts',(-16.8055334255118,-48.4183716585711,
-7.57138648693262));
#30566=CARTESIAN_POINT('Ctrl Pts',(-17.0992034029526,-49.3570623388654,
-7.5696258196945));
#30567=CARTESIAN_POINT('Ctrl Pts',(-15.6825261124555,-39.4829021650677,
1.35489330510232));
#30568=CARTESIAN_POINT('Ctrl Pts',(-15.6710733564743,-39.4817972987419,
1.24538694781336));
#30569=CARTESIAN_POINT('Ctrl Pts',(-15.6596201873397,-39.4806922726919,
1.1358750903288));
#30570=CARTESIAN_POINT('Ctrl Pts',(-15.6108078040333,-39.4759837722005,
0.669158551001817));
#30571=CARTESIAN_POINT('Ctrl Pts',(-15.5740132903121,-39.473708863974,0.326351368866041));
#30572=CARTESIAN_POINT('Ctrl Pts',(-15.4322923841624,-39.540168475028,-1.25360819501648));
#30573=CARTESIAN_POINT('Ctrl Pts',(-15.4208777676315,-39.8187991368524,
-2.51960912778186));
#30574=CARTESIAN_POINT('Ctrl Pts',(-15.5953514322613,-40.8008105435132,
-4.84647586783895));
#30575=CARTESIAN_POINT('Ctrl Pts',(-15.7773622894425,-41.5019188729544,
-5.91572199050949));
#30576=CARTESIAN_POINT('Ctrl Pts',(-16.2896605076835,-43.2240929050568,
-7.69376028687766));
#30577=CARTESIAN_POINT('Ctrl Pts',(-16.6186554012328,-44.2470512648665,
-8.41063186549471));
#30578=CARTESIAN_POINT('Ctrl Pts',(-17.359551447157,-46.4693548995032,-9.3705984062717));
#30579=CARTESIAN_POINT('Ctrl Pts',(-17.7717772858575,-47.6765808868262,
-9.624353786328));
#30580=CARTESIAN_POINT('Ctrl Pts',(-18.1781059077967,-48.8643218056539,
-9.62320046360555));
#30581=CARTESIAN_POINT('Ctrl Pts',(-15.4455672457337,-37.1262286569852,
1.47293201877975));
#30582=CARTESIAN_POINT('Ctrl Pts',(-15.4341140531475,-37.1251237485394,
1.36342148686276));
#30583=CARTESIAN_POINT('Ctrl Pts',(-15.4226614701642,-37.1240190301311,
1.25391940542253));
#30584=CARTESIAN_POINT('Ctrl Pts',(-15.3738484494875,-37.1193093979792,
0.787178992714135));
#30585=CARTESIAN_POINT('Ctrl Pts',(-15.3355356362474,-37.1142341193451,
0.40455974469035));
#30586=CARTESIAN_POINT('Ctrl Pts',(-15.1921664085198,-37.1808604460558,
-1.55402875458989));
#30587=CARTESIAN_POINT('Ctrl Pts',(-15.206847919016,-37.510252183997,-3.10121432122704));
#30588=CARTESIAN_POINT('Ctrl Pts',(-15.4730537974676,-38.7006440565956,
-5.98129145451713));
#30589=CARTESIAN_POINT('Ctrl Pts',(-15.725061187509,-39.5500810470411,-7.29389406578391));
#30590=CARTESIAN_POINT('Ctrl Pts',(-16.4104803825999,-41.6535490822059,
-9.49113593802281));
#30591=CARTESIAN_POINT('Ctrl Pts',(-16.8427247306082,-42.8976498813535,
-10.370828601679));
#30592=CARTESIAN_POINT('Ctrl Pts',(-17.8102574730307,-45.6237335200178,
-11.5604045561632));
#30593=CARTESIAN_POINT('Ctrl Pts',(-18.3423260668094,-47.0873378224416,
-11.8694761541809));
#30594=CARTESIAN_POINT('Ctrl Pts',(-18.8718427994038,-48.5474784324871,
-11.8687142284813));
#30595=CARTESIAN_POINT('Ctrl Pts',(-14.7529241788868,-34.861504297702,1.596470776103));
#30596=CARTESIAN_POINT('Ctrl Pts',(-14.7414705295769,-34.8603993451942,
1.48695587718829));
#30597=CARTESIAN_POINT('Ctrl Pts',(-14.7300185573963,-34.8592949433733,
1.37746402257859));
#30598=CARTESIAN_POINT('Ctrl Pts',(-14.6812048800309,-34.8545841497113,
0.910698635110924));
#30599=CARTESIAN_POINT('Ctrl Pts',(-14.641323265537,-34.8466226370302,0.486448413024372));
#30600=CARTESIAN_POINT('Ctrl Pts',(-14.4963699338215,-34.913734033555,-1.86858636180693));
#30601=CARTESIAN_POINT('Ctrl Pts',(-14.5381447125539,-35.2957699605276,
-3.71029995869199));
#30602=CARTESIAN_POINT('Ctrl Pts',(-14.9006586664723,-36.7049156525157,
-7.1693624749433));
#30603=CARTESIAN_POINT('Ctrl Pts',(-15.2257990212174,-37.7093165664316,
-8.73699595772034));
#30604=CARTESIAN_POINT('Ctrl Pts',(-16.092545148042,-40.2121512289274,-11.3730256981995));
#30605=CARTESIAN_POINT('Ctrl Pts',(-16.6328052292483,-41.6875985735071,
-12.423580519199));
#30606=CARTESIAN_POINT('Ctrl Pts',(-17.8377468920061,-44.9414037540446,
-13.8529470821835));
#30607=CARTESIAN_POINT('Ctrl Pts',(-18.495243694773,-46.6732919100438,-14.2204718557215));
#30608=CARTESIAN_POINT('Ctrl Pts',(-19.1537534053194,-48.4187086763094,
-14.2198708430667));
#30609=CARTESIAN_POINT('Ctrl Pts',(-16.9191631550059,-33.8728645130297,
1.59674373345244));
#30610=CARTESIAN_POINT('Ctrl Pts',(-16.9077095035903,-33.8717595603218,
1.48722881441586));
#30611=CARTESIAN_POINT('Ctrl Pts',(-16.8962575457316,-33.8706551854743,
1.37773700546765));
#30612=CARTESIAN_POINT('Ctrl Pts',(-16.8474438163005,-33.8659442777035,
0.910971509149462));
#30613=CARTESIAN_POINT('Ctrl Pts',(-16.8074600408464,-33.8577588503261,
0.486453085740971));
#30614=CARTESIAN_POINT('Ctrl Pts',(-16.6618156863547,-33.9233571178964,
-1.86860431103707));
#30615=CARTESIAN_POINT('Ctrl Pts',(-16.7047171138049,-34.3078598045567,
-3.70979114471372));
#30616=CARTESIAN_POINT('Ctrl Pts',(-17.0659735849676,-35.7142525408506,
-7.17014261468198));
#30617=CARTESIAN_POINT('Ctrl Pts',(-17.3918853009681,-36.7203421551653,
-8.73670574471736));
#30618=CARTESIAN_POINT('Ctrl Pts',(-18.2583527462481,-39.222566717407,-11.3734544105478));
#30619=CARTESIAN_POINT('Ctrl Pts',(-18.7990691966084,-40.6990131477271,
-12.422171495866));
#30620=CARTESIAN_POINT('Ctrl Pts',(-20.0035017021152,-43.9517037462935,
-13.8545909095196));
#30621=CARTESIAN_POINT('Ctrl Pts',(-20.6613231478854,-45.6843449310521,
-14.2195188099864));
#30622=CARTESIAN_POINT('Ctrl Pts',(-21.3197474319156,-47.429532347212,-14.2201291128083));
#30623=CARTESIAN_POINT('Ctrl Pts',(-18.176174449474,-35.8800194678371,1.4732760894538));
#30624=CARTESIAN_POINT('Ctrl Pts',(-18.1647212542338,-35.8789145591356,
1.36376553217263));
#30625=CARTESIAN_POINT('Ctrl Pts',(-18.1532686893032,-35.8778098747321,
1.25426350829));
#30626=CARTESIAN_POINT('Ctrl Pts',(-18.1044556029969,-35.8731000987406,
0.787522958372421));
#30627=CARTESIAN_POINT('Ctrl Pts',(-18.0660140128963,-35.867742569121,0.404565634785468));
#30628=CARTESIAN_POINT('Ctrl Pts',(-17.9217737308695,-35.9324615528111,
-1.55405138011628));
#30629=CARTESIAN_POINT('Ctrl Pts',(-17.9378754148266,-36.2649627130452,
-3.10057294641604));
#30630=CARTESIAN_POINT('Ctrl Pts',(-18.2024961997114,-37.4518844049459,
-5.98227484333679));
#30631=CARTESIAN_POINT('Ctrl Pts',(-18.4554759130357,-38.3034500513459,
-7.29352824386188));
#30632=CARTESIAN_POINT('Ctrl Pts',(-19.1405438219426,-40.4061490373993,
-9.49167634239581));
#30633=CARTESIAN_POINT('Ctrl Pts',(-19.5733634365382,-41.6515092131651,
-10.3690524868116));
#30634=CARTESIAN_POINT('Ctrl Pts',(-20.5402543714365,-44.3761878888615,
-11.5624766483027));
#30635=CARTESIAN_POINT('Ctrl Pts',(-21.0727284454552,-45.8407435516478,
-11.8682745705592));
#30636=CARTESIAN_POINT('Ctrl Pts',(-21.6021412371496,-47.3005929134933,
-11.8690397849987));
#30637=CARTESIAN_POINT('Ctrl Pts',(-19.8012255369163,-37.6031879890151,
1.35541228259761));
#30638=CARTESIAN_POINT('Ctrl Pts',(-19.7897727769317,-37.6020831223045,
1.24590588705071));
#30639=CARTESIAN_POINT('Ctrl Pts',(-19.7783196350267,-37.6009781475451,
1.13639411638292));
#30640=CARTESIAN_POINT('Ctrl Pts',(-19.7295071527293,-37.5962694300918,
0.66967737009692));
#30641=CARTESIAN_POINT('Ctrl Pts',(-19.6925183989934,-37.5935687898309,
0.326360253165228));
#30642=CARTESIAN_POINT('Ctrl Pts',(-19.5494836419035,-37.6571514683751,
-1.25364232213017));
#30643=CARTESIAN_POINT('Ctrl Pts',(-19.5402111377933,-37.9404722137081,
-2.51864171289113));
#30644=CARTESIAN_POINT('Ctrl Pts',(-19.7122939334867,-38.9172493885169,
-4.84795915806269));
#30645=CARTESIAN_POINT('Ctrl Pts',(-19.895771390238,-39.6215684668484,-5.91517020461549));
#30646=CARTESIAN_POINT('Ctrl Pts',(-20.4075397474893,-41.3425825070781,
-7.69457540344745));
#30647=CARTESIAN_POINT('Ctrl Pts',(-20.7374023418787,-42.3674404421053,
-8.40795287041159));
#30648=CARTESIAN_POINT('Ctrl Pts',(-21.4773303202423,-44.5876249069951,
-9.37372383737758));
#30649=CARTESIAN_POINT('Ctrl Pts',(-21.8901596096273,-45.7962902185076,
-9.62254086002985));
#30650=CARTESIAN_POINT('Ctrl Pts',(-22.296339606421,-46.9835874904388,-9.6236915153537));
#30651=CARTESIAN_POINT('Ctrl Pts',(-21.7318648520657,-38.9761478068777,
1.24768188077458));
#30652=CARTESIAN_POINT('Ctrl Pts',(-21.7204124896908,-38.9750429785251,
1.13817928700318));
#30653=CARTESIAN_POINT('Ctrl Pts',(-21.7089588230812,-38.9739377437724,
1.02865861227348));
#30654=CARTESIAN_POINT('Ctrl Pts',(-21.6601468824655,-38.9692299709343,
0.561963612064401));
#30655=CARTESIAN_POINT('Ctrl Pts',(-21.6244657828418,-38.9689131059758,
0.254842414697181));
#30656=CARTESIAN_POINT('Ctrl Pts',(-21.4823916742034,-39.0311461269472,
-0.97892201467465));
#30657=CARTESIAN_POINT('Ctrl Pts',(-21.450145680808,-39.2699975980215,-1.98636136654028));
#30658=CARTESIAN_POINT('Ctrl Pts',(-21.5373444678282,-40.054032746971,-3.8107879053363));
#30659=CARTESIAN_POINT('Ctrl Pts',(-21.6574204222689,-40.6240414198954,
-4.65460264907096));
#30660=CARTESIAN_POINT('Ctrl Pts',(-22.0106492052165,-41.9958794972643,
-6.05121512496137));
#30661=CARTESIAN_POINT('Ctrl Pts',(-22.2464512872363,-42.8192932220575,
-6.61423873309305));
#30662=CARTESIAN_POINT('Ctrl Pts',(-22.7787172285155,-44.5778891652519,
-7.37244739477071));
#30663=CARTESIAN_POINT('Ctrl Pts',(-23.0822022983039,-45.5526929856245,
-7.56862230174279));
#30664=CARTESIAN_POINT('Ctrl Pts',(-23.3756641324465,-46.490698762655,-7.57037421505983));
#30665=CARTESIAN_POINT('Ctrl Pts',(-19.5640700378121,-32.4071044310925,
1.59647086199751));
#30666=CARTESIAN_POINT('Ctrl Pts',(-19.5174819665884,-32.4092782047833,
1.15259176011195));
#30667=CARTESIAN_POINT('Ctrl Pts',(-19.4599676462981,-32.4027440988463,
0.635573083870355));
#30668=CARTESIAN_POINT('Ctrl Pts',(-19.3175602025801,-32.4953140196741,
-1.86858636177345));
#30669=CARTESIAN_POINT('Ctrl Pts',(-19.4132791553027,-32.8675162010731,
-3.7102999586904));
#30670=CARTESIAN_POINT('Ctrl Pts',(-19.9726455811605,-34.2107277069995,
-7.16936247494489));
#30671=CARTESIAN_POINT('Ctrl Pts',(-20.4374176294115,-35.1586329709599,
-8.73699595768469));
#30672=CARTESIAN_POINT('Ctrl Pts',(-21.6515320408422,-37.5126415502852,
-11.3730256982353));
#30673=CARTESIAN_POINT('Ctrl Pts',(-22.3962711037445,-38.8961839421996,
-12.423580519285));
#30674=CARTESIAN_POINT('Ctrl Pts',(-24.0520129553695,-41.9453890000367,
-13.8529470820976));
#30675=CARTESIAN_POINT('Ctrl Pts',(-24.9492907716223,-43.5660774805332,
-14.220471855655));
#30676=CARTESIAN_POINT('Ctrl Pts',(-25.8494965077556,-45.2000127177928,
-14.2198708430668));
#30677=CARTESIAN_POINT('Ctrl Pts',(-19.8251119861392,-31.4917047963494,
1.62964630360508));
#30678=CARTESIAN_POINT('Ctrl Pts',(-19.7789125871832,-31.4938604347953,
1.18947037066722));
#30679=CARTESIAN_POINT('Ctrl Pts',(-19.7204885320786,-31.4865951547092,
0.664244043748249));
#30680=CARTESIAN_POINT('Ctrl Pts',(-19.5774004975844,-31.5789716510579,
-1.95287905126329));
#30681=CARTESIAN_POINT('Ctrl Pts',(-19.6827016273729,-31.9647082139024,
-3.8733738707834));
#30682=CARTESIAN_POINT('Ctrl Pts',(-20.2755200063962,-33.3615921546183,
-7.48792130214242));
#30683=CARTESIAN_POINT('Ctrl Pts',(-20.7658646319509,-34.348223580536,-9.1236083623051));
#30684=CARTESIAN_POINT('Ctrl Pts',(-22.0432057314562,-36.8010916838934,
-11.8774049927262));
#30685=CARTESIAN_POINT('Ctrl Pts',(-22.8255734412877,-38.242119875778,-12.9732563609107));
#30686=CARTESIAN_POINT('Ctrl Pts',(-24.5642317984401,-41.421965661227,-14.4676858045243));
#30687=CARTESIAN_POINT('Ctrl Pts',(-25.5051223583005,-43.1092121218843,
-14.8501851005247));
#30688=CARTESIAN_POINT('Ctrl Pts',(-26.4503875219921,-44.8138361237938,
-14.8499483202528));
#30689=CARTESIAN_POINT('Ctrl Pts',(-20.6265086564331,-30.9769588736644,
1.62975548654484));
#30690=CARTESIAN_POINT('Ctrl Pts',(-20.5803155398565,-30.9791142189677,
1.18963941047879));
#30691=CARTESIAN_POINT('Ctrl Pts',(-20.5218547654337,-30.9718018056147,
0.664246485816634));
#30692=CARTESIAN_POINT('Ctrl Pts',(-20.3783842202168,-31.0635831036134,
-1.95288623095009));
#30693=CARTESIAN_POINT('Ctrl Pts',(-20.4842718449966,-31.4502321915287,
-3.8731703451935));
#30694=CARTESIAN_POINT('Ctrl Pts',(-21.0764356360931,-32.8460977418056,
-7.48823335803642));
#30695=CARTESIAN_POINT('Ctrl Pts',(-21.5671817964434,-33.8333538619715,
-9.12349227713591));
#30696=CARTESIAN_POINT('Ctrl Pts',(-22.8443778274613,-36.285996273475,-11.8775764776334));
#30697=CARTESIAN_POINT('Ctrl Pts',(-23.6269831007732,-37.727394052712,-12.9726927515238));
#30698=CARTESIAN_POINT('Ctrl Pts',(-25.36537641937,-40.9068275275002,-14.4683433355123));
#30699=CARTESIAN_POINT('Ctrl Pts',(-26.3064386089277,-42.5943534697001,
-14.8498038985575));
#30700=CARTESIAN_POINT('Ctrl Pts',(-27.2516566664768,-44.2988917118188,
-14.8500516281494));
#30701=CARTESIAN_POINT('Ctrl Pts',(-21.5675617135469,-31.1202396243798,
1.59674381934691));
#30702=CARTESIAN_POINT('Ctrl Pts',(-21.5209893482663,-31.122412665213,1.15301435964159));
#30703=CARTESIAN_POINT('Ctrl Pts',(-21.4633832296834,-31.1157607261045,
0.635579189041325));
#30704=CARTESIAN_POINT('Ctrl Pts',(-21.3200195091683,-31.2068426510793,
-1.86860431099046));
#30705=CARTESIAN_POINT('Ctrl Pts',(-21.4172046993669,-31.5813261451459,
-3.70979114471806));
#30706=CARTESIAN_POINT('Ctrl Pts',(-21.9749346553982,-32.9219916749607,
-7.17014261467751));
#30707=CARTESIAN_POINT('Ctrl Pts',(-22.4407105406403,-33.8714586745724,
-8.7367057447581));
#30708=CARTESIAN_POINT('Ctrl Pts',(-23.6544622808573,-36.2249030242154,
-11.3734544105068));
#30709=CARTESIAN_POINT('Ctrl Pts',(-24.399795252463,-37.6093693845273,-12.4221714958032));
#30710=CARTESIAN_POINT('Ctrl Pts',(-26.0548745076895,-40.6575436657269,
-13.8545909095822));
#30711=CARTESIAN_POINT('Ctrl Pts',(-26.9525808297975,-42.2789313088314,
-14.2195188100006));
#30712=CARTESIAN_POINT('Ctrl Pts',(-27.8526693689673,-43.9126516878552,
-14.2201291128082));
#30713=CARTESIAN_POINT('Ctrl Pts',(-19.4238236466309,-32.4262389885812,
0.));
#30714=CARTESIAN_POINT('Ctrl Pts',(-19.3175602025801,-32.4953140196741,
-1.86858636177345));
#30715=CARTESIAN_POINT('Ctrl Pts',(-19.4132791553027,-32.8675162010731,
-3.7102999586904));
#30716=CARTESIAN_POINT('Ctrl Pts',(-19.9726455811605,-34.2107277069995,
-7.1693624749449));
#30717=CARTESIAN_POINT('Ctrl Pts',(-20.4374176294115,-35.1586329709647,
-8.73699595768469));
#30718=CARTESIAN_POINT('Ctrl Pts',(-21.1062276306812,-36.4553678306274,
-10.1890856763522));
#30719=CARTESIAN_POINT('Ctrl Pts',(-21.1694051501835,-36.5772356450483,
-10.3203928635213));
#30720=CARTESIAN_POINT('Ctrl Pts',(-21.2339499719768,-36.7011717789787,
-10.4488603766065));
#30721=CARTESIAN_POINT('Ctrl Pts',(-21.4269965203142,-31.1388779521429,
1.60982338570648E-15));
#30722=CARTESIAN_POINT('Ctrl Pts',(-21.3200195091683,-31.2068426510793,
-1.86860431099046));
#30723=CARTESIAN_POINT('Ctrl Pts',(-21.4172046993669,-31.5813261451459,
-3.70979114471806));
#30724=CARTESIAN_POINT('Ctrl Pts',(-21.9749346553982,-32.9219916749607,
-7.17014261467751));
#30725=CARTESIAN_POINT('Ctrl Pts',(-22.4407105406403,-33.8714586745724,
-8.7367057447581));
#30726=CARTESIAN_POINT('Ctrl Pts',(-23.1127335196157,-35.1745000052626,
-10.1966053555706));
#30727=CARTESIAN_POINT('Ctrl Pts',(-23.1794761614793,-35.3032131351437,
-10.335023194225));
#30728=CARTESIAN_POINT('Ctrl Pts',(-23.2477447519538,-35.4342359672548,
-10.4702558450959));
#30729=CARTESIAN_POINT('Ctrl Pts',(-21.2519768052526,-39.2156436908076,
1.24689101061708));
#30730=CARTESIAN_POINT('Ctrl Pts',(-21.2013209149673,-39.2180072667115,
0.76425478003098));
#30731=CARTESIAN_POINT('Ctrl Pts',(-21.1532057605615,-39.2189297793998,
0.33294871411375));
#30732=CARTESIAN_POINT('Ctrl Pts',(-21.0158614972049,-39.3102413216955,
-0.978870002760954));
#30733=CARTESIAN_POINT('Ctrl Pts',(-21.0136870732031,-39.5446400894738,
-1.98783577086067));
#30734=CARTESIAN_POINT('Ctrl Pts',(-21.2163201815384,-40.3156627551842,
-3.80852727286451));
#30735=CARTESIAN_POINT('Ctrl Pts',(-21.4133857818753,-40.8582554869495,
-4.65544360718471));
#30736=CARTESIAN_POINT('Ctrl Pts',(-21.9593030415369,-42.1674955178372,
-6.04997283346917));
#30737=CARTESIAN_POINT('Ctrl Pts',(-22.3081680037039,-42.9462925343122,
-6.61832169913048));
#30738=CARTESIAN_POINT('Ctrl Pts',(-23.0872105665505,-44.6142260746701,
-7.36768403068697));
#30739=CARTESIAN_POINT('Ctrl Pts',(-23.5251300588757,-45.5338656769775,
-7.57138648679969));
#30740=CARTESIAN_POINT('Ctrl Pts',(-23.9494005117258,-46.4212082443697,
-7.56962581969477));
#30741=CARTESIAN_POINT('Ctrl Pts',(-21.1419034541628,-36.8491669828397,
1.35489339099702));
#30742=CARTESIAN_POINT('Ctrl Pts',(-21.0925068841194,-36.8514717995378,
0.884255638223336));
#30743=CARTESIAN_POINT('Ctrl Pts',(-21.0414705341173,-36.8500676110308,
0.426397004062705));
#30744=CARTESIAN_POINT('Ctrl Pts',(-20.9023665809131,-36.9414623772438,
-1.2536081950493));
#30745=CARTESIAN_POINT('Ctrl Pts',(-20.9307214264281,-37.2188814500692,
-2.51960912778008));
#30746=CARTESIAN_POINT('Ctrl Pts',(-21.2431739952357,-38.1660672051982,
-4.84647586784088));
#30747=CARTESIAN_POINT('Ctrl Pts',(-21.5231103629228,-38.8341364170915,
-5.91572199044039));
#30748=CARTESIAN_POINT('Ctrl Pts',(-22.275285042685,-40.4658735625616,-7.69376028694706));
#30749=CARTESIAN_POINT('Ctrl Pts',(-22.7465133961109,-41.4315988261922,
-8.41063186564328));
#30750=CARTESIAN_POINT('Ctrl Pts',(-23.7961349711067,-43.5258421132357,
-9.37059840612348));
#30751=CARTESIAN_POINT('Ctrl Pts',(-24.3759711161681,-44.662114427047,-9.62435378624255));
#30752=CARTESIAN_POINT('Ctrl Pts',(-24.947197055425,-45.7799392638235,-9.62320046360572));
#30753=CARTESIAN_POINT('Ctrl Pts',(-20.5719668778721,-34.5502037758217,
1.47293210467435));
#30754=CARTESIAN_POINT('Ctrl Pts',(-20.5239438427388,-34.5524445041313,
1.01538103753069));
#30755=CARTESIAN_POINT('Ctrl Pts',(-20.4697337816482,-34.5485225227141,
0.52858078608683));
#30756=CARTESIAN_POINT('Ctrl Pts',(-20.3289202010286,-34.6403421915222,
-1.55402875458901));
#30757=CARTESIAN_POINT('Ctrl Pts',(-20.3903296068154,-34.9642917998438,
-3.10121432122654));
#30758=CARTESIAN_POINT('Ctrl Pts',(-20.8232363201018,-36.1046821530358,
-5.9812914545177));
#30759=CARTESIAN_POINT('Ctrl Pts',(-21.1935661261691,-36.9096087088301,
-7.29389406574109));
#30760=CARTESIAN_POINT('Ctrl Pts',(-22.1713634554283,-38.8941211502923,
-9.49113593806581));
#30761=CARTESIAN_POINT('Ctrl Pts',(-22.7762621832877,-40.0640440126673,
-10.3708286017747));
#30762=CARTESIAN_POINT('Ctrl Pts',(-24.1219089894863,-42.6246857849748,
-11.5604045560678));
#30763=CARTESIAN_POINT('Ctrl Pts',(-24.8568545017496,-43.9976714499935,
-11.8694761541382));
#30764=CARTESIAN_POINT('Ctrl Pts',(-25.5887811923514,-45.3675918458117,
-11.8687142284814));
#30765=CARTESIAN_POINT('Ctrl Pts',(-19.5640700378121,-32.4071044310925,
1.59647086199751));
#30766=CARTESIAN_POINT('Ctrl Pts',(-19.5174819665884,-32.4092782047833,
1.15259176011195));
#30767=CARTESIAN_POINT('Ctrl Pts',(-19.4599676462981,-32.4027440988463,
0.635573083870355));
#30768=CARTESIAN_POINT('Ctrl Pts',(-19.3175602025801,-32.4953140196741,
-1.86858636177345));
#30769=CARTESIAN_POINT('Ctrl Pts',(-19.4132791553027,-32.8675162010731,
-3.7102999586904));
#30770=CARTESIAN_POINT('Ctrl Pts',(-19.9726455811605,-34.2107277069995,
-7.1693624749449));
#30771=CARTESIAN_POINT('Ctrl Pts',(-20.4374176294115,-35.1586329709647,
-8.73699595768469));
#30772=CARTESIAN_POINT('Ctrl Pts',(-21.6515320408422,-37.5126415502804,
-11.3730256982353));
#30773=CARTESIAN_POINT('Ctrl Pts',(-22.3962711037445,-38.8961839422044,
-12.423580519285));
#30774=CARTESIAN_POINT('Ctrl Pts',(-24.0520129553695,-41.9453890000319,
-13.8529470820976));
#30775=CARTESIAN_POINT('Ctrl Pts',(-24.9492907716337,-43.5660774805306,
-14.2204718556692));
#30776=CARTESIAN_POINT('Ctrl Pts',(-25.8494965077556,-45.2000127177928,
-14.2198708430668));
#30777=CARTESIAN_POINT('Ctrl Pts',(-21.5675617135469,-31.1202396243798,
1.59674381934691));
#30778=CARTESIAN_POINT('Ctrl Pts',(-21.5209893482663,-31.122412665213,1.15301435964159));
#30779=CARTESIAN_POINT('Ctrl Pts',(-21.4633832296834,-31.1157607261045,
0.635579189041325));
#30780=CARTESIAN_POINT('Ctrl Pts',(-21.3200195091683,-31.2068426510793,
-1.86860431099046));
#30781=CARTESIAN_POINT('Ctrl Pts',(-21.4172046993669,-31.5813261451459,
-3.70979114471806));
#30782=CARTESIAN_POINT('Ctrl Pts',(-21.9749346553982,-32.9219916749607,
-7.17014261467751));
#30783=CARTESIAN_POINT('Ctrl Pts',(-22.4407105406403,-33.8714586745724,
-8.7367057447581));
#30784=CARTESIAN_POINT('Ctrl Pts',(-23.6544622808573,-36.2249030242154,
-11.3734544105068));
#30785=CARTESIAN_POINT('Ctrl Pts',(-24.399795252463,-37.6093693845273,-12.4221714958032));
#30786=CARTESIAN_POINT('Ctrl Pts',(-26.0548745076895,-40.6575436657269,
-13.8545909095822));
#30787=CARTESIAN_POINT('Ctrl Pts',(-26.9525808297975,-42.2789313088314,
-14.2195188100006));
#30788=CARTESIAN_POINT('Ctrl Pts',(-27.8526693689673,-43.9126516878552,
-14.2201291128082));
#30789=CARTESIAN_POINT('Ctrl Pts',(-23.0974263782807,-32.9280732767459,
1.47327617534837));
#30790=CARTESIAN_POINT('Ctrl Pts',(-23.0494231409448,-32.9303130812748,
1.01591373652303));
#30791=CARTESIAN_POINT('Ctrl Pts',(-22.9950973654386,-32.9262425677154,
0.528588481832317));
#30792=CARTESIAN_POINT('Ctrl Pts',(-22.8530783701147,-33.0161865744793,
-1.55405138009885));
#30793=CARTESIAN_POINT('Ctrl Pts',(-22.9163360108656,-33.3430118437433,
-3.10057294642025));
#30794=CARTESIAN_POINT('Ctrl Pts',(-23.3471799063629,-34.4801929200436,
-5.98227484333246));
#30795=CARTESIAN_POINT('Ctrl Pts',(-23.7187750781387,-35.2870880890182,
-7.29352824390976));
#30796=CARTESIAN_POINT('Ctrl Pts',(-24.6961152497918,-37.270889302571,-9.4916763423477));
#30797=CARTESIAN_POINT('Ctrl Pts',(-25.3017626168359,-38.4419768539591,
-10.3690524867152));
#30798=CARTESIAN_POINT('Ctrl Pts',(-26.6465742010127,-41.0013193023666,
-11.5624766483988));
#30799=CARTESIAN_POINT('Ctrl Pts',(-27.3820564590795,-42.3751889385656,
-11.8682745706114));
#30800=CARTESIAN_POINT('Ctrl Pts',(-28.1138388177854,-43.7448358429353,
-11.8690397849985));
#30801=CARTESIAN_POINT('Ctrl Pts',(-24.9511692381919,-34.4024335442871,
1.35541236849225));
#30802=CARTESIAN_POINT('Ctrl Pts',(-24.9018025300712,-34.4047369675988,
0.885059132416527));
#30803=CARTESIAN_POINT('Ctrl Pts',(-24.8505916427358,-34.4031087412849,
0.42640861190673));
#30804=CARTESIAN_POINT('Ctrl Pts',(-24.7096695075361,-34.4916743608874,
-1.25364232213804));
#30805=CARTESIAN_POINT('Ctrl Pts',(-24.7408121301759,-34.7734309242996,
-2.51864171290121));
#30806=CARTESIAN_POINT('Ctrl Pts',(-25.0501532567909,-35.715775980658,-4.84795915805251));
#30807=CARTESIAN_POINT('Ctrl Pts',(-25.3319982333056,-36.3868145416348,
-5.91517020468245));
#30808=CARTESIAN_POINT('Ctrl Pts',(-26.0834833614037,-38.0174789095995,
-7.6945754033802));
#30809=CARTESIAN_POINT('Ctrl Pts',(-26.5558409214639,-38.9849609268016,
-8.40795287026731));
#30810=CARTESIAN_POINT('Ctrl Pts',(-27.604202692975,-41.0772443843362,-9.37372383752152));
#30811=CARTESIAN_POINT('Ctrl Pts',(-28.184840983779,-42.2148554923143,-9.62254086005825));
#30812=CARTESIAN_POINT('Ctrl Pts',(-28.7558566730951,-43.3322623493511,
-9.62369151535353));
#30813=CARTESIAN_POINT('Ctrl Pts',(-27.0575499832998,-35.4866599889491,
1.24768196666929));
#30814=CARTESIAN_POINT('Ctrl Pts',(-27.0069396045581,-35.489021441235,0.765479358362176));
#30815=CARTESIAN_POINT('Ctrl Pts',(-26.9585584437084,-35.489602505485,0.332966405236331));
#30816=CARTESIAN_POINT('Ctrl Pts',(-26.8184431506468,-35.5766022410826,
-0.978922014702958));
#30817=CARTESIAN_POINT('Ctrl Pts',(-26.8205174834931,-35.8176116315986,
-1.98636136655743));
#30818=CARTESIAN_POINT('Ctrl Pts',(-27.0184085480051,-36.5812567520118,
-3.81078790531902));
#30819=CARTESIAN_POINT('Ctrl Pts',(-27.2183829945192,-37.1283749683008,
-4.65460264917133));
#30820=CARTESIAN_POINT('Ctrl Pts',(-27.7632493317924,-38.4359800152694,
-6.05121512486059));
#30821=CARTESIAN_POINT('Ctrl Pts',(-28.1138352796158,-39.217454440471,-6.61423873286722));
#30822=CARTESIAN_POINT('Ctrl Pts',(-28.8909578185681,-40.8824010709202,
-7.37244739499603));
#30823=CARTESIAN_POINT('Ctrl Pts',(-29.3300828959493,-41.8040923655683,
-7.56862230180927));
#30824=CARTESIAN_POINT('Ctrl Pts',(-29.7540498521217,-42.6907866227636,
-7.57037421505956));
#30825=CARTESIAN_POINT('Ctrl Pts',(-23.9769478445537,-29.2929893708798,
1.59647090706393));
#30826=CARTESIAN_POINT('Ctrl Pts',(-23.9311433315013,-29.3017711927832,
1.15259179089974));
#30827=CARTESIAN_POINT('Ctrl Pts',(-23.8732845217115,-29.3034887354924,
0.635573104333306));
#30828=CARTESIAN_POINT('Ctrl Pts',(-23.7455006526456,-29.4153831213402,
-1.86858636180619));
#30829=CARTESIAN_POINT('Ctrl Pts',(-23.8932152178165,-29.7701745937408,
-3.71029995872295));
#30830=CARTESIAN_POINT('Ctrl Pts',(-24.6380470280763,-31.0201080010757,
-7.16936247491227));
#30831=CARTESIAN_POINT('Ctrl Pts',(-25.2329893514594,-31.8922209971881,
-8.73699595769179));
#30832=CARTESIAN_POINT('Ctrl Pts',(-26.769756179009,-34.049482667342,-11.373025698228));
#30833=CARTESIAN_POINT('Ctrl Pts',(-27.7038134837039,-35.3129551734355,
-12.4235805192132));
#30834=CARTESIAN_POINT('Ctrl Pts',(-29.7766493956151,-38.0954870862277,
-13.8529470821691));
#30835=CARTESIAN_POINT('Ctrl Pts',(-30.8954422365109,-39.5719833475712,
-14.2204718557357));
#30836=CARTESIAN_POINT('Ctrl Pts',(-32.0190184050856,-41.0611748464153,
-14.2198708430667));
#30837=CARTESIAN_POINT('Ctrl Pts',(-24.1050578112643,-28.3497570418624,
1.62964634867152));
#30838=CARTESIAN_POINT('Ctrl Pts',(-24.0596354334582,-28.3584655992883,
1.18947040157868));
#30839=CARTESIAN_POINT('Ctrl Pts',(-24.0007720917085,-28.3595888789067,
0.664244065133585));
#30840=CARTESIAN_POINT('Ctrl Pts',(-23.8722870320922,-28.4713886672088,
-1.95287905129543));
#30841=CARTESIAN_POINT('Ctrl Pts',(-24.0314123849458,-28.8382130746034,
-3.87337387080275));
#30842=CARTESIAN_POINT('Ctrl Pts',(-24.8169940395268,-30.1365118994154,
-7.48792130212306));
#30843=CARTESIAN_POINT('Ctrl Pts',(-25.442759955772,-31.043317523795,-9.1236083623051));
#30844=CARTESIAN_POINT('Ctrl Pts',(-27.0561790920293,-33.2894343746864,
-11.8774049927261));
#30845=CARTESIAN_POINT('Ctrl Pts',(-28.0356631205829,-34.6044524433959,
-12.9732563608822));
#30846=CARTESIAN_POINT('Ctrl Pts',(-30.2091636816484,-37.5044951004748,
-14.4676858045526));
#30847=CARTESIAN_POINT('Ctrl Pts',(-31.3805975394681,-39.0406651371313,
-14.8501851005579));
#30848=CARTESIAN_POINT('Ctrl Pts',(-32.5588345556906,-40.5934132658116,
-14.8499483202528));
#30849=CARTESIAN_POINT('Ctrl Pts',(-24.8250414362345,-27.7261998529423,
1.62975553161129));
#30850=CARTESIAN_POINT('Ctrl Pts',(-24.7796252351427,-27.7349072261465,
1.18963944139595));
#30851=CARTESIAN_POINT('Ctrl Pts',(-24.7207188400697,-27.7359890779444,
0.664246507200263));
#30852=CARTESIAN_POINT('Ctrl Pts',(-24.5917704575631,-27.8472541630956,
-1.95288623097697));
#30853=CARTESIAN_POINT('Ctrl Pts',(-24.7516062016228,-28.2148983404681,
-3.87317034519611));
#30854=CARTESIAN_POINT('Ctrl Pts',(-25.5363949989286,-29.512282298103,-7.48823335803388));
#30855=CARTESIAN_POINT('Ctrl Pts',(-26.1626472662077,-30.4196491139262,
-9.12349227712643));
#30856=CARTESIAN_POINT('Ctrl Pts',(-27.7758906912596,-32.6655632155557,
-11.8775764776429));
#30857=CARTESIAN_POINT('Ctrl Pts',(-28.7556624629977,-33.9809133009309,
-12.9726927515337));
#30858=CARTESIAN_POINT('Ctrl Pts',(-30.9288420053122,-36.8805855630443,
-14.4683433355025));
#30859=CARTESIAN_POINT('Ctrl Pts',(-32.1004855202296,-38.4170078110375,
-14.8498038985243));
#30860=CARTESIAN_POINT('Ctrl Pts',(-33.2786637049092,-39.9696777567513,
-14.8500516281495));
#30861=CARTESIAN_POINT('Ctrl Pts',(-25.7769069069791,-27.7340963985796,
1.59674386441336));
#30862=CARTESIAN_POINT('Ctrl Pts',(-25.7311178357117,-27.7428752599244,
1.15301439044302));
#30863=CARTESIAN_POINT('Ctrl Pts',(-25.6731513926139,-27.7444892330898,
0.635579209500005));
#30864=CARTESIAN_POINT('Ctrl Pts',(-25.5442092163241,-27.8550468610477,
-1.86860431101006));
#30865=CARTESIAN_POINT('Ctrl Pts',(-25.693699759515,-28.2118877583881,-3.70979114470276));
#30866=CARTESIAN_POINT('Ctrl Pts',(-26.4365494265749,-29.4595339978089,
-7.17014261469294));
#30867=CARTESIAN_POINT('Ctrl Pts',(-27.0327076275534,-30.3330499725233,
-8.73670574474391));
#30868=CARTESIAN_POINT('Ctrl Pts',(-28.56903517708,-32.4898047695082,-11.3734544105212));
#30869=CARTESIAN_POINT('Ctrl Pts',(-29.5038118397362,-33.7541073172778,
-12.4221714958516));
#30870=CARTESIAN_POINT('Ctrl Pts',(-31.5758452047796,-36.5357132426467,
-13.8545909095341));
#30871=CARTESIAN_POINT('Ctrl Pts',(-32.695161691107,-38.0128405673125,-14.2195188099342));
#30872=CARTESIAN_POINT('Ctrl Pts',(-33.818591278132,-39.5018360737644,-14.2201291128083));
#30873=CARTESIAN_POINT('Ctrl Pts',(-23.84085208622,-29.3318883095341,0.));
#30874=CARTESIAN_POINT('Ctrl Pts',(-23.7455006526456,-29.4153831213402,
-1.86858636180619));
#30875=CARTESIAN_POINT('Ctrl Pts',(-23.8932152178166,-29.7701745937408,
-3.71029995872415));
#30876=CARTESIAN_POINT('Ctrl Pts',(-24.6380470280763,-31.0201080010757,
-7.16936247491107));
#30877=CARTESIAN_POINT('Ctrl Pts',(-25.2329893514618,-31.8922209971881,
-8.7369959576894));
#30878=CARTESIAN_POINT('Ctrl Pts',(-26.079536443074,-33.0805753785961,-10.1890856763512));
#30879=CARTESIAN_POINT('Ctrl Pts',(-26.1594145048188,-33.1922116559192,
-10.3203928635188));
#30880=CARTESIAN_POINT('Ctrl Pts',(-26.2409403042445,-33.3057006128373,
-10.4488603766022));
#30881=CARTESIAN_POINT('Ctrl Pts',(-25.6404249706859,-27.7725495286737,
1.99840144432528E-15));
#30882=CARTESIAN_POINT('Ctrl Pts',(-25.5442092163241,-27.8550468610477,
-1.86860431101006));
#30883=CARTESIAN_POINT('Ctrl Pts',(-25.693699759515,-28.2118877583881,-3.70979114470276));
#30884=CARTESIAN_POINT('Ctrl Pts',(-26.4365494265749,-29.4595339978089,
-7.17014261469294));
#30885=CARTESIAN_POINT('Ctrl Pts',(-27.0327076275534,-30.3330499725233,
-8.73670574474391));
#30886=CARTESIAN_POINT('Ctrl Pts',(-27.8833324977841,-31.5271893797546,
-10.1966053555717));
#30887=CARTESIAN_POINT('Ctrl Pts',(-27.9677135840461,-31.6450939272826,
-10.3350231942274));
#30888=CARTESIAN_POINT('Ctrl Pts',(-28.0539337918609,-31.7650675024727,
-10.4702558450997));
#30889=CARTESIAN_POINT('Ctrl Pts',(-26.6166303184857,-35.7920133394054,
1.24689105568337));
#30890=CARTESIAN_POINT('Ctrl Pts',(-26.5668264024408,-35.8015619426292,
0.764254809540774));
#30891=CARTESIAN_POINT('Ctrl Pts',(-26.5193322761002,-35.8093225655935,
0.332948724830941));
#30892=CARTESIAN_POINT('Ctrl Pts',(-26.396380965813,-35.9192508155956,-0.978870002770901));
#30893=CARTESIAN_POINT('Ctrl Pts',(-26.4275870967871,-36.1515731946737,
-1.98783577092234));
#30894=CARTESIAN_POINT('Ctrl Pts',(-26.7378856585374,-36.8859102633355,
-3.80852727280253));
#30895=CARTESIAN_POINT('Ctrl Pts',(-27.0101644118782,-37.3949348243987,
-4.6554436072131));
#30896=CARTESIAN_POINT('Ctrl Pts',(-27.73684930433,-38.6131565530251,-6.0499728334401));
#30897=CARTESIAN_POINT('Ctrl Pts',(-28.1929976957773,-39.3343778781062,
-6.61832169896238));
#30898=CARTESIAN_POINT('Ctrl Pts',(-29.2014824203258,-40.8744649436983,
-7.36768403085421));
#30899=CARTESIAN_POINT('Ctrl Pts',(-29.7658228849728,-41.7224214992554,
-7.57138648700874));
#30900=CARTESIAN_POINT('Ctrl Pts',(-30.3120568904485,-42.5403522177284,
-7.56962581969447));
#30901=CARTESIAN_POINT('Ctrl Pts',(-26.1708926054254,-33.4652890233054,
1.35489343606335));
#30902=CARTESIAN_POINT('Ctrl Pts',(-26.1223268292952,-33.4746002454545,
0.884255668130519));
#30903=CARTESIAN_POINT('Ctrl Pts',(-26.0716101167996,-33.4804735791548,
0.4263970177884));
#30904=CARTESIAN_POINT('Ctrl Pts',(-25.94692887169,-33.5907346359716,-1.25360819506359));
#30905=CARTESIAN_POINT('Ctrl Pts',(-26.014475956126,-33.8612946673281,-2.51960912782488));
#30906=CARTESIAN_POINT('Ctrl Pts',(-26.4585467959957,-34.7543728004604,
-4.84647586779589));
#30907=CARTESIAN_POINT('Ctrl Pts',(-26.8307099768485,-35.3758029321247,
-5.91572199045934));
#30908=CARTESIAN_POINT('Ctrl Pts',(-27.8074490109262,-36.8838857283296,
-7.69376028692768));
#30909=CARTESIAN_POINT('Ctrl Pts',(-28.4113179739206,-37.7727185143413,
-8.41063186552333));
#30910=CARTESIAN_POINT('Ctrl Pts',(-29.7482978092831,-39.6962686996464,
-9.37059840624287));
#30911=CARTESIAN_POINT('Ctrl Pts',(-30.4839404690738,-40.7384561125312,
-9.62435378637076));
#30912=CARTESIAN_POINT('Ctrl Pts',(-31.2084352127804,-41.7636091770246,
-9.62320046360554));
#30913=CARTESIAN_POINT('Ctrl Pts',(-25.2795805846978,-31.2708363785845,
1.47293214974073));
#30914=CARTESIAN_POINT('Ctrl Pts',(-25.232365242191,-31.2798886902734,1.01538106786938));
#30915=CARTESIAN_POINT('Ctrl Pts',(-25.1781488031009,-31.2837215247365,
0.528580803103268));
#30916=CARTESIAN_POINT('Ctrl Pts',(-25.0518358019867,-31.394646464622,-1.554028754611));
#30917=CARTESIAN_POINT('Ctrl Pts',(-25.1587229846876,-31.7065592632734,
-3.10121432126163));
#30918=CARTESIAN_POINT('Ctrl Pts',(-25.7495178005009,-32.7737330382101,
-5.98129145448249));
#30919=CARTESIAN_POINT('Ctrl Pts',(-26.2306311757314,-33.5177631757313,
-7.29389406574815));
#30920=CARTESIAN_POINT('Ctrl Pts',(-27.4809015052032,-35.3429210732409,
-9.49113593805845));
#30921=CARTESIAN_POINT('Ctrl Pts',(-28.2461406191133,-36.4148497431898,
-10.3708286016981));
#30922=CARTESIAN_POINT('Ctrl Pts',(-29.9425080008753,-38.7579223666493,
-11.560404556144));
#30923=CARTESIAN_POINT('Ctrl Pts',(-30.8653690604188,-40.0123393656214,
-11.8694761542094));
#30924=CARTESIAN_POINT('Ctrl Pts',(-31.784805792174,-41.2641519184871,-11.8687142284813));
#30925=CARTESIAN_POINT('Ctrl Pts',(-23.9769478445537,-29.2929893708798,
1.59647090706393));
#30926=CARTESIAN_POINT('Ctrl Pts',(-23.9311433315013,-29.3017711927832,
1.15259179089975));
#30927=CARTESIAN_POINT('Ctrl Pts',(-23.8732845217115,-29.3034887354924,
0.635573104333306));
#30928=CARTESIAN_POINT('Ctrl Pts',(-23.7455006526456,-29.4153831213402,
-1.86858636180619));
#30929=CARTESIAN_POINT('Ctrl Pts',(-23.8932152178166,-29.7701745937408,
-3.71029995872415));
#30930=CARTESIAN_POINT('Ctrl Pts',(-24.6380470280763,-31.0201080010757,
-7.16936247491107));
#30931=CARTESIAN_POINT('Ctrl Pts',(-25.2329893514618,-31.8922209971881,
-8.7369959576894));
#30932=CARTESIAN_POINT('Ctrl Pts',(-26.7697561790066,-34.049482667342,-11.3730256982303));
#30933=CARTESIAN_POINT('Ctrl Pts',(-27.7038134837062,-35.3129551734307,
-12.423580519218));
#30934=CARTESIAN_POINT('Ctrl Pts',(-29.7766493956127,-38.0954870862325,
-13.8529470821643));
#30935=CARTESIAN_POINT('Ctrl Pts',(-30.8954422365098,-39.5719833475698,
-14.2204718557357));
#30936=CARTESIAN_POINT('Ctrl Pts',(-32.0190184050856,-41.0611748464153,
-14.2198708430667));
#30937=CARTESIAN_POINT('Ctrl Pts',(-25.7769069069791,-27.7340963985796,
1.59674386441336));
#30938=CARTESIAN_POINT('Ctrl Pts',(-25.7311178357117,-27.7428752599244,
1.15301439044302));
#30939=CARTESIAN_POINT('Ctrl Pts',(-25.6731513926139,-27.7444892330898,
0.635579209500005));
#30940=CARTESIAN_POINT('Ctrl Pts',(-25.5442092163241,-27.8550468610477,
-1.86860431101006));
#30941=CARTESIAN_POINT('Ctrl Pts',(-25.693699759515,-28.2118877583881,-3.70979114470396));
#30942=CARTESIAN_POINT('Ctrl Pts',(-26.4365494265749,-29.4595339978089,
-7.17014261469174));
#30943=CARTESIAN_POINT('Ctrl Pts',(-27.0327076275534,-30.3330499725233,
-8.73670574474391));
#30944=CARTESIAN_POINT('Ctrl Pts',(-28.56903517708,-32.4898047695081,-11.3734544105212));
#30945=CARTESIAN_POINT('Ctrl Pts',(-29.5038118397362,-33.7541073172778,
-12.4221714958564));
#30946=CARTESIAN_POINT('Ctrl Pts',(-31.5758452047796,-36.5357132426467,
-13.8545909095293));
#30947=CARTESIAN_POINT('Ctrl Pts',(-32.6951616911162,-38.0128405673056,
-14.2195188099294));
#30948=CARTESIAN_POINT('Ctrl Pts',(-33.818591278132,-39.5018360737644,-14.2201291128083));
#30949=CARTESIAN_POINT('Ctrl Pts',(-27.54848130917,-29.3058064687039,1.47327622041477));
#30950=CARTESIAN_POINT('Ctrl Pts',(-27.5012854314845,-29.3148550485271,
1.01591376687878));
#30951=CARTESIAN_POINT('Ctrl Pts',(-27.4469333174786,-29.3185573305633,
0.528588498843375));
#30952=CARTESIAN_POINT('Ctrl Pts',(-27.3191602364347,-29.4277972482744,
-1.55405138010428));
#30953=CARTESIAN_POINT('Ctrl Pts',(-27.428286091058,-29.7422934066342,-3.10057294639553));
#30954=CARTESIAN_POINT('Ctrl Pts',(-28.0165823577485,-30.8065841399291,
-5.98227484335734));
#30955=CARTESIAN_POINT('Ctrl Pts',(-28.4992283820293,-31.5523827727592,
-7.29352824389559));
#30956=CARTESIAN_POINT('Ctrl Pts',(-29.7489449887903,-33.3769017419095,
-9.49167634236217));
#30957=CARTESIAN_POINT('Ctrl Pts',(-30.5150908743223,-34.449876703528,-10.3690524867828));
#30958=CARTESIAN_POINT('Ctrl Pts',(-32.2104466224207,-36.7917820929022,
-11.5624766483316));
#30959=CARTESIAN_POINT('Ctrl Pts',(-33.1339647666498,-38.0469976785157,
-11.8682745705117));
#30960=CARTESIAN_POINT('Ctrl Pts',(-34.0532197137071,-39.2985600643047,
-11.8690397849987));
#30961=CARTESIAN_POINT('Ctrl Pts',(-29.5931790826754,-30.5013447592651,
1.35541241355862));
#30962=CARTESIAN_POINT('Ctrl Pts',(-29.5446426662248,-30.5106503524655,
0.885059162349651));
#30963=CARTESIAN_POINT('Ctrl Pts',(-29.4937213090619,-30.5163267679905,
0.426408625624299));
#30964=CARTESIAN_POINT('Ctrl Pts',(-29.3668377587822,-30.6240462289814,
-1.25364232212737));
#30965=CARTESIAN_POINT('Ctrl Pts',(-29.4377615342147,-30.8985028596602,
-2.5186417128575));
#30966=CARTESIAN_POINT('Ctrl Pts',(-29.8780636984474,-31.7872323695308,
-4.84795915809644));
#30967=CARTESIAN_POINT('Ctrl Pts',(-30.2525386437904,-32.4113300033621,
-5.91517020466357));
#30968=CARTESIAN_POINT('Ctrl Pts',(-31.2284424726378,-33.918449074776,-7.69457540339954));
#30969=CARTESIAN_POINT('Ctrl Pts',(-31.8336791606395,-34.8088600302412,
-8.40795287037808));
#30970=CARTESIAN_POINT('Ctrl Pts',(-33.1691331027958,-36.7306496231332,
-9.3737238374113));
#30971=CARTESIAN_POINT('Ctrl Pts',(-33.9057602738009,-37.7740480458484,
-9.6225408599538));
#30972=CARTESIAN_POINT('Ctrl Pts',(-34.6299874229479,-38.7988173067562,
-9.62369151535372));
#30973=CARTESIAN_POINT('Ctrl Pts',(-31.8324214200721,-31.2747661069639,
1.24768201173563));
#30974=CARTESIAN_POINT('Ctrl Pts',(-31.7826622501122,-31.2843061312878,
0.765479387912171));
#30975=CARTESIAN_POINT('Ctrl Pts',(-31.7348562317659,-31.2917666379301,
0.33296641594115));
#30976=CARTESIAN_POINT('Ctrl Pts',(-31.6085484626271,-31.3978213276697,
-0.978922014674862));
#30977=CARTESIAN_POINT('Ctrl Pts',(-31.6449008941757,-31.6360823820121,
-1.98636136648275));
#30978=CARTESIAN_POINT('Ctrl Pts',(-31.9494557448252,-32.3637918610199,
-3.81078790539403));
#30979=CARTESIAN_POINT('Ctrl Pts',(-32.2252577802593,-32.8768818719414,
-4.65460264913821));
#30980=CARTESIAN_POINT('Ctrl Pts',(-32.9506697646498,-34.0936348201774,
-6.05121512489441));
#30981=CARTESIAN_POINT('Ctrl Pts',(-33.4089026595357,-34.8172613799685,
-6.61423873304044));
#30982=CARTESIAN_POINT('Ctrl Pts',(-34.4150618218505,-36.3546651862003,
-7.37244739482366));
#30983=CARTESIAN_POINT('Ctrl Pts',(-34.9808875865548,-37.2044809779807,
-7.56862230162397));
#30984=CARTESIAN_POINT('Ctrl Pts',(-35.5267289204024,-38.021813177295,-7.57037421505986));
#30985=CARTESIAN_POINT('Ctrl Pts',(-27.9017241322579,-25.5825535213024,
1.59647090706389));
#30986=CARTESIAN_POINT('Ctrl Pts',(-27.8576356266559,-25.5977646187898,
1.15259179090242));
#30987=CARTESIAN_POINT('Ctrl Pts',(-27.8006101679571,-25.6076988465251,
0.635573104329219));
#30988=CARTESIAN_POINT('Ctrl Pts',(-27.6900511858225,-25.7366398496109,
-1.86858636179435));
#30989=CARTESIAN_POINT('Ctrl Pts',(-27.8867543207323,-26.0667980818921,
-3.71029995871567));
#30990=CARTESIAN_POINT('Ctrl Pts',(-28.8018888878676,-27.1980083507359,
-7.1693624749194));
#30991=CARTESIAN_POINT('Ctrl Pts',(-29.5148901762754,-27.9765753734451,
-8.73699595772763));
#30992=CARTESIAN_POINT('Ctrl Pts',(-31.3430252789425,-29.89317450793,-11.373025698192));
#30993=CARTESIAN_POINT('Ctrl Pts',(-32.4473861124854,-31.0108564714034,
-12.4235805192132));
#30994=CARTESIAN_POINT('Ctrl Pts',(-34.8951191227831,-33.4700709137458,
-13.852947082169));
#30995=CARTESIAN_POINT('Ctrl Pts',(-36.2126515924275,-34.7723177498595,
-14.2204718557594));
#30996=CARTESIAN_POINT('Ctrl Pts',(-37.5367254229125,-36.0864498658149,
-14.2198708430666));
#30997=CARTESIAN_POINT('Ctrl Pts',(-27.8942941678685,-24.6306899881721,
1.62964634867148));
#30998=CARTESIAN_POINT('Ctrl Pts',(-27.8505734813071,-24.6457741833911,
1.18947040157796));
#30999=CARTESIAN_POINT('Ctrl Pts',(-27.7924691428838,-24.655263156583,0.664244065133));
#31000=CARTESIAN_POINT('Ctrl Pts',(-27.6812026446472,-24.7842103148066,
-1.95287905129388));
#31001=CARTESIAN_POINT('Ctrl Pts',(-27.8909128870847,-25.1246550797521,
-3.87337387080265));
#31002=CARTESIAN_POINT('Ctrl Pts',(-28.8532656404615,-26.2979391683561,
-7.48792130212299));
#31003=CARTESIAN_POINT('Ctrl Pts',(-29.6017140577926,-27.1064590437618,
-9.12360836233377));
#31004=CARTESIAN_POINT('Ctrl Pts',(-31.518366669829,-29.1001001804546,-11.8774049926974));
#31005=CARTESIAN_POINT('Ctrl Pts',(-32.6750275470923,-30.2623381501783,
-12.9732563608822));
#31006=CARTESIAN_POINT('Ctrl Pts',(-35.23912410816,-32.8235411735974,-14.4676858045526));
#31007=CARTESIAN_POINT('Ctrl Pts',(-36.6172542487524,-34.1773627942107,
-14.8501851005579));
#31008=CARTESIAN_POINT('Ctrl Pts',(-38.0044776097608,-35.5466255754746,
-14.8499483202528));
#31009=CARTESIAN_POINT('Ctrl Pts',(-28.5182079571718,-23.9110153591929,
1.62975553161125));
#31010=CARTESIAN_POINT('Ctrl Pts',(-28.4744932159222,-23.9260975032042,
1.18963944139177));
#31011=CARTESIAN_POINT('Ctrl Pts',(-28.4163403666074,-23.9355515973836,
0.664246507203993));
#31012=CARTESIAN_POINT('Ctrl Pts',(-28.3045391652295,-24.0640354326691,
-1.95288623098812));
#31013=CARTESIAN_POINT('Ctrl Pts',(-28.5150692335544,-24.4051905243133,
-3.87317034520081));
#31014=CARTESIAN_POINT('Ctrl Pts',(-29.4765070006364,-25.577681893135,-7.48823335802902));
#31015=CARTESIAN_POINT('Ctrl Pts',(-30.225516684522,-26.3866880329016,-9.12349227713835));
#31016=CARTESIAN_POINT('Ctrl Pts',(-32.1419665195937,-28.3801534903166,
-11.877576477631));
#31017=CARTESIAN_POINT('Ctrl Pts',(-33.2989594621267,-29.5426791471387,
-12.9726927515433));
#31018=CARTESIAN_POINT('Ctrl Pts',(-35.8626855592739,-32.1035612314167,
-14.4683433354929));
#31019=CARTESIAN_POINT('Ctrl Pts',(-37.2410591163492,-33.4576026589017,
-14.849803898491));
#31020=CARTESIAN_POINT('Ctrl Pts',(-38.628213118051,-34.8267964255887,-14.8500516281495));
#31021=CARTESIAN_POINT('Ctrl Pts',(-29.4615086055162,-23.7833669488545,
1.5967438644133));
#31022=CARTESIAN_POINT('Ctrl Pts',(-29.4174349631938,-23.7985729183137,
1.15301439043676));
#31023=CARTESIAN_POINT('Ctrl Pts',(-29.3602882272664,-23.8084199485298,
0.635579209506715));
#31024=CARTESIAN_POINT('Ctrl Pts',(-29.248392487277,-23.9362026442577,-1.86860431102996));
#31025=CARTESIAN_POINT('Ctrl Pts',(-29.4471451869125,-24.2681366932806,
-3.70979114471347));
#31026=CARTESIAN_POINT('Ctrl Pts',(-30.3599922882989,-25.3973651626973,
-7.17014261468209));
#31027=CARTESIAN_POINT('Ctrl Pts',(-31.0743967431037,-26.1771478462935,
-8.73670574474148));
#31028=CARTESIAN_POINT('Ctrl Pts',(-32.9020249033495,-28.0933077825863,
-11.3734544105236));
#31029=CARTESIAN_POINT('Ctrl Pts',(-34.0072159000762,-29.2117089638021,
-12.4221714958708));
#31030=CARTESIAN_POINT('Ctrl Pts',(-36.454022750563,-31.6701210582965,-13.854590909515));
#31031=CARTESIAN_POINT('Ctrl Pts',(-37.7721633453332,-32.9729180118679,
-14.2195188098961));
#31032=CARTESIAN_POINT('Ctrl Pts',(-39.096064193638,-34.2868769911002,-14.2201291128084));
#31033=CARTESIAN_POINT('Ctrl Pts',(-27.7725495286738,-25.6404249706858,
0.));
#31034=CARTESIAN_POINT('Ctrl Pts',(-27.6900511858225,-25.7366398496109,
-1.86858636179435));
#31035=CARTESIAN_POINT('Ctrl Pts',(-27.8867543207323,-26.0667980818921,
-3.71029995871567));
#31036=CARTESIAN_POINT('Ctrl Pts',(-28.8018888878676,-27.1980083507359,
-7.1693624749194));
#31037=CARTESIAN_POINT('Ctrl Pts',(-29.5148901762754,-27.9765753734451,
-8.73699595772763));
#31038=CARTESIAN_POINT('Ctrl Pts',(-30.5219411006572,-29.0323578083627,
-10.1890856763484));
#31039=CARTESIAN_POINT('Ctrl Pts',(-30.6168936176569,-29.1314899559173,
-10.3203928635139));
#31040=CARTESIAN_POINT('Ctrl Pts',(-30.7137407645416,-29.2322214279374,
-10.4488603765957));
#31041=CARTESIAN_POINT('Ctrl Pts',(-29.3318883095342,-23.8408520862199,
1.11022302462516E-15));
#31042=CARTESIAN_POINT('Ctrl Pts',(-29.248392487277,-23.9362026442577,-1.86860431102996));
#31043=CARTESIAN_POINT('Ctrl Pts',(-29.4471451869125,-24.2681366932806,
-3.70979114471347));
#31044=CARTESIAN_POINT('Ctrl Pts',(-30.3599922882989,-25.3973651626973,
-7.17014261468209));
#31045=CARTESIAN_POINT('Ctrl Pts',(-31.0743967431037,-26.1771478462935,
-8.73670574474148));
#31046=CARTESIAN_POINT('Ctrl Pts',(-32.0863072351854,-27.2380760953858,
-10.1966053555729));
#31047=CARTESIAN_POINT('Ctrl Pts',(-32.1866090102636,-27.342771863985,-10.3350231942299));
#31048=CARTESIAN_POINT('Ctrl Pts',(-32.2890256406274,-27.4492538662409,
-10.4702558451036));
#31049=CARTESIAN_POINT('Ctrl Pts',(-31.4394459897279,-31.6397608122767,
1.24689105568322));
#31050=CARTESIAN_POINT('Ctrl Pts',(-31.3915079136553,-31.656300060737,0.764254809555862));
#31051=CARTESIAN_POINT('Ctrl Pts',(-31.3456016608202,-31.6707408106673,
0.332948724813886));
#31052=CARTESIAN_POINT('Ctrl Pts',(-31.2395462388184,-31.7970479454233,
-0.978870002720858));
#31053=CARTESIAN_POINT('Ctrl Pts',(-31.3034976581266,-32.0225645221647,
-1.9878357708888));
#31054=CARTESIAN_POINT('Ctrl Pts',(-31.7151448890446,-32.7052670087001,
-3.80852727283614));
#31055=CARTESIAN_POINT('Ctrl Pts',(-32.0570939852818,-33.1703611269164,
-4.65544360725139));
#31056=CARTESIAN_POINT('Ctrl Pts',(-32.9497533018099,-34.2727650719354,
-6.04997283340185));
#31057=CARTESIAN_POINT('Ctrl Pts',(-33.5038992565468,-34.9217287192801,
-6.61832169894314));
#31058=CARTESIAN_POINT('Ctrl Pts',(-34.7212963022536,-36.302617578697,-7.36768403087334));
#31059=CARTESIAN_POINT('Ctrl Pts',(-35.4005693948026,-37.0616291372609,
-7.57138648705137));
#31060=CARTESIAN_POINT('Ctrl Pts',(-36.0576472036355,-37.7934972961798,
-7.56962581969424));
#31061=CARTESIAN_POINT('Ctrl Pts',(-30.6671178491336,-29.4001542854017,
1.35489343606322));
#31062=CARTESIAN_POINT('Ctrl Pts',(-30.6203715276488,-29.4162823633143,
0.884255668139903));
#31063=CARTESIAN_POINT('Ctrl Pts',(-30.5710069006851,-29.4293136556735,
0.426397017777568));
#31064=CARTESIAN_POINT('Ctrl Pts',(-30.4632865153969,-29.5561964051703,
-1.25360819503185));
#31065=CARTESIAN_POINT('Ctrl Pts',(-30.5686507749895,-29.8143895731036,
-2.51960912780089));
#31066=CARTESIAN_POINT('Ctrl Pts',(-31.1352998840585,-30.6351795888068,
-4.84647586781987));
#31067=CARTESIAN_POINT('Ctrl Pts',(-31.5921137090052,-31.1973201148342,
-5.91572199048803));
#31068=CARTESIAN_POINT('Ctrl Pts',(-32.7735335073842,-32.5510483450287,
-7.69376028689897));
#31069=CARTESIAN_POINT('Ctrl Pts',(-33.4977500492304,-33.344894581048,-8.41063186551369));
#31070=CARTESIAN_POINT('Ctrl Pts',(-35.0948710910953,-35.0585937299339,
-9.37059840625243));
#31071=CARTESIAN_POINT('Ctrl Pts',(-35.9713447024848,-35.9854803115381,
-9.62435378641347));
#31072=CARTESIAN_POINT('Ctrl Pts',(-36.834359626899,-36.8970924436851,-9.62320046360538));
#31073=CARTESIAN_POINT('Ctrl Pts',(-29.4725749263794,-27.3548849305455,
1.47293214974064));
#31074=CARTESIAN_POINT('Ctrl Pts',(-29.4271284462447,-27.3705645465865,
1.01538106787477));
#31075=CARTESIAN_POINT('Ctrl Pts',(-29.3740093215551,-27.3820741720689,
0.528580803096812));
#31076=CARTESIAN_POINT('Ctrl Pts',(-29.2647682695533,-27.5098462703849,
-1.55402875459216));
#31077=CARTESIAN_POINT('Ctrl Pts',(-29.4149573143427,-27.8033726143276,
-3.101214321246));
#31078=CARTESIAN_POINT('Ctrl Pts',(-30.151613353974,-28.7756052303093,-5.98129145449804));
#31079=CARTESIAN_POINT('Ctrl Pts',(-30.7337162174556,-29.4435926415972,
-7.29389406578162));
#31080=CARTESIAN_POINT('Ctrl Pts',(-32.2310076487022,-31.0722410437307,
-9.49113593802495));
#31081=CARTESIAN_POINT('Ctrl Pts',(-33.1410090871408,-32.024354144657,-10.3708286016932));
#31082=CARTESIAN_POINT('Ctrl Pts',(-35.1535638963654,-34.102159417596,-11.5604045561488));
#31083=CARTESIAN_POINT('Ctrl Pts',(-36.2455537133794,-35.2124714378061,
-11.8694761542426));
#31084=CARTESIAN_POINT('Ctrl Pts',(-37.3337834058788,-36.3206928540898,
-11.8687142284811));
#31085=CARTESIAN_POINT('Ctrl Pts',(-27.9017241322579,-25.5825535213024,
1.59647090706389));
#31086=CARTESIAN_POINT('Ctrl Pts',(-27.8576356266559,-25.5977646187898,
1.15259179090242));
#31087=CARTESIAN_POINT('Ctrl Pts',(-27.8006101679571,-25.6076988465251,
0.635573104329223));
#31088=CARTESIAN_POINT('Ctrl Pts',(-27.6900511858225,-25.7366398496109,
-1.86858636179435));
#31089=CARTESIAN_POINT('Ctrl Pts',(-27.8867543207323,-26.0667980818921,
-3.71029995871567));
#31090=CARTESIAN_POINT('Ctrl Pts',(-28.8018888878676,-27.1980083507359,
-7.1693624749194));
#31091=CARTESIAN_POINT('Ctrl Pts',(-29.5148901762754,-27.9765753734451,
-8.73699595772763));
#31092=CARTESIAN_POINT('Ctrl Pts',(-31.3430252789425,-29.89317450793,-11.373025698192));
#31093=CARTESIAN_POINT('Ctrl Pts',(-32.4473861124854,-31.0108564714034,
-12.4235805192132));
#31094=CARTESIAN_POINT('Ctrl Pts',(-34.8951191227831,-33.4700709137458,
-13.852947082169));
#31095=CARTESIAN_POINT('Ctrl Pts',(-36.2126515924275,-34.7723177498594,
-14.2204718557404));
#31096=CARTESIAN_POINT('Ctrl Pts',(-37.5367254229125,-36.0864498658149,
-14.2198708430666));
#31097=CARTESIAN_POINT('Ctrl Pts',(-29.4615086055162,-23.7833669488545,
1.5967438644133));
#31098=CARTESIAN_POINT('Ctrl Pts',(-29.4174349631938,-23.7985729183137,
1.15301439043676));
#31099=CARTESIAN_POINT('Ctrl Pts',(-29.3602882272664,-23.8084199485298,
0.635579209506715));
#31100=CARTESIAN_POINT('Ctrl Pts',(-29.248392487277,-23.9362026442577,-1.86860431102996));
#31101=CARTESIAN_POINT('Ctrl Pts',(-29.4471451869125,-24.268136693283,-3.70979114471227));
#31102=CARTESIAN_POINT('Ctrl Pts',(-30.3599922882989,-25.3973651626949,
-7.17014261468329));
#31103=CARTESIAN_POINT('Ctrl Pts',(-31.0743967431037,-26.1771478462935,
-8.73670574474149));
#31104=CARTESIAN_POINT('Ctrl Pts',(-32.9020249033495,-28.0933077825863,
-11.3734544105236));
#31105=CARTESIAN_POINT('Ctrl Pts',(-34.0072159000762,-29.2117089638045,
-12.4221714958708));
#31106=CARTESIAN_POINT('Ctrl Pts',(-36.454022750563,-31.6701210582941,-13.854590909515));
#31107=CARTESIAN_POINT('Ctrl Pts',(-37.7721633453175,-32.9729180118855,
-14.2195188099009));
#31108=CARTESIAN_POINT('Ctrl Pts',(-39.096064193638,-34.2868769911001,-14.2201291128084));
#31109=CARTESIAN_POINT('Ctrl Pts',(-31.4387285991344,-25.0869579521469,
1.47327622041467));
#31110=CARTESIAN_POINT('Ctrl Pts',(-31.3933008545932,-25.1026311041689,
1.01591376687352));
#31111=CARTESIAN_POINT('Ctrl Pts',(-31.3400288564346,-25.1140308146317,
0.528588498850527));
#31112=CARTESIAN_POINT('Ctrl Pts',(-31.2291027822934,-25.2403428328586,
-1.55405138012545));
#31113=CARTESIAN_POINT('Ctrl Pts',(-31.3818753630052,-25.5361076454293,
-3.10057294640389));
#31114=CARTESIAN_POINT('Ctrl Pts',(-32.1156479855591,-26.5058421456065,
-5.98227484334892));
#31115=CARTESIAN_POINT('Ctrl Pts',(-32.6995195810811,-27.1753619327956,
-7.29352824387644));
#31116=CARTESIAN_POINT('Ctrl Pts',(-34.1961719966593,-28.8034567128286,
-9.49167634238131));
#31117=CARTESIAN_POINT('Ctrl Pts',(-35.1072198799242,-29.7564764086336,
-10.3690524868068));
#31118=CARTESIAN_POINT('Ctrl Pts',(-37.1186072377929,-31.8332702987844,
-11.5624766483077));
#31119=CARTESIAN_POINT('Ctrl Pts',(-38.2113611019678,-32.9442792642464,
-11.8682745704737));
#31120=CARTESIAN_POINT('Ctrl Pts',(-39.2993752576342,-34.0522789304537,
-11.8690397849988));
#31121=CARTESIAN_POINT('Ctrl Pts',(-33.632757135987,-25.9793365537799,1.35541241355846));
#31122=CARTESIAN_POINT('Ctrl Pts',(-33.5860390742569,-25.9954548817124,
0.885059162342653));
#31123=CARTESIAN_POINT('Ctrl Pts',(-33.5364438612593,-26.0083203842374,
0.426408625633996));
#31124=CARTESIAN_POINT('Ctrl Pts',(-33.4261818802089,-26.133000828325,-1.25364232215596));
#31125=CARTESIAN_POINT('Ctrl Pts',(-33.5354430048895,-26.3945703806125,
-2.51864171286469));
#31126=CARTESIAN_POINT('Ctrl Pts',(-34.0977429244459,-27.211592374279,-4.84795915808926));
#31127=CARTESIAN_POINT('Ctrl Pts',(-34.5572246086141,-27.7760442527838,
-5.91517020462051));
#31128=CARTESIAN_POINT('Ctrl Pts',(-35.7376805505111,-29.1289374295152,
-7.69457540344261));
#31129=CARTESIAN_POINT('Ctrl Pts',(-36.463475492835,-29.9241511239475,-8.40795287040691));
#31130=CARTESIAN_POINT('Ctrl Pts',(-38.0588356145443,-31.636324758031,-9.3737238373826));
#31131=CARTESIAN_POINT('Ctrl Pts',(-38.9364560608509,-32.5642699125021,
-9.62254085988727));
#31132=CARTESIAN_POINT('Ctrl Pts',(-39.7991514935067,-33.4755402303455,
-9.62369151535387));
#31133=CARTESIAN_POINT('Ctrl Pts',(-35.9592765491246,-26.4262081762393,
1.24768201173543));
#31134=CARTESIAN_POINT('Ctrl Pts',(-35.9113815427857,-26.4427325650909,
0.765479387902019));
#31135=CARTESIAN_POINT('Ctrl Pts',(-35.8651238615775,-26.4569206403349,
0.332966415955371));
#31136=CARTESIAN_POINT('Ctrl Pts',(-35.7551948794087,-26.5798713158822,
-0.978922014716766));
#31137=CARTESIAN_POINT('Ctrl Pts',(-35.8250853790451,-26.8105337258487,
-1.98636136649238));
#31138=CARTESIAN_POINT('Ctrl Pts',(-36.2301041572687,-27.4874934974146,
-3.81078790538449));
#31139=CARTESIAN_POINT('Ctrl Pts',(-36.5761192475516,-27.9561102697828,
-4.65460264906168));
#31140=CARTESIAN_POINT('Ctrl Pts',(-37.4673095829948,-29.0572415380562,
-6.05121512497099));
#31141=CARTESIAN_POINT('Ctrl Pts',(-38.0238611245252,-29.7082892825274,
-6.61423873306931));
#31142=CARTESIAN_POINT('Ctrl Pts',(-39.2385744113842,-31.08685315642,-7.37244739479499));
#31143=CARTESIAN_POINT('Ctrl Pts',(-39.9195822825557,-31.8474936465318,
-7.56862230155737));
#31144=CARTESIAN_POINT('Ctrl Pts',(-40.5761862384897,-32.5788252613915,
-7.57037421506009));
#31145=CARTESIAN_POINT('Ctrl Pts',(-31.2585017743464,-21.3513306581893,
1.5964708619975));
#31146=CARTESIAN_POINT('Ctrl Pts',(-31.2170267923822,-21.3726613764954,
1.15259176010419));
#31147=CARTESIAN_POINT('Ctrl Pts',(-31.1619955607693,-21.3906100567219,
0.635573083876073));
#31148=CARTESIAN_POINT('Ctrl Pts',(-31.0709121283971,-21.5339728088745,
-1.86858636179032));
#31149=CARTESIAN_POINT('Ctrl Pts',(-31.3125995244277,-21.8327767315655,
-3.71029995869747));
#31150=CARTESIAN_POINT('Ctrl Pts',(-32.3794073476997,-22.8222356829231,
-7.16936247493759));
#31151=CARTESIAN_POINT('Ctrl Pts',(-33.1959529508923,-23.4914073530275,
-8.73699595768452));
#31152=CARTESIAN_POINT('Ctrl Pts',(-35.2782407701427,-25.1283275201853,
-11.3730256982351));
#31153=CARTESIAN_POINT('Ctrl Pts',(-36.5304235306209,-26.0774661593507,
-12.4235805192512));
#31154=CARTESIAN_POINT('Ctrl Pts',(-39.3032248537559,-28.1633006173621,
-13.852947082131));
#31155=CARTESIAN_POINT('Ctrl Pts',(-40.7926757902182,-29.2647880382123,
-14.220471855574));
#31156=CARTESIAN_POINT('Ctrl Pts',(-42.2902929581064,-30.3771088306743,
-14.2198708430667));
#31157=CARTESIAN_POINT('Ctrl Pts',(-31.1156831315056,-20.4102131175329,
1.62964630360509));
#31158=CARTESIAN_POINT('Ctrl Pts',(-31.0745541646235,-20.4313658791528,
1.18947037065693));
#31159=CARTESIAN_POINT('Ctrl Pts',(-31.0183916684119,-20.4490273774703,
0.664244043755391));
#31160=CARTESIAN_POINT('Ctrl Pts',(-30.9266087973868,-20.5924969121563,
-1.95287905128436));
#31161=CARTESIAN_POINT('Ctrl Pts',(-31.1826348335827,-20.8996315610389,
-3.8733738707857));
#31162=CARTESIAN_POINT('Ctrl Pts',(-32.3021679589144,-21.9240162327835,
-7.48792130213993));
#31163=CARTESIAN_POINT('Ctrl Pts',(-33.1580626257291,-22.6177912263194,
-9.12360836230261));
#31164=CARTESIAN_POINT('Ctrl Pts',(-35.3389311938565,-24.3183718641586,
-11.8774049927285));
#31165=CARTESIAN_POINT('Ctrl Pts',(-36.649222639852,-25.3041699213976,-12.9732563608962));
#31166=CARTESIAN_POINT('Ctrl Pts',(-39.5517175889612,-27.4743946039037,
-14.4676858045385));
#31167=CARTESIAN_POINT('Ctrl Pts',(-41.1084892565552,-28.618307904635,-14.8501851004628));
#31168=CARTESIAN_POINT('Ctrl Pts',(-42.6764590955598,-29.776211096424,-14.8499483202528));
#31169=CARTESIAN_POINT('Ctrl Pts',(-31.6308259996107,-19.6090715485704,
1.62975548654487));
#31170=CARTESIAN_POINT('Ctrl Pts',(-31.5897026256008,-19.6302214337556,
1.18963941046845));
#31171=CARTESIAN_POINT('Ctrl Pts',(-31.5334871484746,-19.6478553118982,
0.664246485824284));
#31172=CARTESIAN_POINT('Ctrl Pts',(-31.4411090790738,-19.7909423357851,
-1.95288623097265));
#31173=CARTESIAN_POINT('Ctrl Pts',(-31.6980476865419,-20.0986634078754,
-3.87317034519465));
#31174=CARTESIAN_POINT('Ctrl Pts',(-32.8165623230563,-21.1223936447321,
-7.48823335803519));
#31175=CARTESIAN_POINT('Ctrl Pts',(-33.6730817461571,-21.8165700765847,
-9.12349227712632));
#31176=CARTESIAN_POINT('Ctrl Pts',(-35.8537245995411,-23.5170056814859,
-11.8775764776429));
#31177=CARTESIAN_POINT('Ctrl Pts',(-37.1643856730156,-24.5030412397768,
-12.9726927515238));
#31178=CARTESIAN_POINT('Ctrl Pts',(-40.0664682545546,-26.6730009723283,
-14.4683433355124));
#31179=CARTESIAN_POINT('Ctrl Pts',(-41.6235121428231,-27.8170972008458,
-14.8498038985385));
#31180=CARTESIAN_POINT('Ctrl Pts',(-43.1914035066775,-28.9749419513884,
-14.8500516281495));
#31181=CARTESIAN_POINT('Ctrl Pts',(-32.546358944609,-19.3484767357832,1.59674381934694));
#31182=CARTESIAN_POINT('Ctrl Pts',(-32.5048979448244,-19.3698002629962,
1.15301435963279));
#31183=CARTESIAN_POINT('Ctrl Pts',(-32.4497342609268,-19.3876798927917,
0.635579189048305));
#31184=CARTESIAN_POINT('Ctrl Pts',(-32.3571628326124,-19.5300863679464,
-1.86860431101105));
#31185=CARTESIAN_POINT('Ctrl Pts',(-32.6011316568376,-19.8303563486603,
-3.70979114471446));
#31186=CARTESIAN_POINT('Ctrl Pts',(-33.6653932580424,-20.818179212791,-7.17014261468111));
#31187=CARTESIAN_POINT('Ctrl Pts',(-34.4835007519621,-21.4883544786787,
-8.73670574475098));
#31188=CARTESIAN_POINT('Ctrl Pts',(-36.5652242843543,-23.1249120635156,
-11.373454410514));
#31189=CARTESIAN_POINT('Ctrl Pts',(-37.8183311135274,-24.0746444552904,
-12.4221714958225));
#31190=CARTESIAN_POINT('Ctrl Pts',(-40.5901015177415,-26.1598165384319,
-13.8545909095632));
#31191=CARTESIAN_POINT('Ctrl Pts',(-42.0802326794301,-27.2617619321623,
-14.219518810015));
#31192=CARTESIAN_POINT('Ctrl Pts',(-43.5776539859008,-28.3739359680852,
-14.2201291128084));
#31193=CARTESIAN_POINT('Ctrl Pts',(-31.1388779521429,-21.4269965203141,
0.));
#31194=CARTESIAN_POINT('Ctrl Pts',(-31.0709121283971,-21.5339728088745,
-1.86858636179032));
#31195=CARTESIAN_POINT('Ctrl Pts',(-31.3125995244325,-21.8327767315655,
-3.71029995869628));
#31196=CARTESIAN_POINT('Ctrl Pts',(-32.3794073476949,-22.8222356829231,
-7.1693624749388));
#31197=CARTESIAN_POINT('Ctrl Pts',(-33.1959529508875,-23.4914073530251,
-8.73699595768692));
#31198=CARTESIAN_POINT('Ctrl Pts',(-34.3430070554517,-24.3931251555404,
-10.1890856763507));
#31199=CARTESIAN_POINT('Ctrl Pts',(-34.4511010682896,-24.4777351286599,
-10.3203928635182));
#31200=CARTESIAN_POINT('Ctrl Pts',(-34.561298034014,-24.5636585134826,-10.4488603766016));
#31201=CARTESIAN_POINT('Ctrl Pts',(-32.4262389885813,-19.4238236466308,
5.55111512312578E-17));
#31202=CARTESIAN_POINT('Ctrl Pts',(-32.3571628326124,-19.5300863679464,
-1.86860431101105));
#31203=CARTESIAN_POINT('Ctrl Pts',(-32.6011316568376,-19.8303563486603,
-3.70979114471446));
#31204=CARTESIAN_POINT('Ctrl Pts',(-33.6653932580424,-20.818179212791,-7.17014261468111));
#31205=CARTESIAN_POINT('Ctrl Pts',(-34.4835007519621,-21.4883544786787,
-8.73670574475098));
#31206=CARTESIAN_POINT('Ctrl Pts',(-35.6360972865638,-22.3944741298273,
-10.1966053555709));
#31207=CARTESIAN_POINT('Ctrl Pts',(-35.7502778955778,-22.4838298155547,
-10.3350231942257));
#31208=CARTESIAN_POINT('Ctrl Pts',(-35.8668060412531,-22.5746525783681,
-10.4702558450969));
#31209=CARTESIAN_POINT('Ctrl Pts',(-35.622245200284,-26.8434139987114,1.24689101061694));
#31210=CARTESIAN_POINT('Ctrl Pts',(-35.5771488466483,-26.8666072002778,
0.76425478004101));
#31211=CARTESIAN_POINT('Ctrl Pts',(-35.5337649882637,-26.8874341048637,
0.332948714107228));
#31212=CARTESIAN_POINT('Ctrl Pts',(-35.4467644378207,-27.0275488741708,
-0.978870002741806));
#31213=CARTESIAN_POINT('Ctrl Pts',(-35.5421592790146,-27.2416687814337,
-1.98783577087493));
#31214=CARTESIAN_POINT('Ctrl Pts',(-36.0467752285009,-27.8588388319703,
-3.80852727285));
#31215=CARTESIAN_POINT('Ctrl Pts',(-36.4514335703522,-28.2705345323084,
-4.65544360719879));
#31216=CARTESIAN_POINT('Ctrl Pts',(-37.4918953411247,-29.2346789284782,
-6.04997283345455));
#31217=CARTESIAN_POINT('Ctrl Pts',(-38.1327580455326,-29.7981738697285,
-6.61832169905812));
#31218=CARTESIAN_POINT('Ctrl Pts',(-39.5342847196047,-30.9917536078482,
-7.36768403075847));
#31219=CARTESIAN_POINT('Ctrl Pts',(-40.3146623987948,-31.6463688825735,
-7.57138648661831));
#31220=CARTESIAN_POINT('Ctrl Pts',(-41.069207801424,-32.2772757571273,-7.56962581969434));
#31221=CARTESIAN_POINT('Ctrl Pts',(-34.5390490058877,-24.7365171914566,
1.35489339099692));
#31222=CARTESIAN_POINT('Ctrl Pts',(-34.495073760779,-24.7591338032465,0.884255638227479));
#31223=CARTESIAN_POINT('Ctrl Pts',(-34.4480661428486,-24.7790577744534,
0.426397004060221));
#31224=CARTESIAN_POINT('Ctrl Pts',(-34.3594994945276,-24.9199792485703,
-1.25360819504204));
#31225=CARTESIAN_POINT('Ctrl Pts',(-34.5005360167971,-25.1605494847803,
-2.51960912779196));
#31226=CARTESIAN_POINT('Ctrl Pts',(-35.1782280532587,-25.8923424652779,
-4.8464758678288));
#31227=CARTESIAN_POINT('Ctrl Pts',(-35.7103931102495,-26.383749825687,-5.91572199044976));
#31228=CARTESIAN_POINT('Ctrl Pts',(-37.0724433726275,-27.5555654868557,
-7.6937602869373));
#31229=CARTESIAN_POINT('Ctrl Pts',(-37.9022645329764,-28.2382647528049,
-8.41063186559025));
#31230=CARTESIAN_POINT('Ctrl Pts',(-39.7270140028392,-29.7072268925306,
-9.37059840617594));
#31231=CARTESIAN_POINT('Ctrl Pts',(-40.726476090564,-30.4999439048389,-9.62435378608523));
#31232=CARTESIAN_POINT('Ctrl Pts',(-41.7104427005355,-31.2794573106203,
-9.62320046360545));
#31233=CARTESIAN_POINT('Ctrl Pts',(-33.0655926302367,-22.8820669124603,
1.4729321046743));
#31234=CARTESIAN_POINT('Ctrl Pts',(-33.0228401731413,-22.9040546403855,
1.01538103752956));
#31235=CARTESIAN_POINT('Ctrl Pts',(-32.97189971713,-22.9230067538041,0.528580786088482));
#31236=CARTESIAN_POINT('Ctrl Pts',(-32.8819544477915,-23.0650249379137,
-1.55402875459391));
#31237=CARTESIAN_POINT('Ctrl Pts',(-33.0723879388088,-23.3341894772883,
-3.10121432123244));
#31238=CARTESIAN_POINT('Ctrl Pts',(-33.9399090096342,-24.1916890818838,
-5.98129145451161));
#31239=CARTESIAN_POINT('Ctrl Pts',(-34.6111514256777,-24.770035469683,-7.29389406574571));
#31240=CARTESIAN_POINT('Ctrl Pts',(-36.3249834230578,-26.1690197914205,
-9.49113593806087));
#31241=CARTESIAN_POINT('Ctrl Pts',(-37.3612221809205,-26.98193504625,-10.370828601741));
#31242=CARTESIAN_POINT('Ctrl Pts',(-39.6489946054446,-28.7521748454075,
-11.5604045561011));
#31243=CARTESIAN_POINT('Ctrl Pts',(-40.8878834161069,-29.6957791360099,
-11.8694761540333));
#31244=CARTESIAN_POINT('Ctrl Pts',(-42.1227528511809,-30.6378492234121,
-11.8687142284812));
#31245=CARTESIAN_POINT('Ctrl Pts',(-31.2585017743464,-21.3513306581893,
1.5964708619975));
#31246=CARTESIAN_POINT('Ctrl Pts',(-31.2170267923791,-21.3726613764954,
1.15259176010449));
#31247=CARTESIAN_POINT('Ctrl Pts',(-31.1619955607693,-21.3906100567219,
0.635573083876073));
#31248=CARTESIAN_POINT('Ctrl Pts',(-31.0709121283971,-21.5339728088745,
-1.86858636179032));
#31249=CARTESIAN_POINT('Ctrl Pts',(-31.3125995244325,-21.8327767315655,
-3.71029995869628));
#31250=CARTESIAN_POINT('Ctrl Pts',(-32.3794073476949,-22.8222356829231,
-7.1693624749388));
#31251=CARTESIAN_POINT('Ctrl Pts',(-33.1959529508875,-23.4914073530251,
-8.73699595768692));
#31252=CARTESIAN_POINT('Ctrl Pts',(-35.2782407701475,-25.1283275201876,
-11.3730256982327));
#31253=CARTESIAN_POINT('Ctrl Pts',(-36.5304235306209,-26.0774661593532,
-12.4235805192512));
#31254=CARTESIAN_POINT('Ctrl Pts',(-39.3032248537558,-28.1633006173597,
-13.852947082131));
#31255=CARTESIAN_POINT('Ctrl Pts',(-40.792675790223,-29.2647880382077,-14.220471855574));
#31256=CARTESIAN_POINT('Ctrl Pts',(-42.2902929581064,-30.3771088306743,
-14.2198708430667));
#31257=CARTESIAN_POINT('Ctrl Pts',(-32.546358944609,-19.3484767357832,1.59674381934694));
#31258=CARTESIAN_POINT('Ctrl Pts',(-32.5048979448244,-19.3698002629962,
1.15301435963279));
#31259=CARTESIAN_POINT('Ctrl Pts',(-32.4497342609268,-19.3876798927917,
0.635579189048305));
#31260=CARTESIAN_POINT('Ctrl Pts',(-32.3571628326124,-19.5300863679464,
-1.86860431101105));
#31261=CARTESIAN_POINT('Ctrl Pts',(-32.6011316568376,-19.8303563486603,
-3.70979114471446));
#31262=CARTESIAN_POINT('Ctrl Pts',(-33.6653932580424,-20.818179212791,-7.17014261468111));
#31263=CARTESIAN_POINT('Ctrl Pts',(-34.4835007519573,-21.4883544786811,
-8.73670574474859));
#31264=CARTESIAN_POINT('Ctrl Pts',(-36.5652242843591,-23.1249120635132,
-11.3734544105164));
#31265=CARTESIAN_POINT('Ctrl Pts',(-37.8183311135274,-24.0746444552904,
-12.4221714958225));
#31266=CARTESIAN_POINT('Ctrl Pts',(-40.5901015177415,-26.1598165384319,
-13.8545909095632));
#31267=CARTESIAN_POINT('Ctrl Pts',(-42.0802326794284,-27.2617619321646,
-14.219518810015));
#31268=CARTESIAN_POINT('Ctrl Pts',(-43.5776539859008,-28.3739359680852,
-14.2201291128084));
#31269=CARTESIAN_POINT('Ctrl Pts',(-34.688974032416,-20.3574113186625,1.47327617534836));
#31270=CARTESIAN_POINT('Ctrl Pts',(-34.6462392002796,-20.3793899820083,
1.01591373651933));
#31271=CARTESIAN_POINT('Ctrl Pts',(-34.5951317842973,-20.3982550553481,
0.528588481835565));
#31272=CARTESIAN_POINT('Ctrl Pts',(-34.5033108528189,-20.5390678245049,
-1.55405138010844));
#31273=CARTESIAN_POINT('Ctrl Pts',(-34.6966201503934,-20.8100803726322,
-3.1005729464179));
#31274=CARTESIAN_POINT('Ctrl Pts',(-35.5609316342885,-21.6655176417209,
-5.98227484333492));
#31275=CARTESIAN_POINT('Ctrl Pts',(-36.2341428589936,-22.2451290911801,
-7.29352824390031));
#31276=CARTESIAN_POINT('Ctrl Pts',(-37.9472635563893,-23.6436563673571,
-9.4916763423574));
#31277=CARTESIAN_POINT('Ctrl Pts',(-38.9846671297029,-24.4573200646131,
-10.3690524867489));
#31278=CARTESIAN_POINT('Ctrl Pts',(-41.2711400509577,-26.2267249209926,
-11.5624766483654));
#31279=CARTESIAN_POINT('Ctrl Pts',(-42.5108843176328,-27.1709103277457,
-11.8682745706116));
#31280=CARTESIAN_POINT('Ctrl Pts',(-43.7455088513557,-28.112791596242,-11.8690397849987));
#31281=CARTESIAN_POINT('Ctrl Pts',(-36.9876692386613,-20.9284639764453,
1.35541236849222));
#31282=CARTESIAN_POINT('Ctrl Pts',(-36.9437205780641,-20.9510669157128,
0.885059132418801));
#31283=CARTESIAN_POINT('Ctrl Pts',(-36.8964611268098,-20.9708596004016,
0.42640861190665));
#31284=CARTESIAN_POINT('Ctrl Pts',(-36.8050653317125,-21.1099628921499,
-1.25364232213785));
#31285=CARTESIAN_POINT('Ctrl Pts',(-36.9504395642135,-21.3533205642746,
-2.51864171289894));
#31286=CARTESIAN_POINT('Ctrl Pts',(-37.6232904342764,-22.0820028300357,
-4.84795915805504));
#31287=CARTESIAN_POINT('Ctrl Pts',(-38.1584251351866,-22.5753183406665,
-5.91517020467311));
#31288=CARTESIAN_POINT('Ctrl Pts',(-39.5194025113629,-23.746444619158,-7.69457540339));
#31289=CARTESIAN_POINT('Ctrl Pts',(-40.3509806159836,-24.4302727949682,
-8.40795287031555));
#31290=CARTESIAN_POINT('Ctrl Pts',(-42.1737699857923,-25.89797555241,-9.37372383747387));
#31291=CARTESIAN_POINT('Ctrl Pts',(-43.1745178860502,-26.6915771512951,
-9.62254086014419));
#31292=CARTESIAN_POINT('Ctrl Pts',(-44.158119610933,-27.4707976903314,-9.6236915153538));
#31293=CARTESIAN_POINT('Ctrl Pts',(-39.3541045014164,-21.0396888561034,
1.24768196666925));
#31294=CARTESIAN_POINT('Ctrl Pts',(-39.3090486643439,-21.062861219838,0.765479358368067));
#31295=CARTESIAN_POINT('Ctrl Pts',(-39.2652809953009,-21.0834880350827,
0.332966405233472));
#31296=CARTESIAN_POINT('Ctrl Pts',(-39.1739686379048,-21.2208317741238,
-0.978922014694586));
#31297=CARTESIAN_POINT('Ctrl Pts',(-39.2759744366033,-21.4391999182154,
-1.98636136654806));
#31298=CARTESIAN_POINT('Ctrl Pts',(-39.7732121280719,-22.0516290335938,
-3.81078790532884));
#31299=CARTESIAN_POINT('Ctrl Pts',(-40.1823964038188,-22.4662328811704,
-4.65460264915733));
#31300=CARTESIAN_POINT('Ctrl Pts',(-41.2212230249915,-23.4293266125112,
-6.05121512487531));
#31301=CARTESIAN_POINT('Ctrl Pts',(-41.8647634287622,-23.9945420871117,
-6.6142387329492));
#31302=CARTESIAN_POINT('Ctrl Pts',(-43.2633027806245,-25.1862024432709,
-7.37244739491497));
#31303=CARTESIAN_POINT('Ctrl Pts',(-44.0456294021901,-25.8421831847813,
-7.56862230193347));
#31304=CARTESIAN_POINT('Ctrl Pts',(-44.7996294168197,-26.4726264127402,
-7.57037421505999));
#31305=CARTESIAN_POINT('Ctrl Pts',(-33.9789464595043,-16.6854562787124,
1.5964707761032));
#31306=CARTESIAN_POINT('Ctrl Pts',(-33.9409293131115,-16.712472384756,1.15259170140102));
#31307=CARTESIAN_POINT('Ctrl Pts',(-33.8890125875502,-16.7380701329957,
0.635573044902023));
#31308=CARTESIAN_POINT('Ctrl Pts',(-33.8192589011655,-16.8929361804564,
-1.86858636180863));
#31309=CARTESIAN_POINT('Ctrl Pts',(-34.1010104999369,-17.1543030074678,
-3.71029995871351));
#31310=CARTESIAN_POINT('Ctrl Pts',(-35.2977744483822,-17.9818681105444,
-7.16936247492166));
#31311=CARTESIAN_POINT('Ctrl Pts',(-36.2012418527657,-18.52802202229,-8.73699595772984));
#31312=CARTESIAN_POINT('Ctrl Pts',(-38.4952930131949,-19.8519402484793,
-11.3730256981899));
#31313=CARTESIAN_POINT('Ctrl Pts',(-39.8698068706361,-20.6132138376926,
-12.4235805192373));
#31314=CARTESIAN_POINT('Ctrl Pts',(-42.9112302679262,-22.2832067364649,
-13.852947082145));
#31315=CARTESIAN_POINT('Ctrl Pts',(-44.542278745562,-23.1615116346327,-14.220471855593));
#31316=CARTESIAN_POINT('Ctrl Pts',(-46.1829520838074,-24.0493774600892,
-14.2198708430667));
#31317=CARTESIAN_POINT('Ctrl Pts',(-33.7036465139254,-15.7742431696986,
1.62964621771081));
#31318=CARTESIAN_POINT('Ctrl Pts',(-33.6659465347885,-15.8010338873349,
1.18947031171706));
#31319=CARTESIAN_POINT('Ctrl Pts',(-33.6128691890195,-15.8265083724895,
0.664244003023023));
#31320=CARTESIAN_POINT('Ctrl Pts',(-33.5424383800422,-15.9815796560817,
-1.95287905130295));
#31321=CARTESIAN_POINT('Ctrl Pts',(-33.8395682582167,-16.2491518132483,
-3.8733738708029));
#31322=CARTESIAN_POINT('Ctrl Pts',(-35.0934912894295,-17.1037835504083,
-7.48792130212284));
#31323=CARTESIAN_POINT('Ctrl Pts',(-36.039408658731,-17.6686904035875,-9.12360836232398));
#31324=CARTESIAN_POINT('Ctrl Pts',(-38.4400969876706,-19.0415916253474,
-11.8774049927072));
#31325=CARTESIAN_POINT('Ctrl Pts',(-39.8773452471794,-19.8308817644304,
-12.9732563608919));
#31326=CARTESIAN_POINT('Ctrl Pts',(-43.0591521575018,-21.5659485894734,
-14.4676858045429));
#31327=CARTESIAN_POINT('Ctrl Pts',(-44.7628739705109,-22.4766667942929,
-14.8501851005009));
#31328=CARTESIAN_POINT('Ctrl Pts',(-46.4796709429185,-23.3996388269523,
-14.8499483202528));
#31329=CARTESIAN_POINT('Ctrl Pts',(-34.0995316375869,-14.9079435927954,
1.62975540065056));
#31330=CARTESIAN_POINT('Ctrl Pts',(-34.0618367850434,-14.9347306673279,
1.18963935152099));
#31331=CARTESIAN_POINT('Ctrl Pts',(-34.0087030668448,-14.9601853534011,
0.664246445090203));
#31332=CARTESIAN_POINT('Ctrl Pts',(-33.9376286808235,-15.1149627251836,
-1.95288623098664));
#31333=CARTESIAN_POINT('Ctrl Pts',(-34.2357452983146,-15.3829854641729,
-3.87317034520824));
#31334=CARTESIAN_POINT('Ctrl Pts',(-35.4885670716678,-16.237114373715,-7.48823335802167));
#31335=CARTESIAN_POINT('Ctrl Pts',(-36.4351599687878,-16.8023296670664,
-9.12349227711899));
#31336=CARTESIAN_POINT('Ctrl Pts',(-38.8356042400472,-18.1751194546594,
-11.8775764776503));
#31337=CARTESIAN_POINT('Ctrl Pts',(-40.273252164705,-18.9645920738991,-12.9726927515338));
#31338=CARTESIAN_POINT('Ctrl Pts',(-43.4546131984608,-20.6994553318364,
-14.4683433355024));
#31339=CARTESIAN_POINT('Ctrl Pts',(-45.1586304946511,-21.610315861468,-14.8498038985814));
#31340=CARTESIAN_POINT('Ctrl Pts',(-46.8753414736305,-22.5332412158905,
-14.8500516281495));
#31341=CARTESIAN_POINT('Ctrl Pts',(-34.9686592686579,-14.5197073364544,
1.59674373345257));
#31342=CARTESIAN_POINT('Ctrl Pts',(-34.9306549387506,-14.5467143347365,
1.15301430091077));
#31343=CARTESIAN_POINT('Ctrl Pts',(-34.8785972821108,-14.5722625852753,
0.635579150069985));
#31344=CARTESIAN_POINT('Ctrl Pts',(-34.8072346531258,-14.7263938532101,
-1.86860431101787));
#31345=CARTESIAN_POINT('Ctrl Pts',(-35.0914531001935,-14.9888871347756,
-3.70979114472567));
#31346=CARTESIAN_POINT('Ctrl Pts',(-36.2854639039658,-15.8151951688146,
-7.17014261466994));
#31347=CARTESIAN_POINT('Ctrl Pts',(-37.1906201279053,-16.3621201809922,
-8.73670574471494));
#31348=CARTESIAN_POINT('Ctrl Pts',(-39.4840611441388,-17.6857598217545,
-11.3734544105501));
#31349=CARTESIAN_POINT('Ctrl Pts',(-40.8595741644358,-18.4474896113692,
-12.4221714958517));
#31350=CARTESIAN_POINT('Ctrl Pts',(-43.899882870338,-20.1169735923676,-13.854590909534));
#31351=CARTESIAN_POINT('Ctrl Pts',(-45.5316698257921,-20.9956349957552,
-14.2195188101196));
#31352=CARTESIAN_POINT('Ctrl Pts',(-47.1721284105873,-21.8833834324347,
-14.2201291128084));
#31353=CARTESIAN_POINT('Ctrl Pts',(-33.8713086176152,-16.7773762111442,
0.));
#31354=CARTESIAN_POINT('Ctrl Pts',(-33.8192589011655,-16.8929361804564,
-1.86858636180863));
#31355=CARTESIAN_POINT('Ctrl Pts',(-34.1010104999369,-17.1543030074678,
-3.71029995871351));
#31356=CARTESIAN_POINT('Ctrl Pts',(-35.2977744483822,-17.9818681105444,
-7.16936247492166));
#31357=CARTESIAN_POINT('Ctrl Pts',(-36.2012418527657,-18.5280220222852,
-8.73699595772984));
#31358=CARTESIAN_POINT('Ctrl Pts',(-37.4649484236404,-19.2573188185412,
-10.1890856763468));
#31359=CARTESIAN_POINT('Ctrl Pts',(-37.5839834499235,-19.3256842021906,
-10.320392863511));
#31360=CARTESIAN_POINT('Ctrl Pts',(-37.7052869420397,-19.3950503475036,
-10.4488603765919));
#31361=CARTESIAN_POINT('Ctrl Pts',(-34.8604849513723,-14.6113821712782,
6.38378239159465E-15));
#31362=CARTESIAN_POINT('Ctrl Pts',(-34.8072346531258,-14.7263938532101,
-1.86860431101787));
#31363=CARTESIAN_POINT('Ctrl Pts',(-35.0914531001935,-14.9888871347756,
-3.70979114472567));
#31364=CARTESIAN_POINT('Ctrl Pts',(-36.2854639039658,-15.8151951688146,
-7.17014261466994));
#31365=CARTESIAN_POINT('Ctrl Pts',(-37.1906201279053,-16.3621201809922,
-8.73670574471494));
#31366=CARTESIAN_POINT('Ctrl Pts',(-38.4604391631867,-17.0949852513367,
-10.1966053555752));
#31367=CARTESIAN_POINT('Ctrl Pts',(-38.5861742181901,-17.1671818301296,
-10.3350231942337));
#31368=CARTESIAN_POINT('Ctrl Pts',(-38.7144417021566,-17.2404964639767,
-10.4702558451082));
#31369=CARTESIAN_POINT('Ctrl Pts',(-39.0798782217544,-21.5006126898293,
1.24689092472233));
#31370=CARTESIAN_POINT('Ctrl Pts',(-39.0385416232223,-21.5299876965017,
0.764254723795939));
#31371=CARTESIAN_POINT('Ctrl Pts',(-38.9985633313699,-21.5567767789462,
0.332948693683721));
#31372=CARTESIAN_POINT('Ctrl Pts',(-38.9323887326868,-21.7078468489021,
-0.978870002731641));
#31373=CARTESIAN_POINT('Ctrl Pts',(-39.0572850320307,-21.9062112228121,
-1.98783577086975));
#31374=CARTESIAN_POINT('Ctrl Pts',(-39.6445971746952,-22.4452850348649,
-3.80852727285524));
#31375=CARTESIAN_POINT('Ctrl Pts',(-40.1037270849374,-22.7952013801937,
-4.65544360729441));
#31376=CARTESIAN_POINT('Ctrl Pts',(-41.2708105092392,-23.6014590278078,
-6.04997283335897));
#31377=CARTESIAN_POINT('Ctrl Pts',(-41.9853438466739,-24.0680141309499,
-6.61832169900558));
#31378=CARTESIAN_POINT('Ctrl Pts',(-43.5424691073585,-25.0499869064575,
-7.36768403081101));
#31379=CARTESIAN_POINT('Ctrl Pts',(-44.4080651340567,-25.5868798182086,
-7.5713864865375));
#31380=CARTESIAN_POINT('Ctrl Pts',(-45.2447177621909,-26.1039819636367,
-7.56962581969439));
#31381=CARTESIAN_POINT('Ctrl Pts',(-37.707864724394,-19.569315945402,1.35489330510239));
#31382=CARTESIAN_POINT('Ctrl Pts',(-37.6675557657917,-19.5979606808283,
0.884255581219552));
#31383=CARTESIAN_POINT('Ctrl Pts',(-37.6238620982313,-19.6243717351791,
0.426396977907638));
#31384=CARTESIAN_POINT('Ctrl Pts',(-37.5562521484444,-19.7764631777536,
-1.25360819503831));
#31385=CARTESIAN_POINT('Ctrl Pts',(-37.7300898366018,-19.9945131659726,
-2.51960912778906));
#31386=CARTESIAN_POINT('Ctrl Pts',(-38.5050289449581,-20.6224119165131,
-4.84647586783176));
#31387=CARTESIAN_POINT('Ctrl Pts',(-39.1017118879154,-21.0330824745317,
-5.91572199051186));
#31388=CARTESIAN_POINT('Ctrl Pts',(-40.6166651990263,-21.9991307790679,
-7.69376028687524));
#31389=CARTESIAN_POINT('Ctrl Pts',(-41.5351982120125,-22.5567852866265,
-8.41063186556173));
#31390=CARTESIAN_POINT('Ctrl Pts',(-43.550429472657,-23.7511065841626,-9.37059840620446));
#31391=CARTESIAN_POINT('Ctrl Pts',(-44.6525338708919,-24.3935165948524,
-9.62435378606624));
#31392=CARTESIAN_POINT('Ctrl Pts',(-45.7374214437731,-25.0250626292175,
-9.62320046360548));
#31393=CARTESIAN_POINT('Ctrl Pts',(-35.9854902185572,-17.9434360021529,
1.47293201877987));
#31394=CARTESIAN_POINT('Ctrl Pts',(-35.9463021021891,-17.9712842340159,
1.01538097969052));
#31395=CARTESIAN_POINT('Ctrl Pts',(-35.8985773174064,-17.997293023891,0.52858075367214));
#31396=CARTESIAN_POINT('Ctrl Pts',(-35.8297588571567,-18.1506662116799,
-1.55402875459979));
#31397=CARTESIAN_POINT('Ctrl Pts',(-36.0565601177375,-18.3899895327109,
-3.1012143212414));
#31398=CARTESIAN_POINT('Ctrl Pts',(-37.0372859924679,-19.1152999068477,
-5.98129145450272));
#31399=CARTESIAN_POINT('Ctrl Pts',(-37.7840034012004,-19.592231806371,-7.29389406578866));
#31400=CARTESIAN_POINT('Ctrl Pts',(-39.6794872875132,-20.7330727614972,
-9.49113593801798));
#31401=CARTESIAN_POINT('Ctrl Pts',(-40.8208685319662,-21.3902415598682,
-10.3708286017221));
#31402=CARTESIAN_POINT('Ctrl Pts',(-43.3372861226137,-22.8168789077003,
-11.56040455612));
#31403=CARTESIAN_POINT('Ctrl Pts',(-44.6978537235209,-23.5745664065252,
-11.8694761540143));
#31404=CARTESIAN_POINT('Ctrl Pts',(-46.0542245204212,-24.331307334807,-11.8687142284812));
#31405=CARTESIAN_POINT('Ctrl Pts',(-33.9789464595043,-16.6854562787123,
1.5964707761032));
#31406=CARTESIAN_POINT('Ctrl Pts',(-33.9409293131115,-16.712472384756,1.15259170140102));
#31407=CARTESIAN_POINT('Ctrl Pts',(-33.8890125875502,-16.7380701329957,
0.635573044902023));
#31408=CARTESIAN_POINT('Ctrl Pts',(-33.8192589011655,-16.8929361804564,
-1.86858636180863));
#31409=CARTESIAN_POINT('Ctrl Pts',(-34.1010104999369,-17.1543030074678,
-3.71029995871351));
#31410=CARTESIAN_POINT('Ctrl Pts',(-35.2977744483822,-17.9818681105444,
-7.16936247492166));
#31411=CARTESIAN_POINT('Ctrl Pts',(-36.2012418527657,-18.5280220222852,
-8.73699595772984));
#31412=CARTESIAN_POINT('Ctrl Pts',(-38.4952930131949,-19.8519402484841,
-11.3730256981899));
#31413=CARTESIAN_POINT('Ctrl Pts',(-39.8698068706361,-20.6132138376926,
-12.4235805192373));
#31414=CARTESIAN_POINT('Ctrl Pts',(-42.9112302679262,-22.2832067364649,
-13.852947082145));
#31415=CARTESIAN_POINT('Ctrl Pts',(-44.542278745567,-23.1615116346235,-14.2204718555787));
#31416=CARTESIAN_POINT('Ctrl Pts',(-46.1829520838074,-24.0493774600892,
-14.2198708430667));
#31417=CARTESIAN_POINT('Ctrl Pts',(-34.9686592686579,-14.5197073364544,
1.59674373345257));
#31418=CARTESIAN_POINT('Ctrl Pts',(-34.9306549387506,-14.5467143347365,
1.15301430091077));
#31419=CARTESIAN_POINT('Ctrl Pts',(-34.8785972821108,-14.5722625852752,
0.635579150069985));
#31420=CARTESIAN_POINT('Ctrl Pts',(-34.8072346531258,-14.7263938532101,
-1.86860431101787));
#31421=CARTESIAN_POINT('Ctrl Pts',(-35.0914531001935,-14.9888871347744,
-3.70979114472567));
#31422=CARTESIAN_POINT('Ctrl Pts',(-36.2854639039658,-15.8151951688158,
-7.17014261466994));
#31423=CARTESIAN_POINT('Ctrl Pts',(-37.1906201279053,-16.3621201809898,
-8.73670574471733));
#31424=CARTESIAN_POINT('Ctrl Pts',(-39.4840611441388,-17.6857598217569,
-11.3734544105477));
#31425=CARTESIAN_POINT('Ctrl Pts',(-40.8595741644358,-18.4474896113716,
-12.4221714958517));
#31426=CARTESIAN_POINT('Ctrl Pts',(-43.899882870338,-20.1169735923652,-13.854590909534));
#31427=CARTESIAN_POINT('Ctrl Pts',(-45.5316698257919,-20.9956349957574,
-14.2195188101196));
#31428=CARTESIAN_POINT('Ctrl Pts',(-47.1721284105873,-21.8833834324347,
-14.2201291128084));
#31429=CARTESIAN_POINT('Ctrl Pts',(-37.2330519862577,-15.2134465003402,
1.47327608945385));
#31430=CARTESIAN_POINT('Ctrl Pts',(-37.1938800254351,-15.241283251608,1.01591367865882));
#31431=CARTESIAN_POINT('Ctrl Pts',(-37.1459775929371,-15.2672296481901,
0.528588449413829));
#31432=CARTESIAN_POINT('Ctrl Pts',(-37.0751310137706,-15.4196766250222,
-1.55405138009984));
#31433=CARTESIAN_POINT('Ctrl Pts',(-37.3050418083478,-15.6604198747703,
-3.10057294641723));
#31434=CARTESIAN_POINT('Ctrl Pts',(-38.2822972641641,-16.3841456768376,
-5.98227484333557));
#31435=CARTESIAN_POINT('Ctrl Pts',(-39.031143479052,-16.8620495708756,-7.29352824384753));
#31436=CARTESIAN_POINT('Ctrl Pts',(-40.9258582608669,-18.0025393609684,
-9.49167634241016));
#31437=CARTESIAN_POINT('Ctrl Pts',(-42.0684989791458,-18.6602832132111,
-10.369052486778));
#31438=CARTESIAN_POINT('Ctrl Pts',(-44.5835114688962,-20.0862790553914,
-11.5624766483363));
#31439=CARTESIAN_POINT('Ctrl Pts',(-45.945008519911,-20.8444200113532,-11.8682745707305));
#31440=CARTESIAN_POINT('Ctrl Pts',(-47.3011100364938,-21.6010088957271,
-11.8690397849987));
#31441=CARTESIAN_POINT('Ctrl Pts',(-39.5896190563861,-15.4515482289401,
1.35541228259756));
#31442=CARTESIAN_POINT('Ctrl Pts',(-39.5493344659456,-15.4801756476575,
0.885059075375416));
#31443=CARTESIAN_POINT('Ctrl Pts',(-39.5053728442148,-15.506492591361,0.42640858574592));
#31444=CARTESIAN_POINT('Ctrl Pts',(-39.4347037901406,-15.6571869876943,
-1.25364232211228));
#31445=CARTESIAN_POINT('Ctrl Pts',(-39.6132317302865,-15.8773787191765,
-2.51864171288157));
#31446=CARTESIAN_POINT('Ctrl Pts',(-40.3829362474672,-16.5028873873736,
-4.84795915807232));
#31447=CARTESIAN_POINT('Ctrl Pts',(-40.9828301658835,-16.9150240490638,
-5.91517020459162));
#31448=CARTESIAN_POINT('Ctrl Pts',(-42.4966234015636,-17.8805426753577,
-7.69457540347142));
#31449=CARTESIAN_POINT('Ctrl Pts',(-43.4170561364076,-18.4390645629071,
-8.40795287035897));
#31450=CARTESIAN_POINT('Ctrl Pts',(-45.4301680192413,-19.6324182482015,
-9.37372383743044));
#31451=CARTESIAN_POINT('Ctrl Pts',(-46.5336710320569,-20.2755208514245,
-9.62254086027733));
#31452=CARTESIAN_POINT('Ctrl Pts',(-47.618155754582,-20.9068289285809,-9.62369151535378));
#31453=CARTESIAN_POINT('Ctrl Pts',(-41.9477963710448,-15.224862147993,1.24768188077444));
#31454=CARTESIAN_POINT('Ctrl Pts',(-41.9064969112055,-15.2542107628561,
0.76547930207016));
#31455=CARTESIAN_POINT('Ctrl Pts',(-41.8661102394621,-15.2808564144436,
0.332966384797566));
#31456=CARTESIAN_POINT('Ctrl Pts',(-41.795273363368,-15.429797293463,-0.978922014651145));
#31457=CARTESIAN_POINT('Ctrl Pts',(-41.9273179171823,-15.6314258258578,
-1.98636136652118));
#31458=CARTESIAN_POINT('Ctrl Pts',(-42.5066521964273,-16.1668569942327,
-3.81078790535555));
#31459=CARTESIAN_POINT('Ctrl Pts',(-42.9706758457924,-16.519007778584,-4.654602649028));
#31460=CARTESIAN_POINT('Ctrl Pts',(-44.1359912383645,-17.3244581615128,
-6.05121512500453));
#31461=CARTESIAN_POINT('Ctrl Pts',(-44.853419877635,-17.7923352091663,-6.61423873300694));
#31462=CARTESIAN_POINT('Ctrl Pts',(-46.4073150662767,-18.7728332795684,
-7.37244739485722));
#31463=CARTESIAN_POINT('Ctrl Pts',(-47.275034524054,-19.3108003961669,-7.56862230213317));
#31464=CARTESIAN_POINT('Ctrl Pts',(-48.1110813316861,-19.827521231076,-7.57037421505994));
#31465=CARTESIAN_POINT('Ctrl Pts',(-36.007677782744,-11.6799141290249,1.59647068126645));
#31466=CARTESIAN_POINT('Ctrl Pts',(-35.9738923911276,-11.7120656519311,
1.15259163660754));
#31467=CARTESIAN_POINT('Ctrl Pts',(-35.9261470465067,-11.7447913705128,
0.635573001841871));
#31468=CARTESIAN_POINT('Ctrl Pts',(-35.8791430893777,-11.9080080866994,
-1.86858636174462));
#31469=CARTESIAN_POINT('Ctrl Pts',(-36.1952232408322,-12.1266171430312,
-3.71029995867732));
#31470=CARTESIAN_POINT('Ctrl Pts',(-37.4975806517,-12.775441558893,-7.1693624749576));
#31471=CARTESIAN_POINT('Ctrl Pts',(-38.469577866188,-13.1874595938152,-8.73699595771281));
#31472=CARTESIAN_POINT('Ctrl Pts',(-40.9286921018457,-14.17142472135,-11.3730256982067));
#31473=CARTESIAN_POINT('Ctrl Pts',(-42.3975559177885,-14.7293359258714,
-12.4235805192177));
#31474=CARTESIAN_POINT('Ctrl Pts',(-45.6456867796162,-15.9494910259031,
-13.8529470821644));
#31475=CARTESIAN_POINT('Ctrl Pts',(-47.3851293551721,-16.5867336459591,
-14.2204718556976));
#31476=CARTESIAN_POINT('Ctrl Pts',(-49.1354594857179,-17.2320701170946,
-14.2198708430666));
#31477=CARTESIAN_POINT('Ctrl Pts',(-35.6055008474196,-10.8171551228318,
1.62964612287405));
#31478=CARTESIAN_POINT('Ctrl Pts',(-35.5719973186168,-10.8490384138699,
1.18947024666155));
#31479=CARTESIAN_POINT('Ctrl Pts',(-35.5230856250742,-10.8818072974723,
0.664243958022171));
#31480=CARTESIAN_POINT('Ctrl Pts',(-35.47544064564,-11.0453235253696,-1.95287905124124));
#31481=CARTESIAN_POINT('Ctrl Pts',(-35.8076256583572,-11.2678861931963,
-3.87337387076198));
#31482=CARTESIAN_POINT('Ctrl Pts',(-37.1704123385762,-11.9353671582147,
-7.48792130216354));
#31483=CARTESIAN_POINT('Ctrl Pts',(-38.1870962603682,-12.3599059967852,
-9.12360836231895));
#31484=CARTESIAN_POINT('Ctrl Pts',(-40.7587332590465,-13.3771794922095,
-11.8774049927121));
#31485=CARTESIAN_POINT('Ctrl Pts',(-42.2936801020475,-13.9538940422505,
-12.9732563608771));
#31486=CARTESIAN_POINT('Ctrl Pts',(-45.6900265604505,-15.2184820528514,
-14.4676858045575));
#31487=CARTESIAN_POINT('Ctrl Pts',(-47.5060156561304,-15.8774655648083,
-14.8501851005579));
#31488=CARTESIAN_POINT('Ctrl Pts',(-49.3366907261818,-16.5467173899503,
-14.8499483202528));
#31489=CARTESIAN_POINT('Ctrl Pts',(-35.8740691471581,-9.90333289917197,
1.6297553058138));
#31490=CARTESIAN_POINT('Ctrl Pts',(-35.8405701742826,-9.93521185459824,
1.18963928645476));
#31491=CARTESIAN_POINT('Ctrl Pts',(-35.7915998644032,-9.96796916327536,
0.664246400093167));
#31492=CARTESIAN_POINT('Ctrl Pts',(-35.7432760306098,-10.1312860615242,
-1.95288623093664));
#31493=CARTESIAN_POINT('Ctrl Pts',(-36.0765018635479,-10.3541542972557,
-3.87317034516857));
#31494=CARTESIAN_POINT('Ctrl Pts',(-37.4381269352784,-11.0212942780522,
-7.48823335806122));
#31495=CARTESIAN_POINT('Ctrl Pts',(-38.4555234045969,-11.4460422796819,
-9.12349227712835));
#31496=CARTESIAN_POINT('Ctrl Pts',(-41.0269029710421,-12.4632402082154,
-11.877576477641));
#31497=CARTESIAN_POINT('Ctrl Pts',(-42.5622713807909,-13.0400785027476,
-12.9726927515335));
#31498=CARTESIAN_POINT('Ctrl Pts',(-45.9581475304014,-14.3045284731053,
-14.4683433355027));
#31499=CARTESIAN_POINT('Ctrl Pts',(-47.7744493565958,-14.9636108095647,
-14.8498038985338));
#31500=CARTESIAN_POINT('Ctrl Pts',(-49.6050326655023,-15.6328286697391,
-14.8500516281495));
#31501=CARTESIAN_POINT('Ctrl Pts',(-36.6790985320904,-9.39535856987525,
1.59674363861582));
#31502=CARTESIAN_POINT('Ctrl Pts',(-36.6453245303195,-9.42749925374606,
1.15301423608824));
#31503=CARTESIAN_POINT('Ctrl Pts',(-36.5974326448229,-9.46019603501911,
0.635579107019359));
#31504=CARTESIAN_POINT('Ctrl Pts',(-36.5487315518213,-9.62291442708968,
-1.86860431098312));
#31505=CARTESIAN_POINT('Ctrl Pts',(-36.8674137538258,-9.84228740318107,
-3.70979114469078));
#31506=CARTESIAN_POINT('Ctrl Pts',(-38.1668671434388,-10.4902593584854,
-7.17014261470479));
#31507=CARTESIAN_POINT('Ctrl Pts',(-39.1406457267621,-10.902800301061,-8.73670574473392));
#31508=CARTESIAN_POINT('Ctrl Pts',(-41.5991163818324,-11.8865765113604,
-11.3734544105312));
#31509=CARTESIAN_POINT('Ctrl Pts',(-43.0690341146564,-12.4447970771118,
-12.4221714958467));
#31510=CARTESIAN_POINT('Ctrl Pts',(-46.3159892044841,-13.6646070765402,
-13.8545909095391));
#31511=CARTESIAN_POINT('Ctrl Pts',(-48.0562134772108,-14.3020974767622,
-14.2195188099628));
#31512=CARTESIAN_POINT('Ctrl Pts',(-49.8063143340192,-14.9473483165667,
-14.2201291128084));
#31513=CARTESIAN_POINT('Ctrl Pts',(-35.914217116421,-11.7862169042732,0.));
#31514=CARTESIAN_POINT('Ctrl Pts',(-35.8791430893777,-11.9080080866994,
-1.86858636174462));
#31515=CARTESIAN_POINT('Ctrl Pts',(-36.1952232408322,-12.1266171430312,
-3.71029995867732));
#31516=CARTESIAN_POINT('Ctrl Pts',(-37.4975806517,-12.775441558893,-7.1693624749576));
#31517=CARTESIAN_POINT('Ctrl Pts',(-38.469577866188,-13.1874595938152,-8.73699595771042));
#31518=CARTESIAN_POINT('Ctrl Pts',(-39.8242114819221,-13.7294890038935,
-10.1890856763483));
#31519=CARTESIAN_POINT('Ctrl Pts',(-39.9517643117907,-13.7802180759912,
-10.3203928635135));
#31520=CARTESIAN_POINT('Ctrl Pts',(-40.0817049410149,-13.8316148870952,
-10.4488603765949));
#31521=CARTESIAN_POINT('Ctrl Pts',(-36.5850719698905,-9.5014950906651,-3.88578058618805E-16));
#31522=CARTESIAN_POINT('Ctrl Pts',(-36.5487315518213,-9.62291442708968,
-1.86860431098312));
#31523=CARTESIAN_POINT('Ctrl Pts',(-36.8674137538258,-9.84228740318107,
-3.70979114469078));
#31524=CARTESIAN_POINT('Ctrl Pts',(-38.1668671434388,-10.4902593584854,
-7.17014261470479));
#31525=CARTESIAN_POINT('Ctrl Pts',(-39.1406457267621,-10.902800301061,-8.73670574473392));
#31526=CARTESIAN_POINT('Ctrl Pts',(-40.5018374092127,-11.4474917709757,
-10.1966053555729));
#31527=CARTESIAN_POINT('Ctrl Pts',(-40.6365673070899,-11.5010595286717,
-10.3350231942294));
#31528=CARTESIAN_POINT('Ctrl Pts',(-40.7739629732778,-11.5553735590168,
-10.4702558451022));
#31529=CARTESIAN_POINT('Ctrl Pts',(-41.7419576204996,-15.7201209119709,
1.24689082988559));
#31530=CARTESIAN_POINT('Ctrl Pts',(-41.7052222707547,-15.7550797323953,
0.764254661700912));
#31531=CARTESIAN_POINT('Ctrl Pts',(-41.6694633881739,-15.7872856429804,
0.332948671129863));
#31532=CARTESIAN_POINT('Ctrl Pts',(-41.625461864821,-15.9462356620226,-0.978870002708281));
#31533=CARTESIAN_POINT('Ctrl Pts',(-41.777317093697,-16.124806375996,-1.98783577088221));
#31534=CARTESIAN_POINT('Ctrl Pts',(-42.435369447998,-16.574809961301,-3.80852727284257));
#31535=CARTESIAN_POINT('Ctrl Pts',(-42.9396243659164,-16.8558236638087,
-4.65544360725108));
#31536=CARTESIAN_POINT('Ctrl Pts',(-44.2095709903314,-17.4877814824203,
-6.04997283340197));
#31537=CARTESIAN_POINT('Ctrl Pts',(-44.9832291228107,-17.8478990309026,
-6.6183216989813));
#31538=CARTESIAN_POINT('Ctrl Pts',(-46.6642543902183,-18.5982747098319,
-7.36768403083496));
#31539=CARTESIAN_POINT('Ctrl Pts',(-47.5974477252332,-19.0065156676779,
-7.57138648693225));
#31540=CARTESIAN_POINT('Ctrl Pts',(-48.4991757443115,-19.3992863750338,
-7.56962581969416));
#31541=CARTESIAN_POINT('Ctrl Pts',(-40.1090570584212,-14.0037398626876,
1.35489321026565));
#31542=CARTESIAN_POINT('Ctrl Pts',(-40.0732349602028,-14.0378295966248,
0.884255518285778));
#31543=CARTESIAN_POINT('Ctrl Pts',(-40.0337447201299,-14.0701900799496,
0.426396949023618));
#31544=CARTESIAN_POINT('Ctrl Pts',(-39.9884678119751,-14.2303553472505,
-1.2536081950084));
#31545=CARTESIAN_POINT('Ctrl Pts',(-40.1915678319234,-14.4214462185192,
-2.51960912778971));
#31546=CARTESIAN_POINT('Ctrl Pts',(-41.0479784866769,-14.9326685312541,
-4.84647586783093));
#31547=CARTESIAN_POINT('Ctrl Pts',(-41.6970325717046,-15.2542422185918,
-5.91572199048531));
#31548=CARTESIAN_POINT('Ctrl Pts',(-43.3340488506278,-15.994857208877,-7.69376028690158));
#31549=CARTESIAN_POINT('Ctrl Pts',(-44.322595033069,-16.4161147204105,-8.41063186553746));
#31550=CARTESIAN_POINT('Ctrl Pts',(-46.4872837874829,-17.3114822382755,
-9.37059840622849));
#31551=CARTESIAN_POINT('Ctrl Pts',(-47.6695948287912,-17.7905076322675,
-9.624353786323));
#31552=CARTESIAN_POINT('Ctrl Pts',(-48.8333181822473,-18.2612298390049,
-9.62320046360533));
#31553=CARTESIAN_POINT('Ctrl Pts',(-38.1728270004195,-12.6395284821798,
1.47293192394313));
#31554=CARTESIAN_POINT('Ctrl Pts',(-38.1380009815277,-12.6726703073981,
1.01538091584584));
#31555=CARTESIAN_POINT('Ctrl Pts',(-38.0944634070467,-12.7052063084716,
0.528580717863993));
#31556=CARTESIAN_POINT('Ctrl Pts',(-38.0481727007017,-12.8668122636162,
-1.55402875455616));
#31557=CARTESIAN_POINT('Ctrl Pts',(-38.3067247111946,-13.0714224335838,
-3.10121432122184));
#31558=CARTESIAN_POINT('Ctrl Pts',(-39.3806906392157,-13.6497783496959,
-5.98129145452209));
#31559=CARTESIAN_POINT('Ctrl Pts',(-40.1876820275573,-14.0155868029206,
-7.29389406576927));
#31560=CARTESIAN_POINT('Ctrl Pts',(-42.2262312169725,-14.8750601592863,
-9.4911359380372));
#31561=CARTESIAN_POINT('Ctrl Pts',(-43.4495197173534,-15.36310443968,-10.3708286017026));
#31562=CARTESIAN_POINT('Ctrl Pts',(-46.1433554687509,-16.4170971138883,
-11.5604045561393));
#31563=CARTESIAN_POINT('Ctrl Pts',(-47.5979046271491,-16.9734434882789,
-11.8694761541855));
#31564=CARTESIAN_POINT('Ctrl Pts',(-49.0481649878422,-17.5294501945615,
-11.8687142284811));
#31565=CARTESIAN_POINT('Ctrl Pts',(-36.007677782744,-11.6799141290249,1.59647068126645));
#31566=CARTESIAN_POINT('Ctrl Pts',(-35.9738923911276,-11.7120656519311,
1.15259163660754));
#31567=CARTESIAN_POINT('Ctrl Pts',(-35.9261470465067,-11.7447913705128,
0.635573001841871));
#31568=CARTESIAN_POINT('Ctrl Pts',(-35.8791430893777,-11.9080080866994,
-1.86858636174462));
#31569=CARTESIAN_POINT('Ctrl Pts',(-36.1952232408322,-12.1266171430312,
-3.71029995867732));
#31570=CARTESIAN_POINT('Ctrl Pts',(-37.4975806517,-12.775441558893,-7.1693624749576));
#31571=CARTESIAN_POINT('Ctrl Pts',(-38.469577866188,-13.1874595938152,-8.73699595771042));
#31572=CARTESIAN_POINT('Ctrl Pts',(-40.9286921018457,-14.17142472135,-11.3730256982091));
#31573=CARTESIAN_POINT('Ctrl Pts',(-42.3975559177885,-14.7293359258726,
-12.4235805192177));
#31574=CARTESIAN_POINT('Ctrl Pts',(-45.6456867796163,-15.9494910259019,
-13.8529470821644));
#31575=CARTESIAN_POINT('Ctrl Pts',(-47.3851293551747,-16.5867336459529,
-14.2204718556976));
#31576=CARTESIAN_POINT('Ctrl Pts',(-49.1354594857179,-17.2320701170946,
-14.2198708430666));
#31577=CARTESIAN_POINT('Ctrl Pts',(-36.6790985320904,-9.39535856987524,
1.59674363861582));
#31578=CARTESIAN_POINT('Ctrl Pts',(-36.6453245303195,-9.42749925374605,
1.15301423608824));
#31579=CARTESIAN_POINT('Ctrl Pts',(-36.5974326448229,-9.46019603501911,
0.635579107019359));
#31580=CARTESIAN_POINT('Ctrl Pts',(-36.5487315518213,-9.62291442708968,
-1.86860431098312));
#31581=CARTESIAN_POINT('Ctrl Pts',(-36.8674137538258,-9.84228740318107,
-3.70979114469079));
#31582=CARTESIAN_POINT('Ctrl Pts',(-38.1668671434388,-10.4902593584854,
-7.17014261470479));
#31583=CARTESIAN_POINT('Ctrl Pts',(-39.1406457267669,-10.902800301061,-8.73670574473393));
#31584=CARTESIAN_POINT('Ctrl Pts',(-41.5991163818276,-11.8865765113604,
-11.3734544105312));
#31585=CARTESIAN_POINT('Ctrl Pts',(-43.0690341146515,-12.4447970771106,
-12.4221714958515));
#31586=CARTESIAN_POINT('Ctrl Pts',(-46.3159892044889,-13.6646070765414,
-13.8545909095343));
#31587=CARTESIAN_POINT('Ctrl Pts',(-48.0562134772077,-14.3020974767599,
-14.2195188099628));
#31588=CARTESIAN_POINT('Ctrl Pts',(-49.8063143340192,-14.9473483165667,
-14.2201291128085));
#31589=CARTESIAN_POINT('Ctrl Pts',(-39.019172373722,-9.7597797859694,1.47327599461711));
#31590=CARTESIAN_POINT('Ctrl Pts',(-38.9843607120683,-9.79290794827359,
1.01591361477635));
#31591=CARTESIAN_POINT('Ctrl Pts',(-38.940638418548,-9.82540747302369,0.528588413617701));
#31592=CARTESIAN_POINT('Ctrl Pts',(-38.8922084230933,-9.98638527613126,
-1.55405138009309));
#31593=CARTESIAN_POINT('Ctrl Pts',(-39.1540403939526,-10.1919583891645,
-3.10057294640141));
#31594=CARTESIAN_POINT('Ctrl Pts',(-40.2243457187586,-10.7692397539638,
-5.98227484335149));
#31595=CARTESIAN_POINT('Ctrl Pts',(-41.0335825742976,-11.1357073474839,
-7.29352824387615));
#31596=CARTESIAN_POINT('Ctrl Pts',(-43.071320511685,-11.9949425681867,-9.4916763423817));
#31597=CARTESIAN_POINT('Ctrl Pts',(-44.2959375049236,-12.4833768074015,
-10.3690524867827));
#31598=CARTESIAN_POINT('Ctrl Pts',(-46.9882911615408,-13.5369344722681,
-11.5624766483318));
#31599=CARTESIAN_POINT('Ctrl Pts',(-48.4438248432715,-14.0935974137185,
-11.8682745705641));
#31600=CARTESIAN_POINT('Ctrl Pts',(-49.8937970264261,-14.6494919462611,
-11.8690397849988));
#31601=CARTESIAN_POINT('Ctrl Pts',(-41.3856383979639,-9.66008352082097,
1.35541218776083));
#31602=CARTESIAN_POINT('Ctrl Pts',(-41.3498379554194,-9.69415264636012,
0.885059012386286));
#31603=CARTESIAN_POINT('Ctrl Pts',(-41.3100690951961,-9.72645811078408,
0.426408556880046));
#31604=CARTESIAN_POINT('Ctrl Pts',(-41.2615653996735,-9.88567590770738,
-1.25364232213799));
#31605=CARTESIAN_POINT('Ctrl Pts',(-41.4696127334847,-10.0782192299367,
-2.51864171288723));
#31606=CARTESIAN_POINT('Ctrl Pts',(-42.3205019334041,-10.5878207479002,
-4.84795915806691));
#31607=CARTESIAN_POINT('Ctrl Pts',(-42.9729429590492,-10.9103886466196,
-5.91517020462989));
#31608=CARTESIAN_POINT('Ctrl Pts',(-44.6087355895268,-11.6506444460178,
-7.69457540343341));
#31609=CARTESIAN_POINT('Ctrl Pts',(-45.5992855983476,-12.0724901502325,
-8.4079528703733));
#31610=CARTESIAN_POINT('Ctrl Pts',(-47.7617388416023,-12.9672015236625,
-9.37372383741637));
#31611=CARTESIAN_POINT('Ctrl Pts',(-48.9455328277903,-13.446713416981,-9.62254086002058));
#31612=CARTESIAN_POINT('Ctrl Pts',(-50.1088235664895,-13.9172574201605,
-9.62369151535393));
#31613=CARTESIAN_POINT('Ctrl Pts',(-43.6875520748214,-9.100101154168,1.24768178593771));
#31614=CARTESIAN_POINT('Ctrl Pts',(-43.6508497297522,-9.13502856602996,
0.765479239891048));
#31615=CARTESIAN_POINT('Ctrl Pts',(-43.6146662116282,-9.1671506241679,0.332966362271342));
#31616=CARTESIAN_POINT('Ctrl Pts',(-43.5657468507465,-9.32465663564633,
-0.978922014712551));
#31617=CARTESIAN_POINT('Ctrl Pts',(-43.7251421134098,-9.50544098101819,
-1.98636136653877));
#31618=CARTESIAN_POINT('Ctrl Pts',(-44.3747794050838,-9.95297436781101,
-3.81078790533841));
#31619=CARTESIAN_POINT('Ctrl Pts',(-44.8841962446822,-10.2355033142702,
-4.6546026490903));
#31620=CARTESIAN_POINT('Ctrl Pts',(-46.1522779478725,-10.8669137021975,
-6.05121512494264));
#31621=CARTESIAN_POINT('Ctrl Pts',(-46.9289900443881,-11.2279276952588,
-6.61423873304056));
#31622=CARTESIAN_POINT('Ctrl Pts',(-48.6066082448179,-11.9773033666356,
-7.37244739482399));
#31623=CARTESIAN_POINT('Ctrl Pts',(-49.5420562727445,-12.3863053996863,
-7.56862230172892));
#31624=CARTESIAN_POINT('Ctrl Pts',(-50.4431303715412,-12.7787848949965,
-7.57037421506017));
#31625=CARTESIAN_POINT('Ctrl Pts',(-37.3033966274914,-6.43660260973375,
1.59647061166179));
#31626=CARTESIAN_POINT('Ctrl Pts',(-37.2745307626585,-6.47323503721974,
1.15259158903741));
#31627=CARTESIAN_POINT('Ctrl Pts',(-37.2319287549561,-6.51242252436172,
0.635572970257452));
#31628=CARTESIAN_POINT('Ctrl Pts',(-37.2086313911891,-6.68066728817659,
-1.86858636175417));
#31629=CARTESIAN_POINT('Ctrl Pts',(-37.5526056149658,-6.85206832389808,
-3.71029995869313));
#31630=CARTESIAN_POINT('Ctrl Pts',(-38.9340442470254,-7.30894385837246,
-7.16936247494213));
#31631=CARTESIAN_POINT('Ctrl Pts',(-39.9547842113923,-7.57843851744686,
-8.73699595769433));
#31632=CARTESIAN_POINT('Ctrl Pts',(-42.5289010478687,-8.20241985396338,
-11.3730256982255));
#31633=CARTESIAN_POINT('Ctrl Pts',(-44.0622129909323,-8.54561121037124,
-12.4235805192426));
#31634=CARTESIAN_POINT('Ctrl Pts',(-47.4509287397419,-9.2910896727123,-13.8529470821398));
#31635=CARTESIAN_POINT('Ctrl Pts',(-49.2633553782971,-9.67429759299236,
-14.2204718555978));
#31636=CARTESIAN_POINT('Ctrl Pts',(-51.0877106274638,-10.063967519702,-14.2198708430667));
#31637=CARTESIAN_POINT('Ctrl Pts',(-36.7825298650421,-5.63986099173596,
1.62964605326941));
#31638=CARTESIAN_POINT('Ctrl Pts',(-36.7539048206774,-5.67618780432318,
1.18947019889892));
#31639=CARTESIAN_POINT('Ctrl Pts',(-36.7101544788345,-5.7155840058739,0.664243925013534));
#31640=CARTESIAN_POINT('Ctrl Pts',(-36.6862652424053,-5.88421645978634,
-1.95287905125288));
#31641=CARTESIAN_POINT('Ctrl Pts',(-37.0467430607447,-6.05723890421492,
-3.87337387078137));
#31642=CARTESIAN_POINT('Ctrl Pts',(-38.4906509831416,-6.5239811093709,-7.48792130214445));
#31643=CARTESIAN_POINT('Ctrl Pts',(-39.5574047046893,-6.79950954685142,
-9.12360836230283));
#31644=CARTESIAN_POINT('Ctrl Pts',(-42.2476392596962,-7.44044656127135,
-11.8774049927284));
#31645=CARTESIAN_POINT('Ctrl Pts',(-43.8490375949647,-7.79284527693345,
-12.9732563608876));
#31646=CARTESIAN_POINT('Ctrl Pts',(-47.3907837817603,-8.56121110825465,
-14.4676858045473));
#31647=CARTESIAN_POINT('Ctrl Pts',(-49.2820718587483,-8.9550449238883,-14.8501851004961));
#31648=CARTESIAN_POINT('Ctrl Pts',(-51.1893577615276,-9.3569525036808,-14.8499483202528));
#31649=CARTESIAN_POINT('Ctrl Pts',(-36.918314064762,-4.69711890654748,1.62975523620919));
#31650=CARTESIAN_POINT('Ctrl Pts',(-36.8896929129475,-4.73344077927094,
1.18963923868388));
#31651=CARTESIAN_POINT('Ctrl Pts',(-36.8458829040885,-4.77283386569197,
0.664246367084094));
#31652=CARTESIAN_POINT('Ctrl Pts',(-36.8212933554976,-4.94136562989336,
-1.95288623094736));
#31653=CARTESIAN_POINT('Ctrl Pts',(-37.1828448868644,-5.11454240782316,
-3.87317034518908));
#31654=CARTESIAN_POINT('Ctrl Pts',(-38.6255544971456,-5.58111241361319,
-7.48823335804086));
#31655=CARTESIAN_POINT('Ctrl Pts',(-39.6930432805175,-5.85674647908712,
-9.12349227711692));
#31656=CARTESIAN_POINT('Ctrl Pts',(-42.3830122693083,-6.49764533220352,
-11.8775764776524));
#31657=CARTESIAN_POINT('Ctrl Pts',(-43.9848454910638,-6.85010653761332,
-12.9726927515151));
#31658=CARTESIAN_POINT('Ctrl Pts',(-47.5261065109321,-7.61840266566205,
-14.4683433355211));
#31659=CARTESIAN_POINT('Ctrl Pts',(-49.4177181995047,-8.01228979371233,
-14.8498038985148));
#31660=CARTESIAN_POINT('Ctrl Pts',(-51.3249084414063,-8.41417681322632,
-14.8500516281495));
#31661=CARTESIAN_POINT('Ctrl Pts',(-37.6428571267913,-4.07974739676256,
1.59674356901123));
#31662=CARTESIAN_POINT('Ctrl Pts',(-37.6140009933228,-4.11636747458817,
1.15301418850057));
#31663=CARTESIAN_POINT('Ctrl Pts',(-37.5712498180903,-4.15554717390732,
0.635579075433858));
#31664=CARTESIAN_POINT('Ctrl Pts',(-37.5462016739223,-4.32354021344296,
-1.86860431099037));
#31665=CARTESIAN_POINT('Ctrl Pts',(-37.8928601802435,-4.4953270829205,-3.70979114471123));
#31666=CARTESIAN_POINT('Ctrl Pts',(-39.2713030320569,-4.95177211897637,
-7.17014261468437));
#31667=CARTESIAN_POINT('Ctrl Pts',(-40.2938806509817,-5.22153084803759,
-8.73670574472958));
#31668=CARTESIAN_POINT('Ctrl Pts',(-42.8673335718798,-5.84541678129231,
-11.3734544105354));
#31669=CARTESIAN_POINT('Ctrl Pts',(-44.4017327311728,-6.18876436207153,
-12.4221714958137));
#31670=CARTESIAN_POINT('Ctrl Pts',(-47.7892355626787,-6.93406856623023,
-13.8545909095719));
#31671=CARTESIAN_POINT('Ctrl Pts',(-49.6024712046778,-7.31741049752272,
-14.219518810015));
#31672=CARTESIAN_POINT('Ctrl Pts',(-51.4265873271606,-7.70702829356582,
-14.2201291128083));
#31673=CARTESIAN_POINT('Ctrl Pts',(-37.2260157227863,-6.55512420987395,
0.));
#31674=CARTESIAN_POINT('Ctrl Pts',(-37.2086313911891,-6.6806672881766,-1.86858636175417));
#31675=CARTESIAN_POINT('Ctrl Pts',(-37.5526056149658,-6.85206832389809,
-3.71029995869313));
#31676=CARTESIAN_POINT('Ctrl Pts',(-38.9340442470254,-7.30894385837246,
-7.16936247494213));
#31677=CARTESIAN_POINT('Ctrl Pts',(-39.9547842113923,-7.57843851744686,
-8.73699595769433));
#31678=CARTESIAN_POINT('Ctrl Pts',(-41.3727684379707,-7.92216638570902,
-10.1890856763496));
#31679=CARTESIAN_POINT('Ctrl Pts',(-41.5062424636379,-7.95422644864132,
-10.320392863516));
#31680=CARTESIAN_POINT('Ctrl Pts',(-41.6421750134749,-7.98660763468004,
-10.4488603765984));
#31681=CARTESIAN_POINT('Ctrl Pts',(-37.5648924257372,-4.19818497005525,
2.22044604925031E-16));
#31682=CARTESIAN_POINT('Ctrl Pts',(-37.5462016739223,-4.32354021344296,
-1.86860431099037));
#31683=CARTESIAN_POINT('Ctrl Pts',(-37.8928601802435,-4.4953270829205,-3.70979114471123));
#31684=CARTESIAN_POINT('Ctrl Pts',(-39.2713030320569,-4.95177211897637,
-7.17014261468437));
#31685=CARTESIAN_POINT('Ctrl Pts',(-40.2938806509817,-5.22153084803759,
-8.73670574472958));
#31686=CARTESIAN_POINT('Ctrl Pts',(-41.7187350432356,-5.56696037000185,
-10.196605355573));
#31687=CARTESIAN_POINT('Ctrl Pts',(-41.8597170717902,-5.60080882153321,
-10.3350231942292));
#31688=CARTESIAN_POINT('Ctrl Pts',(-42.0034439406492,-5.63501657134766,
-10.4702558451014));
#31689=CARTESIAN_POINT('Ctrl Pts',(-43.5542911395532,-9.61961280540204,
1.24689076028084));
#31690=CARTESIAN_POINT('Ctrl Pts',(-43.5229048631346,-9.65944377882554,
0.764254616128654));
#31691=CARTESIAN_POINT('Ctrl Pts',(-43.4920933360729,-9.69641089756863,
0.332948654576497));
#31692=CARTESIAN_POINT('Ctrl Pts',(-43.4711606313199,-9.86000510219415,
-0.978870002690684));
#31693=CARTESIAN_POINT('Ctrl Pts',(-43.64688345522,-10.0151469714386,-1.98783577088957));
#31694=CARTESIAN_POINT('Ctrl Pts',(-44.3622799727875,-10.3669195547583,
-3.80852727283549));
#31695=CARTESIAN_POINT('Ctrl Pts',(-44.9013947224019,-10.5733099858333,
-4.65544360724204));
#31696=CARTESIAN_POINT('Ctrl Pts',(-46.2483520959889,-11.0181031366258,
-6.04997283341153));
#31697=CARTESIAN_POINT('Ctrl Pts',(-47.0653855748303,-11.2644521757634,
-6.61832169905394));
#31698=CARTESIAN_POINT('Ctrl Pts',(-48.8360900223873,-11.7679552730237,
-7.36768403076297));
#31699=CARTESIAN_POINT('Ctrl Pts',(-49.8178835406428,-12.0392336678774,
-7.57138648670422));
#31700=CARTESIAN_POINT('Ctrl Pts',(-50.7663303683512,-12.2996772587581,
-7.56962581969452));
#31701=CARTESIAN_POINT('Ctrl Pts',(-41.6937446593044,-8.15308801979197,
1.35489314066094));
#31702=CARTESIAN_POINT('Ctrl Pts',(-41.6631386548957,-8.191928783576,0.884255472092365));
#31703=CARTESIAN_POINT('Ctrl Pts',(-41.6286557481926,-8.2295799292397,0.426396927828607));
#31704=CARTESIAN_POINT('Ctrl Pts',(-41.6066335880859,-8.39455851882582,
-1.25360819499871));
#31705=CARTESIAN_POINT('Ctrl Pts',(-41.8348614091216,-8.55480021406848,
-2.51960912779946));
#31706=CARTESIAN_POINT('Ctrl Pts',(-42.755309558977,-8.93893907696394,-4.84647586782143));
#31707=CARTESIAN_POINT('Ctrl Pts',(-43.4435219166218,-9.16486958068287,
-5.91572199047626));
#31708=CARTESIAN_POINT('Ctrl Pts',(-45.1692762327319,-9.66497447127328,
-7.69376028691099));
#31709=CARTESIAN_POINT('Ctrl Pts',(-46.2077116350052,-9.94125939867522,
-8.41063186558134));
#31710=CARTESIAN_POINT('Ctrl Pts',(-48.4777910627081,-10.5194460361869,
-9.37059840618507));
#31711=CARTESIAN_POINT('Ctrl Pts',(-49.7162403037897,-10.8253352376767,
-9.62435378616625));
#31712=CARTESIAN_POINT('Ctrl Pts',(-50.9351093861917,-11.1256510703087,
-9.62320046360557));
#31713=CARTESIAN_POINT('Ctrl Pts',(-39.5830751094923,-7.07831661167196,
1.47293185433845));
#31714=CARTESIAN_POINT('Ctrl Pts',(-39.5533201442369,-7.11607735826761,
1.0153808689781));
#31715=CARTESIAN_POINT('Ctrl Pts',(-39.5148560779746,-7.15447823086432,
0.528580691593616));
#31716=CARTESIAN_POINT('Ctrl Pts',(-39.4920354699321,-7.32102712269281,
-1.55402875455564));
#31717=CARTESIAN_POINT('Ctrl Pts',(-39.7770748570174,-7.48675886860325,
-3.1012143212364));
#31718=CARTESIAN_POINT('Ctrl Pts',(-40.9224179890687,-7.90638666802899,
-5.98129145450779));
#31719=CARTESIAN_POINT('Ctrl Pts',(-41.7732553395368,-8.15362486974972,
-7.29389406576026));
#31720=CARTESIAN_POINT('Ctrl Pts',(-43.9133708492508,-8.71423422839074,
-9.49113593804649));
#31721=CARTESIAN_POINT('Ctrl Pts',(-45.1936639793565,-9.02321881658609,
-10.3708286017322));
#31722=CARTESIAN_POINT('Ctrl Pts',(-48.0100791640002,-9.68311056588415,
-11.5604045561101));
#31723=CARTESIAN_POINT('Ctrl Pts',(-49.5289994534967,-10.0267902081586,
-11.8694761540715));
#31724=CARTESIAN_POINT('Ctrl Pts',(-51.0436262593385,-10.3707439991146,
-11.8687142284813));
#31725=CARTESIAN_POINT('Ctrl Pts',(-37.3033966274914,-6.43660260973375,
1.59647061166179));
#31726=CARTESIAN_POINT('Ctrl Pts',(-37.2745307626585,-6.47323503721974,
1.15259158903741));
#31727=CARTESIAN_POINT('Ctrl Pts',(-37.2319287549561,-6.51242252436172,
0.635572970257452));
#31728=CARTESIAN_POINT('Ctrl Pts',(-37.2086313911891,-6.6806672881766,-1.86858636175417));
#31729=CARTESIAN_POINT('Ctrl Pts',(-37.5526056149658,-6.85206832389808,
-3.71029995869313));
#31730=CARTESIAN_POINT('Ctrl Pts',(-38.9340442470254,-7.30894385837246,
-7.16936247494213));
#31731=CARTESIAN_POINT('Ctrl Pts',(-39.9547842113923,-7.57843851744686,
-8.73699595769433));
#31732=CARTESIAN_POINT('Ctrl Pts',(-42.5289010478687,-8.2024198539634,-11.3730256982255));
#31733=CARTESIAN_POINT('Ctrl Pts',(-44.0622129909323,-8.54561121037124,
-12.4235805192426));
#31734=CARTESIAN_POINT('Ctrl Pts',(-47.4509287397419,-9.2910896727123,-13.8529470821398));
#31735=CARTESIAN_POINT('Ctrl Pts',(-49.263355378298,-9.67429759298781,-14.2204718555978));
#31736=CARTESIAN_POINT('Ctrl Pts',(-51.0877106274638,-10.063967519702,-14.2198708430667));
#31737=CARTESIAN_POINT('Ctrl Pts',(-37.6428571267913,-4.07974739676256,
1.59674356901123));
#31738=CARTESIAN_POINT('Ctrl Pts',(-37.6140009933228,-4.11636747458817,
1.15301418850057));
#31739=CARTESIAN_POINT('Ctrl Pts',(-37.5712498180903,-4.15554717390732,
0.635579075433858));
#31740=CARTESIAN_POINT('Ctrl Pts',(-37.5462016739223,-4.32354021344296,
-1.86860431099037));
#31741=CARTESIAN_POINT('Ctrl Pts',(-37.8928601802435,-4.4953270829205,-3.70979114471123));
#31742=CARTESIAN_POINT('Ctrl Pts',(-39.2713030320569,-4.95177211897636,
-7.17014261468437));
#31743=CARTESIAN_POINT('Ctrl Pts',(-40.2938806509817,-5.22153084803759,
-8.73670574472958));
#31744=CARTESIAN_POINT('Ctrl Pts',(-42.8673335718798,-5.84541678129231,
-11.3734544105354));
#31745=CARTESIAN_POINT('Ctrl Pts',(-44.4017327311728,-6.18876436207153,
-12.4221714958137));
#31746=CARTESIAN_POINT('Ctrl Pts',(-47.7892355626787,-6.93406856623022,
-13.8545909095719));
#31747=CARTESIAN_POINT('Ctrl Pts',(-49.6024712046779,-7.31741049752216,
-14.219518810015));
#31748=CARTESIAN_POINT('Ctrl Pts',(-51.4265873271606,-7.70702829356582,
-14.2201291128083));
#31749=CARTESIAN_POINT('Ctrl Pts',(-40.0109749372547,-4.10743210000935,
1.47327592501251));
#31750=CARTESIAN_POINT('Ctrl Pts',(-39.9812322386616,-4.14517727949942,
1.01591356788712));
#31751=CARTESIAN_POINT('Ctrl Pts',(-39.9425801423964,-4.18356833531871,
0.528588387345957));
#31752=CARTESIAN_POINT('Ctrl Pts',(-39.9175526247628,-4.34979992137534,
-1.55405138008967));
#31753=CARTESIAN_POINT('Ctrl Pts',(-40.2059756280345,-4.51601802195226,
-3.10057294641937));
#31754=CARTESIAN_POINT('Ctrl Pts',(-41.3475424919847,-4.93510316560563,
-5.9822748433334));
#31755=CARTESIAN_POINT('Ctrl Pts',(-42.200696259442,-5.18267423522269,-7.29352824387884));
#31756=CARTESIAN_POINT('Ctrl Pts',(-44.3399748842863,-5.74316333527725,
-9.49167634237876));
#31757=CARTESIAN_POINT('Ctrl Pts',(-45.6216384820464,-6.05234484883429,
-10.3690524867304));
#31758=CARTESIAN_POINT('Ctrl Pts',(-48.4365247491692,-6.71201694062915,
-11.5624766483838));
#31759=CARTESIAN_POINT('Ctrl Pts',(-49.9564645932,-7.05586981549073,-11.8682745705877));
#31760=CARTESIAN_POINT('Ctrl Pts',(-51.4707901907297,-7.39975358641511,
-11.8690397849987));
#31761=CARTESIAN_POINT('Ctrl Pts',(-42.339165491681,-3.67196736957056,1.35541211815623));
#31762=CARTESIAN_POINT('Ctrl Pts',(-42.3085779896418,-3.71078465277919,
0.885058966159984));
#31763=CARTESIAN_POINT('Ctrl Pts',(-42.2738114687052,-3.74842099134944,
0.426408535682965));
#31764=CARTESIAN_POINT('Ctrl Pts',(-42.2484605261705,-3.91292097416349,
-1.25364232212393));
#31765=CARTESIAN_POINT('Ctrl Pts',(-42.4817920098702,-4.07389626033816,
-2.51864171289909));
#31766=CARTESIAN_POINT('Ctrl Pts',(-43.396544242274,-4.45721661077528,-4.84795915805471));
#31767=CARTESIAN_POINT('Ctrl Pts',(-44.0882505573392,-4.68364919432705,
-5.91517020464438));
#31768=CARTESIAN_POINT('Ctrl Pts',(-45.8127425618219,-5.18357269340747,
-7.6945754034185));
#31769=CARTESIAN_POINT('Ctrl Pts',(-46.8532451029838,-5.46015465231553,
-8.40795287030642));
#31770=CARTESIAN_POINT('Ctrl Pts',(-49.1210183946318,-6.03800997039364,
-9.37372383748275));
#31771=CARTESIAN_POINT('Ctrl Pts',(-50.3610047224977,-6.3441696743126,-9.62254086010597));
#31772=CARTESIAN_POINT('Ctrl Pts',(-51.5794202324976,-6.64437068472187,
-9.62369151535368));
#31773=CARTESIAN_POINT('Ctrl Pts',(-44.5379552064474,-2.790088343341,1.24768171633315));
#31774=CARTESIAN_POINT('Ctrl Pts',(-44.5065971288718,-2.82988353081354,
0.765479194268018));
#31775=CARTESIAN_POINT('Ctrl Pts',(-44.4753533549367,-2.86682808256602,
0.332966345714832));
#31776=CARTESIAN_POINT('Ctrl Pts',(-44.4493473654519,-3.02969285879393,
-0.978922014688285));
#31777=CARTESIAN_POINT('Ctrl Pts',(-44.6328485090435,-3.18595276917332,
-1.98636136655288));
#31778=CARTESIAN_POINT('Ctrl Pts',(-45.3395640714125,-3.53647788533013,
-3.81078790532369));
#31779=CARTESIAN_POINT('Ctrl Pts',(-45.8840038433993,-3.7436335193008,-4.65460264911415));
#31780=CARTESIAN_POINT('Ctrl Pts',(-47.229037370506,-4.18815021742915,-6.0512151249181));
#31781=CARTESIAN_POINT('Ctrl Pts',(-48.0492213058428,-4.4349519522404,-6.61423873293507));
#31782=CARTESIAN_POINT('Ctrl Pts',(-49.8164110494045,-4.93795009675474,
-7.3724473949287));
#31783=CARTESIAN_POINT('Ctrl Pts',(-50.8005446234514,-5.20966094395016,
-7.56862230188086));
#31784=CARTESIAN_POINT('Ctrl Pts',(-51.7483027430072,-5.46990934942787,
-7.57037421505979));
#31785=CARTESIAN_POINT('Ctrl Pts',(-37.8397258902528,-1.06226042836983,
1.59647049649061));
#31786=CARTESIAN_POINT('Ctrl Pts',(-37.8163671782138,-1.10262802813137,
1.15259151033015));
#31787=CARTESIAN_POINT('Ctrl Pts',(-37.7797757625724,-1.14747953738618,
0.635572917992124));
#31788=CARTESIAN_POINT('Ctrl Pts',(-37.7806592587368,-1.3173273690917,-1.86858636175756));
#31789=CARTESIAN_POINT('Ctrl Pts',(-38.1455252315402,-1.43803115336822,
-3.71029995869359));
#31790=CARTESIAN_POINT('Ctrl Pts',(-39.5779229780038,-1.6936571382057,-7.16936247494164));
#31791=CARTESIAN_POINT('Ctrl Pts',(-40.6266263701707,-1.81514228728191,
-8.73699595770662));
#31792=CARTESIAN_POINT('Ctrl Pts',(-43.2633442117449,-2.06643737217002,
-11.3730256982132));
#31793=CARTESIAN_POINT('Ctrl Pts',(-44.8298904725261,-2.18792249430067,
-12.423580519232));
#31794=CARTESIAN_POINT('Ctrl Pts',(-48.290206627889,-2.44354852691099,-13.8529470821504));
#31795=CARTESIAN_POINT('Ctrl Pts',(-50.1387215498246,-2.56492073909757,
-14.2204718556739));
#31796=CARTESIAN_POINT('Ctrl Pts',(-51.9999633056261,-2.69099156569442,
-14.2198708430667));
#31797=CARTESIAN_POINT('Ctrl Pts',(-37.2107726459064,-0.347755560296676,
1.62964593809825));
#31798=CARTESIAN_POINT('Ctrl Pts',(-37.187608809593,-0.387786383581497,
1.18947011987297));
#31799=CARTESIAN_POINT('Ctrl Pts',(-37.149910451344,-0.433007907801872,
0.664243870391023));
#31800=CARTESIAN_POINT('Ctrl Pts',(-37.1502632733282,-0.60332371572967,
-1.95287905125797));
#31801=CARTESIAN_POINT('Ctrl Pts',(-37.5316956084247,-0.723283698714533,
-3.87337387077939));
#31802=CARTESIAN_POINT('Ctrl Pts',(-39.0273309715372,-0.979785618813286,
-7.48792130214639));
#31803=CARTESIAN_POINT('Ctrl Pts',(-40.122438463387,-1.10069469071833,-9.12360836231754));
#31804=CARTESIAN_POINT('Ctrl Pts',(-42.8765051571204,-1.35224759481462,
-11.8774049927137));
#31805=CARTESIAN_POINT('Ctrl Pts',(-44.5117551326353,-1.4731566546783,-12.9732563608865));
#31806=CARTESIAN_POINT('Ctrl Pts',(-48.1268013090037,-1.72965859379875,
-14.4676858045483));
#31807=CARTESIAN_POINT('Ctrl Pts',(-50.0548871962075,-1.85032539217923,
-14.8501851005246));
#31808=CARTESIAN_POINT('Ctrl Pts',(-51.9999570907662,-1.97670704765964,
-14.8499483202528));
#31809=CARTESIAN_POINT('Ctrl Pts',(-37.2110085708708,0.604714876209623,
1.62975512103804));
#31810=CARTESIAN_POINT('Ctrl Pts',(-37.1878478844851,0.564689496473117,
1.18963915964644));
#31811=CARTESIAN_POINT('Ctrl Pts',(-37.1500900231858,0.5194625641754,0.664246312460969));
#31812=CARTESIAN_POINT('Ctrl Pts',(-37.1497353315531,0.349146756271212,
-1.95288623095124));
#31813=CARTESIAN_POINT('Ctrl Pts',(-37.5322524147683,0.229186815971294,
-3.87317034518232));
#31814=CARTESIAN_POINT('Ctrl Pts',(-39.0266771563376,-0.0273151950943185,
-7.48823335804761));
#31815=CARTESIAN_POINT('Ctrl Pts',(-40.1225272605685,-0.14822420964857,
-9.12349227713884));
#31816=CARTESIAN_POINT('Ctrl Pts',(-42.8763256602482,-0.399777134882658,
-11.8775764776305));
#31817=CARTESIAN_POINT('Ctrl Pts',(-44.5120149889433,-0.520686157638547,
-12.9726927515284));
#31818=CARTESIAN_POINT('Ctrl Pts',(-48.1265710168888,-0.777188149416765,
-14.4683433355077));
#31819=CARTESIAN_POINT('Ctrl Pts',(-50.0549848089133,-0.897861662839052,
-14.8498038985338));
#31820=CARTESIAN_POINT('Ctrl Pts',(-51.9999570902567,-1.02423658127892,
-14.8500516281495));
#31821=CARTESIAN_POINT('Ctrl Pts',(-37.8403157026637,1.31891566289592,1.59674345384007));
#31822=CARTESIAN_POINT('Ctrl Pts',(-37.8169648654319,1.27856167200519,1.15301410976464));
#31823=CARTESIAN_POINT('Ctrl Pts',(-37.7802246921753,1.23369664255699,0.635579023166993));
#31824=CARTESIAN_POINT('Ctrl Pts',(-37.7793394043038,1.06384881091044,-1.86860431099072));
#31825=CARTESIAN_POINT('Ctrl Pts',(-38.1469172474041,0.943145133346677,
-3.70979114470212));
#31826=CARTESIAN_POINT('Ctrl Pts',(-39.5762884400003,0.687518921091354,
-7.17014261469349));
#31827=CARTESIAN_POINT('Ctrl Pts',(-40.6268483631268,0.566033915392139,
-8.73670574474909));
#31828=CARTESIAN_POINT('Ctrl Pts',(-43.2628954695621,0.314738777660199,
-11.373454410516));
#31829=CARTESIAN_POINT('Ctrl Pts',(-44.8305401132913,0.193253748298748,
-12.4221714958415));
#31830=CARTESIAN_POINT('Ctrl Pts',(-48.2896308976067,-0.0623724159560662,
-13.8545909095441));
#31831=CARTESIAN_POINT('Ctrl Pts',(-50.138965660225,-0.183762141924027,
-14.2195188100055));
#31832=CARTESIAN_POINT('Ctrl Pts',(-51.9999633043523,-0.309815399742648,
-14.2201291128083));
#31833=CARTESIAN_POINT('Ctrl Pts',(-37.7800000000001,-1.19058808997893,
0.));
#31834=CARTESIAN_POINT('Ctrl Pts',(-37.7806592587368,-1.3173273690917,-1.86858636175756));
#31835=CARTESIAN_POINT('Ctrl Pts',(-38.1455252315402,-1.43803115336822,
-3.71029995869359));
#31836=CARTESIAN_POINT('Ctrl Pts',(-39.5779229780038,-1.6936571382057,-7.16936247494164));
#31837=CARTESIAN_POINT('Ctrl Pts',(-40.6266263701707,-1.81514228728206,
-8.73699595770662));
#31838=CARTESIAN_POINT('Ctrl Pts',(-42.0790951378327,-1.95357130555297,
-10.1890856763502));
#31839=CARTESIAN_POINT('Ctrl Pts',(-42.215773213043,-1.96630970889372,-10.3203928635173));
#31840=CARTESIAN_POINT('Ctrl Pts',(-42.3549304887756,-1.97901608230199,
-10.4488603766005));
#31841=CARTESIAN_POINT('Ctrl Pts',(-37.7800000000001,1.19058808997921,9.99200722162641E-16));
#31842=CARTESIAN_POINT('Ctrl Pts',(-37.7793394043038,1.06384881091044,-1.86860431099072));
#31843=CARTESIAN_POINT('Ctrl Pts',(-38.1469172474041,0.943145133346677,
-3.70979114470212));
#31844=CARTESIAN_POINT('Ctrl Pts',(-39.5762884400003,0.687518921091354,
-7.17014261469349));
#31845=CARTESIAN_POINT('Ctrl Pts',(-40.6268483631268,0.566033915392139,
-8.73670574474909));
#31846=CARTESIAN_POINT('Ctrl Pts',(-42.0863595386742,0.426898290317344,
-10.1966053555722));
#31847=CARTESIAN_POINT('Ctrl Pts',(-42.2307237103631,0.413458201811568,
-10.3350231942284));
#31848=CARTESIAN_POINT('Ctrl Pts',(-42.3778559173172,0.400053103664163,
-10.4702558451011));
#31849=CARTESIAN_POINT('Ctrl Pts',(-44.4799848904464,-3.32327712822001,
1.24689064510956));
#31850=CARTESIAN_POINT('Ctrl Pts',(-44.4545866216563,-3.36716940899891,
0.764254540719541));
#31851=CARTESIAN_POINT('Ctrl Pts',(-44.4293496851003,-3.40814518985126,
0.332948627189092));
#31852=CARTESIAN_POINT('Ctrl Pts',(-44.4319119278341,-3.5730532724153,-0.978870002669229));
#31853=CARTESIAN_POINT('Ctrl Pts',(-44.6279251367563,-3.70160805587855,
-1.98783577088437));
#31854=CARTESIAN_POINT('Ctrl Pts',(-45.38610240764,-3.94798856177068,-3.80852727284065));
#31855=CARTESIAN_POINT('Ctrl Pts',(-45.949102167262,-4.07555420744993,-4.65544360722782));
#31856=CARTESIAN_POINT('Ctrl Pts',(-47.3456501222141,-4.32412798455906,
-6.04997283342565));
#31857=CARTESIAN_POINT('Ctrl Pts',(-48.18942650203,-4.4516935582084,-6.61832169901018));
#31858=CARTESIAN_POINT('Ctrl Pts',(-50.0137636932357,-4.69807420295161,
-7.36768403080659));
#31859=CARTESIAN_POINT('Ctrl Pts',(-51.0241709100446,-4.82686758917973,
-7.57138648682792));
#31860=CARTESIAN_POINT('Ctrl Pts',(-52.0000289040989,-4.94968218283394,
-7.56962581969448));
#31861=CARTESIAN_POINT('Ctrl Pts',(-42.4296678529921,-2.13646282181002,
1.35489302548969));
#31862=CARTESIAN_POINT('Ctrl Pts',(-42.4049009926057,-2.17926392766553,
0.884255395659172));
#31863=CARTESIAN_POINT('Ctrl Pts',(-42.3761273929606,-2.22143926476923,
0.426396892758864));
#31864=CARTESIAN_POINT('Ctrl Pts',(-42.3778082879602,-2.38787268687571,
-1.25360819498431));
#31865=CARTESIAN_POINT('Ctrl Pts',(-42.6265178497854,-2.51400314727506,
-2.51960912779415));
#31866=CARTESIAN_POINT('Ctrl Pts',(-43.592265824811,-2.76323860082922,-4.84647586782669));
#31867=CARTESIAN_POINT('Ctrl Pts',(-44.3056264360906,-2.88892662741274,
-5.91572199046927));
#31868=CARTESIAN_POINT('Ctrl Pts',(-46.0849874081721,-3.138340724919,-7.69376028691788));
#31869=CARTESIAN_POINT('Ctrl Pts',(-47.1521724801633,-3.26402870377879,
-8.41063186555663));
#31870=CARTESIAN_POINT('Ctrl Pts',(-49.481430310228,-3.51326424840763,-9.37059840620967));
#31871=CARTESIAN_POINT('Ctrl Pts',(-50.750806496017,-3.63979023544967,-9.62435378626137));
#31872=CARTESIAN_POINT('Ctrl Pts',(-52.0000086477592,-3.76358612954908,
-9.62320046360553));
#31873=CARTESIAN_POINT('Ctrl Pts',(-40.1875259567355,-1.37301063256228,
1.47293173916724));
#31874=CARTESIAN_POINT('Ctrl Pts',(-40.1634477706347,-1.4146215988494,1.01538079143144));
#31875=CARTESIAN_POINT('Ctrl Pts',(-40.1308402311895,-1.45810560976085,
0.528580648123612));
#31876=CARTESIAN_POINT('Ctrl Pts',(-40.1319542826431,-1.62620698164256,
-1.55402875454962));
#31877=CARTESIAN_POINT('Ctrl Pts',(-40.4376784663554,-1.74968648306518,
-3.10121432123338));
#31878=CARTESIAN_POINT('Ctrl Pts',(-41.6310829191806,-2.00204375396032,
-5.98129145451077));
#31879=CARTESIAN_POINT('Ctrl Pts',(-42.5084456369507,-2.12567864734773,
-7.29389406576292));
#31880=CARTESIAN_POINT('Ctrl Pts',(-44.706560886716,-2.37601161837734,-9.49113593804378));
#31881=CARTESIAN_POINT('Ctrl Pts',(-46.0177955705402,-2.49964647926416,
-10.3708286017169));
#31882=CARTESIAN_POINT('Ctrl Pts',(-48.8994560970704,-2.75200381048057,
-11.5604045561253));
#31883=CARTESIAN_POINT('Ctrl Pts',(-50.4518266808772,-2.87602039417437,
-11.8694761541285));
#31884=CARTESIAN_POINT('Ctrl Pts',(-51.9999864978575,-3.00091936260182,
-11.8687142284813));
#31885=CARTESIAN_POINT('Ctrl Pts',(-37.8397258902528,-1.06226042836983,
1.59647049649061));
#31886=CARTESIAN_POINT('Ctrl Pts',(-37.8163671782138,-1.10262802813137,
1.15259151033015));
#31887=CARTESIAN_POINT('Ctrl Pts',(-37.7797757625724,-1.14747953738618,
0.635572917992124));
#31888=CARTESIAN_POINT('Ctrl Pts',(-37.7806592587368,-1.3173273690917,-1.86858636175756));
#31889=CARTESIAN_POINT('Ctrl Pts',(-38.1455252315402,-1.43803115336822,
-3.71029995869359));
#31890=CARTESIAN_POINT('Ctrl Pts',(-39.5779229780038,-1.6936571382057,-7.16936247494164));
#31891=CARTESIAN_POINT('Ctrl Pts',(-40.6266263701707,-1.81514228728206,
-8.73699595770662));
#31892=CARTESIAN_POINT('Ctrl Pts',(-43.2633442117449,-2.06643737216986,
-11.3730256982132));
#31893=CARTESIAN_POINT('Ctrl Pts',(-44.829890472526,-2.18792249430096,-12.423580519232));
#31894=CARTESIAN_POINT('Ctrl Pts',(-48.290206627889,-2.44354852691069,-13.8529470821504));
#31895=CARTESIAN_POINT('Ctrl Pts',(-50.1387215498246,-2.56492073909667,
-14.2204718556739));
#31896=CARTESIAN_POINT('Ctrl Pts',(-51.9999633056261,-2.69099156569442,
-14.2198708430667));
#31897=CARTESIAN_POINT('Ctrl Pts',(-37.8403157026637,1.31891566289592,1.59674345384007));
#31898=CARTESIAN_POINT('Ctrl Pts',(-37.8169648654319,1.2785616720052,1.15301410976464));
#31899=CARTESIAN_POINT('Ctrl Pts',(-37.7802246921753,1.23369664255699,0.635579023166993));
#31900=CARTESIAN_POINT('Ctrl Pts',(-37.7793394043038,1.06384881091045,-1.86860431099072));
#31901=CARTESIAN_POINT('Ctrl Pts',(-38.1469172474041,0.943145133346679,
-3.70979114470212));
#31902=CARTESIAN_POINT('Ctrl Pts',(-39.5762884400003,0.687518921091357,
-7.17014261469349));
#31903=CARTESIAN_POINT('Ctrl Pts',(-40.6268483631268,0.566033915392151,
-8.73670574474909));
#31904=CARTESIAN_POINT('Ctrl Pts',(-43.2628954695621,0.314738777660206,
-11.373454410516));
#31905=CARTESIAN_POINT('Ctrl Pts',(-44.8305401132913,0.193253748298752,
-12.4221714958415));
#31906=CARTESIAN_POINT('Ctrl Pts',(-48.2896308976067,-0.0623724159560593,
-13.8545909095441));
#31907=CARTESIAN_POINT('Ctrl Pts',(-50.138965660225,-0.183762141924011,
-14.2195188100055));
#31908=CARTESIAN_POINT('Ctrl Pts',(-51.9999633043523,-0.309815399742647,
-14.2201291128083));
#31909=CARTESIAN_POINT('Ctrl Pts',(-40.1882694324258,1.62853105321851,1.47327580984132));
#31910=CARTESIAN_POINT('Ctrl Pts',(-40.1642011727661,1.58693724130854,1.01591349030302));
#31911=CARTESIAN_POINT('Ctrl Pts',(-40.131406120005,1.54343618780035,0.528588343874024));
#31912=CARTESIAN_POINT('Ctrl Pts',(-40.1302905677598,1.37533481599316,-1.55405138007982));
#31913=CARTESIAN_POINT('Ctrl Pts',(-40.4394331428155,1.25185544908462,-3.10057294640439));
#31914=CARTESIAN_POINT('Ctrl Pts',(-41.6290225365131,0.999497891523314,
-5.98227484334839));
#31915=CARTESIAN_POINT('Ctrl Pts',(-42.5087254655197,0.875863178866758,
-7.29352824389351));
#31916=CARTESIAN_POINT('Ctrl Pts',(-44.7059952341549,0.625530141225346,
-9.49167634236414));
#31917=CARTESIAN_POINT('Ctrl Pts',(-46.018614461608,0.501895397276723,-10.369052486768));
#31918=CARTESIAN_POINT('Ctrl Pts',(-48.898730372315,0.249537900119352,-11.5624766483463));
#31919=CARTESIAN_POINT('Ctrl Pts',(-50.4521347865908,0.125494944839277,
-11.8682745705877));
#31920=CARTESIAN_POINT('Ctrl Pts',(-51.9999864962518,0.000622417322863719,
-11.8690397849987));
#31921=CARTESIAN_POINT('Ctrl Pts',(-42.4307892712954,2.39089944281244,1.35541200298501));
#31922=CARTESIAN_POINT('Ctrl Pts',(-42.4060373834038,2.34812421168677,0.885058889671389));
#31923=CARTESIAN_POINT('Ctrl Pts',(-42.3769809488765,2.30592316845675,0.426408500610301));
#31924=CARTESIAN_POINT('Ctrl Pts',(-42.3752988309043,2.13948974646265,-1.25364232210375));
#31925=CARTESIAN_POINT('Ctrl Pts',(-42.6291645083404,2.01335948895693,-2.51864171287944));
#31926=CARTESIAN_POINT('Ctrl Pts',(-43.5891580556361,1.76412360301131,-4.8479591580744));
#31927=CARTESIAN_POINT('Ctrl Pts',(-44.3060485143004,1.63843584903247,-5.91517020465661));
#31928=CARTESIAN_POINT('Ctrl Pts',(-46.084134208595,1.38902165105224,-7.69457540340634));
#31929=CARTESIAN_POINT('Ctrl Pts',(-47.1534076509246,1.26333384857631,-8.40795287034413));
#31930=CARTESIAN_POINT('Ctrl Pts',(-49.4803356664663,1.01409805365021,-9.37372383744511));
#31931=CARTESIAN_POINT('Ctrl Pts',(-50.7512717901674,0.8875230677712,-9.62254086005841));
#31932=CARTESIAN_POINT('Ctrl Pts',(-52.0000086453373,0.76377627707492,-9.62369151535371));
#31933=CARTESIAN_POINT('Ctrl Pts',(-44.4816940061639,3.57672261477362,1.24768160116191));
#31934=CARTESIAN_POINT('Ctrl Pts',(-44.4563185564429,3.53286976879546,0.765479118775378));
#31935=CARTESIAN_POINT('Ctrl Pts',(-44.4306505608096,3.49185481010524,0.332966318322973));
#31936=CARTESIAN_POINT('Ctrl Pts',(-44.4280873491905,3.32694672771256,-0.978922014658035));
#31937=CARTESIAN_POINT('Ctrl Pts',(-44.631958819594,3.19839225347229,-1.98636136652375));
#31938=CARTESIAN_POINT('Ctrl Pts',(-45.381365961698,2.95201108858753,-3.81078790535288));
#31939=CARTESIAN_POINT('Ctrl Pts',(-45.9497454423884,2.82444585837497,-4.65460264912874));
#31940=CARTESIAN_POINT('Ctrl Pts',(-47.3443497895892,2.57587192813805,-6.05121512490362));
#31941=CARTESIAN_POINT('Ctrl Pts',(-48.1913089840218,2.44830662330916,-6.61423873299694));
#31942=CARTESIAN_POINT('Ctrl Pts',(-50.0120953836924,2.20192559709565,-7.37244739486697));
#31943=CARTESIAN_POINT('Ctrl Pts',(-51.0248803821906,2.07303718494182,-7.56862230179044));
#31944=CARTESIAN_POINT('Ctrl Pts',(-52.0000289004077,1.95031777657942,-7.57037421505984));
#31945=CARTESIAN_POINT('Ctrl Pts',(-37.6057474666452,4.33370633274489,1.59647061166167));
#31946=CARTESIAN_POINT('Ctrl Pts',(-37.6014604087211,4.32302794314895,1.48695576756414));
#31947=CARTESIAN_POINT('Ctrl Pts',(-37.5971743516736,4.31235100760161,1.37746396775989));
#31948=CARTESIAN_POINT('Ctrl Pts',(-37.5789019782659,4.26684181644195,0.910698635112159));
#31949=CARTESIAN_POINT('Ctrl Pts',(-37.5600270135807,4.23081870485879,0.486448413019324));
#31950=CARTESIAN_POINT('Ctrl Pts',(-37.5835818541665,4.07282953635717,-1.8685863617356));
#31951=CARTESIAN_POINT('Ctrl Pts',(-37.9619119570033,4.00528018449519,-3.71029995871943));
#31952=CARTESIAN_POINT('Ctrl Pts',(-39.4161093304632,3.95610755720103,-7.1693624749157));
#31953=CARTESIAN_POINT('Ctrl Pts',(-40.4714275735225,3.98510500543641,-8.73699595769429));
#31954=CARTESIAN_POINT('Ctrl Pts',(-43.1170704486978,4.1116118153854,-11.3730256982255));
#31955=CARTESIAN_POINT('Ctrl Pts',(-44.6849606628027,4.21430601437161,-12.4235805192234));
#31956=CARTESIAN_POINT('Ctrl Pts',(-48.1464351665736,4.45373622022133,-13.852947082159));
#31957=CARTESIAN_POINT('Ctrl Pts',(-49.993407938683,4.59667050421463,-14.2204718556549));
#31958=CARTESIAN_POINT('Ctrl Pts',(-51.8536466863969,4.73676521641199,-14.2198708430668));
#31959=CARTESIAN_POINT('Ctrl Pts',(-36.8815114147052,4.95142919224145,1.6296460532693));
#31960=CARTESIAN_POINT('Ctrl Pts',(-36.8772243107663,4.94075068802638,1.52013003366919));
#31961=CARTESIAN_POINT('Ctrl Pts',(-36.8729383891555,4.93007388724636,1.41064098632203));
#31962=CARTESIAN_POINT('Ctrl Pts',(-36.8546656346297,4.88456461021452,0.943868932650714));
#31963=CARTESIAN_POINT('Ctrl Pts',(-36.8348655943225,4.84834678143282,0.508392298446954));
#31964=CARTESIAN_POINT('Ctrl Pts',(-36.8579890764718,4.68985095932364,-1.95287905122974));
#31965=CARTESIAN_POINT('Ctrl Pts',(-37.2526110659712,4.62539547710255,-3.87337387080524));
#31966=CARTESIAN_POINT('Ctrl Pts',(-38.7695270468993,4.58435548148662,-7.48792130212039));
#31967=CARTESIAN_POINT('Ctrl Pts',(-39.8706950784938,4.62052713520107,-9.12360836230517));
#31968=CARTESIAN_POINT('Ctrl Pts',(-42.6325290552102,4.76347923308833,-11.877404992726));
#31969=CARTESIAN_POINT('Ctrl Pts',(-44.2683416970911,4.87652118890886,-12.973256360878));
#31970=CARTESIAN_POINT('Ctrl Pts',(-47.8830959478462,5.13710478162807,-14.4676858045569));
#31971=CARTESIAN_POINT('Ctrl Pts',(-49.8087293766818,5.29206142837056,-14.8501851005009));
#31972=CARTESIAN_POINT('Ctrl Pts',(-51.7519872491301,5.44377846349967,-14.8499483202528));
#31973=CARTESIAN_POINT('Ctrl Pts',(-36.7461942621622,5.89423842867625,1.62975523620908));
#31974=CARTESIAN_POINT('Ctrl Pts',(-36.7419071579067,5.88355992367606,1.52023920855918));
#31975=CARTESIAN_POINT('Ctrl Pts',(-36.7376212482649,5.87288312535246,1.41075017947915));
#31976=CARTESIAN_POINT('Ctrl Pts',(-36.719348444076,5.82737384119746,0.943978082261264));
#31977=CARTESIAN_POINT('Ctrl Pts',(-36.6994509531039,5.79114203694912,0.508394167533837));
#31978=CARTESIAN_POINT('Ctrl Pts',(-36.7219158272034,5.63255152132131,-1.95288623092271));
#31979=CARTESIAN_POINT('Ctrl Pts',(-37.1176115175746,5.56825045710434,-3.87317034520815));
#31980=CARTESIAN_POINT('Ctrl Pts',(-38.6333292122811,5.52703808203503,-7.48823335802159));
#31981=CARTESIAN_POINT('Ctrl Pts',(-39.7352322893736,5.5633154772789,-9.12349227711925));
#31982=CARTESIAN_POINT('Ctrl Pts',(-42.496800705893,5.70622937201901,-11.87757647765));
#31983=CARTESIAN_POINT('Ctrl Pts',(-44.1330482236871,5.81933389104568,-12.9726927515247));
#31984=CARTESIAN_POINT('Ctrl Pts',(-47.7473173225239,6.07984767625072,-14.4683433355114));
#31985=CARTESIAN_POINT('Ctrl Pts',(-49.6732762742263,6.23484434202318,-14.8498038985576));
#31986=CARTESIAN_POINT('Ctrl Pts',(-51.6164365682427,6.38655415380911,-14.8500516281495));
#31987=CARTESIAN_POINT('Ctrl Pts',(-37.2674545852877,6.69072942383186,1.59674356901112));
#31988=CARTESIAN_POINT('Ctrl Pts',(-37.263167526575,6.680051032273,1.48722870478903));
#31989=CARTESIAN_POINT('Ctrl Pts',(-37.2588814994477,6.66937410286672,1.37773695065262));
#31990=CARTESIAN_POINT('Ctrl Pts',(-37.2406090018804,6.6238648938997,0.910971509138724));
#31991=CARTESIAN_POINT('Ctrl Pts',(-37.2214904105359,6.58780684365017,0.48645308573652));
#31992=CARTESIAN_POINT('Ctrl Pts',(-37.2433987309883,6.42958094134897,-1.86860431096801));
#31993=CARTESIAN_POINT('Ctrl Pts',(-37.624413086019,6.36241763449877,-3.70979114472192));
#31994=CARTESIAN_POINT('Ctrl Pts',(-39.0756147439105,6.31281405857297,-7.1701426146735));
#31995=CARTESIAN_POINT('Ctrl Pts',(-40.1327706007244,6.3420758606307,-8.73670574473669));
#31996=CARTESIAN_POINT('Ctrl Pts',(-42.7777495754025,6.46848716271241,-11.3734544105282));
#31997=CARTESIAN_POINT('Ctrl Pts',(-44.3467269792927,6.57133776971453,-12.4221714958329));
#31998=CARTESIAN_POINT('Ctrl Pts',(-47.806988603268,6.81059345677706,-13.8545909095527));
#31999=CARTESIAN_POINT('Ctrl Pts',(-49.6547753637294,6.95362708074825,-14.2195188100197));
#32000=CARTESIAN_POINT('Ctrl Pts',(-51.5147699841784,7.09370444218559,-14.2201291128083));
#32001=CARTESIAN_POINT('Ctrl Pts',(-37.5648924257371,4.19818497005551,0.));
#32002=CARTESIAN_POINT('Ctrl Pts',(-37.5835818541665,4.07282953635717,-1.8685863617356));
#32003=CARTESIAN_POINT('Ctrl Pts',(-37.9619119570033,4.00528018449519,-3.71029995871943));
#32004=CARTESIAN_POINT('Ctrl Pts',(-39.4161093304632,3.95610755720103,-7.1693624749157));
#32005=CARTESIAN_POINT('Ctrl Pts',(-40.4714275735225,3.98510500543642,-8.73699595769429));
#32006=CARTESIAN_POINT('Ctrl Pts',(-41.92881280678,4.05479285274799,-10.1890856763504));
#32007=CARTESIAN_POINT('Ctrl Pts',(-42.0659125600695,4.06163542615554,-10.3203928635174));
#32008=CARTESIAN_POINT('Ctrl Pts',(-42.2054617208597,4.06886253049829,-10.4488603766002));
#32009=CARTESIAN_POINT('Ctrl Pts',(-37.2260157226955,6.55512420933882,-4.87766496047995E-9));
#32010=CARTESIAN_POINT('Ctrl Pts',(-37.243398731537,6.42958094105718,-1.86860431419405));
#32011=CARTESIAN_POINT('Ctrl Pts',(-37.6244130865614,6.36241763433584,-3.70979114625967));
#32012=CARTESIAN_POINT('Ctrl Pts',(-38.3500139148987,6.3376158464277,-5.43996687972819));
#32013=CARTESIAN_POINT('Ctrl Pts',(-39.0756147438695,6.31281405849791,-7.17014261470714));
#32014=CARTESIAN_POINT('Ctrl Pts',(-40.1327706007051,6.34207586058859,-8.7367057447602));
#32015=CARTESIAN_POINT('Ctrl Pts',(-41.4552600880589,6.40528151166132,-10.0550800776384));
#32016=CARTESIAN_POINT('Ctrl Pts',(-41.5972271209419,6.41206653251029,-10.1966053555764));
#32017=CARTESIAN_POINT('Ctrl Pts',(-41.7420345975428,6.41930840847686,-10.3350231942305));
#32018=CARTESIAN_POINT('Ctrl Pts',(-41.8895769551533,6.42697885114131,-10.4702558451008));
#32019=CARTESIAN_POINT('Ctrl Pts',(-44.5001944306519,3.04071090848703,1.24689076028072));
#32020=CARTESIAN_POINT('Ctrl Pts',(-44.4959078567086,3.03003372440579,1.13738827963299));
#32021=CARTESIAN_POINT('Ctrl Pts',(-44.4916204363957,3.01935537993451,1.02786752739767));
#32022=CARTESIAN_POINT('Ctrl Pts',(-44.4733518105235,2.9738470557106,0.561172897445051));
#32023=CARTESIAN_POINT('Ctrl Pts',(-44.463701217077,2.93980180526124,0.254828874448762));
#32024=CARTESIAN_POINT('Ctrl Pts',(-44.488157628525,2.78663561816024,-0.97887000271182));
#32025=CARTESIAN_POINT('Ctrl Pts',(-44.7004709588269,2.68728492514594,-1.98783577088727));
#32026=CARTESIAN_POINT('Ctrl Pts',(-45.485994680174,2.55131209327259,-3.80852727283799));
#32027=CARTESIAN_POINT('Ctrl Pts',(-46.0614183982389,2.50516810166005,-4.65544360721341));
#32028=CARTESIAN_POINT('Ctrl Pts',(-47.4791272455575,2.45787394352684,-6.04997283344033));
#32029=CARTESIAN_POINT('Ctrl Pts',(-48.3324696724478,2.45168870251976,-6.61832169900605));
#32030=CARTESIAN_POINT('Ctrl Pts',(-50.1733013631053,2.46744610981289,-7.36768403081099));
#32031=CARTESIAN_POINT('Ctrl Pts',(-51.1917533012898,2.48375959427692,-7.57138648673751));
#32032=CARTESIAN_POINT('Ctrl Pts',(-52.1751568070597,2.50107414862785,-7.56962581969461));
#32033=CARTESIAN_POINT('Ctrl Pts',(-42.3018453782487,3.92365461890858,1.35489314066083));
#32034=CARTESIAN_POINT('Ctrl Pts',(-42.2975586546965,3.91297706217519,1.24538683818762));
#32035=CARTESIAN_POINT('Ctrl Pts',(-42.2932716614844,3.90229915402396,1.13587503551223));
#32036=CARTESIAN_POINT('Ctrl Pts',(-42.275001852934,3.85679055844576,0.669158551014111));
#32037=CARTESIAN_POINT('Ctrl Pts',(-42.2624528820652,3.82212739678175,0.326351368872599));
#32038=CARTESIAN_POINT('Ctrl Pts',(-42.2862930185762,3.66742334692284,-1.25360819500681));
#32039=CARTESIAN_POINT('Ctrl Pts',(-42.5504213117424,3.57797177380988,-2.51960912780189));
#32040=CARTESIAN_POINT('Ctrl Pts',(-43.5418092681773,3.46871344469679,-4.84647586781908));
#32041=CARTESIAN_POINT('Ctrl Pts',(-44.2657961681649,3.44582654101586,-5.91572199045955));
#32042=CARTESIAN_POINT('Ctrl Pts',(-46.0625411381428,3.45218058836645,-7.69376028692778));
#32043=CARTESIAN_POINT('Ctrl Pts',(-47.1367510692374,3.47964820283165,-8.4106318655574));
#32044=CARTESIAN_POINT('Ctrl Pts',(-49.4777703293181,3.56443746806506,-9.37059840620908));
#32045=CARTESIAN_POINT('Ctrl Pts',(-50.7522326212179,3.61985039974676,-9.62435378620432));
#32046=CARTESIAN_POINT('Ctrl Pts',(-52.0063376889004,3.67509457152191,-9.62320046360563));
#32047=CARTESIAN_POINT('Ctrl Pts',(-39.9738746787523,4.36024590432563,1.47293185433834));
#32048=CARTESIAN_POINT('Ctrl Pts',(-39.969587791779,4.34956794053916,1.36342137723756));
#32049=CARTESIAN_POINT('Ctrl Pts',(-39.9653012588855,4.33889050812397,1.25391935060529));
#32050=CARTESIAN_POINT('Ctrl Pts',(-39.9470301849496,4.29338161981705,0.787178992719804));
#32051=CARTESIAN_POINT('Ctrl Pts',(-39.9313665239408,4.25805061593316,0.404559744691303));
#32052=CARTESIAN_POINT('Ctrl Pts',(-39.9549022371146,4.10171804395403,-1.55402875455033));
#32053=CARTESIAN_POINT('Ctrl Pts',(-40.2750875547445,4.02300447358394,-3.10121432124956));
#32054=CARTESIAN_POINT('Ctrl Pts',(-41.4922590551962,3.94305499752666,-5.98129145449459));
#32055=CARTESIAN_POINT('Ctrl Pts',(-42.3782865653892,3.94554026237538,-7.29389406575069));
#32056=CARTESIAN_POINT('Ctrl Pts',(-44.5896542676445,4.01057973632249,-9.49113593805607));
#32057=CARTESIAN_POINT('Ctrl Pts',(-45.9051375482497,4.0748114520141,-10.3708286017082));
#32058=CARTESIAN_POINT('Ctrl Pts',(-48.7933811184128,4.23512580635715,-11.5604045561341));
#32059=CARTESIAN_POINT('Ctrl Pts',(-50.3476002080614,4.33329690120631,-11.8694761541143));
#32060=CARTESIAN_POINT('Ctrl Pts',(-51.8977769668582,4.42999533819672,-11.8687142284813));
#32061=CARTESIAN_POINT('Ctrl Pts',(-37.6057474666452,4.33370633274489,1.59647061166167));
#32062=CARTESIAN_POINT('Ctrl Pts',(-37.6014604087211,4.32302794314895,1.48695576756414));
#32063=CARTESIAN_POINT('Ctrl Pts',(-37.5971743516736,4.31235100760161,1.37746396775989));
#32064=CARTESIAN_POINT('Ctrl Pts',(-37.5789019782659,4.26684181644196,0.910698635112159));
#32065=CARTESIAN_POINT('Ctrl Pts',(-37.5600270135807,4.23081870485879,0.486448413019324));
#32066=CARTESIAN_POINT('Ctrl Pts',(-37.5835818541665,4.07282953635717,-1.8685863617356));
#32067=CARTESIAN_POINT('Ctrl Pts',(-37.9619119570033,4.00528018449519,-3.71029995871943));
#32068=CARTESIAN_POINT('Ctrl Pts',(-39.4161093304632,3.95610755720103,-7.1693624749157));
#32069=CARTESIAN_POINT('Ctrl Pts',(-40.4714275735225,3.98510500543642,-8.73699595769429));
#32070=CARTESIAN_POINT('Ctrl Pts',(-43.1170704486978,4.1116118153854,-11.3730256982255));
#32071=CARTESIAN_POINT('Ctrl Pts',(-44.6849606628027,4.21430601437221,-12.4235805192234));
#32072=CARTESIAN_POINT('Ctrl Pts',(-48.1464351665736,4.45373622022074,-13.852947082159));
#32073=CARTESIAN_POINT('Ctrl Pts',(-49.9934079386831,4.59667050421464,-14.2204718556549));
#32074=CARTESIAN_POINT('Ctrl Pts',(-51.8536466863969,4.73676521641199,-14.2198708430668));
#32075=CARTESIAN_POINT('Ctrl Pts',(-37.2674545852877,6.69072942383186,1.59674356901112));
#32076=CARTESIAN_POINT('Ctrl Pts',(-37.263167526575,6.68005103227299,1.48722870478903));
#32077=CARTESIAN_POINT('Ctrl Pts',(-37.2588814994477,6.66937410286672,1.37773695065262));
#32078=CARTESIAN_POINT('Ctrl Pts',(-37.2406090018803,6.62386489389971,0.910971509138724));
#32079=CARTESIAN_POINT('Ctrl Pts',(-37.2214904105359,6.58780684365017,0.48645308573652));
#32080=CARTESIAN_POINT('Ctrl Pts',(-37.2433987309883,6.42958094134897,-1.86860431096802));
#32081=CARTESIAN_POINT('Ctrl Pts',(-37.6244130860238,6.36241763449877,-3.70979114472193));
#32082=CARTESIAN_POINT('Ctrl Pts',(-39.0756147439057,6.31281405857297,-7.1701426146735));
#32083=CARTESIAN_POINT('Ctrl Pts',(-40.1327706007196,6.3420758606307,-8.7367057447367));
#32084=CARTESIAN_POINT('Ctrl Pts',(-42.7777495754072,6.4684871627124,-11.3734544105282));
#32085=CARTESIAN_POINT('Ctrl Pts',(-44.3467269792975,6.57133776971454,-12.4221714958329));
#32086=CARTESIAN_POINT('Ctrl Pts',(-47.8069886032632,6.81059345677706,-13.8545909095527));
#32087=CARTESIAN_POINT('Ctrl Pts',(-49.6547753637331,6.95362708074793,-14.2195188100197));
#32088=CARTESIAN_POINT('Ctrl Pts',(-51.5147699841784,7.09370444218559,-14.2201291128083));
#32089=CARTESIAN_POINT('Ctrl Pts',(-39.5474466673498,7.33134203123354,1.47327592501242));
#32090=CARTESIAN_POINT('Ctrl Pts',(-39.5431597793819,7.3206640649734,1.36376542254399));
#32091=CARTESIAN_POINT('Ctrl Pts',(-39.5388732842043,7.30998664029854,1.25426345347746));
#32092=CARTESIAN_POINT('Ctrl Pts',(-39.5206020537614,7.26447772954494,0.787522958362851));
#32093=CARTESIAN_POINT('Ctrl Pts',(-39.5046312942642,7.22910268445617,0.404565634787169));
#32094=CARTESIAN_POINT('Ctrl Pts',(-39.5260915209543,7.07247170264163,-1.55405138007959));
#32095=CARTESIAN_POINT('Ctrl Pts',(-39.849660416496,6.99424475323091,-3.10057294641452));
#32096=CARTESIAN_POINT('Ctrl Pts',(-41.0630557303939,6.91375205389509,-5.98227484333816));
#32097=CARTESIAN_POINT('Ctrl Pts',(-41.9513996061357,6.91657054442171,-7.29352824388359));
#32098=CARTESIAN_POINT('Ctrl Pts',(-44.1619304425256,6.98148962792627,-9.49167634237396));
#32099=CARTESIAN_POINT('Ctrl Pts',(-45.4787841574542,7.04591850046845,-10.369052486764));
#32100=CARTESIAN_POINT('Ctrl Pts',(-48.3654988573771,7.20601286880697,-11.5624766483502));
#32101=CARTESIAN_POINT('Ctrl Pts',(-49.9207450076547,7.30430498991027,-11.8682745706258));
#32102=CARTESIAN_POINT('Ctrl Pts',(-51.4706130322883,7.40098575043911,-11.8690397849986));
#32103=CARTESIAN_POINT('Ctrl Pts',(-41.6586445536368,8.40509445805904,1.35541211815616));
#32104=CARTESIAN_POINT('Ctrl Pts',(-41.6543578285816,8.39441689759386,1.24590577741992));
#32105=CARTESIAN_POINT('Ctrl Pts',(-41.6500708922605,8.38373900111844,1.13639406157341));
#32106=CARTESIAN_POINT('Ctrl Pts',(-41.6318008476447,8.33823037168265,0.669677370086285));
#32107=CARTESIAN_POINT('Ctrl Pts',(-41.6187886661146,8.30350078066026,0.326360253172907));
#32108=CARTESIAN_POINT('Ctrl Pts',(-41.6394982516697,8.14834662563191,-1.25364232212485));
#32109=CARTESIAN_POINT('Ctrl Pts',(-41.9087301497829,8.05962904511491,-2.5186417128775));
#32110=CARTESIAN_POINT('Ctrl Pts',(-42.8944223117343,7.94955134754417,-4.84795915807629));
#32111=CARTESIAN_POINT('Ctrl Pts',(-43.6219030915765,7.927167063359,-5.91517020464915));
#32112=CARTESIAN_POINT('Ctrl Pts',(-45.4173857785771,7.9333395203096,-7.69457540341371));
#32113=CARTESIAN_POINT('Ctrl Pts',(-46.4936627982941,7.96110451544745,-8.40795287034476));
#32114=CARTESIAN_POINT('Ctrl Pts',(-48.832375993634,8.04556196575667,-9.37372383744437));
#32115=CARTESIAN_POINT('Ctrl Pts',(-50.1083893187814,8.10114839964074,-9.62254086011549));
#32116=CARTESIAN_POINT('Ctrl Pts',(-51.3620268377999,8.15637495641934,-9.62369151535365));
#32117=CARTESIAN_POINT('Ctrl Pts',(-43.5199138025264,9.87072183560205,1.24768171633308));
#32118=CARTESIAN_POINT('Ctrl Pts',(-43.5156272262978,9.86004464583405,1.1381791773697));
#32119=CARTESIAN_POINT('Ctrl Pts',(-43.5113398926855,9.84936631915668,1.02865855746757));
#32120=CARTESIAN_POINT('Ctrl Pts',(-43.4930709070328,9.80385794333174,0.561963612050125));
#32121=CARTESIAN_POINT('Ctrl Pts',(-43.4827143498822,9.76971145014305,0.254842414710469));
#32122=CARTESIAN_POINT('Ctrl Pts',(-43.5023995944666,9.6158592729741,-0.978922014698472));
#32123=CARTESIAN_POINT('Ctrl Pts',(-43.7224911564956,9.51762723325487,-1.98636136651214));
#32124=CARTESIAN_POINT('Ctrl Pts',(-44.4993341100792,9.3804056296222,-3.81078790536449));
#32125=CARTESIAN_POINT('Ctrl Pts',(-45.0800827322848,9.33502766338411,-4.65460264911893));
#32126=CARTESIAN_POINT('Ctrl Pts',(-46.4958677767967,9.28745674946867,-6.05121512491333));
#32127=CARTESIAN_POINT('Ctrl Pts',(-47.3523605835637,9.2817247362875,-6.61423873300218));
#32128=CARTESIAN_POINT('Ctrl Pts',(-49.1896776789234,9.29697643567186,-7.37244739486155));
#32129=CARTESIAN_POINT('Ctrl Pts',(-50.2104967199979,9.31353425505037,-7.56862230187132));
#32130=CARTESIAN_POINT('Ctrl Pts',(-51.1931844250964,9.33084205690745,-7.57037421505974));
#32131=CARTESIAN_POINT('Ctrl Pts',(-36.6062244663075,9.64145132693343,1.5964706812662));
#32132=CARTESIAN_POINT('Ctrl Pts',(-36.5951848118755,9.59613798296134,1.15259163661763));
#32133=CARTESIAN_POINT('Ctrl Pts',(-36.57271173128,9.54279427445571,0.635573001827313));
#32134=CARTESIAN_POINT('Ctrl Pts',(-36.6214111051725,9.38007537749595,-1.86858636170199));
#32135=CARTESIAN_POINT('Ctrl Pts',(-37.0055036281526,9.36705556804786,-3.71029995870504));
#32136=CARTESIAN_POINT('Ctrl Pts',(-38.451897363611,9.52533731124315,-7.1693624749302));
#32137=CARTESIAN_POINT('Ctrl Pts',(-39.4923472214662,9.70422705234564,-8.73699595770811));
#32138=CARTESIAN_POINT('Ctrl Pts',(-42.09305747065,10.2059604432804,-11.3730256982116));
#32139=CARTESIAN_POINT('Ctrl Pts',(-43.6303739147953,10.5307434056437,-12.423580519237));
#32140=CARTESIAN_POINT('Ctrl Pts',(-47.0225411280958,11.2603557414264,-13.8529470821453));
#32141=CARTESIAN_POINT('Ctrl Pts',(-48.8303727110256,11.6646867918221,-14.2204718556263));
#32142=CARTESIAN_POINT('Ctrl Pts',(-50.6517393542018,12.0680951184147,-14.2198708430666));
#32143=CARTESIAN_POINT('Ctrl Pts',(-35.8014489642672,10.1498171217997,1.62964612287382));
#32144=CARTESIAN_POINT('Ctrl Pts',(-35.7905014108219,10.1048818153751,1.18947024667539));
#32145=CARTESIAN_POINT('Ctrl Pts',(-35.7670704718544,10.0508712183131,0.664243958002629));
#32146=CARTESIAN_POINT('Ctrl Pts',(-35.8153925117153,9.88755379323324,-1.95287905118396));
#32147=CARTESIAN_POINT('Ctrl Pts',(-36.2151707898863,9.87991493951249,-3.87337387079329));
#32148=CARTESIAN_POINT('Ctrl Pts',(-37.7224873536581,10.0551723244044,-7.48792130213255));
#32149=CARTESIAN_POINT('Ctrl Pts',(-38.8072993194189,10.2476883531559,-9.12360836232142));
#32150=CARTESIAN_POINT('Ctrl Pts',(-41.5206776037716,10.7822353605362,-11.8774049927098));
#32151=CARTESIAN_POINT('Ctrl Pts',(-43.1237524839735,11.1269271238125,-12.9732563608916));
#32152=CARTESIAN_POINT('Ctrl Pts',(-46.6646288366134,11.89929151789,-14.4676858045432));
#32153=CARTESIAN_POINT('Ctrl Pts',(-48.548609463595,12.3267171393501,-14.8501851004771));
#32154=CARTESIAN_POINT('Ctrl Pts',(-50.4504961875093,12.7534443437023,-14.8499483202528));
#32155=CARTESIAN_POINT('Ctrl Pts',(-35.5333334012201,11.0637722809465,1.62975530581362));
#32156=CARTESIAN_POINT('Ctrl Pts',(-35.5223873364771,11.0188430850026,1.18963928646867));
#32157=CARTESIAN_POINT('Ctrl Pts',(-35.4989008284127,10.9648105349916,0.664246400071012));
#32158=CARTESIAN_POINT('Ctrl Pts',(-35.5465440138952,10.8012937803065,-1.95288623087167));
#32159=CARTESIAN_POINT('Ctrl Pts',(-35.9473630882428,10.7939605764042,-3.87317034519864));
#32160=CARTESIAN_POINT('Ctrl Pts',(-37.4535180947772,10.9688768025096,-7.48823335803139));
#32161=CARTESIAN_POINT('Ctrl Pts',(-38.5390425757456,11.1616021043726,-9.12349227713797));
#32162=CARTESIAN_POINT('Ctrl Pts',(-41.2521634397885,11.6960735043055,-11.8775764776314));
#32163=CARTESIAN_POINT('Ctrl Pts',(-42.8556598658218,12.040889083279,-12.9726927515335));
#32164=CARTESIAN_POINT('Ctrl Pts',(-46.3960659393421,12.813115336064,-14.4683433355027));
#32165=CARTESIAN_POINT('Ctrl Pts',(-48.2803630805299,13.2406268959519,-14.8498038985528));
#32166=CARTESIAN_POINT('Ctrl Pts',(-50.182154247211,13.6673330636264,-14.8500516281495));
#32167=CARTESIAN_POINT('Ctrl Pts',(-35.9359355586898,11.9263392248004,1.59674363861568));
#32168=CARTESIAN_POINT('Ctrl Pts',(-35.924899625982,11.8810411570281,1.15301423610205));
#32169=CARTESIAN_POINT('Ctrl Pts',(-35.9022876226749,11.8276425661526,0.635579106998265));
#32170=CARTESIAN_POINT('Ctrl Pts',(-35.9492898606247,11.6644253451772,-1.86860431092127));
#32171=CARTESIAN_POINT('Ctrl Pts',(-36.3359843740511,11.6521696602785,-3.70979114471603));
#32172=CARTESIAN_POINT('Ctrl Pts',(-37.7794742164016,11.809598506505,-7.17014261467971));
#32173=CARTESIAN_POINT('Ctrl Pts',(-38.8217053622759,11.9890114303897,-8.73670574475068));
#32174=CARTESIAN_POINT('Ctrl Pts',(-41.4217720606996,12.4905558027012,-11.3734544105145));
#32175=CARTESIAN_POINT('Ctrl Pts',(-42.9601423694208,12.8156483043099,-12.4221714958467));
#32176=CARTESIAN_POINT('Ctrl Pts',(-46.3511338849127,13.5449152868614,-13.8545909095391));
#32177=CARTESIAN_POINT('Ctrl Pts',(-48.1597570334068,13.9494605087261,-14.2195188100293));
#32178=CARTESIAN_POINT('Ctrl Pts',(-49.9808845034561,14.3528169182249,-14.2201291128084));
#32179=CARTESIAN_POINT('Ctrl Pts',(-36.5850719698905,9.50149509066535,0.));
#32180=CARTESIAN_POINT('Ctrl Pts',(-36.6214111051725,9.38007537749594,-1.86858636170199));
#32181=CARTESIAN_POINT('Ctrl Pts',(-37.0055036281526,9.36705556804786,-3.71029995870503));
#32182=CARTESIAN_POINT('Ctrl Pts',(-38.451897363611,9.52533731124314,-7.1693624749302));
#32183=CARTESIAN_POINT('Ctrl Pts',(-39.492347221471,9.70422705234564,-8.73699595770811));
#32184=CARTESIAN_POINT('Ctrl Pts',(-40.9249807596918,9.9806131216229,-10.1890856763501));
#32185=CARTESIAN_POINT('Ctrl Pts',(-41.0597112354463,10.006897376716,-10.3203928635172));
#32186=CARTESIAN_POINT('Ctrl Pts',(-41.1968114628076,10.0339108358061,-10.4488603766004));
#32187=CARTESIAN_POINT('Ctrl Pts',(-35.914217116421,11.7862169042734,-1.22124532708767E-15));
#32188=CARTESIAN_POINT('Ctrl Pts',(-35.9492898606247,11.6644253451772,-1.86860431092127));
#32189=CARTESIAN_POINT('Ctrl Pts',(-36.3359843740511,11.6521696602785,-3.70979114471603));
#32190=CARTESIAN_POINT('Ctrl Pts',(-37.7794742164016,11.809598506505,-7.17014261467971));
#32191=CARTESIAN_POINT('Ctrl Pts',(-38.8217053622759,11.9890114303897,-8.73670574475068));
#32192=CARTESIAN_POINT('Ctrl Pts',(-40.2612951155293,12.2667035909867,-10.196605355572));
#32193=CARTESIAN_POINT('Ctrl Pts',(-40.4035980344055,12.2944800077075,-10.3350231942279));
#32194=CARTESIAN_POINT('Ctrl Pts',(-40.5485470057464,12.3230698430838,-10.4702558451006));
#32195=CARTESIAN_POINT('Ctrl Pts',(-43.6145083358836,9.34279883641509,1.24689082988537));
#32196=CARTESIAN_POINT('Ctrl Pts',(-43.6025047583784,9.29352897570348,0.764254661685365));
#32197=CARTESIAN_POINT('Ctrl Pts',(-43.5898343018983,9.24710292813362,0.332948671153414));
#32198=CARTESIAN_POINT('Ctrl Pts',(-43.6387527331905,9.08959664356559,-0.978870002777604));
#32199=CARTESIAN_POINT('Ctrl Pts',(-43.8630440977203,9.02147253460984,-1.98783577088221));
#32200=CARTESIAN_POINT('Ctrl Pts',(-44.6599232717658,8.99867539144857,-3.80852727284259));
#32201=CARTESIAN_POINT('Ctrl Pts',(-45.2360569807998,9.03489241252397,-4.65544360722721));
#32202=CARTESIAN_POINT('Ctrl Pts',(-46.6460662566679,9.18984064605092,-6.04997283342596));
#32203=CARTESIAN_POINT('Ctrl Pts',(-47.4916031396373,9.30516165135672,-6.61832169900054));
#32204=CARTESIAN_POINT('Ctrl Pts',(-49.3114553051051,9.5827363353036,-7.36768403081585));
#32205=CARTESIAN_POINT('Ctrl Pts',(-50.3172192201065,9.74382459494245,-7.57138648668015));
#32206=CARTESIAN_POINT('Ctrl Pts',(-51.2881489781559,9.90091582292617,-7.56962581969428));
#32207=CARTESIAN_POINT('Ctrl Pts',(-41.3128793157233,9.90389776310336,1.35489321026544));
#32208=CARTESIAN_POINT('Ctrl Pts',(-41.3011741506654,9.85585276552896,0.884255518278619));
#32209=CARTESIAN_POINT('Ctrl Pts',(-41.2854482448446,9.80727935893038,0.426396949034063));
#32210=CARTESIAN_POINT('Ctrl Pts',(-41.3339507669686,9.64806121736179,-1.25360819503921));
#32211=CARTESIAN_POINT('Ctrl Pts',(-41.6081209011007,9.5971095076056,-2.51960912779453));
#32212=CARTESIAN_POINT('Ctrl Pts',(-42.6049670390268,9.63005248742562,-4.84647586782619));
#32213=CARTESIAN_POINT('Ctrl Pts',(-43.3248419422851,9.71043261801081,-5.9157219904686));
#32214=CARTESIAN_POINT('Ctrl Pts',(-45.1023943639257,9.97242546014147,-7.69376028691838));
#32215=CARTESIAN_POINT('Ctrl Pts',(-46.1617613376966,10.1524895065124,-8.4106318655567));
#32216=CARTESIAN_POINT('Ctrl Pts',(-48.466885626621,10.5695775166739,-9.37059840620937));
#32217=CARTESIAN_POINT('Ctrl Pts',(-49.7204896475891,10.8058013195906,-9.62435378613754));
#32218=CARTESIAN_POINT('Ctrl Pts',(-50.9539676685889,11.0389609452144,-9.62320046360541));
#32219=CARTESIAN_POINT('Ctrl Pts',(-38.9464705831155,10.0047404051439,1.47293192394291));
#32220=CARTESIAN_POINT('Ctrl Pts',(-38.9350908951662,9.95803136027088,1.01538091584758));
#32221=CARTESIAN_POINT('Ctrl Pts',(-38.9160550470335,9.90712214456995,0.528580717861568));
#32222=CARTESIAN_POINT('Ctrl Pts',(-38.9644836025053,9.74614391854898,-1.55402875454917));
#32223=CARTESIAN_POINT('Ctrl Pts',(-39.2926120042888,9.71379866052871,-3.10121432124109));
#32224=CARTESIAN_POINT('Ctrl Pts',(-40.5087724506345,9.80788452010445,-5.98129145450301));
#32225=CARTESIAN_POINT('Ctrl Pts',(-41.3854277882649,9.93643935035659,-7.29389406576453));
#32226=CARTESIAN_POINT('Ctrl Pts',(-43.5650308736069,10.3155272531459,-9.49113593804205));
#32227=CARTESIAN_POINT('Ctrl Pts',(-44.8579833049637,10.5663179729168,-10.3708286017171));
#32228=CARTESIAN_POINT('Ctrl Pts',(-47.6940136086746,11.1360404748698,-11.560404556125));
#32229=CARTESIAN_POINT('Ctrl Pts',(-49.2184417855036,11.4544007679043,-11.8694761540619));
#32230=CARTESIAN_POINT('Ctrl Pts',(-50.7390783576438,11.770728108961,-11.8687142284812));
#32231=CARTESIAN_POINT('Ctrl Pts',(-36.6062244663075,9.64145132693344,1.5964706812662));
#32232=CARTESIAN_POINT('Ctrl Pts',(-36.5951848118755,9.59613798296134,1.15259163661763));
#32233=CARTESIAN_POINT('Ctrl Pts',(-36.57271173128,9.54279427445571,0.635573001827313));
#32234=CARTESIAN_POINT('Ctrl Pts',(-36.6214111051725,9.38007537749594,-1.86858636170199));
#32235=CARTESIAN_POINT('Ctrl Pts',(-37.0055036281526,9.36705556804786,-3.71029995870503));
#32236=CARTESIAN_POINT('Ctrl Pts',(-38.451897363611,9.52533731124314,-7.1693624749302));
#32237=CARTESIAN_POINT('Ctrl Pts',(-39.492347221471,9.70422705234564,-8.73699595770811));
#32238=CARTESIAN_POINT('Ctrl Pts',(-42.0930574706453,10.2059604432804,-11.3730256982116));
#32239=CARTESIAN_POINT('Ctrl Pts',(-43.6303739147953,10.5307434056437,-12.423580519237));
#32240=CARTESIAN_POINT('Ctrl Pts',(-47.0225411280958,11.2603557414264,-13.8529470821453));
#32241=CARTESIAN_POINT('Ctrl Pts',(-48.8303727110256,11.6646867918221,-14.2204718556263));
#32242=CARTESIAN_POINT('Ctrl Pts',(-50.6517393542018,12.0680951184147,-14.2198708430666));
#32243=CARTESIAN_POINT('Ctrl Pts',(-35.9359355586898,11.9263392248004,1.59674363861568));
#32244=CARTESIAN_POINT('Ctrl Pts',(-35.924899625982,11.8810411570281,1.15301423610205));
#32245=CARTESIAN_POINT('Ctrl Pts',(-35.9022876226749,11.8276425661526,0.635579106998265));
#32246=CARTESIAN_POINT('Ctrl Pts',(-35.9492898606247,11.6644253451772,-1.86860431092127));
#32247=CARTESIAN_POINT('Ctrl Pts',(-36.3359843740511,11.6521696602785,-3.70979114471722));
#32248=CARTESIAN_POINT('Ctrl Pts',(-37.7794742164016,11.809598506505,-7.17014261467851));
#32249=CARTESIAN_POINT('Ctrl Pts',(-38.8217053622759,11.9890114303897,-8.73670574475307));
#32250=CARTESIAN_POINT('Ctrl Pts',(-41.4217720606996,12.4905558027012,-11.3734544105121));
#32251=CARTESIAN_POINT('Ctrl Pts',(-42.9601423694208,12.8156483043111,-12.4221714958467));
#32252=CARTESIAN_POINT('Ctrl Pts',(-46.3511338849127,13.5449152868602,-13.8545909095391));
#32253=CARTESIAN_POINT('Ctrl Pts',(-48.159757033407,13.9494605087261,-14.2195188100293));
#32254=CARTESIAN_POINT('Ctrl Pts',(-49.9808845034561,14.3528169182249,-14.2201291128084));
#32255=CARTESIAN_POINT('Ctrl Pts',(-38.1015519292156,12.8849080239688,1.47327599461702));
#32256=CARTESIAN_POINT('Ctrl Pts',(-38.0901769326121,12.8382182351928,1.0159136147825));
#32257=CARTESIAN_POINT('Ctrl Pts',(-38.0709659683617,12.787239838666,0.528588413607038));
#32258=CARTESIAN_POINT('Ctrl Pts',(-38.1172552346282,12.6256334607371,-1.55405138006188));
#32259=CARTESIAN_POINT('Ctrl Pts',(-38.4486635210218,12.5942514039233,-3.10057294641456));
#32260=CARTESIAN_POINT('Ctrl Pts',(-39.6611635256837,12.6872621620782,-5.9822748433383));
#32261=CARTESIAN_POINT('Ctrl Pts',(-40.5400642286511,12.8164764794374,-7.29352824389523));
#32262=CARTESIAN_POINT('Ctrl Pts',(-42.7188560995434,13.1953261187531,-9.49167634236253));
#32263=CARTESIAN_POINT('Ctrl Pts',(-44.0131369578426,13.4465070217416,-10.3690524867731));
#32264=CARTESIAN_POINT('Ctrl Pts',(-46.8476852602797,14.0157941959106,-11.5624766483414));
#32265=CARTESIAN_POINT('Ctrl Pts',(-48.3731128199116,14.3344204492882,-11.8682745706306));
#32266=CARTESIAN_POINT('Ctrl Pts',(-49.8934463159786,14.6506863563568,-11.8690397849988));
#32267=CARTESIAN_POINT('Ctrl Pts',(-40.0384499621469,14.2481859850621,1.35541218776081));
#32268=CARTESIAN_POINT('Ctrl Pts',(-40.0267518732657,14.2001700323356,0.885059012385724));
#32269=CARTESIAN_POINT('Ctrl Pts',(-40.0107618318058,14.1514922771421,0.42640855687806));
#32270=CARTESIAN_POINT('Ctrl Pts',(-40.0560375664346,13.9913266653952,-1.25364232213227));
#32271=CARTESIAN_POINT('Ctrl Pts',(-40.3351549001509,13.9418277959651,-2.51864171288711));
#32272=CARTESIAN_POINT('Ctrl Pts',(-41.3264798268871,13.9731491512543,-4.84795915806681));
#32273=CARTESIAN_POINT('Ctrl Pts',(-42.049741517119,14.0545240163351,-5.9151702046561));
#32274=CARTESIAN_POINT('Ctrl Pts',(-43.8260703470018,14.3161574747981,-7.69457540340699));
#32275=CARTESIAN_POINT('Ctrl Pts',(-44.8874410477371,14.4968100523227,-8.40795287035882));
#32276=CARTESIAN_POINT('Ctrl Pts',(-47.1903299665196,14.9132414377163,-9.37372383743066));
#32277=CARTESIAN_POINT('Ctrl Pts',(-48.4454445415192,15.1498577118804,-9.62254086012515));
#32278=CARTESIAN_POINT('Ctrl Pts',(-49.6784622796991,15.3829333626942,-9.62369151535384));
#32279=CARTESIAN_POINT('Ctrl Pts',(-41.6721936506077,15.9637816213006,1.24768178593779));
#32280=CARTESIAN_POINT('Ctrl Pts',(-41.6602008576572,15.9145560268582,0.765479239885611));
#32281=CARTESIAN_POINT('Ctrl Pts',(-41.6471278409878,15.8679709451247,0.332966362275953));
#32282=CARTESIAN_POINT('Ctrl Pts',(-41.6911284345662,15.7090206532942,-0.978922014726203));
#32283=CARTESIAN_POINT('Ctrl Pts',(-41.9229596586979,15.6431107691499,-1.98636136652895));
#32284=CARTESIAN_POINT('Ctrl Pts',(-42.7114241414665,15.6178421628833,-3.81078790534779));
#32285=CARTESIAN_POINT('Ctrl Pts',(-43.2927195379906,15.6555752251637,-4.65460264912839));
#32286=CARTESIAN_POINT('Ctrl Pts',(-44.7008639790628,15.8099757341941,-6.05121512490418));
#32287=CARTESIAN_POINT('Ctrl Pts',(-45.5494546745316,15.926193699927,-6.61423873300684));
#32288=CARTESIAN_POINT('Ctrl Pts',(-47.3658999879521,16.2027676442764,-7.3724473948574));
#32289=CARTESIAN_POINT('Ctrl Pts',(-48.3739721396694,16.3644346257032,-7.56862230190484));
#32290=CARTESIAN_POINT('Ctrl Pts',(-49.3441943438429,16.5214173008837,-7.57037421506003));
#32291=CARTESIAN_POINT('Ctrl Pts',(-34.8615042977019,14.752924178887,1.59647077610298));
#32292=CARTESIAN_POINT('Ctrl Pts',(-34.857025771947,14.7065009496435,1.1525917014061));
#32293=CARTESIAN_POINT('Ctrl Pts',(-34.8423730342687,14.6505019462284,0.635573044894269));
#32294=CARTESIAN_POINT('Ctrl Pts',(-34.9137340335311,14.4963699338419,-1.86858636178585));
#32295=CARTESIAN_POINT('Ctrl Pts',(-35.2957699604605,14.5381447126175,-3.71029995870276));
#32296=CARTESIAN_POINT('Ctrl Pts',(-36.7049156525828,14.9006586664088,-7.16936247493249));
#32297=CARTESIAN_POINT('Ctrl Pts',(-37.7093165664795,15.2257990211696,-8.7369959577155));
#32298=CARTESIAN_POINT('Ctrl Pts',(-40.2121512288796,16.0925451480898,-11.3730256982043));
#32299=CARTESIAN_POINT('Ctrl Pts',(-41.6875985735023,16.6328052292555,-12.4235805192037));
#32300=CARTESIAN_POINT('Ctrl Pts',(-44.9414037540494,17.8377468919989,-13.8529470821786));
#32301=CARTESIAN_POINT('Ctrl Pts',(-46.6732919100481,18.4952436947574,-14.2204718556881));
#32302=CARTESIAN_POINT('Ctrl Pts',(-48.4187086763094,19.1537534053194,-14.2198708430667));
#32303=CARTESIAN_POINT('Ctrl Pts',(-33.9925722540019,15.1415840475453,1.62964621771058));
#32304=CARTESIAN_POINT('Ctrl Pts',(-33.9881310914378,15.095548115337,1.18947031171891));
#32305=CARTESIAN_POINT('Ctrl Pts',(-33.9726251531373,15.0387526938571,0.664244003018932));
#32306=CARTESIAN_POINT('Ctrl Pts',(-34.043697838502,14.8839745452467,-1.95287905129093));
#32307=CARTESIAN_POINT('Ctrl Pts',(-34.4404940724067,14.9333078251056,-3.87337387078857));
#32308=CARTESIAN_POINT('Ctrl Pts',(-35.9075266006076,15.321294855491,-7.48792130213727));
#32309=CARTESIAN_POINT('Ctrl Pts',(-36.9538988571888,15.6662361881643,-9.1236083623312));
#32310=CARTESIAN_POINT('Ctrl Pts',(-39.5635848920882,16.5814962694126,-11.8774049927));
#32311=CARTESIAN_POINT('Ctrl Pts',(-41.1012880289292,17.1508209097894,-12.9732563608727));
#32312=CARTESIAN_POINT('Ctrl Pts',(-44.4962044519299,18.4192429936658,-14.4676858045621));
#32313=CARTESIAN_POINT('Ctrl Pts',(-46.3001798643524,19.1104364369558,-14.8501851005151));
#32314=CARTESIAN_POINT('Ctrl Pts',(-48.1219785107276,19.8034868749642,-14.8499483202528));
#32315=CARTESIAN_POINT('Ctrl Pts',(-33.597116340133,16.0080796379929,1.62975540065037));
#32316=CARTESIAN_POINT('Ctrl Pts',(-33.5926757814912,15.9620499659323,1.18963935151889));
#32317=CARTESIAN_POINT('Ctrl Pts',(-33.5771179639666,15.9052249066534,0.664246445091293));
#32318=CARTESIAN_POINT('Ctrl Pts',(-33.647547072249,15.7501528462652,-1.95288623098987));
#32319=CARTESIAN_POINT('Ctrl Pts',(-34.0453300100375,15.7999367856098,-3.87317034519032));
#32320=CARTESIAN_POINT('Ctrl Pts',(-35.5112613559224,16.1874208228852,-7.48823335803971));
#32321=CARTESIAN_POINT('Ctrl Pts',(-36.5583090926775,16.5326707000636,-9.12349227715013));
#32322=CARTESIAN_POINT('Ctrl Pts',(-39.1677510874848,17.447819308696,-11.8775764776193));
#32323=CARTESIAN_POINT('Ctrl Pts',(-40.7058538586162,18.0173264967329,-12.9726927515434));
#32324=CARTESIAN_POINT('Ctrl Pts',(-44.1003244488304,19.2855449177099,-14.4683433354928));
#32325=CARTESIAN_POINT('Ctrl Pts',(-45.9046009234708,19.9768684693681,-14.8498038985005));
#32326=CARTESIAN_POINT('Ctrl Pts',(-47.7263079790886,20.6698844856026,-14.8500516281495));
#32327=CARTESIAN_POINT('Ctrl Pts',(-33.8728645130296,16.919163155006,1.59674373345245));
#32328=CARTESIAN_POINT('Ctrl Pts',(-33.8683874970857,16.8727555761311,1.15301430090585));
#32329=CARTESIAN_POINT('Ctrl Pts',(-33.8536050613443,16.816682478221,0.635579150075179));
#32330=CARTESIAN_POINT('Ctrl Pts',(-33.9233571178916,16.6618156863834,-1.86860431103318));
#32331=CARTESIAN_POINT('Ctrl Pts',(-34.3078598045327,16.7047171138864,-3.70979114470774));
#32332=CARTESIAN_POINT('Ctrl Pts',(-35.7142525408745,17.0659735848861,-7.17014261468798));
#32333=CARTESIAN_POINT('Ctrl Pts',(-36.720342155194,17.3918853009154,-8.73670574476044));
#32334=CARTESIAN_POINT('Ctrl Pts',(-39.2225667173783,18.2583527463007,-11.3734544105047));
#32335=CARTESIAN_POINT('Ctrl Pts',(-40.6990131477318,18.7990691966204,-12.4221714958709));
#32336=CARTESIAN_POINT('Ctrl Pts',(-43.9517037462886,20.0035017021032,-13.8545909095149));
#32337=CARTESIAN_POINT('Ctrl Pts',(-45.6843449310622,20.6613231478773,-14.2195188099484));
#32338=CARTESIAN_POINT('Ctrl Pts',(-47.429532347212,21.3197474319156,-14.2201291128084));
#32339=CARTESIAN_POINT('Ctrl Pts',(-34.8604849513722,14.6113821712785,0.));
#32340=CARTESIAN_POINT('Ctrl Pts',(-34.9137340335311,14.4963699338419,-1.86858636178585));
#32341=CARTESIAN_POINT('Ctrl Pts',(-35.2957699604605,14.5381447126175,-3.71029995870396));
#32342=CARTESIAN_POINT('Ctrl Pts',(-36.7049156525828,14.9006586664088,-7.16936247493129));
#32343=CARTESIAN_POINT('Ctrl Pts',(-37.7093165664795,15.225799021172,-8.73699595771789));
#32344=CARTESIAN_POINT('Ctrl Pts',(-39.0880341222376,15.7032568890511,-10.1890856763494));
#32345=CARTESIAN_POINT('Ctrl Pts',(-39.2176525965035,15.748447754191,-10.3203928635156));
#32346=CARTESIAN_POINT('Ctrl Pts',(-39.3495129251727,15.7946976518991,-10.4488603765979));
#32347=CARTESIAN_POINT('Ctrl Pts',(-33.8713086176151,16.7773762111444,1.66533453693773E-16));
#32348=CARTESIAN_POINT('Ctrl Pts',(-33.9233571178916,16.6618156863834,-1.86860431103318));
#32349=CARTESIAN_POINT('Ctrl Pts',(-34.3078598045327,16.7047171138864,-3.70979114470774));
#32350=CARTESIAN_POINT('Ctrl Pts',(-35.7142525408745,17.0659735848861,-7.17014261468798));
#32351=CARTESIAN_POINT('Ctrl Pts',(-36.720342155194,17.3918853009154,-8.73670574476044));
#32352=CARTESIAN_POINT('Ctrl Pts',(-38.1057592455502,17.8716259385927,-10.196605355572));
#32353=CARTESIAN_POINT('Ctrl Pts',(-38.2426607296438,17.9193714483236,-10.3350231942284));
#32354=CARTESIAN_POINT('Ctrl Pts',(-38.382065571659,17.9682986698096,-10.4702558451019));
#32355=CARTESIAN_POINT('Ctrl Pts',(-41.8409566234847,15.4546943255723,1.24689092472229));
#32356=CARTESIAN_POINT('Ctrl Pts',(-41.8360870570322,15.4042176703914,0.764254723812363));
#32357=CARTESIAN_POINT('Ctrl Pts',(-41.8301526811182,15.356460975121,0.332948693666065));
#32358=CARTESIAN_POINT('Ctrl Pts',(-41.9009886759728,15.207519693579,-0.978870002679738));
#32359=CARTESIAN_POINT('Ctrl Pts',(-42.1326921493261,15.1720089790277,-1.98783577089606));
#32360=CARTESIAN_POINT('Ctrl Pts',(-42.9247046141597,15.2628516087108,-3.80852727282881));
#32361=CARTESIAN_POINT('Ctrl Pts',(-43.4898198932031,15.3806923683063,-4.65544360720821));
#32362=CARTESIAN_POINT('Ctrl Pts',(-44.8634258749837,15.7347286943737,-6.04997283344502));
#32363=CARTESIAN_POINT('Ctrl Pts',(-45.6839445213885,15.9692083429235,-6.61832169892883));
#32364=CARTESIAN_POINT('Ctrl Pts',(-47.4457702195768,16.5029496832554,-7.36768403088772));
#32365=CARTESIAN_POINT('Ctrl Pts',(-48.4183716585645,16.8055334254949,-7.57138648688498));
#32366=CARTESIAN_POINT('Ctrl Pts',(-49.3570623388652,17.0992034029529,-7.5696258196944));
#32367=CARTESIAN_POINT('Ctrl Pts',(-39.4829021650676,15.6825261124556,1.35489330510232));
#32368=CARTESIAN_POINT('Ctrl Pts',(-39.4781536574581,15.6333043216781,0.884255581230426));
#32369=CARTESIAN_POINT('Ctrl Pts',(-39.4695005333236,15.5829872885716,0.426396977895696));
#32370=CARTESIAN_POINT('Ctrl Pts',(-39.5401684750185,15.4322923841483,-1.25360819500321));
#32371=CARTESIAN_POINT('Ctrl Pts',(-39.8187991367997,15.4208777676018,-2.51960912780342));
#32372=CARTESIAN_POINT('Ctrl Pts',(-40.8008105435659,15.5953514322915,-4.84647586781735));
#32373=CARTESIAN_POINT('Ctrl Pts',(-41.5019188729544,15.7773622894618,-5.91572199046159));
#32374=CARTESIAN_POINT('Ctrl Pts',(-43.2240929050568,16.2896605076646,-7.69376028692545));
#32375=CARTESIAN_POINT('Ctrl Pts',(-44.2470512648569,16.6186554012354,-8.41063186550418));
#32376=CARTESIAN_POINT('Ctrl Pts',(-46.4693548995128,17.3595514471548,-9.37059840626199));
#32377=CARTESIAN_POINT('Ctrl Pts',(-47.6765808868229,17.7717772858477,-9.62435378628037));
#32378=CARTESIAN_POINT('Ctrl Pts',(-48.8643218056538,18.1781059077968,-9.62320046360549));
#32379=CARTESIAN_POINT('Ctrl Pts',(-37.1262286569851,15.4455672457339,1.47293201877974));
#32380=CARTESIAN_POINT('Ctrl Pts',(-37.1216121877099,15.3977141299005,1.01538097969802));
#32381=CARTESIAN_POINT('Ctrl Pts',(-37.1100152319898,15.3446140089039,0.528580753663548));
#32382=CARTESIAN_POINT('Ctrl Pts',(-37.1808604460415,15.1921664085235,-1.55402875457453));
#32383=CARTESIAN_POINT('Ctrl Pts',(-37.5102521839442,15.2068479190352,-3.10121432124141));
#32384=CARTESIAN_POINT('Ctrl Pts',(-38.7006440566484,15.4730537974485,-5.98129145450273));
#32385=CARTESIAN_POINT('Ctrl Pts',(-39.550081047065,15.7250611874948,-7.29389406576472));
#32386=CARTESIAN_POINT('Ctrl Pts',(-41.653549082182,16.4104803826143,-9.4911359380419));
#32387=CARTESIAN_POINT('Ctrl Pts',(-42.8976498813487,16.8427247306107,-10.3708286016838));
#32388=CARTESIAN_POINT('Ctrl Pts',(-45.6237335200226,17.8102574730284,-11.5604045561584));
#32389=CARTESIAN_POINT('Ctrl Pts',(-47.0873378224411,18.3423260668025,-11.8694761541428));
#32390=CARTESIAN_POINT('Ctrl Pts',(-48.547478432487,18.8718427994039,-11.8687142284812));
#32391=CARTESIAN_POINT('Ctrl Pts',(-34.8615042977019,14.752924178887,1.59647077610298));
#32392=CARTESIAN_POINT('Ctrl Pts',(-34.857025771947,14.7065009496435,1.1525917014061));
#32393=CARTESIAN_POINT('Ctrl Pts',(-34.8423730342687,14.6505019462284,0.635573044894269));
#32394=CARTESIAN_POINT('Ctrl Pts',(-34.9137340335311,14.4963699338419,-1.86858636178585));
#32395=CARTESIAN_POINT('Ctrl Pts',(-35.2957699604605,14.5381447126175,-3.71029995870396));
#32396=CARTESIAN_POINT('Ctrl Pts',(-36.7049156525828,14.9006586664088,-7.16936247493129));
#32397=CARTESIAN_POINT('Ctrl Pts',(-37.7093165664795,15.225799021172,-8.73699595771789));
#32398=CARTESIAN_POINT('Ctrl Pts',(-40.2121512288796,16.0925451480874,-11.3730256982019));
#32399=CARTESIAN_POINT('Ctrl Pts',(-41.6875985735023,16.6328052292555,-12.4235805192037));
#32400=CARTESIAN_POINT('Ctrl Pts',(-44.9414037540494,17.8377468919989,-13.8529470821786));
#32401=CARTESIAN_POINT('Ctrl Pts',(-46.6732919100457,18.4952436947636,-14.2204718556929));
#32402=CARTESIAN_POINT('Ctrl Pts',(-48.4187086763094,19.1537534053194,-14.2198708430667));
#32403=CARTESIAN_POINT('Ctrl Pts',(-33.8728645130296,16.9191631550061,1.59674373345245));
#32404=CARTESIAN_POINT('Ctrl Pts',(-33.8683874970857,16.8727555761311,1.15301430090585));
#32405=CARTESIAN_POINT('Ctrl Pts',(-33.8536050613443,16.816682478221,0.635579150075179));
#32406=CARTESIAN_POINT('Ctrl Pts',(-33.9233571178916,16.6618156863834,-1.86860431103318));
#32407=CARTESIAN_POINT('Ctrl Pts',(-34.3078598045327,16.7047171138864,-3.70979114470774));
#32408=CARTESIAN_POINT('Ctrl Pts',(-35.7142525408745,17.0659735848861,-7.17014261468798));
#32409=CARTESIAN_POINT('Ctrl Pts',(-36.7203421551987,17.3918853009154,-8.73670574475805));
#32410=CARTESIAN_POINT('Ctrl Pts',(-39.2225667173735,18.2583527463006,-11.3734544105071));
#32411=CARTESIAN_POINT('Ctrl Pts',(-40.6990131477318,18.7990691966228,-12.4221714958757));
#32412=CARTESIAN_POINT('Ctrl Pts',(-43.9517037462886,20.0035017021008,-13.8545909095101));
#32413=CARTESIAN_POINT('Ctrl Pts',(-45.6843449310646,20.6613231478728,-14.2195188099532));
#32414=CARTESIAN_POINT('Ctrl Pts',(-47.429532347212,21.3197474319156,-14.2201291128084));
#32415=CARTESIAN_POINT('Ctrl Pts',(-35.880019467837,18.1761744494742,1.47327608945385));
#32416=CARTESIAN_POINT('Ctrl Pts',(-35.8754049017175,18.1283410613835,1.015913678653));
#32417=CARTESIAN_POINT('Ctrl Pts',(-35.8636444578228,18.0751475421239,0.528588449421553));
#32418=CARTESIAN_POINT('Ctrl Pts',(-35.932461552811,17.9217737308839,-1.55405138012259));
#32419=CARTESIAN_POINT('Ctrl Pts',(-36.2649627130451,17.9378754148675,-3.10057294640886));
#32420=CARTESIAN_POINT('Ctrl Pts',(-37.4518844049458,18.2024961996707,-5.982274843344));
#32421=CARTESIAN_POINT('Ctrl Pts',(-38.3034500513458,18.4554759130143,-7.29352824389302));
#32422=CARTESIAN_POINT('Ctrl Pts',(-40.4061490373992,19.1405438219642,-9.49167634236476));
#32423=CARTESIAN_POINT('Ctrl Pts',(-41.6515092131746,19.5733634365479,-10.3690524868116));
#32424=CARTESIAN_POINT('Ctrl Pts',(-44.3761878888518,20.540254371427,-11.5624766483028));
#32425=CARTESIAN_POINT('Ctrl Pts',(-45.840743551661,21.0727284454457,-11.8682745705212));
#32426=CARTESIAN_POINT('Ctrl Pts',(-47.3005929134933,21.6021412371497,-11.8690397849987));
#32427=CARTESIAN_POINT('Ctrl Pts',(-37.603187989015,19.8012255369164,1.35541228259769));
#32428=CARTESIAN_POINT('Ctrl Pts',(-37.5984423520298,19.7520335023962,0.885059075367221));
#32429=CARTESIAN_POINT('Ctrl Pts',(-37.5895426312144,19.7015755924255,0.426408585758618));
#32430=CARTESIAN_POINT('Ctrl Pts',(-37.6571514683988,19.549483641906,-1.2536423221496));
#32431=CARTESIAN_POINT('Ctrl Pts',(-37.9404722137416,19.5402111378006,-2.51864171288158));
#32432=CARTESIAN_POINT('Ctrl Pts',(-38.9172493884832,19.7122939334796,-4.84795915807232));
#32433=CARTESIAN_POINT('Ctrl Pts',(-39.62156846681,19.8957713902405,-5.91517020464428));
#32434=CARTESIAN_POINT('Ctrl Pts',(-41.3425825071162,20.4075397474871,-7.69457540341882));
#32435=CARTESIAN_POINT('Ctrl Pts',(-42.3674404421148,20.7374023418884,-8.40795287041649));
#32436=CARTESIAN_POINT('Ctrl Pts',(-44.5876249069854,21.4773303202329,-9.37372383737288));
#32437=CARTESIAN_POINT('Ctrl Pts',(-45.7962902185241,21.8901596096075,-9.62254085999184));
#32438=CARTESIAN_POINT('Ctrl Pts',(-46.9835874904387,22.2963396064212,-9.62369151535377));
#32439=CARTESIAN_POINT('Ctrl Pts',(-38.9761478068776,21.7318648520658,1.24768188077471));
#32440=CARTESIAN_POINT('Ctrl Pts',(-38.9712826154474,21.6814335473931,0.765479302057181));
#32441=CARTESIAN_POINT('Ctrl Pts',(-38.9649724098685,21.6334621464558,0.332966384817446));
#32442=CARTESIAN_POINT('Ctrl Pts',(-39.0311461269804,21.482391674194,-0.978922014709598));
#32443=CARTESIAN_POINT('Ctrl Pts',(-39.2699975980932,21.450145680789,-1.98636136652356));
#32444=CARTESIAN_POINT('Ctrl Pts',(-40.0540327468988,21.5373444678476,-3.81078790535314));
#32445=CARTESIAN_POINT('Ctrl Pts',(-40.6240414198234,21.657420422293,-4.65460264910458));
#32446=CARTESIAN_POINT('Ctrl Pts',(-41.9958794973358,22.0106492051928,-6.051215124928));
#32447=CARTESIAN_POINT('Ctrl Pts',(-42.8192932220765,22.2464512872438,-6.61423873309801));
#32448=CARTESIAN_POINT('Ctrl Pts',(-44.5778891652326,22.7787172285086,-7.37244739476607));
#32449=CARTESIAN_POINT('Ctrl Pts',(-45.5526929856396,23.0822022983076,-7.56862230169532));
#32450=CARTESIAN_POINT('Ctrl Pts',(-46.4906987626549,23.3756641324467,-7.57037421505994));
#32451=CARTESIAN_POINT('Ctrl Pts',(-31.1202396243797,21.567561713547,1.59674381934676));
#32452=CARTESIAN_POINT('Ctrl Pts',(-31.1224126652072,21.520989348265,1.15301435962634));
#32453=CARTESIAN_POINT('Ctrl Pts',(-31.1157607260923,21.4633832297208,0.635579189057524));
#32454=CARTESIAN_POINT('Ctrl Pts',(-31.2068426511149,21.320019509059,-1.86860431103819));
#32455=CARTESIAN_POINT('Ctrl Pts',(-31.5813261451172,21.4172046994746,-3.70979114470734));
#32456=CARTESIAN_POINT('Ctrl Pts',(-32.9219916749895,21.9749346552901,-7.17014261468839));
#32457=CARTESIAN_POINT('Ctrl Pts',(-33.8714586745438,22.4407105406856,-8.73670574473668));
#32458=CARTESIAN_POINT('Ctrl Pts',(-36.2249030242442,23.6544622808116,-11.3734544105284));
#32459=CARTESIAN_POINT('Ctrl Pts',(-37.609369384537,24.39979525241,-12.4221714958177));
#32460=CARTESIAN_POINT('Ctrl Pts',(-40.6575436657173,26.0548745077421,-13.854590909568));
#32461=CARTESIAN_POINT('Ctrl Pts',(-42.2789313088126,26.9525808298053,-14.2195188100055));
#32462=CARTESIAN_POINT('Ctrl Pts',(-43.9126516878553,27.8526693689671,-14.2201291128083));
#32463=CARTESIAN_POINT('Ctrl Pts',(-32.9280732767458,23.0974263782808,1.47327617534825));
#32464=CARTESIAN_POINT('Ctrl Pts',(-32.9303130812698,23.0494231409436,1.01591373651662));
#32465=CARTESIAN_POINT('Ctrl Pts',(-32.9262425677185,22.9950973654565,0.528588481838949));
#32466=CARTESIAN_POINT('Ctrl Pts',(-33.0161865744697,22.8530783700625,-1.55405138011843));
#32467=CARTESIAN_POINT('Ctrl Pts',(-33.3430118437576,22.9163360109255,-3.10057294640473));
#32468=CARTESIAN_POINT('Ctrl Pts',(-34.4801929200291,23.347179906303,-5.98227484334812));
#32469=CARTESIAN_POINT('Ctrl Pts',(-35.287088088999,23.7187750781554,-7.29352824388356));
#32470=CARTESIAN_POINT('Ctrl Pts',(-37.2708893025901,24.6961152497751,-9.49167634237414));
#32471=CARTESIAN_POINT('Ctrl Pts',(-38.441976853959,25.3017626168119,-10.3690524867345));
#32472=CARTESIAN_POINT('Ctrl Pts',(-41.0013193023666,26.6465742010366,-11.5624766483798));
#32473=CARTESIAN_POINT('Ctrl Pts',(-42.3751889385489,27.3820564590927,-11.8682745706115));
#32474=CARTESIAN_POINT('Ctrl Pts',(-43.7448358429354,28.1138388177854,-11.8690397849987));
#32475=CARTESIAN_POINT('Ctrl Pts',(-34.402433544287,24.951169238192,1.35541236849215));
#32476=CARTESIAN_POINT('Ctrl Pts',(-34.4047369675988,24.9018025300722,0.885059132417908));
#32477=CARTESIAN_POINT('Ctrl Pts',(-34.4031087413091,24.8505916427384,0.426408611904495));
#32478=CARTESIAN_POINT('Ctrl Pts',(-34.491674360816,24.7096695075291,-1.25364232213153));
#32479=CARTESIAN_POINT('Ctrl Pts',(-34.7734309243617,24.740812130188,-2.51864171287491));
#32480=CARTESIAN_POINT('Ctrl Pts',(-35.7157759805954,25.0501532567791,-4.84795915807897));
#32481=CARTESIAN_POINT('Ctrl Pts',(-36.3868145416537,25.3319982332986,-5.91517020464913));
#32482=CARTESIAN_POINT('Ctrl Pts',(-38.0174789095801,26.083483361411,-7.69457540341387));
#32483=CARTESIAN_POINT('Ctrl Pts',(-38.984960926787,26.5558409214617,-8.4079528702915));
#32484=CARTESIAN_POINT('Ctrl Pts',(-41.0772443843504,27.6042026929775,-9.37372383749777));
#32485=CARTESIAN_POINT('Ctrl Pts',(-42.2148554923058,28.1848409837727,-9.6225408600775));
#32486=CARTESIAN_POINT('Ctrl Pts',(-43.332262349351,28.7558566730953,-9.62369151535374));
#32487=CARTESIAN_POINT('Ctrl Pts',(-35.486659988949,27.0575499832999,1.24768196666921));
#32488=CARTESIAN_POINT('Ctrl Pts',(-35.4890214412267,27.0069396045613,0.765479358370163));
#32489=CARTESIAN_POINT('Ctrl Pts',(-35.4896025055318,26.9585584436997,0.332966405226273));
#32490=CARTESIAN_POINT('Ctrl Pts',(-35.5766022409445,26.8184431506731,-0.97892201467345));
#32491=CARTESIAN_POINT('Ctrl Pts',(-35.8176116317276,26.8205174834717,-1.98636136651437));
#32492=CARTESIAN_POINT('Ctrl Pts',(-36.5812567518819,27.0184085480268,-3.81078790536229));
#32493=CARTESIAN_POINT('Ctrl Pts',(-37.1283749683434,27.2183829944883,-4.65460264912373));
#32494=CARTESIAN_POINT('Ctrl Pts',(-38.4359800152259,27.7632493318237,-6.05121512490869));
#32495=CARTESIAN_POINT('Ctrl Pts',(-39.2174544404323,28.1138352796401,-6.61423873291071));
#32496=CARTESIAN_POINT('Ctrl Pts',(-40.8824010709582,28.8909578185445,-7.37244739495321));
#32497=CARTESIAN_POINT('Ctrl Pts',(-41.8040923655509,29.3300828959434,-7.56862230183338));
#32498=CARTESIAN_POINT('Ctrl Pts',(-42.6907866227634,29.7540498521221,-7.57037421505989));
#32499=CARTESIAN_POINT('Ctrl Pts',(-31.1388779521428,21.4269965203143,6.66133814775094E-16));
#32500=CARTESIAN_POINT('Ctrl Pts',(-31.2068426511149,21.320019509059,-1.86860431103819));
#32501=CARTESIAN_POINT('Ctrl Pts',(-31.5813261451172,21.4172046994746,-3.70979114470734));
#32502=CARTESIAN_POINT('Ctrl Pts',(-32.9219916749895,21.9749346552901,-7.17014261468839));
#32503=CARTESIAN_POINT('Ctrl Pts',(-33.8714586745438,22.4407105406856,-8.73670574473668));
#32504=CARTESIAN_POINT('Ctrl Pts',(-35.174500005265,23.1127335196102,-10.1966053555722));
#32505=CARTESIAN_POINT('Ctrl Pts',(-35.3032131351478,23.1794761614689,-10.3350231942278));
#32506=CARTESIAN_POINT('Ctrl Pts',(-35.4342359672601,23.247744751939,-10.4702558450996));
#32507=CARTESIAN_POINT('Ctrl Pts',(-39.2156436908076,21.2519768052527,1.24689101061711));
#32508=CARTESIAN_POINT('Ctrl Pts',(-39.2180072667082,21.2013209149781,0.764254780044368));
#32509=CARTESIAN_POINT('Ctrl Pts',(-39.2189297793852,21.1532057605131,0.332948714099626));
#32510=CARTESIAN_POINT('Ctrl Pts',(-39.3102413217382,21.0158614973477,-0.978870002719474));
#32511=CARTESIAN_POINT('Ctrl Pts',(-39.5446400894402,21.0136870730836,-1.98783577088449));
#32512=CARTESIAN_POINT('Ctrl Pts',(-40.3156627552177,21.2163201816587,-3.80852727284038));
#32513=CARTESIAN_POINT('Ctrl Pts',(-40.8582554869351,21.4133857818112,-4.65544360722271));
#32514=CARTESIAN_POINT('Ctrl Pts',(-42.1674955178514,21.959303041602,-6.04997283343062));
#32515=CARTESIAN_POINT('Ctrl Pts',(-42.9462925343072,22.3081680037475,-6.61832169909177));
#32516=CARTESIAN_POINT('Ctrl Pts',(-44.6142260746748,23.0872105665078,-7.36768403072499));
#32517=CARTESIAN_POINT('Ctrl Pts',(-45.5338656769843,23.5251300588861,-7.57138648682314));
#32518=CARTESIAN_POINT('Ctrl Pts',(-46.4212082443694,23.9494005117262,-7.56962581969446));
#32519=CARTESIAN_POINT('Ctrl Pts',(-36.8491669828396,21.1419034541629,1.35489339099699));
#32520=CARTESIAN_POINT('Ctrl Pts',(-36.8514717995443,21.0925068841255,0.884255638228302));
#32521=CARTESIAN_POINT('Ctrl Pts',(-36.8500676110146,21.0414705340931,0.426397004057789));
#32522=CARTESIAN_POINT('Ctrl Pts',(-36.9414623772912,20.9023665809846,-1.25360819503494));
#32523=CARTESIAN_POINT('Ctrl Pts',(-37.2188814500308,20.930721426378,-2.51960912779677));
#32524=CARTESIAN_POINT('Ctrl Pts',(-38.1660672052366,21.2431739952863,-4.84647586782401));
#32525=CARTESIAN_POINT('Ctrl Pts',(-38.8341364170724,21.5231103628896,-5.91572199046653));
#32526=CARTESIAN_POINT('Ctrl Pts',(-40.4658735625807,22.2752850427188,-7.69376028692058));
#32527=CARTESIAN_POINT('Ctrl Pts',(-41.4315988261873,22.7465133961231,-8.4106318656095));
#32528=CARTESIAN_POINT('Ctrl Pts',(-43.5258421132404,23.7961349710949,-9.37059840615683));
#32529=CARTESIAN_POINT('Ctrl Pts',(-44.662114427036,24.3759711161915,-9.6243537862471));
#32530=CARTESIAN_POINT('Ctrl Pts',(-45.7799392638233,24.9471970554251,-9.62320046360553));
#32531=CARTESIAN_POINT('Ctrl Pts',(-34.5502037758216,20.5719668778723,1.47293210467427));
#32532=CARTESIAN_POINT('Ctrl Pts',(-34.5524445041311,20.5239438427405,1.01538103752678));
#32533=CARTESIAN_POINT('Ctrl Pts',(-34.5485225226913,20.4697337816475,0.52858078609168));
#32534=CARTESIAN_POINT('Ctrl Pts',(-34.6403421915888,20.3289202010311,-1.55402875460338));
#32535=CARTESIAN_POINT('Ctrl Pts',(-34.9642917997815,20.3903296068275,-3.10121432123848));
#32536=CARTESIAN_POINT('Ctrl Pts',(-36.1046821530982,20.8232363200899,-5.98129145450567));
#32537=CARTESIAN_POINT('Ctrl Pts',(-36.909608708792,21.193566126174,-7.29389406575294));
#32538=CARTESIAN_POINT('Ctrl Pts',(-38.8941211503306,22.1713634554236,-9.49113593805375));
#32539=CARTESIAN_POINT('Ctrl Pts',(-40.0640440126769,22.7762621832733,-10.3708286017602));
#32540=CARTESIAN_POINT('Ctrl Pts',(-42.6246857849653,24.1219089895008,-11.560404556082));
#32541=CARTESIAN_POINT('Ctrl Pts',(-43.9976714499894,24.85685450176,-11.8694761541476));
#32542=CARTESIAN_POINT('Ctrl Pts',(-45.3675918458117,25.5887811923515,-11.8687142284812));
#32543=CARTESIAN_POINT('Ctrl Pts',(-32.4071044310924,19.5640700378122,1.59647086199739));
#32544=CARTESIAN_POINT('Ctrl Pts',(-32.4092782047768,19.5174819665907,1.15259176009847));
#32545=CARTESIAN_POINT('Ctrl Pts',(-32.4027440988122,19.4599676463217,0.635573083885156));
#32546=CARTESIAN_POINT('Ctrl Pts',(-32.4953140197739,19.3175602025112,-1.86858636181704));
#32547=CARTESIAN_POINT('Ctrl Pts',(-32.867516200987,19.413279155377,-3.71029995870358));
#32548=CARTESIAN_POINT('Ctrl Pts',(-34.210727707086,19.9726455810862,-7.16936247493171));
#32549=CARTESIAN_POINT('Ctrl Pts',(-35.1586329709074,20.4374176294472,-8.73699595769419));
#32550=CARTESIAN_POINT('Ctrl Pts',(-37.5126415503381,21.6515320408062,-11.3730256982257));
#32551=CARTESIAN_POINT('Ctrl Pts',(-38.8961839422237,22.3962711037012,-12.4235805192657));
#32552=CARTESIAN_POINT('Ctrl Pts',(-41.9453890000128,24.0520129554125,-13.8529470821167));
#32553=CARTESIAN_POINT('Ctrl Pts',(-43.5660774805196,24.9492907716475,-14.2204718556786));
#32554=CARTESIAN_POINT('Ctrl Pts',(-45.2000127177929,25.8494965077555,-14.2198708430667));
#32555=CARTESIAN_POINT('Ctrl Pts',(-32.4262389885812,19.423823646631,6.93889390390723E-15));
#32556=CARTESIAN_POINT('Ctrl Pts',(-32.4953140197739,19.3175602025112,-1.86858636181704));
#32557=CARTESIAN_POINT('Ctrl Pts',(-32.867516200987,19.413279155377,-3.71029995870358));
#32558=CARTESIAN_POINT('Ctrl Pts',(-34.210727707086,19.9726455810862,-7.16936247493171));
#32559=CARTESIAN_POINT('Ctrl Pts',(-35.1586329709074,20.4374176294472,-8.73699595769419));
#32560=CARTESIAN_POINT('Ctrl Pts',(-36.4553678306327,21.106227630677,-10.1890856763504));
#32561=CARTESIAN_POINT('Ctrl Pts',(-36.5772356450577,21.1694051501756,-10.3203928635177));
#32562=CARTESIAN_POINT('Ctrl Pts',(-36.7011717789913,21.2339499719654,-10.4488603766012));
#32563=CARTESIAN_POINT('Ctrl Pts',(-32.4071044310924,19.5640700378122,1.59647086199739));
#32564=CARTESIAN_POINT('Ctrl Pts',(-32.4092782047768,19.5174819665907,1.15259176009847));
#32565=CARTESIAN_POINT('Ctrl Pts',(-32.4027440988122,19.4599676463217,0.635573083885156));
#32566=CARTESIAN_POINT('Ctrl Pts',(-32.4953140197739,19.3175602025112,-1.86858636181704));
#32567=CARTESIAN_POINT('Ctrl Pts',(-32.867516200987,19.413279155377,-3.71029995870358));
#32568=CARTESIAN_POINT('Ctrl Pts',(-34.210727707086,19.9726455810862,-7.16936247493171));
#32569=CARTESIAN_POINT('Ctrl Pts',(-35.1586329709074,20.4374176294472,-8.73699595769419));
#32570=CARTESIAN_POINT('Ctrl Pts',(-37.5126415503381,21.6515320408062,-11.3730256982257));
#32571=CARTESIAN_POINT('Ctrl Pts',(-38.8961839422237,22.3962711037012,-12.4235805192657));
#32572=CARTESIAN_POINT('Ctrl Pts',(-41.9453890000128,24.0520129554125,-13.8529470821167));
#32573=CARTESIAN_POINT('Ctrl Pts',(-43.5660774805196,24.9492907716475,-14.2204718556786));
#32574=CARTESIAN_POINT('Ctrl Pts',(-45.2000127177929,25.8494965077555,-14.2198708430667));
#32575=CARTESIAN_POINT('Ctrl Pts',(-31.4917047963494,19.8251119861393,1.62964630360494));
#32576=CARTESIAN_POINT('Ctrl Pts',(-31.4938604347888,19.7789125871878,1.18947037065042));
#32577=CARTESIAN_POINT('Ctrl Pts',(-31.48659515468,19.7204885321119,0.664244043766078));
#32578=CARTESIAN_POINT('Ctrl Pts',(-31.5789716511435,19.577400497487,-1.95287905131582));
#32579=CARTESIAN_POINT('Ctrl Pts',(-31.9647082138306,19.6827016274759,-3.87337387078821));
#32580=CARTESIAN_POINT('Ctrl Pts',(-33.3615921546903,20.275520006293,-7.48792130213766));
#32581=CARTESIAN_POINT('Ctrl Pts',(-34.3482235804788,20.7658646320009,-9.12360836230511));
#32582=CARTESIAN_POINT('Ctrl Pts',(-36.801091683951,22.0432057314057,-11.8774049927262));
#32583=CARTESIAN_POINT('Ctrl Pts',(-38.2421198758022,22.8255734412324,-12.9732563609011));
#32584=CARTESIAN_POINT('Ctrl Pts',(-41.4219656612033,24.5642317984951,-14.4676858045338));
#32585=CARTESIAN_POINT('Ctrl Pts',(-43.1092121218766,25.5051223583055,-14.8501851005342));
#32586=CARTESIAN_POINT('Ctrl Pts',(-44.8138361237939,26.4503875219919,-14.8499483202528));
#32587=CARTESIAN_POINT('Ctrl Pts',(-30.9769588736643,20.6265086564332,1.62975548654469));
#32588=CARTESIAN_POINT('Ctrl Pts',(-30.9791142189643,20.5803155398589,1.1896394104614));
#32589=CARTESIAN_POINT('Ctrl Pts',(-30.9718018055912,20.5218547654718,0.664246485835027));
#32590=CARTESIAN_POINT('Ctrl Pts',(-31.0635831036823,20.3783842201051,-1.95288623100427));
#32591=CARTESIAN_POINT('Ctrl Pts',(-31.4502321914808,20.4842718451115,-3.87317034518997));
#32592=CARTESIAN_POINT('Ctrl Pts',(-32.8460977418536,21.0764356359779,-7.48823335804009));
#32593=CARTESIAN_POINT('Ctrl Pts',(-33.8333538619286,21.5671817964958,-9.12349227712162));
#32594=CARTESIAN_POINT('Ctrl Pts',(-36.2859962735183,22.8443778274084,-11.8775764776478));
#32595=CARTESIAN_POINT('Ctrl Pts',(-37.7273940527265,23.6269831007203,-12.9726927515238));
#32596=CARTESIAN_POINT('Ctrl Pts',(-40.906827527486,25.3653764194226,-14.4683433355124));
#32597=CARTESIAN_POINT('Ctrl Pts',(-42.5943534696917,26.3064386089228,-14.8498038985481));
#32598=CARTESIAN_POINT('Ctrl Pts',(-44.2988917118189,27.2516566664766,-14.8500516281495));
#32599=CARTESIAN_POINT('Ctrl Pts',(-31.1202396243797,21.567561713547,1.59674381934676));
#32600=CARTESIAN_POINT('Ctrl Pts',(-31.1224126652072,21.520989348265,1.15301435962634));
#32601=CARTESIAN_POINT('Ctrl Pts',(-31.1157607260923,21.4633832297208,0.635579189057524));
#32602=CARTESIAN_POINT('Ctrl Pts',(-31.2068426511149,21.320019509059,-1.86860431103819));
#32603=CARTESIAN_POINT('Ctrl Pts',(-31.5813261451172,21.4172046994746,-3.70979114470735));
#32604=CARTESIAN_POINT('Ctrl Pts',(-32.9219916749894,21.9749346552901,-7.17014261468839));
#32605=CARTESIAN_POINT('Ctrl Pts',(-33.871458674539,22.440710540688,-8.73670574473669));
#32606=CARTESIAN_POINT('Ctrl Pts',(-36.224903024249,23.6544622808092,-11.3734544105285));
#32607=CARTESIAN_POINT('Ctrl Pts',(-37.609369384537,24.3997952524124,-12.4221714958129));
#32608=CARTESIAN_POINT('Ctrl Pts',(-40.6575436657173,26.0548745077397,-13.8545909095728));
#32609=CARTESIAN_POINT('Ctrl Pts',(-42.2789313088166,26.9525808297997,-14.2195188100245));
#32610=CARTESIAN_POINT('Ctrl Pts',(-43.9126516878553,27.8526693689671,-14.2201291128084));
#32611=CARTESIAN_POINT('Ctrl Pts',(-29.2929893708797,23.9769478445538,1.59647090706387));
#32612=CARTESIAN_POINT('Ctrl Pts',(-29.3017711927823,23.9311433314971,1.15259179089162));
#32613=CARTESIAN_POINT('Ctrl Pts',(-29.3034887354907,23.8732845217124,0.635573104344381));
#32614=CARTESIAN_POINT('Ctrl Pts',(-29.4153831213449,23.7455006526433,-1.86858636183877));
#32615=CARTESIAN_POINT('Ctrl Pts',(-29.7701745938413,23.8932152177425,-3.71029995868823));
#32616=CARTESIAN_POINT('Ctrl Pts',(-31.0201080009748,24.6380470281508,-7.16936247494709));
#32617=CARTESIAN_POINT('Ctrl Pts',(-31.8922209971496,25.2329893514979,-8.73699595771819));
#32618=CARTESIAN_POINT('Ctrl Pts',(-34.04948266738,26.769756178971,-11.3730256982017));
#32619=CARTESIAN_POINT('Ctrl Pts',(-35.3129551733011,27.7038134838192,-12.4235805192756));
#32620=CARTESIAN_POINT('Ctrl Pts',(-38.0954870863618,29.7766493955002,-13.8529470821068));
#32621=CARTESIAN_POINT('Ctrl Pts',(-39.5719833475633,30.8954422364741,-14.2204718557262));
#32622=CARTESIAN_POINT('Ctrl Pts',(-41.0611748464153,32.0190184050857,-14.2198708430667));
#32623=CARTESIAN_POINT('Ctrl Pts',(-28.3497570418624,24.1050578112644,1.62964634867147));
#32624=CARTESIAN_POINT('Ctrl Pts',(-28.3584655992857,24.0596354334535,1.18947040156752));
#32625=CARTESIAN_POINT('Ctrl Pts',(-28.3595888789042,24.000772091711,0.66424406514856));
#32626=CARTESIAN_POINT('Ctrl Pts',(-28.4713886672159,23.8722870320852,-1.95287905133948));
#32627=CARTESIAN_POINT('Ctrl Pts',(-28.8382130746991,24.0314123848382,-3.87337387078001));
#32628=CARTESIAN_POINT('Ctrl Pts',(-30.1365118993193,24.8169940396349,-7.48792130214588));
#32629=CARTESIAN_POINT('Ctrl Pts',(-31.0433175237566,25.4427599558226,-9.12360836232668));
#32630=CARTESIAN_POINT('Ctrl Pts',(-33.2894343747244,27.0561790919793,-11.8774049927046));
#32631=CARTESIAN_POINT('Ctrl Pts',(-34.6044524432567,28.0356631207245,-12.973256360911));
#32632=CARTESIAN_POINT('Ctrl Pts',(-37.5044951006137,30.2091636815072,-14.4676858045239));
#32633=CARTESIAN_POINT('Ctrl Pts',(-39.0406651371294,31.3805975394391,-14.8501851005484));
#32634=CARTESIAN_POINT('Ctrl Pts',(-40.5934132658116,32.5588345556907,-14.8499483202528));
#32635=CARTESIAN_POINT('Ctrl Pts',(-27.7261998529423,24.8250414362346,1.62975553161125));
#32636=CARTESIAN_POINT('Ctrl Pts',(-27.7349072261382,24.7796252351385,1.18963944138304));
#32637=CARTESIAN_POINT('Ctrl Pts',(-27.7359890779435,24.720718840073,0.664246507217367));
#32638=CARTESIAN_POINT('Ctrl Pts',(-27.8472541630979,24.5917704575537,-1.95288623102729));
#32639=CARTESIAN_POINT('Ctrl Pts',(-28.2148983405374,24.751606201496,-3.87317034519134));
#32640=CARTESIAN_POINT('Ctrl Pts',(-29.5122822980333,25.536394999056,-7.48823335803871));
#32641=CARTESIAN_POINT('Ctrl Pts',(-30.4196491139021,26.1626472662679,-9.12349227714079));
#32642=CARTESIAN_POINT('Ctrl Pts',(-32.6655632155794,27.7758906912001,-11.8775764776286));
#32643=CARTESIAN_POINT('Ctrl Pts',(-33.9809133008013,28.7556624631466,-12.9726927515193));
#32644=CARTESIAN_POINT('Ctrl Pts',(-36.8805855631737,30.9288420051638,-14.4683433355169));
#32645=CARTESIAN_POINT('Ctrl Pts',(-38.4170078110451,32.1004855202031,-14.849803898529));
#32646=CARTESIAN_POINT('Ctrl Pts',(-39.9696777567512,33.2786637049092,-14.8500516281495));
#32647=CARTESIAN_POINT('Ctrl Pts',(-27.7340963985795,25.7769069069792,1.59674386441333));
#32648=CARTESIAN_POINT('Ctrl Pts',(-27.7428752599128,25.7311178357017,1.15301439043128));
#32649=CARTESIAN_POINT('Ctrl Pts',(-27.7444892330881,25.6731513926165,0.635579209516401));
#32650=CARTESIAN_POINT('Ctrl Pts',(-27.8550468610524,25.5442092163171,-1.8686043110583));
#32651=CARTESIAN_POINT('Ctrl Pts',(-28.2118877584287,25.6936997593906,-3.70979114471355));
#32652=CARTESIAN_POINT('Ctrl Pts',(-29.459533997768,26.4365494266998,-7.17014261468215));
#32653=CARTESIAN_POINT('Ctrl Pts',(-30.3330499725088,27.0327076276087,-8.73670574475106));
#32654=CARTESIAN_POINT('Ctrl Pts',(-32.4898047695223,28.5690351770253,-11.373454410514));
#32655=CARTESIAN_POINT('Ctrl Pts',(-33.7541073171722,29.5038118398731,-12.4221714958132));
#32656=CARTESIAN_POINT('Ctrl Pts',(-36.5357132427521,31.5758452046431,-13.8545909095725));
#32657=CARTESIAN_POINT('Ctrl Pts',(-38.0128405673296,32.6951616910819,-14.2195188099437));
#32658=CARTESIAN_POINT('Ctrl Pts',(-39.5018360737643,33.8185912781321,-14.2201291128084));
#32659=CARTESIAN_POINT('Ctrl Pts',(-29.331888309534,23.8408520862201,0.));
#32660=CARTESIAN_POINT('Ctrl Pts',(-29.4153831213449,23.7455006526433,-1.86858636183877));
#32661=CARTESIAN_POINT('Ctrl Pts',(-29.7701745938413,23.8932152177425,-3.71029995868823));
#32662=CARTESIAN_POINT('Ctrl Pts',(-31.0201080009748,24.6380470281508,-7.16936247494709));
#32663=CARTESIAN_POINT('Ctrl Pts',(-31.8922209971496,25.2329893514979,-8.73699595771819));
#32664=CARTESIAN_POINT('Ctrl Pts',(-33.0805753786004,26.0795364430711,-10.1890856763491));
#32665=CARTESIAN_POINT('Ctrl Pts',(-33.1922116559259,26.1594145048145,-10.3203928635157));
#32666=CARTESIAN_POINT('Ctrl Pts',(-33.3057006128448,26.2409403042404,-10.4488603765989));
#32667=CARTESIAN_POINT('Ctrl Pts',(-27.7725495286736,25.640424970686,5.55111512312578E-17));
#32668=CARTESIAN_POINT('Ctrl Pts',(-27.8550468610524,25.5442092163171,-1.8686043110583));
#32669=CARTESIAN_POINT('Ctrl Pts',(-28.2118877584287,25.6936997593906,-3.70979114471355));
#32670=CARTESIAN_POINT('Ctrl Pts',(-29.459533997768,26.4365494266998,-7.17014261468215));
#32671=CARTESIAN_POINT('Ctrl Pts',(-30.3330499725088,27.0327076276087,-8.73670574475106));
#32672=CARTESIAN_POINT('Ctrl Pts',(-31.5271893797574,27.8833324977795,-10.1966053555727));
#32673=CARTESIAN_POINT('Ctrl Pts',(-31.6450939272868,27.9677135840395,-10.335023194229));
#32674=CARTESIAN_POINT('Ctrl Pts',(-31.7650675024774,28.0539337918545,-10.4702558451016));
#32675=CARTESIAN_POINT('Ctrl Pts',(-35.7920133394053,26.6166303184858,1.24689105568334));
#32676=CARTESIAN_POINT('Ctrl Pts',(-35.8015619426389,26.5668264024534,0.764254809553763));
#32677=CARTESIAN_POINT('Ctrl Pts',(-35.8093225655934,26.5193322760963,0.332948724812664));
#32678=CARTESIAN_POINT('Ctrl Pts',(-35.9192508155956,26.396380965825,-0.978870002717184));
#32679=CARTESIAN_POINT('Ctrl Pts',(-36.151573194664,26.4275870969477,-1.98783577086484));
#32680=CARTESIAN_POINT('Ctrl Pts',(-36.885910263345,26.7378856583767,-3.80852727286012));
#32681=CARTESIAN_POINT('Ctrl Pts',(-37.394934824389,27.0101644118135,-4.65544360724195));
#32682=CARTESIAN_POINT('Ctrl Pts',(-38.6131565530345,27.7368493043946,-6.04997283341153));
#32683=CARTESIAN_POINT('Ctrl Pts',(-39.3343778781397,28.1929976956455,-6.61832169911591));
#32684=CARTESIAN_POINT('Ctrl Pts',(-40.8744649436646,29.2014824204577,-7.36768403070085));
#32685=CARTESIAN_POINT('Ctrl Pts',(-41.722421499192,29.7658228850063,-7.57138648695631));
#32686=CARTESIAN_POINT('Ctrl Pts',(-42.5403522177283,30.3120568904488,-7.56962581969436));
#32687=CARTESIAN_POINT('Ctrl Pts',(-33.4652890233053,26.1708926054255,1.35489343606331));
#32688=CARTESIAN_POINT('Ctrl Pts',(-33.4746002454611,26.1223268292986,0.884255668136539));
#32689=CARTESIAN_POINT('Ctrl Pts',(-33.4804735791531,26.0716101167974,0.426397017780271));
#32690=CARTESIAN_POINT('Ctrl Pts',(-33.5907346359763,25.9469288716972,-1.25360819503973));
#32691=CARTESIAN_POINT('Ctrl Pts',(-33.8612946673472,26.0144759562051,-2.51960912778176));
#32692=CARTESIAN_POINT('Ctrl Pts',(-34.7543728004411,26.4585467959166,-4.84647586783908));
#32693=CARTESIAN_POINT('Ctrl Pts',(-35.3758029321054,26.8307099768199,-5.91572199047857));
#32694=CARTESIAN_POINT('Ctrl Pts',(-36.8838857283486,27.8074490109549,-7.69376028690863));
#32695=CARTESIAN_POINT('Ctrl Pts',(-37.7727185143269,28.411317973868,-8.41063186563368));
#32696=CARTESIAN_POINT('Ctrl Pts',(-39.6962686996607,29.7482978093359,-9.37059840613264));
#32697=CARTESIAN_POINT('Ctrl Pts',(-40.7384561124906,30.4839404690763,-9.62435378635169));
#32698=CARTESIAN_POINT('Ctrl Pts',(-41.7636091770245,31.2084352127806,-9.62320046360546));
#32699=CARTESIAN_POINT('Ctrl Pts',(-31.2708363785844,25.2795805846979,1.47293214974068));
#32700=CARTESIAN_POINT('Ctrl Pts',(-31.2798886902769,25.2323652421878,1.01538106786831));
#32701=CARTESIAN_POINT('Ctrl Pts',(-31.2837215247332,25.1781488031011,0.528580803105061));
#32702=CARTESIAN_POINT('Ctrl Pts',(-31.3946464646314,25.0518358019868,-1.55402875461628));
#32703=CARTESIAN_POINT('Ctrl Pts',(-31.7065592633163,25.1587229846853,-3.1012143212269));
#32704=CARTESIAN_POINT('Ctrl Pts',(-32.7737330381668,25.7495178005034,-5.9812914545173));
#32705=CARTESIAN_POINT('Ctrl Pts',(-33.5177631757073,26.2306311757364,-7.29389406577215));
#32706=CARTESIAN_POINT('Ctrl Pts',(-35.3429210732647,27.4809015051985,-9.4911359380346));
#32707=CARTESIAN_POINT('Ctrl Pts',(-36.4148497431273,28.246140619147,-10.3708286017653));
#32708=CARTESIAN_POINT('Ctrl Pts',(-38.7579223667115,29.9425080008419,-11.560404556077));
#32709=CARTESIAN_POINT('Ctrl Pts',(-40.0123393655922,30.8653690604201,-11.8694761541998));
#32710=CARTESIAN_POINT('Ctrl Pts',(-41.2641519184871,31.7848057921741,-11.8687142284812));
#32711=CARTESIAN_POINT('Ctrl Pts',(-29.2929893708797,23.9769478445538,1.59647090706387));
#32712=CARTESIAN_POINT('Ctrl Pts',(-29.3017711927823,23.9311433314971,1.15259179089162));
#32713=CARTESIAN_POINT('Ctrl Pts',(-29.3034887354907,23.8732845217124,0.635573104344381));
#32714=CARTESIAN_POINT('Ctrl Pts',(-29.4153831213449,23.7455006526433,-1.86858636183877));
#32715=CARTESIAN_POINT('Ctrl Pts',(-29.7701745938413,23.8932152177425,-3.71029995868823));
#32716=CARTESIAN_POINT('Ctrl Pts',(-31.0201080009748,24.6380470281508,-7.16936247494709));
#32717=CARTESIAN_POINT('Ctrl Pts',(-31.8922209971496,25.2329893514979,-8.73699595771819));
#32718=CARTESIAN_POINT('Ctrl Pts',(-34.04948266738,26.769756178971,-11.3730256982017));
#32719=CARTESIAN_POINT('Ctrl Pts',(-35.3129551733011,27.7038134838192,-12.4235805192756));
#32720=CARTESIAN_POINT('Ctrl Pts',(-38.0954870863618,29.7766493955002,-13.8529470821068));
#32721=CARTESIAN_POINT('Ctrl Pts',(-39.5719833475633,30.8954422364741,-14.2204718557262));
#32722=CARTESIAN_POINT('Ctrl Pts',(-41.0611748464153,32.0190184050857,-14.2198708430667));
#32723=CARTESIAN_POINT('Ctrl Pts',(-27.7340963985795,25.7769069069792,1.59674386441333));
#32724=CARTESIAN_POINT('Ctrl Pts',(-27.7428752599097,25.7311178357017,1.15301439043125));
#32725=CARTESIAN_POINT('Ctrl Pts',(-27.7444892330881,25.6731513926165,0.635579209516401));
#32726=CARTESIAN_POINT('Ctrl Pts',(-27.8550468610524,25.5442092163171,-1.8686043110583));
#32727=CARTESIAN_POINT('Ctrl Pts',(-28.2118877584311,25.6936997593906,-3.70979114471235));
#32728=CARTESIAN_POINT('Ctrl Pts',(-29.4595339977656,26.4365494266998,-7.17014261468335));
#32729=CARTESIAN_POINT('Ctrl Pts',(-30.3330499725136,27.0327076276087,-8.73670574475107));
#32730=CARTESIAN_POINT('Ctrl Pts',(-32.4898047695175,28.5690351770252,-11.373454410514));
#32731=CARTESIAN_POINT('Ctrl Pts',(-33.7541073171722,29.5038118398683,-12.4221714958132));
#32732=CARTESIAN_POINT('Ctrl Pts',(-36.5357132427521,31.5758452046479,-13.8545909095725));
#32733=CARTESIAN_POINT('Ctrl Pts',(-38.0128405673159,32.6951616910965,-14.2195188099295));
#32734=CARTESIAN_POINT('Ctrl Pts',(-39.5018360737643,33.8185912781321,-14.2201291128084));
#32735=CARTESIAN_POINT('Ctrl Pts',(-29.3058064687038,27.5484813091701,1.47327622041476));
#32736=CARTESIAN_POINT('Ctrl Pts',(-29.314855048509,27.5012854314731,1.01591376687318));
#32737=CARTESIAN_POINT('Ctrl Pts',(-29.318557330564,27.4469333174803,0.528588498851873));
#32738=CARTESIAN_POINT('Ctrl Pts',(-29.4277972482719,27.3191602364301,-1.55405138012929));
#32739=CARTESIAN_POINT('Ctrl Pts',(-29.7422934066125,27.4282860909958,-3.10057294641829));
#32740=CARTESIAN_POINT('Ctrl Pts',(-30.8065841399506,28.016582357811,-5.98227484333453));
#32741=CARTESIAN_POINT('Ctrl Pts',(-31.5523827727639,28.4992283820582,-7.29352824389315));
#32742=CARTESIAN_POINT('Ctrl Pts',(-33.3769017419046,29.7489449887618,-9.49167634236451));
#32743=CARTESIAN_POINT('Ctrl Pts',(-34.4498767034895,30.5150908743752,-10.36905248673));
#32744=CARTESIAN_POINT('Ctrl Pts',(-36.7917820929404,32.2104466223681,-11.5624766483843));
#32745=CARTESIAN_POINT('Ctrl Pts',(-38.0469976785282,33.1339647666331,-11.8682745705308));
#32746=CARTESIAN_POINT('Ctrl Pts',(-39.2985600643046,34.0532197137072,-11.8690397849988));
#32747=CARTESIAN_POINT('Ctrl Pts',(-30.5013447592649,29.5931790826756,1.35541241355863));
#32748=CARTESIAN_POINT('Ctrl Pts',(-30.5106503524477,29.5446426662131,0.885059162349099));
#32749=CARTESIAN_POINT('Ctrl Pts',(-30.5163267679929,29.4937213090629,0.426408625626303));
#32750=CARTESIAN_POINT('Ctrl Pts',(-30.6240462289741,29.3668377587799,-1.25364232213325));
#32751=CARTESIAN_POINT('Ctrl Pts',(-30.8985028595643,29.4377615341981,-2.51864171289819));
#32752=CARTESIAN_POINT('Ctrl Pts',(-31.7872323696267,29.8780636984644,-4.84795915805562));
#32753=CARTESIAN_POINT('Ctrl Pts',(-32.4113300033956,30.2525386438001,-5.91517020464911));
#32754=CARTESIAN_POINT('Ctrl Pts',(-33.9184490747425,31.2284424726283,-7.69457540341378));
#32755=CARTESIAN_POINT('Ctrl Pts',(-34.8088600302747,31.8336791606204,-8.40795287028212));
#32756=CARTESIAN_POINT('Ctrl Pts',(-36.7306496230996,33.1691331028151,-9.37372383750715));
#32757=CARTESIAN_POINT('Ctrl Pts',(-37.7740480458323,33.9057602738446,-9.62254085996342));
#32758=CARTESIAN_POINT('Ctrl Pts',(-38.798817306756,34.6299874229481,-9.6236915153538));
#32759=CARTESIAN_POINT('Ctrl Pts',(-31.2747661069637,31.8324214200722,1.24768201173568));
#32760=CARTESIAN_POINT('Ctrl Pts',(-31.2843061312616,31.7826622501022,0.76547938791503));
#32761=CARTESIAN_POINT('Ctrl Pts',(-31.2917666379332,31.734856231766,0.332966415938288));
#32762=CARTESIAN_POINT('Ctrl Pts',(-31.3978213276601,31.6085484626272,-0.978922014666463));
#32763=CARTESIAN_POINT('Ctrl Pts',(-31.6360823818443,31.6449008941949,-1.98636136655456));
#32764=CARTESIAN_POINT('Ctrl Pts',(-32.3637918611878,31.9494557448061,-3.81078790532199));
#32765=CARTESIAN_POINT('Ctrl Pts',(-32.8768818719989,32.2252577802497,-4.6546026491141));
#32766=CARTESIAN_POINT('Ctrl Pts',(-34.0936348201201,32.9506697646595,-6.05121512491815));
#32767=CARTESIAN_POINT('Ctrl Pts',(-34.8172613800643,33.4089026594542,-6.61423873289649));
#32768=CARTESIAN_POINT('Ctrl Pts',(-36.3546651861043,34.4150618219321,-7.37244739496743));
#32769=CARTESIAN_POINT('Ctrl Pts',(-37.2044809779672,34.9808875866207,-7.56862230164793));
#32770=CARTESIAN_POINT('Ctrl Pts',(-38.0218131772948,35.5267289204026,-7.57037421506));
#32771=CARTESIAN_POINT('Ctrl Pts',(-25.5825535213022,27.901724132258,1.59647090706392));
#32772=CARTESIAN_POINT('Ctrl Pts',(-25.5977646187839,27.8576356266619,1.15259179090154));
#32773=CARTESIAN_POINT('Ctrl Pts',(-25.6076988465242,27.8006101679571,0.635573104329545));
#32774=CARTESIAN_POINT('Ctrl Pts',(-25.7366398496131,27.6900511858226,-1.86858636179538));
#32775=CARTESIAN_POINT('Ctrl Pts',(-26.0667980818804,27.8867543207442,-3.71029995871436));
#32776=CARTESIAN_POINT('Ctrl Pts',(-27.1980083507482,28.8018888878555,-7.16936247492051));
#32777=CARTESIAN_POINT('Ctrl Pts',(-27.9765753733663,29.5148901762992,-8.73699595772989));
#32778=CARTESIAN_POINT('Ctrl Pts',(-29.8931745080091,31.3430252789184,-11.3730256981895));
#32779=CARTESIAN_POINT('Ctrl Pts',(-31.0108564712645,32.4473861125716,-12.4235805192514));
#32780=CARTESIAN_POINT('Ctrl Pts',(-33.470070913885,34.8951191226966,-13.8529470821305));
#32781=CARTESIAN_POINT('Ctrl Pts',(-34.7723177498354,36.2126515924125,-14.2204718557451));
#32782=CARTESIAN_POINT('Ctrl Pts',(-36.086449865815,37.5367254229123,-14.2198708430665));
#32783=CARTESIAN_POINT('Ctrl Pts',(-24.6306899881719,27.8942941678687,1.62964634867149));
#32784=CARTESIAN_POINT('Ctrl Pts',(-24.645774183387,27.8505734813085,1.18947040157924));
#32785=CARTESIAN_POINT('Ctrl Pts',(-24.6552631565805,27.7924691428847,0.664244065130957));
#32786=CARTESIAN_POINT('Ctrl Pts',(-24.7842103148136,27.6812026446449,-1.95287905128799));
#32787=CARTESIAN_POINT('Ctrl Pts',(-25.1246550797452,27.8909128870965,-3.87337387080019));
#32788=CARTESIAN_POINT('Ctrl Pts',(-26.2979391683636,28.8532656404492,-7.48792130212534));
#32789=CARTESIAN_POINT('Ctrl Pts',(-27.1064590436759,29.6017140578355,-9.12360836232651));
#32790=CARTESIAN_POINT('Ctrl Pts',(-29.1001001805409,31.5183666697857,-11.8774049927045));
#32791=CARTESIAN_POINT('Ctrl Pts',(-30.2623381500346,32.6750275472119,-12.9732563608965));
#32792=CARTESIAN_POINT('Ctrl Pts',(-32.8235411737415,35.2391241080399,-14.4676858045382));
#32793=CARTESIAN_POINT('Ctrl Pts',(-34.1773627942051,36.6172542487414,-14.8501851005579));
#32794=CARTESIAN_POINT('Ctrl Pts',(-35.5466255754748,38.0044776097606,-14.8499483202527));
#32795=CARTESIAN_POINT('Ctrl Pts',(-23.9110153591928,28.518207957172,1.6297555316112));
#32796=CARTESIAN_POINT('Ctrl Pts',(-23.9260975032013,28.4744932159134,1.18963944139604));
#32797=CARTESIAN_POINT('Ctrl Pts',(-23.9355515973827,28.4163403666075,0.664246507199459));
#32798=CARTESIAN_POINT('Ctrl Pts',(-24.0640354326714,28.3045391652296,-1.95288623097488));
#32799=CARTESIAN_POINT('Ctrl Pts',(-24.4051905243015,28.5150692335709,-3.87317034520081));
#32800=CARTESIAN_POINT('Ctrl Pts',(-25.5776818931472,29.4765070006193,-7.48823335802904));
#32801=CARTESIAN_POINT('Ctrl Pts',(-26.3866880328324,30.225516684584,-9.12349227712161));
#32802=CARTESIAN_POINT('Ctrl Pts',(-28.3801534903862,32.1419665195312,-11.8775764776477));
#32803=CARTESIAN_POINT('Ctrl Pts',(-29.5426791470118,33.2989594622607,-12.9726927515242));
#32804=CARTESIAN_POINT('Ctrl Pts',(-32.103561231544,35.8626855591394,-14.4683433355121));
#32805=CARTESIAN_POINT('Ctrl Pts',(-33.4576026588981,37.2410591163594,-14.8498038984863));
#32806=CARTESIAN_POINT('Ctrl Pts',(-34.8267964255889,38.6282131180508,-14.8500516281496));
#32807=CARTESIAN_POINT('Ctrl Pts',(-23.7833669488544,29.4615086055164,1.59674386441321));
#32808=CARTESIAN_POINT('Ctrl Pts',(-23.7985729183198,29.4174349631855,1.15301439044218));
#32809=CARTESIAN_POINT('Ctrl Pts',(-23.8084199485281,29.3602882272665,0.635579209500779));
#32810=CARTESIAN_POINT('Ctrl Pts',(-23.9362026442624,29.2483924872771,-1.86860431101262));
#32811=CARTESIAN_POINT('Ctrl Pts',(-24.2681366932807,29.4471451869314,-3.70979114471473));
#32812=CARTESIAN_POINT('Ctrl Pts',(-25.3973651626975,30.3599922882794,-7.17014261468097));
#32813=CARTESIAN_POINT('Ctrl Pts',(-26.1771478462482,31.0743967431656,-8.73670574471763));
#32814=CARTESIAN_POINT('Ctrl Pts',(-28.0933077826319,32.9020249032871,-11.3734544105476));
#32815=CARTESIAN_POINT('Ctrl Pts',(-29.2117089637015,34.0072159001959,-12.422171495823));
#32816=CARTESIAN_POINT('Ctrl Pts',(-31.6701210583974,36.4540227504429,-13.854590909563));
#32817=CARTESIAN_POINT('Ctrl Pts',(-32.972918011878,37.7721633453382,-14.2195188099105));
#32818=CARTESIAN_POINT('Ctrl Pts',(-34.2868769911003,39.0960641936379,-14.2201291128085));
#32819=CARTESIAN_POINT('Ctrl Pts',(-25.6404249706857,27.7725495286739,1.04083408558608E-14));
#32820=CARTESIAN_POINT('Ctrl Pts',(-25.7366398496132,27.6900511858226,-1.86858636179538));
#32821=CARTESIAN_POINT('Ctrl Pts',(-26.0667980818804,27.8867543207442,-3.71029995871436));
#32822=CARTESIAN_POINT('Ctrl Pts',(-27.1980083507482,28.8018888878555,-7.16936247492051));
#32823=CARTESIAN_POINT('Ctrl Pts',(-27.9765753733639,29.5148901762992,-8.7369959577275));
#32824=CARTESIAN_POINT('Ctrl Pts',(-29.03235780837,30.5219411006535,-10.1890856763466));
#32825=CARTESIAN_POINT('Ctrl Pts',(-29.1314899559286,30.616893617651,-10.320392863511));
#32826=CARTESIAN_POINT('Ctrl Pts',(-29.2322214279503,30.7137407645344,-10.448860376592));
#32827=CARTESIAN_POINT('Ctrl Pts',(-23.8408520862198,29.3318883095343,-8.88178419700125E-16));
#32828=CARTESIAN_POINT('Ctrl Pts',(-23.9362026442624,29.2483924872771,-1.86860431101262));
#32829=CARTESIAN_POINT('Ctrl Pts',(-24.2681366932807,29.4471451869314,-3.70979114471473));
#32830=CARTESIAN_POINT('Ctrl Pts',(-25.3973651626975,30.3599922882794,-7.17014261468097));
#32831=CARTESIAN_POINT('Ctrl Pts',(-26.1771478462482,31.0743967431656,-8.73670574471763));
#32832=CARTESIAN_POINT('Ctrl Pts',(-27.2380760953908,32.0863072351785,-10.1966053555756));
#32833=CARTESIAN_POINT('Ctrl Pts',(-27.3427718639926,32.1866090102528,-10.335023194234));
#32834=CARTESIAN_POINT('Ctrl Pts',(-27.4492538662495,32.2890256406149,-10.4702558451083));
#32835=CARTESIAN_POINT('Ctrl Pts',(-31.6397608122766,31.4394459897279,1.24689105568327));
#32836=CARTESIAN_POINT('Ctrl Pts',(-31.6563000607263,31.3915079136632,0.764254809546443));
#32837=CARTESIAN_POINT('Ctrl Pts',(-31.6707408106672,31.3456016608171,0.332948724825213));
#32838=CARTESIAN_POINT('Ctrl Pts',(-31.7970479454232,31.239546238828,-0.978870002754192));
#32839=CARTESIAN_POINT('Ctrl Pts',(-32.0225645221741,31.3034976581128,-1.98783577088618));
#32840=CARTESIAN_POINT('Ctrl Pts',(-32.7052670086903,31.7151448890596,-3.80852727283832));
#32841=CARTESIAN_POINT('Ctrl Pts',(-33.1703611269162,32.0570939851866,-4.65544360728939));
#32842=CARTESIAN_POINT('Ctrl Pts',(-34.2727650719352,32.9497533019061,-6.0499728333633));
#32843=CARTESIAN_POINT('Ctrl Pts',(-34.9217287193182,33.5038992564081,-6.61832169905306));
#32844=CARTESIAN_POINT('Ctrl Pts',(-36.3026175786583,34.7212963023931,-7.36768403076268));
#32845=CARTESIAN_POINT('Ctrl Pts',(-37.0616291372176,35.400569394778,-7.57138648706064));
#32846=CARTESIAN_POINT('Ctrl Pts',(-37.7934972961794,36.0576472036357,-7.56962581969389));
#32847=CARTESIAN_POINT('Ctrl Pts',(-29.4001542854016,30.6671178491337,1.35489343606325));
#32848=CARTESIAN_POINT('Ctrl Pts',(-29.4162823633,30.6203715276532,0.884255668134132));
#32849=CARTESIAN_POINT('Ctrl Pts',(-29.4293136556726,30.5710069006836,0.426397017784211));
#32850=CARTESIAN_POINT('Ctrl Pts',(-29.5561964051726,30.4632865154017,-1.25360819505145));
#32851=CARTESIAN_POINT('Ctrl Pts',(-29.814389573106,30.5686507749802,-2.51960912780314));
#32852=CARTESIAN_POINT('Ctrl Pts',(-30.6351795888044,31.1352998840684,-4.84647586781734));
#32853=CARTESIAN_POINT('Ctrl Pts',(-31.1973201148198,31.5921137089528,-5.91572199050937));
#32854=CARTESIAN_POINT('Ctrl Pts',(-32.551048345043,32.7735335074371,-7.69376028687725));
#32855=CARTESIAN_POINT('Ctrl Pts',(-33.3448945810382,33.4977500491683,-8.41063186559017));
#32856=CARTESIAN_POINT('Ctrl Pts',(-35.0585937299434,35.0948710911578,-9.37059840617546));
#32857=CARTESIAN_POINT('Ctrl Pts',(-35.9854803115198,35.9713447024496,-9.62435378640853));
#32858=CARTESIAN_POINT('Ctrl Pts',(-36.8970924436849,36.8343596268991,-9.62320046360515));
#32859=CARTESIAN_POINT('Ctrl Pts',(-27.3548849305453,29.4725749263795,1.47293214974066));
#32860=CARTESIAN_POINT('Ctrl Pts',(-27.3705645465822,29.4271284462505,1.01538106787189));
#32861=CARTESIAN_POINT('Ctrl Pts',(-27.3820741720672,29.3740093215552,0.52858080309974));
#32862=CARTESIAN_POINT('Ctrl Pts',(-27.5098462703896,29.2647682695534,-1.55402875460085));
#32863=CARTESIAN_POINT('Ctrl Pts',(-27.8033726143254,29.4149573143428,-3.10121432124709));
#32864=CARTESIAN_POINT('Ctrl Pts',(-28.7756052303118,30.1516133539741,-5.98129145449675));
#32865=CARTESIAN_POINT('Ctrl Pts',(-29.4435926415566,30.733716217446,-7.29389406578866));
#32866=CARTESIAN_POINT('Ctrl Pts',(-31.0722410437714,32.2310076487118,-9.49113593801764));
#32867=CARTESIAN_POINT('Ctrl Pts',(-32.0243541445899,33.1410090871553,-10.370828601741));
#32868=CARTESIAN_POINT('Ctrl Pts',(-34.1021594176632,35.1535638963511,-11.5604045561007));
#32869=CARTESIAN_POINT('Ctrl Pts',(-35.212471437781,36.2455537133643,-11.869476154252));
#32870=CARTESIAN_POINT('Ctrl Pts',(-36.3206928540897,37.3337834058788,-11.868714228481));
#32871=CARTESIAN_POINT('Ctrl Pts',(-25.5825535213022,27.901724132258,1.59647090706392));
#32872=CARTESIAN_POINT('Ctrl Pts',(-25.5977646187839,27.8576356266619,1.15259179090154));
#32873=CARTESIAN_POINT('Ctrl Pts',(-25.6076988465242,27.8006101679571,0.635573104329545));
#32874=CARTESIAN_POINT('Ctrl Pts',(-25.7366398496132,27.6900511858226,-1.86858636179538));
#32875=CARTESIAN_POINT('Ctrl Pts',(-26.0667980818804,27.8867543207442,-3.71029995871436));
#32876=CARTESIAN_POINT('Ctrl Pts',(-27.1980083507482,28.8018888878555,-7.16936247492051));
#32877=CARTESIAN_POINT('Ctrl Pts',(-27.9765753733639,29.5148901762992,-8.7369959577275));
#32878=CARTESIAN_POINT('Ctrl Pts',(-29.8931745080115,31.3430252789184,-11.3730256981919));
#32879=CARTESIAN_POINT('Ctrl Pts',(-31.0108564712693,32.4473861125668,-12.4235805192514));
#32880=CARTESIAN_POINT('Ctrl Pts',(-33.4700709138802,34.8951191227014,-13.8529470821305));
#32881=CARTESIAN_POINT('Ctrl Pts',(-34.7723177498282,36.2126515924196,-14.2204718557498));
#32882=CARTESIAN_POINT('Ctrl Pts',(-36.086449865815,37.5367254229123,-14.2198708430665));
#32883=CARTESIAN_POINT('Ctrl Pts',(-23.7833669488544,29.4615086055164,1.59674386441321));
#32884=CARTESIAN_POINT('Ctrl Pts',(-23.7985729183197,29.4174349631855,1.15301439044218));
#32885=CARTESIAN_POINT('Ctrl Pts',(-23.8084199485281,29.3602882272665,0.635579209500779));
#32886=CARTESIAN_POINT('Ctrl Pts',(-23.9362026442624,29.2483924872771,-1.86860431101262));
#32887=CARTESIAN_POINT('Ctrl Pts',(-24.2681366932831,29.4471451869314,-3.70979114471473));
#32888=CARTESIAN_POINT('Ctrl Pts',(-25.3973651626951,30.3599922882794,-7.17014261468097));
#32889=CARTESIAN_POINT('Ctrl Pts',(-26.1771478462457,31.0743967431704,-8.73670574471765));
#32890=CARTESIAN_POINT('Ctrl Pts',(-28.0933077826343,32.9020249032823,-11.3734544105476));
#32891=CARTESIAN_POINT('Ctrl Pts',(-29.2117089636991,34.0072159001958,-12.4221714958182));
#32892=CARTESIAN_POINT('Ctrl Pts',(-31.6701210583998,36.4540227504429,-13.8545909095678));
#32893=CARTESIAN_POINT('Ctrl Pts',(-32.972918011877,37.7721633453374,-14.2195188099153));
#32894=CARTESIAN_POINT('Ctrl Pts',(-34.2868769911003,39.0960641936379,-14.2201291128086));
#32895=CARTESIAN_POINT('Ctrl Pts',(-25.0869579521468,31.4387285991345,1.47327622041453));
#32896=CARTESIAN_POINT('Ctrl Pts',(-25.1026311041719,31.3933008545835,1.0159137668782));
#32897=CARTESIAN_POINT('Ctrl Pts',(-25.1140308146307,31.3400288564346,0.528588498845575));
#32898=CARTESIAN_POINT('Ctrl Pts',(-25.2403428328608,31.2291027822935,-1.55405138011097));
#32899=CARTESIAN_POINT('Ctrl Pts',(-25.536107645434,31.3818753630146,-3.10057294640638));
#32900=CARTESIAN_POINT('Ctrl Pts',(-26.5058421456017,32.1156479855494,-5.98227484334664));
#32901=CARTESIAN_POINT('Ctrl Pts',(-27.1753619327859,32.6995195811097,-7.29352824385025));
#32902=CARTESIAN_POINT('Ctrl Pts',(-28.8034567128381,34.1961719966305,-9.49167634240776));
#32903=CARTESIAN_POINT('Ctrl Pts',(-29.7564764086048,35.1072198799865,-10.3690524867446));
#32904=CARTESIAN_POINT('Ctrl Pts',(-31.8332702988131,37.1186072377306,-11.5624766483702));
#32905=CARTESIAN_POINT('Ctrl Pts',(-32.9442792642516,38.2113611019873,-11.8682745704738));
#32906=CARTESIAN_POINT('Ctrl Pts',(-34.0522789304537,39.2993752576343,-11.869039784999));
#32907=CARTESIAN_POINT('Ctrl Pts',(-25.9793365537798,33.6327571359871,1.35541241355826));
#32908=CARTESIAN_POINT('Ctrl Pts',(-25.9954548817196,33.5860390742308,0.885059162349419));
#32909=CARTESIAN_POINT('Ctrl Pts',(-26.0083203842389,33.5364438612578,0.426408625628756));
#32910=CARTESIAN_POINT('Ctrl Pts',(-26.1330008283201,33.4261818802138,-1.25364232214062));
#32911=CARTESIAN_POINT('Ctrl Pts',(-26.3945703806265,33.5354430048991,-2.51864171287205));
#32912=CARTESIAN_POINT('Ctrl Pts',(-27.2115923742643,34.0977429244363,-4.84795915808225));
#32913=CARTESIAN_POINT('Ctrl Pts',(-27.7760442528266,34.5572246086334,-5.91517020458963));
#32914=CARTESIAN_POINT('Ctrl Pts',(-29.1289374294719,35.7376805504921,-7.69457540347394));
#32915=CARTESIAN_POINT('Ctrl Pts',(-29.9241511239976,36.4634754928399,-8.40795287031606));
#32916=CARTESIAN_POINT('Ctrl Pts',(-31.6363247579804,38.0588356145396,-9.37372383747396));
#32917=CARTESIAN_POINT('Ctrl Pts',(-32.5642699125256,38.9364560608696,-9.62254085990179));
#32918=CARTESIAN_POINT('Ctrl Pts',(-33.4755402303454,39.7991514935069,-9.62369151535411));
#32919=CARTESIAN_POINT('Ctrl Pts',(-26.4262081762393,35.9592765491247,1.24768201173514));
#32920=CARTESIAN_POINT('Ctrl Pts',(-26.4427325651026,35.9113815427634,0.765479387909697));
#32921=CARTESIAN_POINT('Ctrl Pts',(-26.4569206403356,35.8651238615744,0.332966415948582));
#32922=CARTESIAN_POINT('Ctrl Pts',(-26.5798713158797,35.7551948794183,-0.978922014696859));
#32923=CARTESIAN_POINT('Ctrl Pts',(-26.8105337258744,35.8250853790548,-1.98636136650463));
#32924=CARTESIAN_POINT('Ctrl Pts',(-27.4874934973876,36.2301041572591,-3.81078790537277));
#32925=CARTESIAN_POINT('Ctrl Pts',(-27.9561102698756,36.5761192475661,-4.65460264902373));
#32926=CARTESIAN_POINT('Ctrl Pts',(-29.0572415379625,37.4673095829807,-6.05121512500961));
#32927=CARTESIAN_POINT('Ctrl Pts',(-29.7082892826565,38.0238611245015,-6.61423873294022));
#32928=CARTESIAN_POINT('Ctrl Pts',(-31.0868531562901,39.2385744114085,-7.37244739492485));
#32929=CARTESIAN_POINT('Ctrl Pts',(-31.8474936465763,39.9195822825963,-7.56862230155307));
#32930=CARTESIAN_POINT('Ctrl Pts',(-32.5788252613913,40.5761862384901,-7.57037421506044));
#32931=CARTESIAN_POINT('Ctrl Pts',(-21.3513306581892,31.2585017743465,1.59647086199749));
#32932=CARTESIAN_POINT('Ctrl Pts',(-21.372661376489,31.2170267923784,1.15259176011709));
#32933=CARTESIAN_POINT('Ctrl Pts',(-21.390610056738,31.1619955607677,0.635573083859853));
#32934=CARTESIAN_POINT('Ctrl Pts',(-21.5339728088269,31.0709121284019,-1.86858636174266));
#32935=CARTESIAN_POINT('Ctrl Pts',(-21.8327767314457,31.3125995244709,-3.7102999587274));
#32936=CARTESIAN_POINT('Ctrl Pts',(-22.822235683043,32.3794073476566,-7.16936247490758));
#32937=CARTESIAN_POINT('Ctrl Pts',(-23.4914073530992,33.1959529508684,-8.73699595766537));
#32938=CARTESIAN_POINT('Ctrl Pts',(-25.1283275201135,35.2782407701667,-11.3730256982543));
#32939=CARTESIAN_POINT('Ctrl Pts',(-26.0774661594562,36.5304235305538,-12.4235805192081));
#32940=CARTESIAN_POINT('Ctrl Pts',(-28.1633006172565,39.303224853823,-13.8529470821741));
#32941=CARTESIAN_POINT('Ctrl Pts',(-29.2647880382077,40.7926757902301,-14.2204718556168));
#32942=CARTESIAN_POINT('Ctrl Pts',(-30.377108830674,42.2902929581066,-14.2198708430667));
#32943=CARTESIAN_POINT('Ctrl Pts',(-20.4102131175328,31.1156831315057,1.62964630360509));
#32944=CARTESIAN_POINT('Ctrl Pts',(-20.4313658791504,31.0745541646192,1.18947037066851));
#32945=CARTESIAN_POINT('Ctrl Pts',(-20.4490273774855,31.0183916684046,0.664244043741713));
#32946=CARTESIAN_POINT('Ctrl Pts',(-20.592496912111,30.9266087974082,-1.95287905124417));
#32947=CARTESIAN_POINT('Ctrl Pts',(-20.8996315609143,31.1826348336499,-3.87337387081084));
#32948=CARTESIAN_POINT('Ctrl Pts',(-21.9240162329082,32.3021679588473,-7.48792130211473));
#32949=CARTESIAN_POINT('Ctrl Pts',(-22.6177912263983,33.1580626256957,-9.12360836229304));
#32950=CARTESIAN_POINT('Ctrl Pts',(-24.3183718640796,35.33893119389,-11.8774049927381));
#32951=CARTESIAN_POINT('Ctrl Pts',(-25.3041699215151,36.6492226397706,-12.9732563608771));
#32952=CARTESIAN_POINT('Ctrl Pts',(-27.4743946037862,39.5517175890428,-14.4676858045577));
#32953=CARTESIAN_POINT('Ctrl Pts',(-28.6183079046236,41.1084892565677,-14.8501851004866));
#32954=CARTESIAN_POINT('Ctrl Pts',(-29.7762110964237,42.67645909556,-14.8499483202528));
#32955=CARTESIAN_POINT('Ctrl Pts',(-19.6090715485703,31.6308259996108,1.62975548654486));
#32956=CARTESIAN_POINT('Ctrl Pts',(-19.6302214337532,31.5897026256002,1.18963941047576));
#32957=CARTESIAN_POINT('Ctrl Pts',(-19.6478553119118,31.5334871484633,0.664246485816154));
#32958=CARTESIAN_POINT('Ctrl Pts',(-19.7909423357445,31.4411090791072,-1.95288623094877));
#32959=CARTESIAN_POINT('Ctrl Pts',(-20.0986634077675,31.6980476866425,-3.87317034520541));
#32960=CARTESIAN_POINT('Ctrl Pts',(-21.12239364484,32.8165623229556,-7.48823335802438));
#32961=CARTESIAN_POINT('Ctrl Pts',(-21.816570076654,33.6730817461045,-9.12349227713351));
#32962=CARTESIAN_POINT('Ctrl Pts',(-23.5170056814165,35.8537245995938,-11.8775764776358));
#32963=CARTESIAN_POINT('Ctrl Pts',(-24.5030412398847,37.1643856729197,-12.9726927515334));
#32964=CARTESIAN_POINT('Ctrl Pts',(-26.6730009722203,40.0664682546505,-14.4683433355028));
#32965=CARTESIAN_POINT('Ctrl Pts',(-27.8170972008357,41.6235121428184,-14.849803898548));
#32966=CARTESIAN_POINT('Ctrl Pts',(-28.9749419513881,43.1914035066778,-14.8500516281495));
#32967=CARTESIAN_POINT('Ctrl Pts',(-19.3484767357831,32.5463589446091,1.59674381934693));
#32968=CARTESIAN_POINT('Ctrl Pts',(-19.3698002629981,32.5048979448427,1.15301435963395));
#32969=CARTESIAN_POINT('Ctrl Pts',(-19.3876798928005,32.4497342609156,0.635579189045957));
#32970=CARTESIAN_POINT('Ctrl Pts',(-19.5300863679201,32.3571628326458,-1.86860431100416));
#32971=CARTESIAN_POINT('Ctrl Pts',(-19.8303563485812,32.6011316569382,-3.70979114471325));
#32972=CARTESIAN_POINT('Ctrl Pts',(-20.8181792128701,33.6653932579417,-7.1701426146823));
#32973=CARTESIAN_POINT('Ctrl Pts',(-21.4883544787337,34.4835007519095,-8.73670574476775));
#32974=CARTESIAN_POINT('Ctrl Pts',(-23.1249120634605,36.565224284407,-11.3734544104973));
#32975=CARTESIAN_POINT('Ctrl Pts',(-24.074644455379,37.8183311134267,-12.4221714958561));
#32976=CARTESIAN_POINT('Ctrl Pts',(-26.1598165383431,40.5901015178423,-13.8545909095296));
#32977=CARTESIAN_POINT('Ctrl Pts',(-27.261761932141,42.0802326794198,-14.2195188100388));
#32978=CARTESIAN_POINT('Ctrl Pts',(-28.373935968085,43.577653985901,-14.2201291128083));
#32979=CARTESIAN_POINT('Ctrl Pts',(-21.4269965203139,31.138877952143,0.));
#32980=CARTESIAN_POINT('Ctrl Pts',(-21.5339728088269,31.0709121284019,-1.86858636174266));
#32981=CARTESIAN_POINT('Ctrl Pts',(-21.8327767314481,31.3125995244709,-3.7102999587262));
#32982=CARTESIAN_POINT('Ctrl Pts',(-22.8222356830406,32.3794073476566,-7.16936247490878));
#32983=CARTESIAN_POINT('Ctrl Pts',(-23.4914073530968,33.1959529508732,-8.73699595766537));
#32984=CARTESIAN_POINT('Ctrl Pts',(-24.3931251555334,34.3430070554536,-10.1890856763534));
#32985=CARTESIAN_POINT('Ctrl Pts',(-24.4777351286485,34.4511010682924,-10.3203928635226));
#32986=CARTESIAN_POINT('Ctrl Pts',(-24.5636585134689,34.561298034017,-10.4488603766072));
#32987=CARTESIAN_POINT('Ctrl Pts',(-19.4238236466307,32.4262389885814,1.66533453693773E-15));
#32988=CARTESIAN_POINT('Ctrl Pts',(-19.5300863679201,32.3571628326458,-1.86860431100416));
#32989=CARTESIAN_POINT('Ctrl Pts',(-19.8303563485812,32.6011316569382,-3.70979114471325));
#32990=CARTESIAN_POINT('Ctrl Pts',(-20.8181792128701,33.6653932579417,-7.1701426146823));
#32991=CARTESIAN_POINT('Ctrl Pts',(-21.4883544787337,34.4835007519095,-8.73670574476775));
#32992=CARTESIAN_POINT('Ctrl Pts',(-22.3944741298215,35.6360972865697,-10.1966053555694));
#32993=CARTESIAN_POINT('Ctrl Pts',(-22.4838298155454,35.7502778955871,-10.3350231942233));
#32994=CARTESIAN_POINT('Ctrl Pts',(-22.5746525783571,35.8668060412641,-10.4702558450944));
#32995=CARTESIAN_POINT('Ctrl Pts',(-26.8434139987113,35.6222452002841,1.24689101061693));
#32996=CARTESIAN_POINT('Ctrl Pts',(-26.8666072002651,35.5771488466243,0.764254780049933));
#32997=CARTESIAN_POINT('Ctrl Pts',(-26.8874341048571,35.5337649882881,0.332948714094922));
#32998=CARTESIAN_POINT('Ctrl Pts',(-27.0275488741897,35.4467644377494,-0.978870002705638));
#32999=CARTESIAN_POINT('Ctrl Pts',(-27.2416687814551,35.5421592788662,-1.98783577089888));
#33000=CARTESIAN_POINT('Ctrl Pts',(-27.8588388319486,36.0467752286497,-3.808527272826));
#33001=CARTESIAN_POINT('Ctrl Pts',(-28.2705345322819,36.4514335704433,-4.65544360715088));
#33002=CARTESIAN_POINT('Ctrl Pts',(-29.2346789285044,37.491895341034,-6.04997283350233));
#33003=CARTESIAN_POINT('Ctrl Pts',(-29.7981738696684,38.1327580456143,-6.61832169894778));
#33004=CARTESIAN_POINT('Ctrl Pts',(-30.991753607908,39.5342847195234,-7.36768403086871));
#33005=CARTESIAN_POINT('Ctrl Pts',(-31.6463688825656,40.3146623988252,-7.57138648666127));
#33006=CARTESIAN_POINT('Ctrl Pts',(-32.2772757571273,41.069207801424,-7.56962581969451));
#33007=CARTESIAN_POINT('Ctrl Pts',(-24.7365171914565,34.5390490058877,1.35489339099691));
#33008=CARTESIAN_POINT('Ctrl Pts',(-24.7591338032395,34.4950737607633,0.884255638235833));
#33009=CARTESIAN_POINT('Ctrl Pts',(-24.7790577744533,34.4480661428601,0.426397004049554));
#33010=CARTESIAN_POINT('Ctrl Pts',(-24.9199792485702,34.3594994944943,-1.25360819501069));
#33011=CARTESIAN_POINT('Ctrl Pts',(-25.1605494847682,34.5005360167157,-2.51960912781112));
#33012=CARTESIAN_POINT('Ctrl Pts',(-25.8923424652897,35.1782280533404,-4.8464758678096));
#33013=CARTESIAN_POINT('Ctrl Pts',(-26.3837498256845,35.7103931102928,-5.91572199041384));
#33014=CARTESIAN_POINT('Ctrl Pts',(-27.555565486858,37.0724433725846,-7.69376028697315));
#33015=CARTESIAN_POINT('Ctrl Pts',(-28.2382647527903,37.9022645330053,-8.41063186551349));
#33016=CARTESIAN_POINT('Ctrl Pts',(-29.7072268925448,39.7270140028106,-9.37059840625263));
#33017=CARTESIAN_POINT('Ctrl Pts',(-30.4999439048329,40.7264760905819,-9.62435378612815));
#33018=CARTESIAN_POINT('Ctrl Pts',(-31.2794573106202,41.7104427005355,-9.62320046360557));
#33019=CARTESIAN_POINT('Ctrl Pts',(-22.8820669124602,33.0655926302368,1.47293210467429));
#33020=CARTESIAN_POINT('Ctrl Pts',(-22.9040546403785,33.0228401731316,1.01538103753903));
#33021=CARTESIAN_POINT('Ctrl Pts',(-22.9230067538105,32.9718997171349,0.52858078607649));
#33022=CARTESIAN_POINT('Ctrl Pts',(-23.0650249378946,32.8819544477773,-1.55402875455868));
#33023=CARTESIAN_POINT('Ctrl Pts',(-23.3341894772259,33.0723879387897,-3.10121432125518));
#33024=CARTESIAN_POINT('Ctrl Pts',(-24.1916890819461,33.9399090096535,-5.9812914544888));
#33025=CARTESIAN_POINT('Ctrl Pts',(-24.7700354697141,34.6111514256874,-7.29389406572176));
#33026=CARTESIAN_POINT('Ctrl Pts',(-26.1690197913893,36.3249834230483,-9.49113593808477));
#33027=CARTESIAN_POINT('Ctrl Pts',(-26.981935046293,37.3612221809014,-10.370828601693));
#33028=CARTESIAN_POINT('Ctrl Pts',(-28.7521748453643,39.6489946054638,-11.5604045561491));
#33029=CARTESIAN_POINT('Ctrl Pts',(-29.6957791360119,40.8878834161158,-11.8694761540572));
#33030=CARTESIAN_POINT('Ctrl Pts',(-30.6378492234119,42.122752851181,-11.8687142284813));
#33031=CARTESIAN_POINT('Ctrl Pts',(-21.3513306581892,31.2585017743465,1.59647086199749));
#33032=CARTESIAN_POINT('Ctrl Pts',(-21.372661376489,31.2170267923722,1.15259176011769));
#33033=CARTESIAN_POINT('Ctrl Pts',(-21.390610056738,31.1619955607677,0.635573083859853));
#33034=CARTESIAN_POINT('Ctrl Pts',(-21.5339728088269,31.0709121284019,-1.86858636174266));
#33035=CARTESIAN_POINT('Ctrl Pts',(-21.8327767314481,31.3125995244709,-3.7102999587262));
#33036=CARTESIAN_POINT('Ctrl Pts',(-22.8222356830406,32.3794073476566,-7.16936247490878));
#33037=CARTESIAN_POINT('Ctrl Pts',(-23.4914073530968,33.1959529508732,-8.73699595766537));
#33038=CARTESIAN_POINT('Ctrl Pts',(-25.1283275201159,35.2782407701619,-11.3730256982543));
#33039=CARTESIAN_POINT('Ctrl Pts',(-26.0774661594586,36.5304235305538,-12.4235805192081));
#33040=CARTESIAN_POINT('Ctrl Pts',(-28.1633006172541,39.303224853823,-13.8529470821741));
#33041=CARTESIAN_POINT('Ctrl Pts',(-29.2647880381977,40.7926757902389,-14.2204718556121));
#33042=CARTESIAN_POINT('Ctrl Pts',(-30.377108830674,42.2902929581066,-14.2198708430667));
#33043=CARTESIAN_POINT('Ctrl Pts',(-19.3484767357831,32.5463589446091,1.59674381934693));
#33044=CARTESIAN_POINT('Ctrl Pts',(-19.3698002629981,32.5048979448426,1.15301435963396));
#33045=CARTESIAN_POINT('Ctrl Pts',(-19.3876798928005,32.4497342609156,0.635579189045957));
#33046=CARTESIAN_POINT('Ctrl Pts',(-19.5300863679201,32.3571628326458,-1.86860431100416));
#33047=CARTESIAN_POINT('Ctrl Pts',(-19.8303563485812,32.6011316569382,-3.70979114471445));
#33048=CARTESIAN_POINT('Ctrl Pts',(-20.8181792128701,33.6653932579417,-7.1701426146811));
#33049=CARTESIAN_POINT('Ctrl Pts',(-21.488354478736,34.4835007519095,-8.73670574476536));
#33050=CARTESIAN_POINT('Ctrl Pts',(-23.1249120634581,36.565224284407,-11.3734544104997));
#33051=CARTESIAN_POINT('Ctrl Pts',(-24.0746444553814,37.8183311134315,-12.4221714958561));
#33052=CARTESIAN_POINT('Ctrl Pts',(-26.1598165383407,40.5901015178374,-13.8545909095296));
#33053=CARTESIAN_POINT('Ctrl Pts',(-27.2617619321434,42.080232679423,-14.2195188100388));
#33054=CARTESIAN_POINT('Ctrl Pts',(-28.373935968085,43.577653985901,-14.2201291128083));
#33055=CARTESIAN_POINT('Ctrl Pts',(-20.3574113186624,34.6889740324161,1.47327617534834));
#33056=CARTESIAN_POINT('Ctrl Pts',(-20.3793899820084,34.6462392002826,1.01591373651538));
#33057=CARTESIAN_POINT('Ctrl Pts',(-20.398255055348,34.5951317842909,0.528588481841054));
#33058=CARTESIAN_POINT('Ctrl Pts',(-20.5390678245047,34.503310852838,-1.5540513801246));
#33059=CARTESIAN_POINT('Ctrl Pts',(-20.8100803726225,34.6966201504605,-3.10057294639873));
#33060=CARTESIAN_POINT('Ctrl Pts',(-21.6655176417304,35.5609316342214,-5.98227484335412));
#33061=CARTESIAN_POINT('Ctrl Pts',(-22.2451290911896,36.2341428589745,-7.29352824392187));
#33062=CARTESIAN_POINT('Ctrl Pts',(-23.6436563673474,37.9472635564085,-9.4916763423359));
#33063=CARTESIAN_POINT('Ctrl Pts',(-24.457320064637,38.984667129655,-10.3690524867921));
#33064=CARTESIAN_POINT('Ctrl Pts',(-26.2267249209685,41.2711400510057,-11.5624766483223));
#33065=CARTESIAN_POINT('Ctrl Pts',(-27.1709103277424,42.5108843176131,-11.8682745706401));
#33066=CARTESIAN_POINT('Ctrl Pts',(-28.1127915962418,43.7455088513559,-11.8690397849987));
#33067=CARTESIAN_POINT('Ctrl Pts',(-20.9284639764452,36.9876692386614,1.3554123684922));
#33068=CARTESIAN_POINT('Ctrl Pts',(-20.9510669157184,36.9437205780771,0.885059132406026));
#33069=CARTESIAN_POINT('Ctrl Pts',(-20.9708596003901,36.8964611268051,0.426408611922349));
#33070=CARTESIAN_POINT('Ctrl Pts',(-21.1099628921831,36.8050653317268,-1.25364232218402));
#33071=CARTESIAN_POINT('Ctrl Pts',(-21.3533205643391,36.9504395642519,-2.51864171285581));
#33072=CARTESIAN_POINT('Ctrl Pts',(-22.0820028299708,37.623290434238,-4.84795915809824));
#33073=CARTESIAN_POINT('Ctrl Pts',(-22.5753183406328,38.1584251351963,-5.91517020471142));
#33074=CARTESIAN_POINT('Ctrl Pts',(-23.7464446191913,39.5194025113534,-7.69457540335175));
#33075=CARTESIAN_POINT('Ctrl Pts',(-24.4302727949248,40.350980615974,-8.40795287038753));
#33076=CARTESIAN_POINT('Ctrl Pts',(-25.897975552453,42.173769985802,-9.37372383740198));
#33077=CARTESIAN_POINT('Ctrl Pts',(-26.691577151263,43.1745178860428,-9.62254086016785));
#33078=CARTESIAN_POINT('Ctrl Pts',(-27.4707976903313,44.158119610933,-9.6236915153537));
#33079=CARTESIAN_POINT('Ctrl Pts',(-21.0396888561033,39.3541045014165,1.24768196666922));
#33080=CARTESIAN_POINT('Ctrl Pts',(-21.0628612198437,39.3090486643518,0.765479358346324));
#33081=CARTESIAN_POINT('Ctrl Pts',(-21.0834880350599,39.2652809952961,0.332966405261353));
#33082=CARTESIAN_POINT('Ctrl Pts',(-21.2208317741903,39.1739686379191,-0.978922014776562));
#33083=CARTESIAN_POINT('Ctrl Pts',(-21.4391999183494,39.2759744366273,-1.9863613664762));
#33084=CARTESIAN_POINT('Ctrl Pts',(-22.0516290334592,39.773212128048,-3.81078790540083));
#33085=CARTESIAN_POINT('Ctrl Pts',(-22.4662328810889,40.1823964038332,-4.65460264921481));
#33086=CARTESIAN_POINT('Ctrl Pts',(-23.4293266125922,41.2212230249772,-6.05121512481796));
#33087=CARTESIAN_POINT('Ctrl Pts',(-23.9945420870012,41.8647634287767,-6.61423873305477));
#33088=CARTESIAN_POINT('Ctrl Pts',(-25.186202443381,43.2633027806102,-7.37244739480955));
#33089=CARTESIAN_POINT('Ctrl Pts',(-25.8421831847333,44.0456294021717,-7.56862230197604));
#33090=CARTESIAN_POINT('Ctrl Pts',(-26.4726264127402,44.7996294168197,-7.57037421505982));
#33091=CARTESIAN_POINT('Ctrl Pts',(-16.6854562787122,33.9789464595043,1.59647077610273));
#33092=CARTESIAN_POINT('Ctrl Pts',(-16.712472384757,33.9409293131097,1.1525917014065));
#33093=CARTESIAN_POINT('Ctrl Pts',(-16.7380701330052,33.8890125875519,0.635573044895123));
#33094=CARTESIAN_POINT('Ctrl Pts',(-16.8929361804277,33.8192589011608,-1.86858636178875));
#33095=CARTESIAN_POINT('Ctrl Pts',(-17.1543030074508,34.1010104999321,-3.71029995868829));
#33096=CARTESIAN_POINT('Ctrl Pts',(-17.9818681105611,35.297774448387,-7.16936247494685));
#33097=CARTESIAN_POINT('Ctrl Pts',(-18.5280220225195,36.2012418527131,-8.73699595767482));
#33098=CARTESIAN_POINT('Ctrl Pts',(-19.8519402482494,38.4952930132476,-11.373025698245));
#33099=CARTESIAN_POINT('Ctrl Pts',(-20.6132138376804,39.869806870641,-12.4235805192421));
#33100=CARTESIAN_POINT('Ctrl Pts',(-22.2832067364767,42.9112302679216,-13.8529470821403));
#33101=CARTESIAN_POINT('Ctrl Pts',(-23.1615116341977,44.5422787457965,-14.2204718557263));
#33102=CARTESIAN_POINT('Ctrl Pts',(-24.0493774600889,46.1829520838076,-14.2198708430668));
#33103=CARTESIAN_POINT('Ctrl Pts',(-15.7742431696985,33.7036465139254,1.62964621771032));
#33104=CARTESIAN_POINT('Ctrl Pts',(-15.8010338873345,33.665946534781,1.18947031172183));
#33105=CARTESIAN_POINT('Ctrl Pts',(-15.8265083724999,33.6128691890196,0.664244003017828));
#33106=CARTESIAN_POINT('Ctrl Pts',(-15.9815796560506,33.5424383800423,-1.95287905128809));
#33107=CARTESIAN_POINT('Ctrl Pts',(-16.2491518132338,33.8395682582168,-3.87337387077528));
#33108=CARTESIAN_POINT('Ctrl Pts',(-17.1037835504226,35.0934912894296,-7.48792130215042));
#33109=CARTESIAN_POINT('Ctrl Pts',(-17.6686904038385,36.039408658621,-9.12360836229767));
#33110=CARTESIAN_POINT('Ctrl Pts',(-19.041591625096,38.4400969877808,-11.8774049927335));
#33111=CARTESIAN_POINT('Ctrl Pts',(-19.8308817644157,39.8773452471795,-12.9732563608919));
#33112=CARTESIAN_POINT('Ctrl Pts',(-21.5659485894875,43.059152157502,-14.467685804543));
#33113=CARTESIAN_POINT('Ctrl Pts',(-22.4766667937812,44.7628739707804,-14.8501851005342));
#33114=CARTESIAN_POINT('Ctrl Pts',(-23.399638826952,46.4796709429187,-14.8499483202528));
#33115=CARTESIAN_POINT('Ctrl Pts',(-14.9079435927953,34.0995316375869,1.62975540065009));
#33116=CARTESIAN_POINT('Ctrl Pts',(-14.9347306673254,34.0618367850384,1.18963935152333));
#33117=CARTESIAN_POINT('Ctrl Pts',(-14.9601853534107,34.0087030668416,0.664246445087989));
#33118=CARTESIAN_POINT('Ctrl Pts',(-15.1149627251549,33.9376286808331,-1.95288623098056));
#33119=CARTESIAN_POINT('Ctrl Pts',(-15.3829854641584,34.2357452983242,-3.87317034518422));
#33120=CARTESIAN_POINT('Ctrl Pts',(-16.2371143737293,35.4885670716582,-7.48823335804566));
#33121=CARTESIAN_POINT('Ctrl Pts',(-16.8023296672983,36.4351599686395,-9.12349227713333));
#33122=CARTESIAN_POINT('Ctrl Pts',(-18.1751194544272,38.8356042401957,-11.877576477636));
#33123=CARTESIAN_POINT('Ctrl Pts',(-18.9645920738869,40.2732521647051,-12.9726927515338));
#33124=CARTESIAN_POINT('Ctrl Pts',(-20.6994553318481,43.454613198461,-14.4683433355024));
#33125=CARTESIAN_POINT('Ctrl Pts',(-21.6103158609432,45.1586304949284,-14.8498038985005));
#33126=CARTESIAN_POINT('Ctrl Pts',(-22.5332412158902,46.8753414736307,-14.8500516281495));
#33127=CARTESIAN_POINT('Ctrl Pts',(-14.5197073364542,34.9686592686579,1.59674373345215));
#33128=CARTESIAN_POINT('Ctrl Pts',(-14.5467143347313,34.9306549387464,1.15301430091079));
#33129=CARTESIAN_POINT('Ctrl Pts',(-14.5722625852828,34.878597282106,0.63557915007054));
#33130=CARTESIAN_POINT('Ctrl Pts',(-14.7263938531874,34.8072346531401,-1.86860431101993));
#33131=CARTESIAN_POINT('Ctrl Pts',(-14.9888871347659,35.0914531002031,-3.70979114470526));
#33132=CARTESIAN_POINT('Ctrl Pts',(-15.8151951688241,36.2854639039562,-7.17014261469034));
#33133=CARTESIAN_POINT('Ctrl Pts',(-16.3621201811738,37.1906201277523,-8.73670574476277));
#33134=CARTESIAN_POINT('Ctrl Pts',(-17.6857598215725,39.484061144292,-11.3734544105023));
#33135=CARTESIAN_POINT('Ctrl Pts',(-18.4474896113593,40.8595741644359,-12.4221714958421));
#33136=CARTESIAN_POINT('Ctrl Pts',(-20.116973592377,43.8998828703382,-13.8545909095436));
#33137=CARTESIAN_POINT('Ctrl Pts',(-20.995634995311,45.5316698260284,-14.2195188099103));
#33138=CARTESIAN_POINT('Ctrl Pts',(-21.8833834324344,47.1721284105875,-14.2201291128083));
#33139=CARTESIAN_POINT('Ctrl Pts',(-16.7773762111441,33.8713086176153,0.));
#33140=CARTESIAN_POINT('Ctrl Pts',(-16.8929361804277,33.8192589011608,-1.86858636178876));
#33141=CARTESIAN_POINT('Ctrl Pts',(-17.1543030074532,34.1010104999321,-3.71029995868829));
#33142=CARTESIAN_POINT('Ctrl Pts',(-17.9818681105587,35.297774448387,-7.16936247494685));
#33143=CARTESIAN_POINT('Ctrl Pts',(-18.5280220225147,36.2012418527083,-8.73699595767244));
#33144=CARTESIAN_POINT('Ctrl Pts',(-19.2573188185175,37.4649484236461,-10.1890856763525));
#33145=CARTESIAN_POINT('Ctrl Pts',(-19.3256842021482,37.5839834499338,-10.3203928635213));
#33146=CARTESIAN_POINT('Ctrl Pts',(-19.3950503474463,37.7052869420536,-10.4488603766057));
#33147=CARTESIAN_POINT('Ctrl Pts',(-14.6113821712781,34.8604849513724,9.43689570931383E-16));
#33148=CARTESIAN_POINT('Ctrl Pts',(-14.7263938531874,34.8072346531401,-1.86860431101993));
#33149=CARTESIAN_POINT('Ctrl Pts',(-14.9888871347659,35.0914531002031,-3.70979114470526));
#33150=CARTESIAN_POINT('Ctrl Pts',(-15.8151951688241,36.2854639039562,-7.17014261469034));
#33151=CARTESIAN_POINT('Ctrl Pts',(-16.3621201811738,37.1906201277523,-8.73670574476277));
#33152=CARTESIAN_POINT('Ctrl Pts',(-17.0949852513166,38.4604391632025,-10.1966053555693));
#33153=CARTESIAN_POINT('Ctrl Pts',(-17.1671818300937,38.5861742182181,-10.3350231942229));
#33154=CARTESIAN_POINT('Ctrl Pts',(-17.2404964639283,38.7144417021938,-10.4702558450934));
#33155=CARTESIAN_POINT('Ctrl Pts',(-21.5006126898292,39.0798782217544,1.24689092472207));
#33156=CARTESIAN_POINT('Ctrl Pts',(-21.5299876965042,39.038541623221,0.764254723801767));
#33157=CARTESIAN_POINT('Ctrl Pts',(-21.556776778946,38.9985633313781,0.332948693675433));
#33158=CARTESIAN_POINT('Ctrl Pts',(-21.7078468489019,38.9323887326631,-0.978870002707473));
#33159=CARTESIAN_POINT('Ctrl Pts',(-21.9062112228192,39.0572850320212,-1.98783577087692));
#33160=CARTESIAN_POINT('Ctrl Pts',(-22.4452850348575,39.6445971747049,-3.80852727284806));
#33161=CARTESIAN_POINT('Ctrl Pts',(-22.795201380093,40.1037270851767,-4.65544360716526));
#33162=CARTESIAN_POINT('Ctrl Pts',(-23.6014590279082,41.270810509,-6.04997283348821));
#33163=CARTESIAN_POINT('Ctrl Pts',(-24.0680141309618,41.9853438466691,-6.61832169902486));
#33164=CARTESIAN_POINT('Ctrl Pts',(-25.0499869064454,43.5424691073633,-7.36768403079195));
#33165=CARTESIAN_POINT('Ctrl Pts',(-25.586879818633,44.4080651337966,-7.57138648700893));
#33166=CARTESIAN_POINT('Ctrl Pts',(-26.1039819636366,45.244717762191,-7.56962581969456));
#33167=CARTESIAN_POINT('Ctrl Pts',(-19.5693159454018,37.707864724394,1.35489330510207));
#33168=CARTESIAN_POINT('Ctrl Pts',(-19.597960680827,37.6675557657844,0.884255581224363));
#33169=CARTESIAN_POINT('Ctrl Pts',(-19.6243717351814,37.6238620982378,0.426396977901309));
#33170=CARTESIAN_POINT('Ctrl Pts',(-19.7764631777463,37.5562521484254,-1.25360819501997));
#33171=CARTESIAN_POINT('Ctrl Pts',(-19.9945131659748,37.7300898365971,-2.51960912778664));
#33172=CARTESIAN_POINT('Ctrl Pts',(-20.6224119165105,38.5050289449629,-4.84647586783417));
#33173=CARTESIAN_POINT('Ctrl Pts',(-21.0330824745244,39.1017118880494,-5.91572199042815));
#33174=CARTESIAN_POINT('Ctrl Pts',(-21.999130779075,40.6166651988924,-7.69376028695902));
#33175=CARTESIAN_POINT('Ctrl Pts',(-22.5567852866311,41.5351982120077,-8.41063186556661));
#33176=CARTESIAN_POINT('Ctrl Pts',(-23.7511065841576,43.5504294726618,-9.37059840619976));
#33177=CARTESIAN_POINT('Ctrl Pts',(-24.3935165950074,44.6525338708004,-9.62435378637091));
#33178=CARTESIAN_POINT('Ctrl Pts',(-25.0250626292173,45.7374214437731,-9.6232004636056));
#33179=CARTESIAN_POINT('Ctrl Pts',(-17.9434360021528,35.9854902185572,1.47293201877948));
#33180=CARTESIAN_POINT('Ctrl Pts',(-17.9712842340148,35.9463021021744,1.01538097969612));
#33181=CARTESIAN_POINT('Ctrl Pts',(-17.9972930238973,35.8985773174081,0.528580753666282));
#33182=CARTESIAN_POINT('Ctrl Pts',(-18.1506662116607,35.829758857152,-1.5540287545829));
#33183=CARTESIAN_POINT('Ctrl Pts',(-18.389989532706,36.0565601177328,-3.10121432122698));
#33184=CARTESIAN_POINT('Ctrl Pts',(-19.1152999068524,37.0372859924728,-5.98129145451712));
#33185=CARTESIAN_POINT('Ctrl Pts',(-19.5922318064713,37.7840034012291,-7.29389406572886));
#33186=CARTESIAN_POINT('Ctrl Pts',(-20.7330727613966,39.6794872874845,-9.49113593807784));
#33187=CARTESIAN_POINT('Ctrl Pts',(-21.3902415598656,40.8208685319662,-10.370828601727));
#33188=CARTESIAN_POINT('Ctrl Pts',(-22.8168789077026,43.3372861226137,-11.5604045561153));
#33189=CARTESIAN_POINT('Ctrl Pts',(-23.5745664064031,44.6978537235883,-11.869476154219));
#33190=CARTESIAN_POINT('Ctrl Pts',(-24.3313073348068,46.0542245204214,-11.8687142284813));
#33191=CARTESIAN_POINT('Ctrl Pts',(-16.6854562787122,33.9789464595043,1.59647077610273));
#33192=CARTESIAN_POINT('Ctrl Pts',(-16.712472384757,33.9409293131097,1.1525917014065));
#33193=CARTESIAN_POINT('Ctrl Pts',(-16.7380701330052,33.8890125875519,0.635573044895126));
#33194=CARTESIAN_POINT('Ctrl Pts',(-16.8929361804277,33.8192589011608,-1.86858636178876));
#33195=CARTESIAN_POINT('Ctrl Pts',(-17.1543030074532,34.1010104999321,-3.71029995868829));
#33196=CARTESIAN_POINT('Ctrl Pts',(-17.9818681105587,35.297774448387,-7.16936247494685));
#33197=CARTESIAN_POINT('Ctrl Pts',(-18.5280220225147,36.2012418527083,-8.73699595767244));
#33198=CARTESIAN_POINT('Ctrl Pts',(-19.8519402482542,38.4952930132523,-11.3730256982474));
#33199=CARTESIAN_POINT('Ctrl Pts',(-20.6132138376827,39.869806870641,-12.4235805192421));
#33200=CARTESIAN_POINT('Ctrl Pts',(-22.2832067364743,42.9112302679216,-13.8529470821403));
#33201=CARTESIAN_POINT('Ctrl Pts',(-23.1615116342073,44.5422787457923,-14.2204718557263));
#33202=CARTESIAN_POINT('Ctrl Pts',(-24.0493774600889,46.1829520838076,-14.2198708430668));
#33203=CARTESIAN_POINT('Ctrl Pts',(-14.5197073364542,34.9686592686579,1.59674373345215));
#33204=CARTESIAN_POINT('Ctrl Pts',(-14.5467143347313,34.9306549387464,1.15301430091079));
#33205=CARTESIAN_POINT('Ctrl Pts',(-14.5722625852828,34.878597282106,0.63557915007054));
#33206=CARTESIAN_POINT('Ctrl Pts',(-14.7263938531874,34.8072346531401,-1.86860431101993));
#33207=CARTESIAN_POINT('Ctrl Pts',(-14.9888871347659,35.0914531002031,-3.70979114470526));
#33208=CARTESIAN_POINT('Ctrl Pts',(-15.8151951688241,36.2854639039562,-7.17014261469035));
#33209=CARTESIAN_POINT('Ctrl Pts',(-16.3621201811738,37.1906201277523,-8.73670574476277));
#33210=CARTESIAN_POINT('Ctrl Pts',(-17.6857598215725,39.484061144292,-11.3734544105023));
#33211=CARTESIAN_POINT('Ctrl Pts',(-18.4474896113593,40.8595741644407,-12.4221714958421));
#33212=CARTESIAN_POINT('Ctrl Pts',(-20.116973592377,43.8998828703334,-13.8545909095436));
#33213=CARTESIAN_POINT('Ctrl Pts',(-20.9956349953185,45.531669826028,-14.2195188099103));
#33214=CARTESIAN_POINT('Ctrl Pts',(-21.8833834324344,47.1721284105875,-14.2201291128083));
#33215=CARTESIAN_POINT('Ctrl Pts',(-15.21344650034,37.2330519862577,1.47327608945353));
#33216=CARTESIAN_POINT('Ctrl Pts',(-15.2412832516021,37.193880025428,1.0159136786565));
#33217=CARTESIAN_POINT('Ctrl Pts',(-15.2672296481932,37.1459775929339,0.528588449417375));
#33218=CARTESIAN_POINT('Ctrl Pts',(-15.4196766250125,37.0751310137801,-1.55405138011061));
#33219=CARTESIAN_POINT('Ctrl Pts',(-15.6604198747701,37.3050418083574,-3.10057294640882));
#33220=CARTESIAN_POINT('Ctrl Pts',(-16.3841456768375,38.2822972641546,-5.982274843344));
#33221=CARTESIAN_POINT('Ctrl Pts',(-16.8620495709161,39.031143478966,-7.29352824391929));
#33222=CARTESIAN_POINT('Ctrl Pts',(-18.0025393609276,40.9258582609531,-9.49167634233843));
#33223=CARTESIAN_POINT('Ctrl Pts',(-18.6602832132086,42.0684989791507,-10.3690524867684));
#33224=CARTESIAN_POINT('Ctrl Pts',(-20.0862790553937,44.5835114688915,-11.5624766483459));
#33225=CARTESIAN_POINT('Ctrl Pts',(-20.84442001122,45.9450085199879,-11.8682745704831));
#33226=CARTESIAN_POINT('Ctrl Pts',(-21.6010088957269,47.3011100364939,-11.8690397849987));
#33227=CARTESIAN_POINT('Ctrl Pts',(-15.45154822894,39.5896190563862,1.35541228259734));
#33228=CARTESIAN_POINT('Ctrl Pts',(-15.4801756476489,39.5493344659328,0.885059075369853));
#33229=CARTESIAN_POINT('Ctrl Pts',(-15.5064925913597,39.5053728442132,0.426408585753786));
#33230=CARTESIAN_POINT('Ctrl Pts',(-15.6571869876978,39.4347037901454,-1.25364232213566));
#33231=CARTESIAN_POINT('Ctrl Pts',(-15.877378719186,39.6132317302961,-2.51864171288877));
#33232=CARTESIAN_POINT('Ctrl Pts',(-16.5028873873638,40.3829362474577,-4.84795915806517));
#33233=CARTESIAN_POINT('Ctrl Pts',(-16.915024048968,40.9828301658262,-5.91517020469925));
#33234=CARTESIAN_POINT('Ctrl Pts',(-17.8805426754533,42.4966234016211,-7.69457540336378));
#33235=CARTESIAN_POINT('Ctrl Pts',(-18.4390645629117,43.4170561363981,-8.40795287034454));
#33236=CARTESIAN_POINT('Ctrl Pts',(-19.6324182481966,45.430168019251,-9.3737238374448));
#33237=CARTESIAN_POINT('Ctrl Pts',(-20.2755208515746,46.533671031965,-9.62254085991564));
#33238=CARTESIAN_POINT('Ctrl Pts',(-20.9068289285808,47.618155754582,-9.6236915153537));
#33239=CARTESIAN_POINT('Ctrl Pts',(-15.2248621479928,41.9477963710448,1.24768188077433));
#33240=CARTESIAN_POINT('Ctrl Pts',(-15.2542107628449,41.9064969111878,0.765479302060699));
#33241=CARTESIAN_POINT('Ctrl Pts',(-15.2808564144377,41.8661102394573,0.332966384810895));
#33242=CARTESIAN_POINT('Ctrl Pts',(-15.4297972934795,41.7952733633823,-0.978922014690554));
#33243=CARTESIAN_POINT('Ctrl Pts',(-15.6314258258816,41.9273179171967,-1.98636136653799));
#33244=CARTESIAN_POINT('Ctrl Pts',(-16.1668569942086,42.506652196413,-3.81078790533882));
#33245=CARTESIAN_POINT('Ctrl Pts',(-16.5190077783543,42.970675845735,-4.65460264919543));
#33246=CARTESIAN_POINT('Ctrl Pts',(-17.3244581617424,44.135991238422,-6.05121512483706));
#33247=CARTESIAN_POINT('Ctrl Pts',(-17.7923352091806,44.8534198776255,-6.61423873298768));
#33248=CARTESIAN_POINT('Ctrl Pts',(-18.772833279554,46.4073150662864,-7.37244739487633));
#33249=CARTESIAN_POINT('Ctrl Pts',(-19.3108003965693,47.2750345238072,-7.56862230159521));
#33250=CARTESIAN_POINT('Ctrl Pts',(-19.827521231076,48.1110813316861,-7.5703742150598));
#33251=CARTESIAN_POINT('Ctrl Pts',(-11.6799141290248,36.0076777827441,1.5964706812662));
#33252=CARTESIAN_POINT('Ctrl Pts',(-11.7120656519288,35.9738923911233,1.15259163661472));
#33253=CARTESIAN_POINT('Ctrl Pts',(-11.7447913705091,35.92614704651,0.635573001832125));
#33254=CARTESIAN_POINT('Ctrl Pts',(-11.90800808671,35.8791430893682,-1.86858636171601));
#33255=CARTESIAN_POINT('Ctrl Pts',(-12.1266171429531,36.1952232408274,-3.71029995871332));
#33256=CARTESIAN_POINT('Ctrl Pts',(-12.7754415589707,37.4975806517049,-7.16936247492168));
#33257=CARTESIAN_POINT('Ctrl Pts',(-13.1874595939467,38.4695778661641,-8.73699595765301));
#33258=CARTESIAN_POINT('Ctrl Pts',(-14.1714247212182,40.9286921018696,-11.3730256982666));
#33259=CARTESIAN_POINT('Ctrl Pts',(-14.7293359258389,42.3975559177982,-12.4235805192321));
#33260=CARTESIAN_POINT('Ctrl Pts',(-15.9494910259352,45.6456867796067,-13.85294708215));
#33261=CARTESIAN_POINT('Ctrl Pts',(-16.586733645961,47.3851293551697,-14.2204718557119));
#33262=CARTESIAN_POINT('Ctrl Pts',(-17.2320701170944,49.135459485718,-14.2198708430666));
#33263=CARTESIAN_POINT('Ctrl Pts',(-10.8171551228317,35.6055008474196,1.62964612287377));
#33264=CARTESIAN_POINT('Ctrl Pts',(-10.8490384138683,35.5719973186131,1.18947024666915));
#33265=CARTESIAN_POINT('Ctrl Pts',(-10.881807297469,35.5230856250774,0.6642439580119));
#33266=CARTESIAN_POINT('Ctrl Pts',(-11.045323525379,35.4754406456305,-1.95287905121106));
#33267=CARTESIAN_POINT('Ctrl Pts',(-11.2678861931098,35.807625658362,-3.87337387079559));
#33268=CARTESIAN_POINT('Ctrl Pts',(-11.9353671583008,37.1704123385714,-7.48792130213002));
#33269=CARTESIAN_POINT('Ctrl Pts',(-12.3599059969334,38.1870962603156,-9.1236083622735));
#33270=CARTESIAN_POINT('Ctrl Pts',(-13.3771794920611,40.7587332590992,-11.8774049927576));
#33271=CARTESIAN_POINT('Ctrl Pts',(-13.9538940422131,42.2936801020572,-12.973256360882));
#33272=CARTESIAN_POINT('Ctrl Pts',(-15.2184820528883,45.690026560441,-14.4676858045528));
#33273=CARTESIAN_POINT('Ctrl Pts',(-15.8774655648087,47.5060156561272,-14.8501851005389));
#33274=CARTESIAN_POINT('Ctrl Pts',(-16.5467173899501,49.3366907261819,-14.8499483202528));
#33275=CARTESIAN_POINT('Ctrl Pts',(-9.90333289917187,35.8740691471581,1.62975530581353));
#33276=CARTESIAN_POINT('Ctrl Pts',(-9.9352118545932,35.8405701742916,1.18963928646021));
#33277=CARTESIAN_POINT('Ctrl Pts',(-9.967969163272,35.7915998644065,0.664246400084043));
#33278=CARTESIAN_POINT('Ctrl Pts',(-10.1312860615336,35.7432760306003,-1.95288623090985));
#33279=CARTESIAN_POINT('Ctrl Pts',(-10.3541542971741,36.0765018635767,-3.87317034519018));
#33280=CARTESIAN_POINT('Ctrl Pts',(-11.0212942781335,37.4381269352497,-7.48823335803968));
#33281=CARTESIAN_POINT('Ctrl Pts',(-11.446042279824,38.4555234045252,-9.12349227710921));
#33282=CARTESIAN_POINT('Ctrl Pts',(-12.4632402080729,41.026902971114,-11.8775764776601));
#33283=CARTESIAN_POINT('Ctrl Pts',(-13.0400785027102,42.5622713808053,-12.9726927515287));
#33284=CARTESIAN_POINT('Ctrl Pts',(-14.3045284731422,45.9581475303872,-14.4683433355075));
#33285=CARTESIAN_POINT('Ctrl Pts',(-14.963610809563,47.7744493565971,-14.8498038985338));
#33286=CARTESIAN_POINT('Ctrl Pts',(-15.6328286697389,49.6050326655024,-14.8500516281495));
#33287=CARTESIAN_POINT('Ctrl Pts',(-9.39535856987515,36.6790985320904,1.59674363861559));
#33288=CARTESIAN_POINT('Ctrl Pts',(-9.42749925373957,36.6453245303234,1.15301423609216));
#33289=CARTESIAN_POINT('Ctrl Pts',(-9.46019603501697,36.5974326448294,0.635579107012493));
#33290=CARTESIAN_POINT('Ctrl Pts',(-9.62291442709551,36.5487315518023,-1.86860431096297));
#33291=CARTESIAN_POINT('Ctrl Pts',(-9.84228740311376,36.8674137538594,-3.70979114470519));
#33292=CARTESIAN_POINT('Ctrl Pts',(-10.4902593585524,38.1668671434053,-7.17014261469044));
#33293=CARTESIAN_POINT('Ctrl Pts',(-10.9028003011769,39.1406457266856,-8.73670574474349));
#33294=CARTESIAN_POINT('Ctrl Pts',(-11.8865765112442,41.599116381909,-11.3734544105216));
#33295=CARTESIAN_POINT('Ctrl Pts',(-12.4447970770804,43.0690341146661,-12.4221714958371));
#33296=CARTESIAN_POINT('Ctrl Pts',(-13.6646070765712,46.3159892044746,-13.8545909095487));
#33297=CARTESIAN_POINT('Ctrl Pts',(-14.3020974767632,48.056213477209,-14.2195188099818));
#33298=CARTESIAN_POINT('Ctrl Pts',(-14.9473483165665,49.8063143340193,-14.2201291128084));
#33299=CARTESIAN_POINT('Ctrl Pts',(-11.786216904273,35.9142171164211,0.));
#33300=CARTESIAN_POINT('Ctrl Pts',(-11.90800808671,35.8791430893682,-1.86858636171601));
#33301=CARTESIAN_POINT('Ctrl Pts',(-12.1266171429531,36.1952232408274,-3.71029995871332));
#33302=CARTESIAN_POINT('Ctrl Pts',(-12.7754415589707,37.4975806517049,-7.16936247492168));
#33303=CARTESIAN_POINT('Ctrl Pts',(-13.1874595939467,38.4695778661641,-8.73699595765301));
#33304=CARTESIAN_POINT('Ctrl Pts',(-13.7294890038794,39.8242114819232,-10.1890856763526));
#33305=CARTESIAN_POINT('Ctrl Pts',(-13.7802180759655,39.9517643117923,-10.3203928635211));
#33306=CARTESIAN_POINT('Ctrl Pts',(-13.8316148870599,40.0817049410166,-10.4488603766049));
#33307=CARTESIAN_POINT('Ctrl Pts',(-9.50149509066497,36.5850719698906,1.66533453693773E-16));
#33308=CARTESIAN_POINT('Ctrl Pts',(-9.62291442709551,36.5487315518023,-1.86860431096297));
#33309=CARTESIAN_POINT('Ctrl Pts',(-9.84228740311376,36.8674137538594,-3.70979114470519));
#33310=CARTESIAN_POINT('Ctrl Pts',(-10.4902593585524,38.1668671434053,-7.17014261469044));
#33311=CARTESIAN_POINT('Ctrl Pts',(-10.9028003011769,39.1406457266856,-8.73670574474349));
#33312=CARTESIAN_POINT('Ctrl Pts',(-11.4474917709624,40.5018374092194,-10.1966053555702));
#33313=CARTESIAN_POINT('Ctrl Pts',(-11.5010595286477,40.6365673071016,-10.3350231942242));
#33314=CARTESIAN_POINT('Ctrl Pts',(-11.555373558984,40.773962973293,-10.4702558450947));
#33315=CARTESIAN_POINT('Ctrl Pts',(-15.7201209119707,41.7419576204997,1.2468908298857));
#33316=CARTESIAN_POINT('Ctrl Pts',(-15.7550797324014,41.7052222707522,0.764254661700232));
#33317=CARTESIAN_POINT('Ctrl Pts',(-15.7872856429843,41.6694633881723,0.332948671132101));
#33318=CARTESIAN_POINT('Ctrl Pts',(-15.9462356620105,41.6254618648259,-0.978870002714873));
#33319=CARTESIAN_POINT('Ctrl Pts',(-16.1248063760318,41.7773170936202,-1.98783577091336));
#33320=CARTESIAN_POINT('Ctrl Pts',(-16.5748099612649,42.4353694480747,-3.80852727281139));
#33321=CARTESIAN_POINT('Ctrl Pts',(-16.8558236637272,42.9396243660456,-4.65544360716497));
#33322=CARTESIAN_POINT('Ctrl Pts',(-17.4877814825015,44.2095709902023,-6.0499728334881));
#33323=CARTESIAN_POINT('Ctrl Pts',(-17.8478990309217,44.9832291227819,-6.61832169900053));
#33324=CARTESIAN_POINT('Ctrl Pts',(-18.5982747098126,46.6642543902471,-7.36768403081583));
#33325=CARTESIAN_POINT('Ctrl Pts',(-19.0065156676629,47.5974477252243,-7.57138648692284));
#33326=CARTESIAN_POINT('Ctrl Pts',(-19.3992863750337,48.4991757443115,-7.56962581969423));
#33327=CARTESIAN_POINT('Ctrl Pts',(-14.0037398626874,40.1090570584213,1.35489321026565));
#33328=CARTESIAN_POINT('Ctrl Pts',(-14.0378295966248,40.0732349602049,0.88425551828651));
#33329=CARTESIAN_POINT('Ctrl Pts',(-14.0701900799515,40.0337447201284,0.426396949022747));
#33330=CARTESIAN_POINT('Ctrl Pts',(-14.2303553472444,39.9884678119799,-1.25360819500586));
#33331=CARTESIAN_POINT('Ctrl Pts',(-14.4214462185203,40.1915678318707,-2.51960912781608));
#33332=CARTESIAN_POINT('Ctrl Pts',(-14.9326685312527,41.0479784867297,-4.84647586780456));
#33333=CARTESIAN_POINT('Ctrl Pts',(-15.2542422185737,41.6970325717764,-5.91572199042071));
#33334=CARTESIAN_POINT('Ctrl Pts',(-15.9948572088948,43.3340488505561,-7.69376028696617));
#33335=CARTESIAN_POINT('Ctrl Pts',(-16.4161147204151,44.3225950330595,-8.4106318655519));
#33336=CARTESIAN_POINT('Ctrl Pts',(-17.3114822382705,46.4872837874926,-9.37059840621415));
#33337=CARTESIAN_POINT('Ctrl Pts',(-17.7905076322735,47.6695948287831,-9.62435378631354));
#33338=CARTESIAN_POINT('Ctrl Pts',(-18.2612298390048,48.8333181822474,-9.62320046360538));
#33339=CARTESIAN_POINT('Ctrl Pts',(-12.6395284821797,38.1728270004196,1.47293192394301));
#33340=CARTESIAN_POINT('Ctrl Pts',(-12.6726703073998,38.1380009815349,1.01538091584913));
#33341=CARTESIAN_POINT('Ctrl Pts',(-12.7052063084714,38.0944634070468,0.528580717859076));
#33342=CARTESIAN_POINT('Ctrl Pts',(-12.8668122636161,38.0481727007018,-1.55402875454173));
#33343=CARTESIAN_POINT('Ctrl Pts',(-13.0714224335465,38.3067247111754,-3.10121432125182));
#33344=CARTESIAN_POINT('Ctrl Pts',(-13.6497783497329,39.3806906392349,-5.98129145449214));
#33345=CARTESIAN_POINT('Ctrl Pts',(-14.0155868029731,40.1876820275718,-7.29389406571664));
#33346=CARTESIAN_POINT('Ctrl Pts',(-14.8750601592335,42.2262312169582,-9.49113593808984));
#33347=CARTESIAN_POINT('Ctrl Pts',(-15.3631044396678,43.4495197173535,-10.3708286017074));
#33348=CARTESIAN_POINT('Ctrl Pts',(-16.4170971139001,46.143355468751,-11.5604045561346));
#33349=CARTESIAN_POINT('Ctrl Pts',(-16.973443488292,47.5979046271405,-11.8694761541855));
#33350=CARTESIAN_POINT('Ctrl Pts',(-17.5294501945613,49.0481649878422,-11.8687142284811));
#33351=CARTESIAN_POINT('Ctrl Pts',(-11.6799141290248,36.0076777827441,1.5964706812662));
#33352=CARTESIAN_POINT('Ctrl Pts',(-11.7120656519288,35.9738923911234,1.15259163661472));
#33353=CARTESIAN_POINT('Ctrl Pts',(-11.7447913705091,35.92614704651,0.635573001832125));
#33354=CARTESIAN_POINT('Ctrl Pts',(-11.90800808671,35.8791430893682,-1.86858636171601));
#33355=CARTESIAN_POINT('Ctrl Pts',(-12.1266171429531,36.1952232408274,-3.71029995871332));
#33356=CARTESIAN_POINT('Ctrl Pts',(-12.7754415589707,37.4975806517049,-7.16936247492168));
#33357=CARTESIAN_POINT('Ctrl Pts',(-13.1874595939467,38.4695778661641,-8.73699595765301));
#33358=CARTESIAN_POINT('Ctrl Pts',(-14.1714247212182,40.9286921018696,-11.3730256982666));
#33359=CARTESIAN_POINT('Ctrl Pts',(-14.7293359258389,42.3975559177982,-12.4235805192321));
#33360=CARTESIAN_POINT('Ctrl Pts',(-15.9494910259353,45.6456867796067,-13.85294708215));
#33361=CARTESIAN_POINT('Ctrl Pts',(-16.5867336459564,47.3851293551714,-14.2204718557261));
#33362=CARTESIAN_POINT('Ctrl Pts',(-17.2320701170944,49.135459485718,-14.2198708430666));
#33363=CARTESIAN_POINT('Ctrl Pts',(-9.39535856987514,36.6790985320904,1.59674363861559));
#33364=CARTESIAN_POINT('Ctrl Pts',(-9.42749925373957,36.6453245303234,1.15301423609216));
#33365=CARTESIAN_POINT('Ctrl Pts',(-9.46019603501696,36.5974326448294,0.635579107012493));
#33366=CARTESIAN_POINT('Ctrl Pts',(-9.6229144270955,36.5487315518023,-1.86860431096297));
#33367=CARTESIAN_POINT('Ctrl Pts',(-9.84228740311375,36.8674137538594,-3.709791144704));
#33368=CARTESIAN_POINT('Ctrl Pts',(-10.4902593585524,38.1668671434053,-7.17014261469164));
#33369=CARTESIAN_POINT('Ctrl Pts',(-10.9028003011769,39.1406457266856,-8.7367057447411));
#33370=CARTESIAN_POINT('Ctrl Pts',(-11.8865765112442,41.599116381909,-11.373454410524));
#33371=CARTESIAN_POINT('Ctrl Pts',(-12.4447970770804,43.0690341146661,-12.4221714958419));
#33372=CARTESIAN_POINT('Ctrl Pts',(-13.6646070765712,46.3159892044746,-13.8545909095439));
#33373=CARTESIAN_POINT('Ctrl Pts',(-14.3020974767647,48.0562134772085,-14.2195188099818));
#33374=CARTESIAN_POINT('Ctrl Pts',(-14.9473483165665,49.8063143340193,-14.2201291128084));
#33375=CARTESIAN_POINT('Ctrl Pts',(-9.75977978596927,39.019172373722,1.47327599461702));
#33376=CARTESIAN_POINT('Ctrl Pts',(-9.79290794826535,38.9843607120663,1.01591361477664));
#33377=CARTESIAN_POINT('Ctrl Pts',(-9.82540747302437,38.9406384185529,0.528588413616415));
#33378=CARTESIAN_POINT('Ctrl Pts',(-9.98638527612875,38.8922084230791,-1.55405138008933));
#33379=CARTESIAN_POINT('Ctrl Pts',(-10.1919583891427,39.1540403939766,-3.1005729464026));
#33380=CARTESIAN_POINT('Ctrl Pts',(-10.7692397539852,40.2243457187347,-5.9822748433503));
#33381=CARTESIAN_POINT('Ctrl Pts',(-11.1357073475209,41.0335825742498,-7.29352824390964));
#33382=CARTESIAN_POINT('Ctrl Pts',(-11.9949425681495,43.0713205117329,-9.49167634234821));
#33383=CARTESIAN_POINT('Ctrl Pts',(-12.4833768073893,44.2959375049237,-10.3690524867635));
#33384=CARTESIAN_POINT('Ctrl Pts',(-13.5369344722799,46.9882911615409,-11.562476648351));
#33385=CARTESIAN_POINT('Ctrl Pts',(-14.0935974137202,48.4438248432674,-11.8682745705641));
#33386=CARTESIAN_POINT('Ctrl Pts',(-14.6494919462609,49.8937970264262,-11.8690397849988));
#33387=CARTESIAN_POINT('Ctrl Pts',(-9.66008352082082,41.385638397964,1.35541218776085));
#33388=CARTESIAN_POINT('Ctrl Pts',(-9.69415264634654,41.3498379554236,0.885059012381331));
#33389=CARTESIAN_POINT('Ctrl Pts',(-9.72645811078717,41.310069095201,0.426408556884646));
#33390=CARTESIAN_POINT('Ctrl Pts',(-9.88567590769772,41.2615653996593,-1.25364232215155));
#33391=CARTESIAN_POINT('Ctrl Pts',(-10.0782192299594,41.4696127334992,-2.51864171286803));
#33392=CARTESIAN_POINT('Ctrl Pts',(-10.5878207478773,42.3205019333897,-4.84795915808608));
#33393=CARTESIAN_POINT('Ctrl Pts',(-10.9103886465764,42.9729429590254,-5.91517020469687));
#33394=CARTESIAN_POINT('Ctrl Pts',(-11.6506444460607,44.6087355895508,-7.69457540336642));
#33395=CARTESIAN_POINT('Ctrl Pts',(-12.0724901502383,45.5992855983428,-8.4079528703493));
#33396=CARTESIAN_POINT('Ctrl Pts',(-12.9672015236564,47.7617388416072,-9.37372383744032));
#33397=CARTESIAN_POINT('Ctrl Pts',(-13.4467134169802,48.9455328277889,-9.62254086000153));
#33398=CARTESIAN_POINT('Ctrl Pts',(-13.9172574201603,50.1088235664895,-9.62369151535392));
#33399=CARTESIAN_POINT('Ctrl Pts',(-9.10010115416782,43.6875520748214,1.24768178593787));
#33400=CARTESIAN_POINT('Ctrl Pts',(-9.13502856601633,43.6508497297507,0.765479239882089));
#33401=CARTESIAN_POINT('Ctrl Pts',(-9.1671506241734,43.6146662116331,0.332966362281924));
#33402=CARTESIAN_POINT('Ctrl Pts',(-9.32465663562954,43.5657468507322,-0.978922014743682));
#33403=CARTESIAN_POINT('Ctrl Pts',(-9.50544098108401,43.7251421134386,-1.98636136650516));
#33404=CARTESIAN_POINT('Ctrl Pts',(-9.95297436774496,44.3747794050551,-3.81078790537194));
#33405=CARTESIAN_POINT('Ctrl Pts',(-10.2355033141481,44.8841962446583,-4.65460264920513));
#33406=CARTESIAN_POINT('Ctrl Pts',(-10.8669137023194,46.1522779478965,-6.0512151248278));
#33407=CARTESIAN_POINT('Ctrl Pts',(-11.2279276952814,46.9289900443738,-6.61423873299737));
#33408=CARTESIAN_POINT('Ctrl Pts',(-11.9773033666127,48.6066082448324,-7.3724473948671));
#33409=CARTESIAN_POINT('Ctrl Pts',(-12.3863053996918,49.5420562727389,-7.56862230169559));
#33410=CARTESIAN_POINT('Ctrl Pts',(-12.7787848949964,50.4431303715412,-7.57037421506015));
#33411=CARTESIAN_POINT('Ctrl Pts',(-6.43660260973351,37.3033966274914,1.59647061166213));
#33412=CARTESIAN_POINT('Ctrl Pts',(-6.47323503721941,37.2745307626499,1.15259158901731));
#33413=CARTESIAN_POINT('Ctrl Pts',(-6.51242252436846,37.2319287549577,0.63557297028587));
#33414=CARTESIAN_POINT('Ctrl Pts',(-6.68066728815624,37.2086313911844,-1.8685863618375));
#33415=CARTESIAN_POINT('Ctrl Pts',(-6.85206832386127,37.5526056149556,-3.71029995870329));
#33416=CARTESIAN_POINT('Ctrl Pts',(-7.30894385840923,38.9340442470357,-7.16936247493174));
#33417=CARTESIAN_POINT('Ctrl Pts',(-7.57843851743967,39.9547842114114,-8.73699595771817));
#33418=CARTESIAN_POINT('Ctrl Pts',(-8.20241985397056,42.5289010478495,-11.3730256982015));
#33419=CARTESIAN_POINT('Ctrl Pts',(-8.54561121040599,44.0622129909419,-12.4235805192329));
#33420=CARTESIAN_POINT('Ctrl Pts',(-9.29108967267749,47.4509287397322,-13.8529470821493));
#33421=CARTESIAN_POINT('Ctrl Pts',(-9.67429759304514,49.2633553782986,-14.2204718556406));
#33422=CARTESIAN_POINT('Ctrl Pts',(-10.063967519702,51.0877106274638,-14.2198708430667));
#33423=CARTESIAN_POINT('Ctrl Pts',(-5.63986099173572,36.7825298650421,1.62964605326979));
#33424=CARTESIAN_POINT('Ctrl Pts',(-5.67618780432403,36.753904820676,1.18947019887616));
#33425=CARTESIAN_POINT('Ctrl Pts',(-5.71558400588145,36.7101544788345,0.664243925045137));
#33426=CARTESIAN_POINT('Ctrl Pts',(-5.88421645976361,36.6862652424053,-1.95287905134559));
#33427=CARTESIAN_POINT('Ctrl Pts',(-6.05723890417332,37.046743060744,-3.87337387078904));
#33428=CARTESIAN_POINT('Ctrl Pts',(-6.52398110941249,38.4906509831423,-7.48792130213652));
#33429=CARTESIAN_POINT('Ctrl Pts',(-6.79950954684187,39.5574047047037,-9.1236083623219));
#33430=CARTESIAN_POINT('Ctrl Pts',(-7.44044656128092,42.2476392596818,-11.8774049927092));
#33431=CARTESIAN_POINT('Ctrl Pts',(-7.79284527697299,43.8490375949694,-12.9732563608828));
#33432=CARTESIAN_POINT('Ctrl Pts',(-8.56121110821509,47.3907837817554,-14.467685804552));
#33433=CARTESIAN_POINT('Ctrl Pts',(-8.95504492395579,49.2820718587439,-14.8501851005484));
#33434=CARTESIAN_POINT('Ctrl Pts',(-9.35695250368079,51.1893577615275,-14.8499483202528));
#33435=CARTESIAN_POINT('Ctrl Pts',(-4.69711890654725,36.9183140647621,1.62975523620955));
#33436=CARTESIAN_POINT('Ctrl Pts',(-4.73344077927283,36.8896929129394,1.18963923866306));
#33437=CARTESIAN_POINT('Ctrl Pts',(-4.77283386569913,36.8458829040853,0.664246367114009));
#33438=CARTESIAN_POINT('Ctrl Pts',(-4.94136562987182,36.8212933555072,-1.95288623103511));
#33439=CARTESIAN_POINT('Ctrl Pts',(-5.11454240778336,37.1828448868685,-3.87317034519198));
#33440=CARTESIAN_POINT('Ctrl Pts',(-5.58111241365297,38.6255544971415,-7.48823335803775));
#33441=CARTESIAN_POINT('Ctrl Pts',(-5.85674647907816,39.6930432805413,-9.12349227713124));
#33442=CARTESIAN_POINT('Ctrl Pts',(-6.4976453322125,42.3830122692843,-11.877576477638));
#33443=CARTESIAN_POINT('Ctrl Pts',(-6.85010653765407,43.9848454910637,-12.9726927515151));
#33444=CARTESIAN_POINT('Ctrl Pts',(-7.61840266562128,47.5261065109321,-14.468343335521));
#33445=CARTESIAN_POINT('Ctrl Pts',(-8.01228979377304,49.4177181994984,-14.8498038986051));
#33446=CARTESIAN_POINT('Ctrl Pts',(-8.41417681322632,51.3249084414062,-14.8500516281495));
#33447=CARTESIAN_POINT('Ctrl Pts',(-4.07974739676235,37.6428571267913,1.59674356901154));
#33448=CARTESIAN_POINT('Ctrl Pts',(-4.11636747459172,37.6140009933267,1.1530141884832));
#33449=CARTESIAN_POINT('Ctrl Pts',(-4.15554717391304,37.5712498180871,0.63557907545804));
#33450=CARTESIAN_POINT('Ctrl Pts',(-4.32354021342559,37.5462016739318,-1.86860431106127));
#33451=CARTESIAN_POINT('Ctrl Pts',(-4.49532708288728,37.8928601802523,-3.70979114471065));
#33452=CARTESIAN_POINT('Ctrl Pts',(-4.95177211900954,39.2713030320479,-7.17014261468482));
#33453=CARTESIAN_POINT('Ctrl Pts',(-5.22153084803041,40.293880650996,-8.73670574474153));
#33454=CARTESIAN_POINT('Ctrl Pts',(-5.84541678129948,42.8673335718654,-11.3734544105234));
#33455=CARTESIAN_POINT('Ctrl Pts',(-6.18876436210449,44.401732731168,-12.4221714958234));
#33456=CARTESIAN_POINT('Ctrl Pts',(-6.93406856619723,47.7892355626834,-13.8545909095623));
#33457=CARTESIAN_POINT('Ctrl Pts',(-7.31741049758119,49.602471204667,-14.2195188100911));
#33458=CARTESIAN_POINT('Ctrl Pts',(-7.70702829356578,51.4265873271605,-14.2201291128084));
#33459=CARTESIAN_POINT('Ctrl Pts',(-6.55512420987382,37.2260157227863,1.04083408558608E-14));
#33460=CARTESIAN_POINT('Ctrl Pts',(-6.68066728815625,37.2086313911844,-1.86858636183749));
#33461=CARTESIAN_POINT('Ctrl Pts',(-6.85206832386186,37.5526056149556,-3.71029995870209));
#33462=CARTESIAN_POINT('Ctrl Pts',(-7.30894385840864,38.9340442470356,-7.16936247493294));
#33463=CARTESIAN_POINT('Ctrl Pts',(-7.57843851743848,39.9547842114066,-8.73699595771578));
#33464=CARTESIAN_POINT('Ctrl Pts',(-7.92216638571018,41.3727684379706,-10.1890856763487));
#33465=CARTESIAN_POINT('Ctrl Pts',(-7.95422644864385,41.5062424636381,-10.3203928635145));
#33466=CARTESIAN_POINT('Ctrl Pts',(-7.98660763468405,41.6421750134759,-10.4488603765967));
#33467=CARTESIAN_POINT('Ctrl Pts',(-4.19818497005511,37.5648924257372,1.0547118733939E-15));
#33468=CARTESIAN_POINT('Ctrl Pts',(-4.32354021342559,37.5462016739318,-1.86860431106127));
#33469=CARTESIAN_POINT('Ctrl Pts',(-4.49532708288728,37.8928601802523,-3.70979114471065));
#33470=CARTESIAN_POINT('Ctrl Pts',(-4.95177211900954,39.2713030320479,-7.17014261468482));
#33471=CARTESIAN_POINT('Ctrl Pts',(-5.22153084803041,40.293880650996,-8.73670574474153));
#33472=CARTESIAN_POINT('Ctrl Pts',(-5.56696037000281,41.7187350432347,-10.1966053555725));
#33473=CARTESIAN_POINT('Ctrl Pts',(-5.60080882153535,41.8597170717889,-10.3350231942285));
#33474=CARTESIAN_POINT('Ctrl Pts',(-5.6350165713511,42.0034439406478,-10.4702558451009));
#33475=CARTESIAN_POINT('Ctrl Pts',(-9.61961280540192,43.5542911395532,1.24689076028089));
#33476=CARTESIAN_POINT('Ctrl Pts',(-9.65944377882146,43.5229048631143,0.764254616140159));
#33477=CARTESIAN_POINT('Ctrl Pts',(-9.69641089756402,43.4920933360794,0.332948654561765));
#33478=CARTESIAN_POINT('Ctrl Pts',(-9.86000510220709,43.4711606313009,-0.978870002647285));
#33479=CARTESIAN_POINT('Ctrl Pts',(-10.0151469714658,43.6468834551719,-1.98783577088628));
#33480=CARTESIAN_POINT('Ctrl Pts',(-10.3669195547307,44.362279972836,-3.8085272728388));
#33481=CARTESIAN_POINT('Ctrl Pts',(-10.5733099858402,44.9013947223877,-4.65544360724677));
#33482=CARTESIAN_POINT('Ctrl Pts',(-11.0181031366183,46.2483520960035,-6.04997283340668));
#33483=CARTESIAN_POINT('Ctrl Pts',(-11.2644521757368,47.065385574864,-6.61832169903466));
#33484=CARTESIAN_POINT('Ctrl Pts',(-11.7679552730498,48.836090022354,-7.36768403078205));
#33485=CARTESIAN_POINT('Ctrl Pts',(-12.0392336678225,49.8178835406777,-7.57138648668505));
#33486=CARTESIAN_POINT('Ctrl Pts',(-12.2996772587578,50.7663303683513,-7.56962581969437));
#33487=CARTESIAN_POINT('Ctrl Pts',(-8.15308801979184,41.6937446593044,1.35489314066107));
#33488=CARTESIAN_POINT('Ctrl Pts',(-8.19192878357286,41.6631386548741,0.884255472094997));
#33489=CARTESIAN_POINT('Ctrl Pts',(-8.22957992923835,41.6286557481991,0.426396927826334));
#33490=CARTESIAN_POINT('Ctrl Pts',(-8.39455851882925,41.6066335880669,-1.2536081949919));
#33491=CARTESIAN_POINT('Ctrl Pts',(-8.55480021407532,41.8348614090877,-2.51960912779828));
#33492=CARTESIAN_POINT('Ctrl Pts',(-8.93893907695677,42.7553095590112,-4.84647586782256));
#33493=CARTESIAN_POINT('Ctrl Pts',(-9.16486958068628,43.4435219166124,-5.91572199048099));
#33494=CARTESIAN_POINT('Ctrl Pts',(-9.66497447126952,45.1692762327416,-7.69376028690614));
#33495=CARTESIAN_POINT('Ctrl Pts',(-9.94125939867021,46.2077116350292,-8.41063186557169));
#33496=CARTESIAN_POINT('Ctrl Pts',(-10.5194460361915,48.4777910626842,-9.37059840619458));
#33497=CARTESIAN_POINT('Ctrl Pts',(-10.8253352376626,49.7162403038104,-9.6243537861852));
#33498=CARTESIAN_POINT('Ctrl Pts',(-11.1256510703085,50.9351093861917,-9.62320046360547));
#33499=CARTESIAN_POINT('Ctrl Pts',(-7.07831661167178,39.5830751094924,1.47293185433868));
#33500=CARTESIAN_POINT('Ctrl Pts',(-7.11607735826593,39.5533201442214,1.01538086897001));
#33501=CARTESIAN_POINT('Ctrl Pts',(-7.1544782308666,39.5148560779778,0.528580691605906));
#33502=CARTESIAN_POINT('Ctrl Pts',(-7.32102712268554,39.4920354699227,-1.55402875459162));
#33503=CARTESIAN_POINT('Ctrl Pts',(-7.48675886858976,39.7770748570026,-3.1012143212373));
#33504=CARTESIAN_POINT('Ctrl Pts',(-7.90638666804229,40.9224179890837,-5.98129145450676));
#33505=CARTESIAN_POINT('Ctrl Pts',(-8.15362486974844,41.7732553395417,-7.29389406576977));
#33506=CARTESIAN_POINT('Ctrl Pts',(-8.71423422839184,43.913370849246,-9.49113593803685));
#33507=CARTESIAN_POINT('Ctrl Pts',(-9.02321881659917,45.1936639793709,-10.3708286017225));
#33508=CARTESIAN_POINT('Ctrl Pts',(-9.68311056587086,48.0100791639859,-11.5604045561196));
#33509=CARTESIAN_POINT('Ctrl Pts',(-10.0267902081675,49.5289994535078,-11.8694761541237));
#33510=CARTESIAN_POINT('Ctrl Pts',(-10.3707439991144,51.0436262593385,-11.8687142284812));
#33511=CARTESIAN_POINT('Ctrl Pts',(-6.43660260973353,37.3033966274914,1.59647061166213));
#33512=CARTESIAN_POINT('Ctrl Pts',(-6.47323503721941,37.2745307626499,1.15259158901731));
#33513=CARTESIAN_POINT('Ctrl Pts',(-6.51242252436846,37.2319287549577,0.63557297028587));
#33514=CARTESIAN_POINT('Ctrl Pts',(-6.68066728815625,37.2086313911843,-1.8685863618375));
#33515=CARTESIAN_POINT('Ctrl Pts',(-6.85206832386186,37.5526056149556,-3.71029995870209));
#33516=CARTESIAN_POINT('Ctrl Pts',(-7.30894385840864,38.9340442470356,-7.16936247493294));
#33517=CARTESIAN_POINT('Ctrl Pts',(-7.57843851743848,39.9547842114066,-8.73699595771578));
#33518=CARTESIAN_POINT('Ctrl Pts',(-8.20241985397175,42.5289010478543,-11.3730256982039));
#33519=CARTESIAN_POINT('Ctrl Pts',(-8.545611210406,44.0622129909466,-12.423580519233));
#33520=CARTESIAN_POINT('Ctrl Pts',(-9.2910896726775,47.4509287397274,-13.8529470821493));
#33521=CARTESIAN_POINT('Ctrl Pts',(-9.67429759304181,49.2633553783029,-14.2204718556406));
#33522=CARTESIAN_POINT('Ctrl Pts',(-10.063967519702,51.0877106274638,-14.2198708430667));
#33523=CARTESIAN_POINT('Ctrl Pts',(-4.07974739676235,37.6428571267913,1.59674356901154));
#33524=CARTESIAN_POINT('Ctrl Pts',(-4.11636747459172,37.6140009933267,1.15301418848321));
#33525=CARTESIAN_POINT('Ctrl Pts',(-4.15554717391304,37.5712498180871,0.635579075458043));
#33526=CARTESIAN_POINT('Ctrl Pts',(-4.32354021342559,37.5462016739318,-1.86860431106127));
#33527=CARTESIAN_POINT('Ctrl Pts',(-4.49532708288667,37.8928601802523,-3.70979114470945));
#33528=CARTESIAN_POINT('Ctrl Pts',(-4.95177211901013,39.2713030320479,-7.17014261468602));
#33529=CARTESIAN_POINT('Ctrl Pts',(-5.2215308480298,40.2938806509912,-8.73670574474154));
#33530=CARTESIAN_POINT('Ctrl Pts',(-5.84541678130007,42.8673335718702,-11.3734544105235));
#33531=CARTESIAN_POINT('Ctrl Pts',(-6.18876436210508,44.4017327311728,-12.4221714958234));
#33532=CARTESIAN_POINT('Ctrl Pts',(-6.93406856619663,47.7892355626786,-13.8545909095623));
#33533=CARTESIAN_POINT('Ctrl Pts',(-7.31741049758291,49.6024712046703,-14.2195188100911));
#33534=CARTESIAN_POINT('Ctrl Pts',(-7.70702829356578,51.4265873271605,-14.2201291128084));
#33535=CARTESIAN_POINT('Ctrl Pts',(-4.10743210000917,40.0109749372548,1.4732759250127));
#33536=CARTESIAN_POINT('Ctrl Pts',(-4.1451772795017,39.9812322386711,1.01591356788184));
#33537=CARTESIAN_POINT('Ctrl Pts',(-4.18356833531979,39.9425801423931,0.528588387352919));
#33538=CARTESIAN_POINT('Ctrl Pts',(-4.34979992137163,39.9175526247723,-1.55405138010999));
#33539=CARTESIAN_POINT('Ctrl Pts',(-4.51601802194056,40.2059756280482,-3.10057294640714));
#33540=CARTESIAN_POINT('Ctrl Pts',(-4.93510316561713,41.3475424919709,-5.98227484334561));
#33541=CARTESIAN_POINT('Ctrl Pts',(-5.1826742352202,42.2006962594516,-7.29352824388366));
#33542=CARTESIAN_POINT('Ctrl Pts',(-5.74316333527953,44.3399748842767,-9.491676342374));
#33543=CARTESIAN_POINT('Ctrl Pts',(-6.05234484884677,45.6216384820463,-10.3690524867497));
#33544=CARTESIAN_POINT('Ctrl Pts',(-6.71201694061643,48.4365247491691,-11.5624766483647));
#33545=CARTESIAN_POINT('Ctrl Pts',(-7.0558698155059,49.9564645931987,-11.8682745706829));
#33546=CARTESIAN_POINT('Ctrl Pts',(-7.39975358641498,51.4707901907297,-11.8690397849987));
#33547=CARTESIAN_POINT('Ctrl Pts',(-3.67196736957042,42.3391654916811,1.35541211815631));
#33548=CARTESIAN_POINT('Ctrl Pts',(-3.71078465278244,42.3085779896597,0.885058966166922));
#33549=CARTESIAN_POINT('Ctrl Pts',(-3.74842099134597,42.2738114687004,0.426408535672664));
#33550=CARTESIAN_POINT('Ctrl Pts',(-3.91292097417315,42.2484605261848,-1.25364232209351));
#33551=CARTESIAN_POINT('Ctrl Pts',(-4.07389626035039,42.4817920098841,-2.51864171287881));
#33552=CARTESIAN_POINT('Ctrl Pts',(-4.45721661076271,43.39654424226,-4.84795915807511));
#33553=CARTESIAN_POINT('Ctrl Pts',(-4.68364919433047,44.0882505573392,-5.91517020463728));
#33554=CARTESIAN_POINT('Ctrl Pts',(-5.18357269340369,45.8127425618219,-7.69457540342575));
#33555=CARTESIAN_POINT('Ctrl Pts',(-5.46015465230814,46.8532451029886,-8.40795287033531));
#33556=CARTESIAN_POINT('Ctrl Pts',(-6.03800997040064,49.121018394627,-9.37372383745409));
#33557=CARTESIAN_POINT('Ctrl Pts',(-6.34416967429387,50.3610047225046,-9.62254086018695));
#33558=CARTESIAN_POINT('Ctrl Pts',(-6.64437068472167,51.5794202324977,-9.62369151535378));
#33559=CARTESIAN_POINT('Ctrl Pts',(-2.79008834334092,44.5379552064474,1.24768171633309));
#33560=CARTESIAN_POINT('Ctrl Pts',(-2.82988353081818,44.5065971288888,0.765479194287426));
#33561=CARTESIAN_POINT('Ctrl Pts',(-2.86682808255848,44.4753533549302,0.332966345687857));
#33562=CARTESIAN_POINT('Ctrl Pts',(-3.02969285881549,44.449347365471,-0.978922014608904));
#33563=CARTESIAN_POINT('Ctrl Pts',(-3.18595276920677,44.632848509067,-1.98636136651854));
#33564=CARTESIAN_POINT('Ctrl Pts',(-3.53647788529618,45.3395640713889,-3.8107879053583));
#33565=CARTESIAN_POINT('Ctrl Pts',(-3.74363351930891,45.8840038433944,-4.65460264909516));
#33566=CARTESIAN_POINT('Ctrl Pts',(-4.18815021742049,47.2290373705107,-6.05121512493738));
#33567=CARTESIAN_POINT('Ctrl Pts',(-4.43495195221376,48.0492213058477,-6.61423873296882));
#33568=CARTESIAN_POINT('Ctrl Pts',(-4.93795009678085,49.8164110493997,-7.37244739489531));
#33569=CARTESIAN_POINT('Ctrl Pts',(-5.20966094389456,50.8005446234645,-7.56862230199518));
#33570=CARTESIAN_POINT('Ctrl Pts',(-5.46990934942758,51.7483027430073,-7.57037421505994));
#33571=CARTESIAN_POINT('Ctrl Pts',(-1.06226042837003,37.8397258902528,1.59647049649061));
#33572=CARTESIAN_POINT('Ctrl Pts',(-1.1026280281322,37.8163671782172,1.15259151032668));
#33573=CARTESIAN_POINT('Ctrl Pts',(-1.14747953738506,37.7797757625757,0.635572917996464));
#33574=CARTESIAN_POINT('Ctrl Pts',(-1.31732736909556,37.7806592587273,-1.86858636177033));
#33575=CARTESIAN_POINT('Ctrl Pts',(-1.43803115336731,38.1455252315354,-3.71029995869598));
#33576=CARTESIAN_POINT('Ctrl Pts',(-1.69365713820691,39.5779229780087,-7.16936247493924));
#33577=CARTESIAN_POINT('Ctrl Pts',(-1.81514228728896,40.6266263701707,-8.73699595770183));
#33578=CARTESIAN_POINT('Ctrl Pts',(-2.06643737216329,43.2633442117449,-11.373025698218));
#33579=CARTESIAN_POINT('Ctrl Pts',(-2.18792249430895,44.8298904725309,-12.4235805192224));
#33580=CARTESIAN_POINT('Ctrl Pts',(-2.44354852690307,48.2902066278842,-13.85294708216));
#33581=CARTESIAN_POINT('Ctrl Pts',(-2.56492073910889,50.1387215498278,-14.2204718556691));
#33582=CARTESIAN_POINT('Ctrl Pts',(-2.69099156569461,51.9999633056261,-14.2198708430667));
#33583=CARTESIAN_POINT('Ctrl Pts',(-0.347755560296872,37.2107726459064,
1.62964593809825));
#33584=CARTESIAN_POINT('Ctrl Pts',(-0.387786383582009,37.1876088095763,
1.18947011987008));
#33585=CARTESIAN_POINT('Ctrl Pts',(-0.433007907800631,37.1499104513488,
0.664243870396088));
#33586=CARTESIAN_POINT('Ctrl Pts',(-0.603323715733815,37.150263273314,-1.95287905127288));
#33587=CARTESIAN_POINT('Ctrl Pts',(-0.723283698713102,37.5316956084199,
-3.87337387078179));
#33588=CARTESIAN_POINT('Ctrl Pts',(-0.979785618814999,39.027330971542,-7.48792130214399));
#33589=CARTESIAN_POINT('Ctrl Pts',(-1.10069469072641,40.1224384633822,-9.12360836231754));
#33590=CARTESIAN_POINT('Ctrl Pts',(-1.35224759480685,42.8765051571252,-11.8774049927137));
#33591=CARTESIAN_POINT('Ctrl Pts',(-1.47315665468807,44.5117551326448,-12.9732563608769));
#33592=CARTESIAN_POINT('Ctrl Pts',(-1.72965859378935,48.1268013089941,-14.4676858045579));
#33593=CARTESIAN_POINT('Ctrl Pts',(-1.85032539219324,50.0548871962143,-14.8501851005342));
#33594=CARTESIAN_POINT('Ctrl Pts',(-1.97670704765985,51.9999570907662,-14.8499483202528));
#33595=CARTESIAN_POINT('Ctrl Pts',(0.604714876209436,37.2110085708708,1.62975512103804));
#33596=CARTESIAN_POINT('Ctrl Pts',(0.564689496472757,37.1878478844499,1.18963915964465));
#33597=CARTESIAN_POINT('Ctrl Pts',(0.519462564176599,37.1500900231906,0.664246312466032));
#33598=CARTESIAN_POINT('Ctrl Pts',(0.34914675626714,37.1497353315388,-1.95288623096613));
#33599=CARTESIAN_POINT('Ctrl Pts',(0.229186815972868,37.5322524147635,-3.87317034518712));
#33600=CARTESIAN_POINT('Ctrl Pts',(-0.0273151950961962,39.0266771563424,
-7.48823335804281));
#33601=CARTESIAN_POINT('Ctrl Pts',(-0.148224209656999,40.1225272605589,
-9.12349227713644));
#33602=CARTESIAN_POINT('Ctrl Pts',(-0.399777134874554,42.8763256602578,
-11.8775764776329));
#33603=CARTESIAN_POINT('Ctrl Pts',(-0.520686157648164,44.5120149889529,
-12.9726927515284));
#33604=CARTESIAN_POINT('Ctrl Pts',(-0.777188149407516,48.1265710168792,
-14.4683433355078));
#33605=CARTESIAN_POINT('Ctrl Pts',(-0.897861662853957,50.0549848089201,
-14.8498038985528));
#33606=CARTESIAN_POINT('Ctrl Pts',(-1.02423658127914,51.9999570902567,-14.8500516281495));
#33607=CARTESIAN_POINT('Ctrl Pts',(1.31891566289573,37.8403157026637,1.59674345384007));
#33608=CARTESIAN_POINT('Ctrl Pts',(1.27856167200511,37.816964865386,1.15301410976404));
#33609=CARTESIAN_POINT('Ctrl Pts',(1.233696642558,37.7802246921785,0.635579023171323));
#33610=CARTESIAN_POINT('Ctrl Pts',(1.06384881090688,37.7793394042942,-1.86860431100347));
#33611=CARTESIAN_POINT('Ctrl Pts',(0.943145133347886,38.1469172473993,-3.70979114470452));
#33612=CARTESIAN_POINT('Ctrl Pts',(0.687518921089835,39.5762884400051,-7.17014261469109));
#33613=CARTESIAN_POINT('Ctrl Pts',(0.566033915384876,40.6268483631173,-8.73670574474909));
#33614=CARTESIAN_POINT('Ctrl Pts',(0.314738777667144,43.2628954695716,-11.373454410516));
#33615=CARTESIAN_POINT('Ctrl Pts',(0.193253748290465,44.8305401132961,-12.4221714958367));
#33616=CARTESIAN_POINT('Ctrl Pts',(-0.062372415948142,48.2896308976019,
-13.8545909095489));
#33617=CARTESIAN_POINT('Ctrl Pts',(-0.183762141934923,50.1389656602283,
-14.2195188100007));
#33618=CARTESIAN_POINT('Ctrl Pts',(-0.309815399742848,51.9999633043523,
-14.2201291128083));
#33619=CARTESIAN_POINT('Ctrl Pts',(-1.19058808997908,37.7800000000001,0.));
#33620=CARTESIAN_POINT('Ctrl Pts',(-1.31732736909556,37.7806592587273,-1.86858636177033));
#33621=CARTESIAN_POINT('Ctrl Pts',(-1.43803115336732,38.1455252315354,-3.71029995869598));
#33622=CARTESIAN_POINT('Ctrl Pts',(-1.69365713820691,39.5779229780087,-7.16936247493924));
#33623=CARTESIAN_POINT('Ctrl Pts',(-1.81514228728896,40.6266263701707,-8.73699595770183));
#33624=CARTESIAN_POINT('Ctrl Pts',(-1.95357130555243,42.0790951378326,-10.1890856763505));
#33625=CARTESIAN_POINT('Ctrl Pts',(-1.96630970889271,42.2157732130427,-10.3203928635177));
#33626=CARTESIAN_POINT('Ctrl Pts',(-1.9790160823007,42.3549304887752,-10.4488603766009));
#33627=CARTESIAN_POINT('Ctrl Pts',(1.19058808997906,37.78,-4.44089209850063E-16));
#33628=CARTESIAN_POINT('Ctrl Pts',(1.06384881090688,37.7793394042942,-1.86860431100347));
#33629=CARTESIAN_POINT('Ctrl Pts',(0.943145133347886,38.1469172473993,-3.70979114470452));
#33630=CARTESIAN_POINT('Ctrl Pts',(0.687518921089835,39.5762884400051,-7.17014261469109));
#33631=CARTESIAN_POINT('Ctrl Pts',(0.566033915384876,40.6268483631173,-8.73670574474909));
#33632=CARTESIAN_POINT('Ctrl Pts',(0.42689829031798,42.0863595386748,-10.1966053555719));
#33633=CARTESIAN_POINT('Ctrl Pts',(0.413458201812741,42.2307237103642,-10.3350231942277));
#33634=CARTESIAN_POINT('Ctrl Pts',(0.400053103665672,42.3778559173188,-10.4702558451));
#33635=CARTESIAN_POINT('Ctrl Pts',(-3.32327712822014,44.4799848904464,1.24689064510954));
#33636=CARTESIAN_POINT('Ctrl Pts',(-3.36716940899972,44.4545866217131,0.764254540719014));
#33637=CARTESIAN_POINT('Ctrl Pts',(-3.40814518985254,44.429349685102,0.332948627185768));
#33638=CARTESIAN_POINT('Ctrl Pts',(-3.5730532724122,44.4319119278293,-0.97887000265947));
#33639=CARTESIAN_POINT('Ctrl Pts',(-3.70160805588082,44.6279251367563,-1.98783577088437));
#33640=CARTESIAN_POINT('Ctrl Pts',(-3.94798856176874,45.38610240764,-3.80852727284065));
#33641=CARTESIAN_POINT('Ctrl Pts',(-4.07555420744412,45.9491021672715,-4.65544360722303));
#33642=CARTESIAN_POINT('Ctrl Pts',(-4.32412798456521,47.3456501222045,-6.04997283343043));
#33643=CARTESIAN_POINT('Ctrl Pts',(-4.4516935582032,48.1894265020396,-6.61832169899101));
#33644=CARTESIAN_POINT('Ctrl Pts',(-4.6980742029572,50.0137636932261,-7.36768403082578));
#33645=CARTESIAN_POINT('Ctrl Pts',(-4.82686758916904,51.0241709100527,-7.57138648682318));
#33646=CARTESIAN_POINT('Ctrl Pts',(-4.94968218283415,52.0000289040989,-7.56962581969448));
#33647=CARTESIAN_POINT('Ctrl Pts',(-2.13646282181017,42.4296678529921,1.35489302548968));
#33648=CARTESIAN_POINT('Ctrl Pts',(-2.17926392766629,42.4049009926309,0.884255395658553));
#33649=CARTESIAN_POINT('Ctrl Pts',(-2.2214392647697,42.3761273929605,0.426396892757908));
#33650=CARTESIAN_POINT('Ctrl Pts',(-2.38787268687498,42.3778082879602,-1.25360819498149));
#33651=CARTESIAN_POINT('Ctrl Pts',(-2.51400314727613,42.6265178497758,-2.51960912779656));
#33652=CARTESIAN_POINT('Ctrl Pts',(-2.76323860082849,43.5922658248206,-4.8464758678243));
#33653=CARTESIAN_POINT('Ctrl Pts',(-2.88892662741111,44.3056264360907,-5.91572199046689));
#33654=CARTESIAN_POINT('Ctrl Pts',(-3.13834072492098,46.0849874081721,-7.69376028692028));
#33655=CARTESIAN_POINT('Ctrl Pts',(-3.26402870377777,47.1521724801729,-8.41063186554706));
#33656=CARTESIAN_POINT('Ctrl Pts',(-3.51326424840902,49.4814303102183,-9.37059840621927));
#33657=CARTESIAN_POINT('Ctrl Pts',(-3.63979023544687,50.7508064960244,-9.62435378625662));
#33658=CARTESIAN_POINT('Ctrl Pts',(-3.7635861295493,52.0000086477592,-9.62320046360554));
#33659=CARTESIAN_POINT('Ctrl Pts',(-1.37301063256245,40.1875259567355,1.47293173916723));
#33660=CARTESIAN_POINT('Ctrl Pts',(-1.4146215988499,40.1634477706497,1.01538079142922));
#33661=CARTESIAN_POINT('Ctrl Pts',(-1.45810560976051,40.1308402311943,0.52858064812525));
#33662=CARTESIAN_POINT('Ctrl Pts',(-1.62620698164421,40.1319542826288,-1.55402875455442));
#33663=CARTESIAN_POINT('Ctrl Pts',(-1.74968648306504,40.4376784663506,-3.10121432123458));
#33664=CARTESIAN_POINT('Ctrl Pts',(-2.00204375396079,41.6310829191854,-5.98129145450958));
#33665=CARTESIAN_POINT('Ctrl Pts',(-2.1256786473503,42.5084456369459,-7.29389406576053));
#33666=CARTESIAN_POINT('Ctrl Pts',(-2.37601161837514,44.7065608867208,-9.49113593804617));
#33667=CARTESIAN_POINT('Ctrl Pts',(-2.49964647926794,46.0177955705498,-10.3708286017073));
#33668=CARTESIAN_POINT('Ctrl Pts',(-2.75200381047716,48.8994560970608,-11.5604045561349));
#33669=CARTESIAN_POINT('Ctrl Pts',(-2.87602039417758,50.4518266808844,-11.8694761541618));
#33670=CARTESIAN_POINT('Ctrl Pts',(-3.00091936260203,51.9999864978575,-11.8687142284813));
#33671=CARTESIAN_POINT('Ctrl Pts',(-1.06226042837003,37.8397258902528,1.59647049649061));
#33672=CARTESIAN_POINT('Ctrl Pts',(-1.1026280281322,37.8163671782172,1.15259151032668));
#33673=CARTESIAN_POINT('Ctrl Pts',(-1.14747953738506,37.7797757625757,0.635572917996464));
#33674=CARTESIAN_POINT('Ctrl Pts',(-1.31732736909556,37.7806592587273,-1.86858636177033));
#33675=CARTESIAN_POINT('Ctrl Pts',(-1.43803115336732,38.1455252315354,-3.71029995869598));
#33676=CARTESIAN_POINT('Ctrl Pts',(-1.69365713820691,39.5779229780087,-7.16936247493924));
#33677=CARTESIAN_POINT('Ctrl Pts',(-1.81514228728896,40.6266263701707,-8.73699595770183));
#33678=CARTESIAN_POINT('Ctrl Pts',(-2.06643737216329,43.2633442117449,-11.373025698218));
#33679=CARTESIAN_POINT('Ctrl Pts',(-2.18792249430954,44.8298904725309,-12.4235805192224));
#33680=CARTESIAN_POINT('Ctrl Pts',(-2.44354852690247,48.2902066278842,-13.85294708216));
#33681=CARTESIAN_POINT('Ctrl Pts',(-2.5649207391089,50.1387215498278,-14.2204718556691));
#33682=CARTESIAN_POINT('Ctrl Pts',(-2.69099156569462,51.9999633056261,-14.2198708430667));
#33683=CARTESIAN_POINT('Ctrl Pts',(1.31891566289574,37.8403157026637,1.59674345384007));
#33684=CARTESIAN_POINT('Ctrl Pts',(1.27856167200497,37.816964865386,1.15301410976406));
#33685=CARTESIAN_POINT('Ctrl Pts',(1.233696642558,37.7802246921785,0.635579023171323));
#33686=CARTESIAN_POINT('Ctrl Pts',(1.06384881090688,37.7793394042942,-1.86860431100347));
#33687=CARTESIAN_POINT('Ctrl Pts',(0.943145133347893,38.1469172473993,-3.70979114470452));
#33688=CARTESIAN_POINT('Ctrl Pts',(0.687518921089845,39.5762884400051,-7.1701426146911));
#33689=CARTESIAN_POINT('Ctrl Pts',(0.566033915384876,40.6268483631173,-8.73670574475149));
#33690=CARTESIAN_POINT('Ctrl Pts',(0.314738777667144,43.2628954695716,-11.3734544105136));
#33691=CARTESIAN_POINT('Ctrl Pts',(0.193253748290465,44.8305401133009,-12.4221714958367));
#33692=CARTESIAN_POINT('Ctrl Pts',(-0.0623724159481351,48.2896308975971,
-13.8545909095489));
#33693=CARTESIAN_POINT('Ctrl Pts',(-0.183762141935176,50.1389656602319,
-14.2195188100007));
#33694=CARTESIAN_POINT('Ctrl Pts',(-0.309815399742848,51.9999633043523,
-14.2201291128083));
#33695=CARTESIAN_POINT('Ctrl Pts',(1.62853105321834,40.1882694324258,1.47327580984132));
#33696=CARTESIAN_POINT('Ctrl Pts',(1.58693724130861,40.1642011727047,1.01591349030511));
#33697=CARTESIAN_POINT('Ctrl Pts',(1.54343618780061,40.1314061200099,0.528588343875644));
#33698=CARTESIAN_POINT('Ctrl Pts',(1.37533481599181,40.1302905677455,-1.55405138008459));
#33699=CARTESIAN_POINT('Ctrl Pts',(1.25185544908535,40.4394331428107,-3.10057294640679));
#33700=CARTESIAN_POINT('Ctrl Pts',(0.99949789152226,41.6290225365179,-5.982274843346));
#33701=CARTESIAN_POINT('Ctrl Pts',(0.875863178863669,42.5087254655101,-7.29352824389351));
#33702=CARTESIAN_POINT('Ctrl Pts',(0.625530141228094,44.7059952341645,-9.49167634236414));
#33703=CARTESIAN_POINT('Ctrl Pts',(0.501895397273555,46.0186144616128,-10.369052486768));
#33704=CARTESIAN_POINT('Ctrl Pts',(0.249537900122171,48.8987303723102,-11.5624766483463));
#33705=CARTESIAN_POINT('Ctrl Pts',(0.12549494483352,50.4521347865942,-11.8682745705925));
#33706=CARTESIAN_POINT('Ctrl Pts',(0.00062241732267218,51.9999864962518,
-11.8690397849987));
#33707=CARTESIAN_POINT('Ctrl Pts',(2.3908994428123,42.4307892712954,1.35541200298501));
#33708=CARTESIAN_POINT('Ctrl Pts',(2.34812421168708,42.4060373833274,0.885058889676137));
#33709=CARTESIAN_POINT('Ctrl Pts',(2.30592316845608,42.3769809488797,0.426408500609331));
#33710=CARTESIAN_POINT('Ctrl Pts',(2.13948974646398,42.3752988308948,-1.2536423221009));
#33711=CARTESIAN_POINT('Ctrl Pts',(2.01335948895661,42.6291645083452,-2.51864171288184));
#33712=CARTESIAN_POINT('Ctrl Pts',(1.76412360301129,43.5891580556313,-4.84795915807201));
#33713=CARTESIAN_POINT('Ctrl Pts',(1.63843584903305,44.306048514286,-5.915170204659));
#33714=CARTESIAN_POINT('Ctrl Pts',(1.38902165105131,46.0841342086093,-7.69457540340395));
#33715=CARTESIAN_POINT('Ctrl Pts',(1.26333384857794,47.1534076509294,-8.40795287035374));
#33716=CARTESIAN_POINT('Ctrl Pts',(1.01409805364822,49.4803356664615,-9.37372383743554));
#33717=CARTESIAN_POINT('Ctrl Pts',(0.887523067773743,50.7512717901712,-9.62254086006318));
#33718=CARTESIAN_POINT('Ctrl Pts',(0.763776277074716,52.0000086453373,-9.62369151535372));
#33719=CARTESIAN_POINT('Ctrl Pts',(3.57672261477347,44.4816940061638,1.24768160116189));
#33720=CARTESIAN_POINT('Ctrl Pts',(3.532869768796,44.4563185563517,0.765479118782403));
#33721=CARTESIAN_POINT('Ctrl Pts',(3.49185481010396,44.4306505608144,0.332966318319628));
#33722=CARTESIAN_POINT('Ctrl Pts',(3.32694672771567,44.4280873491762,-0.978922014648203));
#33723=CARTESIAN_POINT('Ctrl Pts',(3.19839225347182,44.631958819594,-1.98636136652616));
#33724=CARTESIAN_POINT('Ctrl Pts',(2.95201108858767,45.3813659616981,-3.81078790535049));
#33725=CARTESIAN_POINT('Ctrl Pts',(2.82444585837898,45.9497454423788,-4.65460264912874));
#33726=CARTESIAN_POINT('Ctrl Pts',(2.57587192813369,47.3443497895988,-6.05121512490362));
#33727=CARTESIAN_POINT('Ctrl Pts',(2.44830662331527,48.1913089840266,-6.61423873300174));
#33728=CARTESIAN_POINT('Ctrl Pts',(2.20192559708917,50.0120953836876,-7.37244739486218));
#33729=CARTESIAN_POINT('Ctrl Pts',(2.07303718495312,51.024880382195,-7.56862230180471));
#33730=CARTESIAN_POINT('Ctrl Pts',(1.95031777657921,52.0000289004077,-7.57037421505985));
#33731=CARTESIAN_POINT('Ctrl Pts',(4.33370633274505,37.6057474666452,1.59647061166167));
#33732=CARTESIAN_POINT('Ctrl Pts',(4.29042532206453,37.588371419626,1.15259158904763));
#33733=CARTESIAN_POINT('Ctrl Pts',(4.2408228309336,37.5585354835147,0.635572970243792));
#33734=CARTESIAN_POINT('Ctrl Pts',(4.07282953636148,37.5835818541665,-1.86858636171414));
#33735=CARTESIAN_POINT('Ctrl Pts',(4.00528018450669,37.9619119569889,-3.71029995870983));
#33736=CARTESIAN_POINT('Ctrl Pts',(3.95610755718974,39.4161093304775,-7.16936247492528));
#33737=CARTESIAN_POINT('Ctrl Pts',(3.98510500545029,40.4714275735081,-8.73699595768472));
#33738=CARTESIAN_POINT('Ctrl Pts',(4.11161181537177,43.1170704487122,-11.3730256982351));
#33739=CARTESIAN_POINT('Ctrl Pts',(4.21430601437353,44.6849606628027,-12.423580519233));
#33740=CARTESIAN_POINT('Ctrl Pts',(4.45373622021968,48.1464351665736,-13.8529470821494));
#33741=CARTESIAN_POINT('Ctrl Pts',(4.59667050422672,49.9934079386823,-14.2204718556644));
#33742=CARTESIAN_POINT('Ctrl Pts',(4.73676521641214,51.8536466863969,-14.2198708430668));
#33743=CARTESIAN_POINT('Ctrl Pts',(4.9514291922416,36.8815114147052,1.6296460532693));
#33744=CARTESIAN_POINT('Ctrl Pts',(4.90850926387593,36.8642803315734,1.1894701989116));
#33745=CARTESIAN_POINT('Ctrl Pts',(4.85838298962156,36.8334013785589,0.664243924996268));
#33746=CARTESIAN_POINT('Ctrl Pts',(4.68985095932913,36.8579890764766,-1.95287905120227));
#33747=CARTESIAN_POINT('Ctrl Pts',(4.62539547711762,37.252611065952,-3.87337387079324));
#33748=CARTESIAN_POINT('Ctrl Pts',(4.58435548147172,38.7695270469185,-7.48792130213237));
#33749=CARTESIAN_POINT('Ctrl Pts',(4.62052713521612,39.8706950784794,-9.12360836229799));
#33750=CARTESIAN_POINT('Ctrl Pts',(4.76347923307348,42.6325290552246,-11.8774049927332));
#33751=CARTESIAN_POINT('Ctrl Pts',(4.87652118891077,44.2683416970959,-12.9732563608876));
#33752=CARTESIAN_POINT('Ctrl Pts',(5.13710478162637,47.8830959478414,-14.4676858045473));
#33753=CARTESIAN_POINT('Ctrl Pts',(5.29206142838226,49.8087293766846,-14.8501851005056));
#33754=CARTESIAN_POINT('Ctrl Pts',(5.44377846349978,51.7519872491301,-14.8499483202528));
#33755=CARTESIAN_POINT('Ctrl Pts',(5.89423842867639,36.7461942621622,1.62975523620908));
#33756=CARTESIAN_POINT('Ctrl Pts',(5.85132433673285,36.7289655221871,1.18963923869757));
#33757=CARTESIAN_POINT('Ctrl Pts',(5.80118424128265,36.6980284414522,0.664246367065471));
#33758=CARTESIAN_POINT('Ctrl Pts',(5.6325515213262,36.7219158272082,-1.95288623089274));
#33759=CARTESIAN_POINT('Ctrl Pts',(5.56825045711999,37.117611517565,-3.87317034519377));
#33760=CARTESIAN_POINT('Ctrl Pts',(5.52703808201953,38.6333292122907,-7.48823335803598));
#33761=CARTESIAN_POINT('Ctrl Pts',(5.56331547729456,39.7352322893592,-9.12349227711209));
#33762=CARTESIAN_POINT('Ctrl Pts',(5.70622937200357,42.4968007059074,-11.8775764776571));
#33763=CARTESIAN_POINT('Ctrl Pts',(5.81933389104879,44.1330482236871,-12.9726927515247));
#33764=CARTESIAN_POINT('Ctrl Pts',(6.07984767624782,47.7473173225239,-14.4683433355115));
#33765=CARTESIAN_POINT('Ctrl Pts',(6.23484434203113,49.6732762742259,-14.8498038985576));
#33766=CARTESIAN_POINT('Ctrl Pts',(6.38655415380922,51.6164365682427,-14.8500516281495));
#33767=CARTESIAN_POINT('Ctrl Pts',(6.69072942383202,37.2674545852876,1.59674356901112));
#33768=CARTESIAN_POINT('Ctrl Pts',(6.64746300420534,37.2500843961589,1.15301418851277));
#33769=CARTESIAN_POINT('Ctrl Pts',(6.59782596008604,37.2201031407487,0.635579075416795));
#33770=CARTESIAN_POINT('Ctrl Pts',(6.42958094135504,37.2433987309931,-1.86860431094034));
#33771=CARTESIAN_POINT('Ctrl Pts',(6.36241763451085,37.6244130860142,-3.70979114470994));
#33772=CARTESIAN_POINT('Ctrl Pts',(6.31281405856107,39.0756147439152,-7.1701426146855));
#33773=CARTESIAN_POINT('Ctrl Pts',(6.34207586064458,40.1327706007196,-8.73670574472715));
#33774=CARTESIAN_POINT('Ctrl Pts',(6.46848716269878,42.7777495754072,-11.3734544105378));
#33775=CARTESIAN_POINT('Ctrl Pts',(6.57133776971646,44.3467269792927,-12.4221714958377));
#33776=CARTESIAN_POINT('Ctrl Pts',(6.8105934567754,47.806988603268,-13.8545909095479));
#33777=CARTESIAN_POINT('Ctrl Pts',(6.95362708075977,49.6547753637287,-14.2195188100197));
#33778=CARTESIAN_POINT('Ctrl Pts',(7.09370444218574,51.5147699841784,-14.2201291128083));
#33779=CARTESIAN_POINT('Ctrl Pts',(4.19818497005567,37.5648924257371,0.));
#33780=CARTESIAN_POINT('Ctrl Pts',(4.07282953636148,37.5835818541665,-1.86858636171414));
#33781=CARTESIAN_POINT('Ctrl Pts',(4.00528018450669,37.9619119569889,-3.71029995870983));
#33782=CARTESIAN_POINT('Ctrl Pts',(3.95610755718974,39.4161093304775,-7.16936247492528));
#33783=CARTESIAN_POINT('Ctrl Pts',(3.98510500545029,40.4714275735081,-8.73699595768472));
#33784=CARTESIAN_POINT('Ctrl Pts',(4.05479285274666,41.9288128067805,-10.1890856763504));
#33785=CARTESIAN_POINT('Ctrl Pts',(4.06163542615305,42.0659125600701,-10.3203928635173));
#33786=CARTESIAN_POINT('Ctrl Pts',(4.06886253049489,42.2054617208602,-10.4488603766));
#33787=CARTESIAN_POINT('Ctrl Pts',(6.55512420987433,37.2260157227862,1.49880108324396E-15));
#33788=CARTESIAN_POINT('Ctrl Pts',(6.42958094135504,37.2433987309931,-1.86860431094034));
#33789=CARTESIAN_POINT('Ctrl Pts',(6.36241763451085,37.6244130860142,-3.70979114470994));
#33790=CARTESIAN_POINT('Ctrl Pts',(6.31281405856107,39.0756147439152,-7.1701426146855));
#33791=CARTESIAN_POINT('Ctrl Pts',(6.34207586064458,40.1327706007196,-8.73670574472715));
#33792=CARTESIAN_POINT('Ctrl Pts',(6.41206653251571,41.5972271209445,-10.1966053555726));
#33793=CARTESIAN_POINT('Ctrl Pts',(6.41930840847768,41.7420345975434,-10.3350231942287));
#33794=CARTESIAN_POINT('Ctrl Pts',(6.42697885113783,41.8895769551519,-10.470255845101));
#33795=CARTESIAN_POINT('Ctrl Pts',(3.04071090848719,44.5001944306519,1.24689076028073));
#33796=CARTESIAN_POINT('Ctrl Pts',(2.99365083345139,44.4813012009376,0.764254616115602));
#33797=CARTESIAN_POINT('Ctrl Pts',(2.94950053246457,44.4621525981064,0.332948654593303));
#33798=CARTESIAN_POINT('Ctrl Pts',(2.78663561816042,44.488157628525,-0.978870002740165));
#33799=CARTESIAN_POINT('Ctrl Pts',(2.68728492513176,44.7004709588125,-1.98783577089924));
#33800=CARTESIAN_POINT('Ctrl Pts',(2.5513120932872,45.4859946801884,-3.808527272826));
#33801=CARTESIAN_POINT('Ctrl Pts',(2.5051681016477,46.0614183982245,-4.65544360722295));
#33802=CARTESIAN_POINT('Ctrl Pts',(2.45787394353962,47.4791272455719,-6.04997283343073));
#33803=CARTESIAN_POINT('Ctrl Pts',(2.45168870251787,48.3324696724334,-6.61832169901082));
#33804=CARTESIAN_POINT('Ctrl Pts',(2.4674461098152,50.1733013631196,-7.36768403080617));
#33805=CARTESIAN_POINT('Ctrl Pts',(2.48375959427411,51.191753301279,-7.57138648675178));
#33806=CARTESIAN_POINT('Ctrl Pts',(2.50107414862808,52.1751568070596,-7.56962581969456));
#33807=CARTESIAN_POINT('Ctrl Pts',(3.92365461890876,42.3018453782487,1.35489314066083));
#33808=CARTESIAN_POINT('Ctrl Pts',(3.87776447109268,42.2834218397552,0.8842554720871));
#33809=CARTESIAN_POINT('Ctrl Pts',(3.83192350390653,42.2609432866046,0.426396927835306));
#33810=CARTESIAN_POINT('Ctrl Pts',(3.66742334692479,42.286293018581,-1.2536081950185));
#33811=CARTESIAN_POINT('Ctrl Pts',(3.57797177380375,42.5504213117328,-2.51960912780668));
#33812=CARTESIAN_POINT('Ctrl Pts',(3.46871344470325,43.5418092681868,-4.84647586781428));
#33813=CARTESIAN_POINT('Ctrl Pts',(3.44582654101155,44.2657961681553,-5.91572199046192));
#33814=CARTESIAN_POINT('Ctrl Pts',(3.45218058837109,46.0625411381523,-7.69376028692537));
#33815=CARTESIAN_POINT('Ctrl Pts',(3.47964820283096,47.1367510692278,-8.41063186556218));
#33816=CARTESIAN_POINT('Ctrl Pts',(3.56443746806616,49.4777703293277,-9.37059840620427));
#33817=CARTESIAN_POINT('Ctrl Pts',(3.61985039974726,50.7522326212106,-9.62435378621384));
#33818=CARTESIAN_POINT('Ctrl Pts',(3.67509457152212,52.0063376889004,-9.6232004636056));
#33819=CARTESIAN_POINT('Ctrl Pts',(4.36024590432577,39.9738746787522,1.47293185433834));
#33820=CARTESIAN_POINT('Ctrl Pts',(4.31563179085076,39.9559634303423,1.01538086898097));
#33821=CARTESIAN_POINT('Ctrl Pts',(4.26794984367479,39.9298762050513,0.528580691590028));
#33822=CARTESIAN_POINT('Ctrl Pts',(4.10171804395774,39.9549022371194,-1.55402875454521));
#33823=CARTESIAN_POINT('Ctrl Pts',(4.0230044735859,40.2750875547253,-3.10121432124596));
#33824=CARTESIAN_POINT('Ctrl Pts',(3.943054997525,41.4922590552153,-5.98129145449819));
#33825=CARTESIAN_POINT('Ctrl Pts',(3.94554026237911,42.3782865653749,-7.29389406574829));
#33826=CARTESIAN_POINT('Ctrl Pts',(4.01057973631905,44.5896542676588,-9.49113593805846));
#33827=CARTESIAN_POINT('Ctrl Pts',(4.07481145201547,45.9051375482497,-10.3708286017178));
#33828=CARTESIAN_POINT('Ctrl Pts',(4.2351258063561,48.7933811184128,-11.5604045561245));
#33829=CARTESIAN_POINT('Ctrl Pts',(4.33329690121476,50.3476002080609,-11.8694761541191));
#33830=CARTESIAN_POINT('Ctrl Pts',(4.42999533819688,51.8977769668582,-11.8687142284813));
#33831=CARTESIAN_POINT('Ctrl Pts',(4.33370633274505,37.6057474666452,1.59647061166167));
#33832=CARTESIAN_POINT('Ctrl Pts',(4.29042532206453,37.588371419626,1.15259158904763));
#33833=CARTESIAN_POINT('Ctrl Pts',(4.2408228309336,37.5585354835147,0.635572970243792));
#33834=CARTESIAN_POINT('Ctrl Pts',(4.07282953636148,37.5835818541665,-1.86858636171414));
#33835=CARTESIAN_POINT('Ctrl Pts',(4.00528018450669,37.9619119569889,-3.71029995870983));
#33836=CARTESIAN_POINT('Ctrl Pts',(3.95610755718974,39.4161093304775,-7.16936247492528));
#33837=CARTESIAN_POINT('Ctrl Pts',(3.98510500545029,40.4714275735081,-8.73699595768472));
#33838=CARTESIAN_POINT('Ctrl Pts',(4.11161181537177,43.1170704487122,-11.3730256982351));
#33839=CARTESIAN_POINT('Ctrl Pts',(4.21430601437353,44.6849606628027,-12.423580519233));
#33840=CARTESIAN_POINT('Ctrl Pts',(4.45373622021968,48.1464351665736,-13.8529470821494));
#33841=CARTESIAN_POINT('Ctrl Pts',(4.59667050422672,49.9934079386823,-14.2204718556644));
#33842=CARTESIAN_POINT('Ctrl Pts',(4.73676521641214,51.8536466863969,-14.2198708430668));
#33843=CARTESIAN_POINT('Ctrl Pts',(6.69072942383202,37.2674545852876,1.59674356901112));
#33844=CARTESIAN_POINT('Ctrl Pts',(6.64746300420528,37.2500843961589,1.15301418851278));
#33845=CARTESIAN_POINT('Ctrl Pts',(6.59782596008604,37.2201031407487,0.635579075416795));
#33846=CARTESIAN_POINT('Ctrl Pts',(6.42958094135505,37.2433987309931,-1.86860431094034));
#33847=CARTESIAN_POINT('Ctrl Pts',(6.36241763451087,37.6244130860142,-3.70979114471114));
#33848=CARTESIAN_POINT('Ctrl Pts',(6.31281405856107,39.0756147439152,-7.1701426146843));
#33849=CARTESIAN_POINT('Ctrl Pts',(6.34207586064459,40.1327706007148,-8.73670574472715));
#33850=CARTESIAN_POINT('Ctrl Pts',(6.46848716269878,42.777749575412,-11.3734544105378));
#33851=CARTESIAN_POINT('Ctrl Pts',(6.57133776971646,44.3467269792927,-12.4221714958329));
#33852=CARTESIAN_POINT('Ctrl Pts',(6.8105934567754,47.806988603268,-13.8545909095527));
#33853=CARTESIAN_POINT('Ctrl Pts',(6.95362708075977,49.6547753637287,-14.2195188100198));
#33854=CARTESIAN_POINT('Ctrl Pts',(7.09370444218574,51.5147699841784,-14.2201291128083));
#33855=CARTESIAN_POINT('Ctrl Pts',(7.33134203123371,39.5474466673498,1.47327592501241));
#33856=CARTESIAN_POINT('Ctrl Pts',(7.28674631020699,39.5295428029873,1.01591356789178));
#33857=CARTESIAN_POINT('Ctrl Pts',(7.23902080798441,39.5032723984885,0.528588387338081));
#33858=CARTESIAN_POINT('Ctrl Pts',(7.07247170264534,39.526091520959,-1.55405138006663));
#33859=CARTESIAN_POINT('Ctrl Pts',(6.99424475323468,39.8496604164912,-3.10057294640973));
#33860=CARTESIAN_POINT('Ctrl Pts',(6.91375205389164,41.0630557303986,-5.98227484334297));
#33861=CARTESIAN_POINT('Ctrl Pts',(6.91657054442664,41.9513996061356,-7.29352824387643));
#33862=CARTESIAN_POINT('Ctrl Pts',(6.98148962792165,44.1619304425256,-9.49167634238116));
#33863=CARTESIAN_POINT('Ctrl Pts',(7.04591850046981,45.4787841574542,-10.369052486764));
#33864=CARTESIAN_POINT('Ctrl Pts',(7.20601286880595,48.365498857377,-11.5624766483503));
#33865=CARTESIAN_POINT('Ctrl Pts',(7.30430498991546,49.9207450076545,-11.8682745706115));
#33866=CARTESIAN_POINT('Ctrl Pts',(7.40098575043927,51.4706130322883,-11.8690397849987));
#33867=CARTESIAN_POINT('Ctrl Pts',(8.40509445805923,41.6586445536367,1.35541211815614));
#33868=CARTESIAN_POINT('Ctrl Pts',(8.35923205241223,41.6402321528243,0.88505896615835));
#33869=CARTESIAN_POINT('Ctrl Pts',(8.31332538916191,41.6174773021325,0.42640853568319));
#33870=CARTESIAN_POINT('Ctrl Pts',(8.14834662563443,41.6394982516744,-1.25364232212472));
#33871=CARTESIAN_POINT('Ctrl Pts',(8.05962904511026,41.9087301497828,-2.51864171287991));
#33872=CARTESIAN_POINT('Ctrl Pts',(7.94955134754913,42.8944223117342,-4.84795915807392));
#33873=CARTESIAN_POINT('Ctrl Pts',(7.92716706335442,43.621903091586,-5.91517020464439));
#33874=CARTESIAN_POINT('Ctrl Pts',(7.93333952031455,45.4173857785675,-7.69457540341853));
#33875=CARTESIAN_POINT('Ctrl Pts',(7.96110451544885,46.4936627982892,-8.40795287034961));
#33876=CARTESIAN_POINT('Ctrl Pts',(8.04556196575565,48.8323759936388,-9.37372383743963));
#33877=CARTESIAN_POINT('Ctrl Pts',(8.10114839964667,50.1083893187776,-9.62254086010123));
#33878=CARTESIAN_POINT('Ctrl Pts',(8.15637495641955,51.3620268377998,-9.62369151535369));
#33879=CARTESIAN_POINT('Ctrl Pts',(9.87072183560219,43.5199138025263,1.24768171633307));
#33880=CARTESIAN_POINT('Ctrl Pts',(9.82370404146588,43.5010375473779,0.765479194261124));
#33881=CARTESIAN_POINT('Ctrl Pts',(9.77945361533133,43.4814678488037,0.332966345721785));
#33882=CARTESIAN_POINT('Ctrl Pts',(9.61585927297428,43.5023995944714,-0.978922014708797));
#33883=CARTESIAN_POINT('Ctrl Pts',(9.51762723324188,43.7224911565099,-1.98636136651937));
#33884=CARTESIAN_POINT('Ctrl Pts',(9.3804056296356,44.4993341100647,-3.81078790535733));
#33885=CARTESIAN_POINT('Ctrl Pts',(9.33502766337594,45.080082732299,-4.65460264911418));
#33886=CARTESIAN_POINT('Ctrl Pts',(9.28745674947728,46.4958677767823,-6.05121512491815));
#33887=CARTESIAN_POINT('Ctrl Pts',(9.28172473628772,47.3523605835541,-6.61423873299266));
#33888=CARTESIAN_POINT('Ctrl Pts',(9.29697643567208,49.189677678933,-7.37244739487121));
#33889=CARTESIAN_POINT('Ctrl Pts',(9.31353425504065,50.2104967199909,-7.56862230187133));
#33890=CARTESIAN_POINT('Ctrl Pts',(9.33084205690769,51.1931844250963,-7.57037421505979));
#33891=CARTESIAN_POINT('Ctrl Pts',(9.64145132693361,36.6062244663074,1.59647068126639));
#33892=CARTESIAN_POINT('Ctrl Pts',(9.59613798296502,36.5951848118766,1.15259163662228));
#33893=CARTESIAN_POINT('Ctrl Pts',(9.54279427443722,36.5727117312896,0.63557300182231));
#33894=CARTESIAN_POINT('Ctrl Pts',(9.38007537755078,36.6214111051439,-1.86858636168713));
#33895=CARTESIAN_POINT('Ctrl Pts',(9.36705556809957,37.0055036281237,-3.71029995871696));
#33896=CARTESIAN_POINT('Ctrl Pts',(9.52533731119175,38.4518973636396,-7.16936247491812));
#33897=CARTESIAN_POINT('Ctrl Pts',(9.70422705225016,39.4923472214852,-8.73699595765307));
#33898=CARTESIAN_POINT('Ctrl Pts',(10.2059604433763,42.0930574706308,-11.3730256982666));
#33899=CARTESIAN_POINT('Ctrl Pts',(10.5307434056703,43.6303739147712,-12.4235805192466));
#33900=CARTESIAN_POINT('Ctrl Pts',(11.2603557414003,47.0225411281197,-13.8529470821357));
#33901=CARTESIAN_POINT('Ctrl Pts',(11.6646867918734,48.8303727110007,-14.2204718556644));
#33902=CARTESIAN_POINT('Ctrl Pts',(12.0680951184149,50.6517393542017,-14.2198708430667));
#33903=CARTESIAN_POINT('Ctrl Pts',(10.1498171217998,35.8014489642672,1.629646122874));
#33904=CARTESIAN_POINT('Ctrl Pts',(10.1048818153817,35.7905014108269,1.18947024667978));
#33905=CARTESIAN_POINT('Ctrl Pts',(10.0508712182893,35.7670704718624,0.664243957997926));
#33906=CARTESIAN_POINT('Ctrl Pts',(9.88755379330354,35.8153925116915,-1.95287905116997));
#33907=CARTESIAN_POINT('Ctrl Pts',(9.8799149395762,36.2151707898526,-3.8733738708004));
#33908=CARTESIAN_POINT('Ctrl Pts',(10.055172324341,37.7224873536916,-7.48792130212525));
#33909=CARTESIAN_POINT('Ctrl Pts',(10.2476883530401,38.8072993194235,-9.12360836227592));
#33910=CARTESIAN_POINT('Ctrl Pts',(10.7822353606524,41.5206776037667,-11.8774049927552));
#33911=CARTESIAN_POINT('Ctrl Pts',(11.1269271238415,43.1237524839494,-12.9732563608916));
#33912=CARTESIAN_POINT('Ctrl Pts',(11.8992915178615,46.6646288366373,-14.4676858045432));
#33913=CARTESIAN_POINT('Ctrl Pts',(12.3267171394111,48.5486094635681,-14.8501851005151));
#33914=CARTESIAN_POINT('Ctrl Pts',(12.7534443437026,50.4504961875092,-14.8499483202528));
#33915=CARTESIAN_POINT('Ctrl Pts',(11.0637722809467,35.5333334012201,1.62975530581378));
#33916=CARTESIAN_POINT('Ctrl Pts',(11.0188430850089,35.5223873364705,1.18963928647272));
#33917=CARTESIAN_POINT('Ctrl Pts',(10.9648105349674,35.4989008284142,0.664246400067514));
#33918=CARTESIAN_POINT('Ctrl Pts',(10.801293780378,35.5465440138904,-1.95288623086123));
#33919=CARTESIAN_POINT('Ctrl Pts',(10.7939605764728,35.9473630882236,-3.87317034519856));
#33920=CARTESIAN_POINT('Ctrl Pts',(10.9688768024414,37.4535180947963,-7.48823335803128));
#33921=CARTESIAN_POINT('Ctrl Pts',(11.1616021042532,38.5390425757264,-9.12349227711398));
#33922=CARTESIAN_POINT('Ctrl Pts',(11.6960735044253,41.2521634398075,-11.8775764776553));
#33923=CARTESIAN_POINT('Ctrl Pts',(12.0408890833104,42.8556598657977,-12.9726927515335));
#33924=CARTESIAN_POINT('Ctrl Pts',(12.8131153360331,46.3960659393659,-14.4683433355026));
#33925=CARTESIAN_POINT('Ctrl Pts',(13.2406268960164,48.2803630805025,-14.8498038985528));
#33926=CARTESIAN_POINT('Ctrl Pts',(13.6673330636266,50.1821542472109,-14.8500516281495));
#33927=CARTESIAN_POINT('Ctrl Pts',(11.9263392248006,35.9359355586898,1.59674363861582));
#33928=CARTESIAN_POINT('Ctrl Pts',(11.881041157038,35.9248996259739,1.1530142361046));
#33929=CARTESIAN_POINT('Ctrl Pts',(11.8276425661301,35.9022876226716,0.635579106996277));
#33930=CARTESIAN_POINT('Ctrl Pts',(11.664425345244,35.9492898606342,-1.86860431091527));
#33931=CARTESIAN_POINT('Ctrl Pts',(11.652169660341,36.335984374051,-3.70979114470996));
#33932=CARTESIAN_POINT('Ctrl Pts',(11.8095985064428,37.7794742164015,-7.17014261468561));
#33933=CARTESIAN_POINT('Ctrl Pts',(11.9890114302846,38.8217053622519,-8.73670574474104));
#33934=CARTESIAN_POINT('Ctrl Pts',(12.4905558028067,41.4217720607234,-11.373454410524));
#33935=CARTESIAN_POINT('Ctrl Pts',(12.8156483043377,42.9601423694015,-12.422171495837));
#33936=CARTESIAN_POINT('Ctrl Pts',(13.544915286834,46.3511338849317,-13.8545909095487));
#33937=CARTESIAN_POINT('Ctrl Pts',(13.9494605087747,48.1597570333862,-14.2195188100198));
#33938=CARTESIAN_POINT('Ctrl Pts',(14.3528169182251,49.980884503456,-14.2201291128084));
#33939=CARTESIAN_POINT('Ctrl Pts',(9.50149509066547,36.5850719698904,1.04083408558608E-14));
#33940=CARTESIAN_POINT('Ctrl Pts',(9.38007537755078,36.6214111051439,-1.86858636168712));
#33941=CARTESIAN_POINT('Ctrl Pts',(9.36705556810076,37.0055036281238,-3.71029995871695));
#33942=CARTESIAN_POINT('Ctrl Pts',(9.52533731119055,38.4518973636396,-7.16936247491812));
#33943=CARTESIAN_POINT('Ctrl Pts',(9.70422705225135,39.4923472214804,-8.73699595765307));
#33944=CARTESIAN_POINT('Ctrl Pts',(9.98061312163222,40.924980759688,-10.189085676353));
#33945=CARTESIAN_POINT('Ctrl Pts',(10.0068973767326,41.0597112354387,-10.320392863522));
#33946=CARTESIAN_POINT('Ctrl Pts',(10.0339108358286,41.1968114627961,-10.4488603766063));
#33947=CARTESIAN_POINT('Ctrl Pts',(11.7862169042735,35.9142171164209,-6.66133814775094E-16));
#33948=CARTESIAN_POINT('Ctrl Pts',(11.664425345244,35.9492898606342,-1.86860431091527));
#33949=CARTESIAN_POINT('Ctrl Pts',(11.652169660341,36.335984374051,-3.70979114470996));
#33950=CARTESIAN_POINT('Ctrl Pts',(11.8095985064428,37.7794742164015,-7.17014261468561));
#33951=CARTESIAN_POINT('Ctrl Pts',(11.9890114302846,38.8217053622519,-8.73670574474104));
#33952=CARTESIAN_POINT('Ctrl Pts',(12.2667035909977,40.2612951155291,-10.1966053555703));
#33953=CARTESIAN_POINT('Ctrl Pts',(12.2944800077272,40.4035980344044,-10.3350231942244));
#33954=CARTESIAN_POINT('Ctrl Pts',(12.3230698431103,40.5485470057436,-10.470255845095));
#33955=CARTESIAN_POINT('Ctrl Pts',(9.34279883641518,43.6145083358835,1.24689082988549));
#33956=CARTESIAN_POINT('Ctrl Pts',(9.29352897570236,43.6025047583975,0.764254661684727));
#33957=CARTESIAN_POINT('Ctrl Pts',(9.24710292815239,43.5898343019112,0.33294867115195));
#33958=CARTESIAN_POINT('Ctrl Pts',(9.08959664351103,43.6387527331524,-0.978870002773219));
#33959=CARTESIAN_POINT('Ctrl Pts',(9.02147253455122,43.8630440976867,-1.98783577090387));
#33960=CARTESIAN_POINT('Ctrl Pts',(8.99867539150743,44.6599232717994,-3.80852727282109));
#33961=CARTESIAN_POINT('Ctrl Pts',(9.03489241262212,45.2360569808332,-4.65544360715076));
#33962=CARTESIAN_POINT('Ctrl Pts',(9.18984064595293,46.6460662566343,-6.04997283350261));
#33963=CARTESIAN_POINT('Ctrl Pts',(9.30516165133522,47.4916031396421,-6.61832169903423));
#33964=CARTESIAN_POINT('Ctrl Pts',(9.58273633532526,49.3114553051003,-7.3676840307824));
#33965=CARTESIAN_POINT('Ctrl Pts',(9.74382459487429,50.3172192201186,-7.57138648675638));
#33966=CARTESIAN_POINT('Ctrl Pts',(9.90091582292632,51.2881489781559,-7.56962581969435));
#33967=CARTESIAN_POINT('Ctrl Pts',(9.90389776310351,41.3128793157232,1.35489321026558));
#33968=CARTESIAN_POINT('Ctrl Pts',(9.85585276553219,41.3011741506697,0.884255518279171));
#33969=CARTESIAN_POINT('Ctrl Pts',(9.80727935893699,41.2854482448526,0.426396949032127));
#33970=CARTESIAN_POINT('Ctrl Pts',(9.64806121734291,41.3339507669448,-1.25360819503341));
#33971=CARTESIAN_POINT('Ctrl Pts',(9.59710950758293,41.6081209010766,-2.51960912781136));
#33972=CARTESIAN_POINT('Ctrl Pts',(9.63005248744851,42.6049670390508,-4.84647586780943));
#33973=CARTESIAN_POINT('Ctrl Pts',(9.71043261804921,43.3248419422994,-5.91572199041364));
#33974=CARTESIAN_POINT('Ctrl Pts',(9.97242546010331,45.1023943639113,-7.69376028697345));
#33975=CARTESIAN_POINT('Ctrl Pts',(10.1524895065065,46.1617613376918,-8.41063186557115));
#33976=CARTESIAN_POINT('Ctrl Pts',(10.56957751668,48.4668856266258,-9.37059840619505));
#33977=CARTESIAN_POINT('Ctrl Pts',(10.8058013195624,49.72048964759,-9.62435378622801));
#33978=CARTESIAN_POINT('Ctrl Pts',(11.0389609452146,50.9539676685888,-9.62320046360545));
#33979=CARTESIAN_POINT('Ctrl Pts',(10.004740405144,38.9464705831154,1.47293192394307));
#33980=CARTESIAN_POINT('Ctrl Pts',(9.95803136027274,38.9350908951691,1.01538091585011));
#33981=CARTESIAN_POINT('Ctrl Pts',(9.90712214456362,38.9160550470416,0.528580717858437));
#33982=CARTESIAN_POINT('Ctrl Pts',(9.74614391856815,38.9644836024815,-1.55402875453983));
#33983=CARTESIAN_POINT('Ctrl Pts',(9.71379866054205,39.2926120042599,-3.10121432125187));
#33984=CARTESIAN_POINT('Ctrl Pts',(9.80788452009142,40.5087724506632,-5.98129145449219));
#33985=CARTESIAN_POINT('Ctrl Pts',(9.93643935032803,41.3854277882792,-7.29389406570713));
#33986=CARTESIAN_POINT('Ctrl Pts',(10.3155272531748,43.5650308735924,-9.49113593809946));
#33987=CARTESIAN_POINT('Ctrl Pts',(10.5663179729254,44.857983304954,-10.3708286017267));
#33988=CARTESIAN_POINT('Ctrl Pts',(11.1360404748616,47.694013608684,-11.5604045561154));
#33989=CARTESIAN_POINT('Ctrl Pts',(11.4544007679174,49.218441785495,-11.8694761541142));
#33990=CARTESIAN_POINT('Ctrl Pts',(11.7707281089612,50.7390783576437,-11.8687142284812));
#33991=CARTESIAN_POINT('Ctrl Pts',(9.64145132693361,36.6062244663074,1.59647068126639));
#33992=CARTESIAN_POINT('Ctrl Pts',(9.59613798296502,36.5951848118766,1.15259163662228));
#33993=CARTESIAN_POINT('Ctrl Pts',(9.5427942744372,36.5727117312896,0.63557300182231));
#33994=CARTESIAN_POINT('Ctrl Pts',(9.38007537755078,36.6214111051439,-1.86858636168713));
#33995=CARTESIAN_POINT('Ctrl Pts',(9.36705556810076,37.0055036281238,-3.71029995871696));
#33996=CARTESIAN_POINT('Ctrl Pts',(9.52533731119055,38.4518973636396,-7.16936247491812));
#33997=CARTESIAN_POINT('Ctrl Pts',(9.70422705225135,39.4923472214804,-8.73699595765307));
#33998=CARTESIAN_POINT('Ctrl Pts',(10.2059604433751,42.0930574706355,-11.3730256982666));
#33999=CARTESIAN_POINT('Ctrl Pts',(10.5307434056679,43.6303739147712,-12.4235805192466));
#34000=CARTESIAN_POINT('Ctrl Pts',(11.2603557414027,47.0225411281197,-13.8529470821357));
#34001=CARTESIAN_POINT('Ctrl Pts',(11.6646867918773,48.8303727109994,-14.2204718556643));
#34002=CARTESIAN_POINT('Ctrl Pts',(12.0680951184149,50.6517393542017,-14.2198708430667));
#34003=CARTESIAN_POINT('Ctrl Pts',(11.9263392248006,35.9359355586898,1.59674363861582));
#34004=CARTESIAN_POINT('Ctrl Pts',(11.881041157038,35.9248996259739,1.1530142361046));
#34005=CARTESIAN_POINT('Ctrl Pts',(11.8276425661301,35.9022876226716,0.635579106996277));
#34006=CARTESIAN_POINT('Ctrl Pts',(11.664425345244,35.9492898606342,-1.86860431091527));
#34007=CARTESIAN_POINT('Ctrl Pts',(11.652169660341,36.335984374051,-3.70979114470996));
#34008=CARTESIAN_POINT('Ctrl Pts',(11.8095985064428,37.7794742164015,-7.17014261468561));
#34009=CARTESIAN_POINT('Ctrl Pts',(11.9890114302846,38.8217053622519,-8.73670574474104));
#34010=CARTESIAN_POINT('Ctrl Pts',(12.4905558028067,41.4217720607234,-11.373454410524));
#34011=CARTESIAN_POINT('Ctrl Pts',(12.8156483043377,42.9601423694015,-12.422171495837));
#34012=CARTESIAN_POINT('Ctrl Pts',(13.544915286834,46.3511338849317,-13.8545909095487));
#34013=CARTESIAN_POINT('Ctrl Pts',(13.9494605087747,48.1597570333862,-14.2195188100198));
#34014=CARTESIAN_POINT('Ctrl Pts',(14.3528169182251,49.980884503456,-14.2201291128084));
#34015=CARTESIAN_POINT('Ctrl Pts',(12.884908023969,38.1015519292155,1.47327599461714));
#34016=CARTESIAN_POINT('Ctrl Pts',(12.8382182352008,38.0901769325995,1.01591361478258));
#34017=CARTESIAN_POINT('Ctrl Pts',(12.7872398386552,38.0709659683536,0.528588413607706));
#34018=CARTESIAN_POINT('Ctrl Pts',(12.6256334607693,38.1172552346519,-1.5540513800637));
#34019=CARTESIAN_POINT('Ctrl Pts',(12.5942514039498,38.4486635210362,-3.10057294640495));
#34020=CARTESIAN_POINT('Ctrl Pts',(12.687262162052,39.6611635256693,-5.98227484334785));
#34021=CARTESIAN_POINT('Ctrl Pts',(12.8164764793945,40.5400642286032,-7.29352824390238));
#34022=CARTESIAN_POINT('Ctrl Pts',(13.1953261187963,42.7188560995912,-9.4916763423553));
#34023=CARTESIAN_POINT('Ctrl Pts',(13.4465070217538,44.0131369578426,-10.3690524867682));
#34024=CARTESIAN_POINT('Ctrl Pts',(14.0157941958988,46.8476852602796,-11.5624766483461));
#34025=CARTESIAN_POINT('Ctrl Pts',(14.334420449299,48.3731128199111,-11.8682745706068));
#34026=CARTESIAN_POINT('Ctrl Pts',(14.6506863563569,49.8934463159785,-11.8690397849987));
#34027=CARTESIAN_POINT('Ctrl Pts',(14.2481859850623,40.0384499621469,1.35541218776088));
#34028=CARTESIAN_POINT('Ctrl Pts',(14.2001700323452,40.0267518732536,0.885059012382522));
#34029=CARTESIAN_POINT('Ctrl Pts',(14.1514922771427,40.0107618317912,0.426408556881842));
#34030=CARTESIAN_POINT('Ctrl Pts',(13.9913266653942,40.0560375664774,-1.25364232214331));
#34031=CARTESIAN_POINT('Ctrl Pts',(13.9418277959592,40.3351549001892,-2.51864171286796));
#34032=CARTESIAN_POINT('Ctrl Pts',(13.9731491512604,41.3264798268487,-4.847959158086));
#34033=CARTESIAN_POINT('Ctrl Pts',(14.0545240163496,42.0497415170473,-5.91517020468957));
#34034=CARTESIAN_POINT('Ctrl Pts',(14.3161574747839,43.8260703470736,-7.69457540337348));
#34035=CARTESIAN_POINT('Ctrl Pts',(14.496810052318,44.8874410477419,-8.40795287034439));
#34036=CARTESIAN_POINT('Ctrl Pts',(14.9132414377212,47.1903299665148,-9.37372383744498));
#34037=CARTESIAN_POINT('Ctrl Pts',(15.1498577118613,48.4454445415257,-9.62254086010132));
#34038=CARTESIAN_POINT('Ctrl Pts',(15.3829333626944,49.678462279699,-9.62369151535379));
#34039=CARTESIAN_POINT('Ctrl Pts',(15.9637816213007,41.6721936506076,1.24768178593782));
#34040=CARTESIAN_POINT('Ctrl Pts',(15.9145560268702,41.6602008576429,0.765479239879168));
#34041=CARTESIAN_POINT('Ctrl Pts',(15.867970945133,41.6471278409651,0.332966362283221));
#34042=CARTESIAN_POINT('Ctrl Pts',(15.7090206532706,41.6911284346328,-0.978922014747478));
#34043=CARTESIAN_POINT('Ctrl Pts',(15.6431107691165,41.9229596587602,-1.98636136649785));
#34044=CARTESIAN_POINT('Ctrl Pts',(15.617842162917,42.7114241414042,-3.81078790537901));
#34045=CARTESIAN_POINT('Ctrl Pts',(15.6555752252284,43.2927195379046,-4.6546026491858));
#34046=CARTESIAN_POINT('Ctrl Pts',(15.8099757341297,44.700863979149,-6.05121512484675));
#34047=CARTESIAN_POINT('Ctrl Pts',(15.9261936999128,45.5494546745556,-6.6142387329828));
#34048=CARTESIAN_POINT('Ctrl Pts',(16.2027676442909,47.3658999879282,-7.37244739488131));
#34049=CARTESIAN_POINT('Ctrl Pts',(16.3644346256526,48.373972139694,-7.568622301862));
#34050=CARTESIAN_POINT('Ctrl Pts',(16.5214173008838,49.3441943438429,-7.57037421505997));
#34051=CARTESIAN_POINT('Ctrl Pts',(14.7529241788871,34.8615042977019,1.59647077610305));
#34052=CARTESIAN_POINT('Ctrl Pts',(14.7414705295773,34.8603993451984,1.48695587718898));
#34053=CARTESIAN_POINT('Ctrl Pts',(14.7300185573965,34.8592949433739,1.37746402257732));
#34054=CARTESIAN_POINT('Ctrl Pts',(14.6812048800314,34.8545841497086,0.910698635115021));
#34055=CARTESIAN_POINT('Ctrl Pts',(14.6413232655056,34.8466226370598,0.486448413022977));
#34056=CARTESIAN_POINT('Ctrl Pts',(14.4963699339431,34.9137340334406,-1.86858636180158));
#34057=CARTESIAN_POINT('Ctrl Pts',(14.5381447126007,35.295769960475,-3.71029995870877));
#34058=CARTESIAN_POINT('Ctrl Pts',(14.9006586664256,36.7049156525685,-7.1693624749265));
#34059=CARTESIAN_POINT('Ctrl Pts',(15.2257990211744,37.7093165664604,-8.73699595770112));
#34060=CARTESIAN_POINT('Ctrl Pts',(16.092545148085,40.2121512288987,-11.3730256982186));
#34061=CARTESIAN_POINT('Ctrl Pts',(16.6328052294138,41.6875985734161,-12.4235805192612));
#34062=CARTESIAN_POINT('Ctrl Pts',(17.8377468918407,44.9414037541357,-13.852947082121));
#34063=CARTESIAN_POINT('Ctrl Pts',(18.4952436947549,46.6732919100289,-14.2204718556643));
#34064=CARTESIAN_POINT('Ctrl Pts',(19.1537534053194,48.4187086763094,-14.2198708430666));
#34065=CARTESIAN_POINT('Ctrl Pts',(15.1415840475454,33.9925722540019,1.62964621771062));
#34066=CARTESIAN_POINT('Ctrl Pts',(15.1301302752951,33.9914672896363,1.52013014329455));
#34067=CARTESIAN_POINT('Ctrl Pts',(15.1186784705797,33.9903629797961,1.41064104113887));
#34068=CARTESIAN_POINT('Ctrl Pts',(15.0698646034485,33.985651844648,0.943868932657884));
#34069=CARTESIAN_POINT('Ctrl Pts',(15.0295355352143,33.9768575866064,0.50839229845091));
#34070=CARTESIAN_POINT('Ctrl Pts',(14.8839745453764,34.0436978384353,-1.95287905129925));
#34071=CARTESIAN_POINT('Ctrl Pts',(14.9333078250828,34.440494072426,-3.873373870797));
#34072=CARTESIAN_POINT('Ctrl Pts',(15.3212948555137,35.9075266005885,-7.48792130212892));
#34073=CARTESIAN_POINT('Ctrl Pts',(15.666236188169,36.9538988571697,-9.12360836230967));
#34074=CARTESIAN_POINT('Ctrl Pts',(16.5814962694078,39.5635848921074,-11.8774049927216));
#34075=CARTESIAN_POINT('Ctrl Pts',(17.1508209099836,41.1012880288429,-12.9732563609015));
#34076=CARTESIAN_POINT('Ctrl Pts',(18.4192429934717,44.4962044520163,-14.4676858045334));
#34077=CARTESIAN_POINT('Ctrl Pts',(19.1104364369632,46.3001798643402,-14.8501851004961));
#34078=CARTESIAN_POINT('Ctrl Pts',(19.8034868749641,48.1219785107276,-14.8499483202528));
#34079=CARTESIAN_POINT('Ctrl Pts',(16.0080796379931,33.597116340133,1.62975540065037));
#34080=CARTESIAN_POINT('Ctrl Pts',(15.9966258649005,33.5960113756869,1.52023931818545));
#34081=CARTESIAN_POINT('Ctrl Pts',(15.9851740659138,33.5949070766372,1.41075023429468));
#34082=CARTESIAN_POINT('Ctrl Pts',(15.9363601779561,33.5901958958426,0.943978082272566));
#34083=CARTESIAN_POINT('Ctrl Pts',(15.8959902453333,33.5813120719146,0.508394167536556));
#34084=CARTESIAN_POINT('Ctrl Pts',(15.750152846408,33.6475470722109,-1.9528862309875));
#34085=CARTESIAN_POINT('Ctrl Pts',(15.7999367855882,34.0453300100471,-3.87317034519758));
#34086=CARTESIAN_POINT('Ctrl Pts',(16.1874208229068,35.5112613559129,-7.48823335803259));
#34087=CARTESIAN_POINT('Ctrl Pts',(16.5326707000659,36.5583090926536,-9.12349227712147));
#34088=CARTESIAN_POINT('Ctrl Pts',(17.4478193086935,39.1677510875088,-11.877576477648));
#34089=CARTESIAN_POINT('Ctrl Pts',(18.0173264969392,40.7058538585587,-12.9726927515291));
#34090=CARTESIAN_POINT('Ctrl Pts',(19.2855449175038,44.100324448888,-14.4683433355072));
#34091=CARTESIAN_POINT('Ctrl Pts',(19.9768684693761,45.9046009234835,-14.8498038984958));
#34092=CARTESIAN_POINT('Ctrl Pts',(20.6698844856026,47.7263079790887,-14.8500516281495));
#34093=CARTESIAN_POINT('Ctrl Pts',(16.9191631550062,33.8728645130296,1.59674373345244));
#34094=CARTESIAN_POINT('Ctrl Pts',(16.9077095035907,33.8717595603211,1.48722881441631));
#34095=CARTESIAN_POINT('Ctrl Pts',(16.8962575457316,33.8706551854753,1.37773700546685));
#34096=CARTESIAN_POINT('Ctrl Pts',(16.8474438163014,33.8659442776997,0.910971509151797));
#34097=CARTESIAN_POINT('Ctrl Pts',(16.8074600408045,33.8577588503297,0.486453085737103));
#34098=CARTESIAN_POINT('Ctrl Pts',(16.6618156865167,33.923357117882,-1.8686043110222));
#34099=CARTESIAN_POINT('Ctrl Pts',(16.7047171138624,34.3078598045423,-3.70979114471382));
#34100=CARTESIAN_POINT('Ctrl Pts',(17.06597358491,35.714252540865,-7.17014261468207));
#34101=CARTESIAN_POINT('Ctrl Pts',(17.3918853009178,36.7203421551748,-8.73670574472941));
#34102=CARTESIAN_POINT('Ctrl Pts',(18.2583527462983,39.2225667173974,-11.3734544105359));
#34103=CARTESIAN_POINT('Ctrl Pts',(18.7990691968002,40.6990131476935,-12.422171495823));
#34104=CARTESIAN_POINT('Ctrl Pts',(20.0035017019234,43.951703746327,-13.8545909095629));
#34105=CARTESIAN_POINT('Ctrl Pts',(20.6613231478903,45.6843449310794,-14.2195188099295));
#34106=CARTESIAN_POINT('Ctrl Pts',(21.3197474319156,47.4295323472121,-14.2201291128084));
#34107=CARTESIAN_POINT('Ctrl Pts',(14.6113821712786,34.8604849513722,0.));
#34108=CARTESIAN_POINT('Ctrl Pts',(14.4963699339431,34.9137340334406,-1.86858636180158));
#34109=CARTESIAN_POINT('Ctrl Pts',(14.5381447126019,35.295769960475,-3.71029995870877));
#34110=CARTESIAN_POINT('Ctrl Pts',(14.9006586664244,36.7049156525685,-7.16936247492651));
#34111=CARTESIAN_POINT('Ctrl Pts',(15.2257990211768,37.7093165664651,-8.73699595770352));
#34112=CARTESIAN_POINT('Ctrl Pts',(15.7032568890503,39.0880341222379,-10.1890856763496));
#34113=CARTESIAN_POINT('Ctrl Pts',(15.7484477541909,39.2176525965029,-10.3203928635164));
#34114=CARTESIAN_POINT('Ctrl Pts',(15.7946976519012,39.3495129251702,-10.4488603765994));
#34115=CARTESIAN_POINT('Ctrl Pts',(16.7773762106053,33.8713086176789,-4.87766425512972E-9));
#34116=CARTESIAN_POINT('Ctrl Pts',(16.6618156863912,33.9233571184906,-1.86860431424824));
#34117=CARTESIAN_POINT('Ctrl Pts',(16.7047171138587,34.3078598051085,-3.7097911462516));
#34118=CARTESIAN_POINT('Ctrl Pts',(16.8853453492635,35.0110561726706,-5.43996687972851));
#34119=CARTESIAN_POINT('Ctrl Pts',(17.065973584826,35.7142525408467,-7.17014261471587));
#34120=CARTESIAN_POINT('Ctrl Pts',(17.3918853008714,36.7203421551681,-8.73670574475316));
#34121=CARTESIAN_POINT('Ctrl Pts',(17.8251190235963,37.9714544362846,-10.0550800776389));
#34122=CARTESIAN_POINT('Ctrl Pts',(17.8716259385837,38.1057592455494,-10.1966053555778));
#34123=CARTESIAN_POINT('Ctrl Pts',(17.9193714483196,38.2426607296427,-10.3350231942325));
#34124=CARTESIAN_POINT('Ctrl Pts',(17.9682986698117,38.3820655716568,-10.4702558451031));
#34125=CARTESIAN_POINT('Ctrl Pts',(15.4546943255724,41.8409566234847,1.24689092472248));
#34126=CARTESIAN_POINT('Ctrl Pts',(15.4432419692995,41.8398517957221,1.13738838925848));
#34127=CARTESIAN_POINT('Ctrl Pts',(15.4317882611895,41.8387464827965,1.02786758221446));
#34128=CARTESIAN_POINT('Ctrl Pts',(15.382976471443,41.8340390406186,0.561172897424529));
#34129=CARTESIAN_POINT('Ctrl Pts',(15.347591406502,41.8343710194829,0.25482887444235));
#34130=CARTESIAN_POINT('Ctrl Pts',(15.2075196934412,41.9009886759109,-0.978870002714429));
#34131=CARTESIAN_POINT('Ctrl Pts',(15.1720089790472,42.1326921493308,-1.98783577087912));
#34132=CARTESIAN_POINT('Ctrl Pts',(15.2628516086919,42.9247046141549,-3.80852727284543));
#34133=CARTESIAN_POINT('Ctrl Pts',(15.3806923683066,43.4898198932174,-4.65544360724633));
#34134=CARTESIAN_POINT('Ctrl Pts',(15.7347286943739,44.8634258749693,-6.04997283340658));
#34135=CARTESIAN_POINT('Ctrl Pts',(15.9692083427511,45.6839445213788,-6.61832169907737));
#34136=CARTESIAN_POINT('Ctrl Pts',(16.5029496834282,47.4457702195862,-7.36768403073895));
#34137=CARTESIAN_POINT('Ctrl Pts',(16.8055334254904,48.4183716585177,-7.57138648686101));
#34138=CARTESIAN_POINT('Ctrl Pts',(17.0992034029532,49.3570623388651,-7.5696258196942));
#34139=CARTESIAN_POINT('Ctrl Pts',(15.6825261124558,39.4829021650676,1.35489330510245));
#34140=CARTESIAN_POINT('Ctrl Pts',(15.6710733564754,39.4817972987448,1.24538694781347));
#34141=CARTESIAN_POINT('Ctrl Pts',(15.6596201873396,39.4806922726925,1.13587509032859));
#34142=CARTESIAN_POINT('Ctrl Pts',(15.6108078040348,39.4759837721979,0.669158551002801));
#34143=CARTESIAN_POINT('Ctrl Pts',(15.5740132903312,39.47370886399,0.326351368868663));
#34144=CARTESIAN_POINT('Ctrl Pts',(15.4322923840901,39.5401684749661,-1.25360819502657));
#34145=CARTESIAN_POINT('Ctrl Pts',(15.4208777676068,39.8187991368093,-2.51960912779614));
#34146=CARTESIAN_POINT('Ctrl Pts',(15.5953514322868,40.8008105435563,-4.84647586782445));
#34147=CARTESIAN_POINT('Ctrl Pts',(15.777362289462,41.501918872964,-5.91572199048063));
#34148=CARTESIAN_POINT('Ctrl Pts',(16.2896605076648,43.2240929050472,-7.69376028690621));
#34149=CARTESIAN_POINT('Ctrl Pts',(16.6186554011661,44.247051264828,-8.41063186560482));
#34150=CARTESIAN_POINT('Ctrl Pts',(17.3595514472245,46.4693548995415,-9.37059840616123));
#34151=CARTESIAN_POINT('Ctrl Pts',(17.7717772858494,47.6765808867826,-9.62435378627074));
#34152=CARTESIAN_POINT('Ctrl Pts',(18.178105907797,48.8643218056537,-9.62320046360536));
#34153=CARTESIAN_POINT('Ctrl Pts',(15.445567245734,37.1262286569851,1.47293201877982));
#34154=CARTESIAN_POINT('Ctrl Pts',(15.4341140531483,37.1251237485405,1.36342148686314));
#34155=CARTESIAN_POINT('Ctrl Pts',(15.4226614701644,37.1240190301314,1.25391940542181));
#34156=CARTESIAN_POINT('Ctrl Pts',(15.3738484494878,37.1193093979778,0.787178992716546));
#34157=CARTESIAN_POINT('Ctrl Pts',(15.3355356362411,37.1142341193648,0.404559744690755));
#34158=CARTESIAN_POINT('Ctrl Pts',(15.192166408545,37.1808604459796,-1.55402875459149));
#34159=CARTESIAN_POINT('Ctrl Pts',(15.2068479190282,37.5102521839538,-3.10121432124018));
#34160=CARTESIAN_POINT('Ctrl Pts',(15.4730537974558,38.7006440566388,-5.98129145450389));
#34161=CARTESIAN_POINT('Ctrl Pts',(15.7250611874973,39.5500810470602,-7.29389406576467));
#34162=CARTESIAN_POINT('Ctrl Pts',(16.410480382612,41.6535490821868,-9.49113593804184));
#34163=CARTESIAN_POINT('Ctrl Pts',(16.8427247306588,42.8976498812959,-10.3708286017556));
#34164=CARTESIAN_POINT('Ctrl Pts',(17.8102574729806,45.6237335200753,-11.5604045560864));
#34165=CARTESIAN_POINT('Ctrl Pts',(18.342326066798,47.0873378224161,-11.869476154138));
#34166=CARTESIAN_POINT('Ctrl Pts',(18.871842799404,48.547478432487,-11.8687142284811));
#34167=CARTESIAN_POINT('Ctrl Pts',(14.7529241788871,34.8615042977019,1.59647077610305));
#34168=CARTESIAN_POINT('Ctrl Pts',(14.7414705295773,34.8603993451984,1.48695587718898));
#34169=CARTESIAN_POINT('Ctrl Pts',(14.7300185573965,34.8592949433739,1.37746402257732));
#34170=CARTESIAN_POINT('Ctrl Pts',(14.6812048800314,34.8545841497086,0.910698635115021));
#34171=CARTESIAN_POINT('Ctrl Pts',(14.6413232655056,34.8466226370598,0.486448413022977));
#34172=CARTESIAN_POINT('Ctrl Pts',(14.4963699339431,34.9137340334406,-1.86858636180158));
#34173=CARTESIAN_POINT('Ctrl Pts',(14.5381447126019,35.295769960475,-3.71029995870877));
#34174=CARTESIAN_POINT('Ctrl Pts',(14.9006586664244,36.7049156525685,-7.16936247492651));
#34175=CARTESIAN_POINT('Ctrl Pts',(15.2257990211768,37.7093165664651,-8.73699595770352));
#34176=CARTESIAN_POINT('Ctrl Pts',(16.0925451480826,40.212151228894,-11.3730256982162));
#34177=CARTESIAN_POINT('Ctrl Pts',(16.6328052294162,41.6875985734161,-12.4235805192612));
#34178=CARTESIAN_POINT('Ctrl Pts',(17.8377468918383,44.9414037541357,-13.852947082121));
#34179=CARTESIAN_POINT('Ctrl Pts',(18.4952436947468,46.6732919100327,-14.2204718556786));
#34180=CARTESIAN_POINT('Ctrl Pts',(19.1537534053194,48.4187086763094,-14.2198708430666));
#34181=CARTESIAN_POINT('Ctrl Pts',(16.9191631550062,33.8728645130296,1.59674373345244));
#34182=CARTESIAN_POINT('Ctrl Pts',(16.9077095035907,33.8717595603211,1.48722881441631));
#34183=CARTESIAN_POINT('Ctrl Pts',(16.8962575457316,33.8706551854753,1.37773700546685));
#34184=CARTESIAN_POINT('Ctrl Pts',(16.8474438163014,33.8659442776997,0.910971509151797));
#34185=CARTESIAN_POINT('Ctrl Pts',(16.8074600408045,33.8577588503297,0.486453085737103));
#34186=CARTESIAN_POINT('Ctrl Pts',(16.6618156865167,33.923357117882,-1.8686043110222));
#34187=CARTESIAN_POINT('Ctrl Pts',(16.7047171138649,34.3078598045423,-3.70979114471382));
#34188=CARTESIAN_POINT('Ctrl Pts',(17.0659735849076,35.714252540865,-7.17014261468207));
#34189=CARTESIAN_POINT('Ctrl Pts',(17.3918853009202,36.7203421551748,-8.73670574472701));
#34190=CARTESIAN_POINT('Ctrl Pts',(18.2583527462959,39.2225667173974,-11.3734544105383));
#34191=CARTESIAN_POINT('Ctrl Pts',(18.7990691968002,40.6990131476983,-12.422171495823));
#34192=CARTESIAN_POINT('Ctrl Pts',(20.0035017019234,43.9517037463222,-13.8545909095629));
#34193=CARTESIAN_POINT('Ctrl Pts',(20.6613231478936,45.6843449310818,-14.2195188099295));
#34194=CARTESIAN_POINT('Ctrl Pts',(21.3197474319156,47.4295323472121,-14.2201291128084));
#34195=CARTESIAN_POINT('Ctrl Pts',(18.1761744494743,35.8800194678369,1.47327608945381));
#34196=CARTESIAN_POINT('Ctrl Pts',(18.1647212542343,35.8789145591374,1.36376553217266));
#34197=CARTESIAN_POINT('Ctrl Pts',(18.1532686893033,35.8778098747331,1.25426350828991));
#34198=CARTESIAN_POINT('Ctrl Pts',(18.1044556029977,35.8731000987367,0.787522958372509));
#34199=CARTESIAN_POINT('Ctrl Pts',(18.0660140128755,35.8677425691122,0.404565634782747));
#34200=CARTESIAN_POINT('Ctrl Pts',(17.9217737309507,35.9324615528443,-1.55405138010588));
#34201=CARTESIAN_POINT('Ctrl Pts',(17.9378754148555,36.2649627130355,-3.10057294640892));
#34202=CARTESIAN_POINT('Ctrl Pts',(18.2024961996828,37.4518844049553,-5.98227484334405));
#34203=CARTESIAN_POINT('Ctrl Pts',(18.4554759130143,38.3034500513362,-7.29352824387394));
#34204=CARTESIAN_POINT('Ctrl Pts',(19.1405438219643,40.4061490374087,-9.49167634238395));
#34205=CARTESIAN_POINT('Ctrl Pts',(19.5733634366175,41.6515092131842,-10.3690524867446));
#34206=CARTESIAN_POINT('Ctrl Pts',(20.5402543713576,44.3761878888422,-11.56247664837));
#34207=CARTESIAN_POINT('Ctrl Pts',(21.0727284454705,45.8407435516782,-11.8682745705118));
#34208=CARTESIAN_POINT('Ctrl Pts',(21.6021412371498,47.3005929134933,-11.8690397849988));
#34209=CARTESIAN_POINT('Ctrl Pts',(19.8012255369165,37.603187989015,1.35541228259764));
#34210=CARTESIAN_POINT('Ctrl Pts',(19.7897727769317,37.6020831223044,1.24590588705036));
#34211=CARTESIAN_POINT('Ctrl Pts',(19.7783196350271,37.6009781475457,1.13639411638362));
#34212=CARTESIAN_POINT('Ctrl Pts',(19.7295071527289,37.5962694300892,0.66967737009454));
#34213=CARTESIAN_POINT('Ctrl Pts',(19.6925183989912,37.5935687898023,0.326360253163144));
#34214=CARTESIAN_POINT('Ctrl Pts',(19.5494836419133,37.6571514684844,-1.25364232212218));
#34215=CARTESIAN_POINT('Ctrl Pts',(19.5402111377983,37.940472213727,-2.51864171287444));
#34216=CARTESIAN_POINT('Ctrl Pts',(19.7122939334821,38.9172493884975,-4.84795915807957));
#34217=CARTESIAN_POINT('Ctrl Pts',(19.8957713902382,39.6215684668099,-5.91517020463239));
#34218=CARTESIAN_POINT('Ctrl Pts',(20.4075397474896,41.3425825071161,-7.69457540343085));
#34219=CARTESIAN_POINT('Ctrl Pts',(20.7374023418622,42.3674404421722,-8.40795287031109));
#34220=CARTESIAN_POINT('Ctrl Pts',(21.4773303202594,44.5876249069278,-9.37372383747847));
#34221=CARTESIAN_POINT('Ctrl Pts',(21.8901596096332,45.7962902185517,-9.62254085996823));
#34222=CARTESIAN_POINT('Ctrl Pts',(22.2963396064214,46.9835874904387,-9.6236915153539));
#34223=CARTESIAN_POINT('Ctrl Pts',(21.7318648520659,38.9761478068776,1.24768188077462));
#34224=CARTESIAN_POINT('Ctrl Pts',(21.7204124896902,38.975042978526,1.13817928700242));
#34225=CARTESIAN_POINT('Ctrl Pts',(21.7089588230816,38.9739377437727,1.02865861227501));
#34226=CARTESIAN_POINT('Ctrl Pts',(21.6601468824651,38.9692299709329,0.561963612059301));
#34227=CARTESIAN_POINT('Ctrl Pts',(21.6244657828545,38.9689131059274,0.254842414695162));
#34228=CARTESIAN_POINT('Ctrl Pts',(21.4823916741561,39.0311461271326,-0.978922014666903));
#34229=CARTESIAN_POINT('Ctrl Pts',(21.4501456807868,39.2699975980546,-1.98636136650924));
#34230=CARTESIAN_POINT('Ctrl Pts',(21.5373444678502,40.0540327469369,-3.81078790536759));
#34231=CARTESIAN_POINT('Ctrl Pts',(21.6574204222861,40.6240414198376,-4.65460264909511));
#34232=CARTESIAN_POINT('Ctrl Pts',(22.0106492052001,41.9958794973213,-6.05121512493767));
#34233=CARTESIAN_POINT('Ctrl Pts',(22.246451287129,42.8192932221962,-6.6142387329399));
#34234=CARTESIAN_POINT('Ctrl Pts',(22.7787172286239,44.5778891651125,-7.37244739492444));
#34235=CARTESIAN_POINT('Ctrl Pts',(23.0822022983367,45.5526929856933,-7.56862230168617));
#34236=CARTESIAN_POINT('Ctrl Pts',(23.3756641324471,46.4906987626548,-7.57037421506013));
#34237=CARTESIAN_POINT('Ctrl Pts',(19.5640700378123,32.4071044310924,1.59647086199746));
#34238=CARTESIAN_POINT('Ctrl Pts',(19.5525757159953,32.407640749801,1.48695593443964));
#34239=CARTESIAN_POINT('Ctrl Pts',(19.541083132609,32.4081773749034,1.37746405122481));
#34240=CARTESIAN_POINT('Ctrl Pts',(19.4920958892454,32.4104614410692,0.910698635070352));
#34241=CARTESIAN_POINT('Ctrl Pts',(19.4514871706788,32.4082567106452,0.486448412994875));
#34242=CARTESIAN_POINT('Ctrl Pts',(19.3175602025089,32.4953140197786,-1.8685863617208));
#34243=CARTESIAN_POINT('Ctrl Pts',(19.4132791554013,32.8675162009675,-3.71029995872154));
#34244=CARTESIAN_POINT('Ctrl Pts',(19.9726455810625,34.2107277071049,-7.16936247491371));
#34245=CARTESIAN_POINT('Ctrl Pts',(20.4374176293853,35.1586329709741,-8.7369959576679));
#34246=CARTESIAN_POINT('Ctrl Pts',(21.6515320408687,37.5126415502708,-11.373025698252));
#34247=CARTESIAN_POINT('Ctrl Pts',(22.3962711035792,38.8961839423097,-12.4235805192226));
#34248=CARTESIAN_POINT('Ctrl Pts',(24.0520129555351,41.9453889999262,-13.8529470821599));
#34249=CARTESIAN_POINT('Ctrl Pts',(24.949290771548,43.5660774805884,-14.2204718555979));
#34250=CARTESIAN_POINT('Ctrl Pts',(25.8494965077559,45.2000127177925,-14.2198708430668));
#34251=CARTESIAN_POINT('Ctrl Pts',(19.8251119861394,31.4917047963493,1.62964630360506));
#34252=CARTESIAN_POINT('Ctrl Pts',(19.8136175409443,31.4922411208174,1.52013020054019));
#34253=CARTESIAN_POINT('Ctrl Pts',(19.8021251364111,31.4927778131311,1.41064106979313));
#34254=CARTESIAN_POINT('Ctrl Pts',(19.7531376566116,31.4950615682937,0.943868932592553));
#34255=CARTESIAN_POINT('Ctrl Pts',(19.7119675267496,31.4920962479327,0.508392298420167));
#34256=CARTESIAN_POINT('Ctrl Pts',(19.5774004974823,31.5789716511435,-1.95287905120954));
#34257=CARTESIAN_POINT('Ctrl Pts',(19.6827016275074,31.9647082138112,-3.87337387080853));
#34258=CARTESIAN_POINT('Ctrl Pts',(20.2755200062621,33.3615921547092,-7.48792130211721));
#34259=CARTESIAN_POINT('Ctrl Pts',(20.7658646319223,34.3482235805455,-9.1236083622931));
#34260=CARTESIAN_POINT('Ctrl Pts',(22.043205731485,36.8010916838837,-11.8774049927381));
#34261=CARTESIAN_POINT('Ctrl Pts',(22.8255734410865,38.2421198758929,-12.9732563608867));
#34262=CARTESIAN_POINT('Ctrl Pts',(24.5642317986417,41.4219656611118,-14.4676858045482));
#34263=CARTESIAN_POINT('Ctrl Pts',(25.5051223581969,43.1092121219442,-14.8501851004724));
#34264=CARTESIAN_POINT('Ctrl Pts',(26.4503875219925,44.8138361237935,-14.8499483202529));
#34265=CARTESIAN_POINT('Ctrl Pts',(20.6265086564333,30.9769588736642,1.62975548654484));
#34266=CARTESIAN_POINT('Ctrl Pts',(20.615014210394,30.9774951981734,1.52023937542784));
#34267=CARTESIAN_POINT('Ctrl Pts',(20.603521813066,30.978031900352,1.41075026295318));
#34268=CARTESIAN_POINT('Ctrl Pts',(20.5545343061555,30.9803156132948,0.943978082193564));
#34269=CARTESIAN_POINT('Ctrl Pts',(20.513310981293,30.9772674543119,0.508394167507573));
#34270=CARTESIAN_POINT('Ctrl Pts',(20.3783842201005,31.0635831036799,-1.95288623090451));
#34271=CARTESIAN_POINT('Ctrl Pts',(20.4842718451503,31.450232191471,-3.87317034520782));
#34272=CARTESIAN_POINT('Ctrl Pts',(21.0764356359399,32.846097741863,-7.48823335802198));
#34273=CARTESIAN_POINT('Ctrl Pts',(21.56718179641,33.8333538619857,-9.1234922771287));
#34274=CARTESIAN_POINT('Ctrl Pts',(22.8443778274949,36.2859962734605,-11.8775764776405));
#34275=CARTESIAN_POINT('Ctrl Pts',(23.6269831005624,37.7273940528029,-12.9726927515381));
#34276=CARTESIAN_POINT('Ctrl Pts',(25.3653764195812,40.906827527409,-14.4683433354979));
#34277=CARTESIAN_POINT('Ctrl Pts',(26.3064386088075,42.5943534697472,-14.8498038985242));
#34278=CARTESIAN_POINT('Ctrl Pts',(27.2516566664772,44.2988917118185,-14.8500516281494));
#34279=CARTESIAN_POINT('Ctrl Pts',(21.5675617135471,31.1202396243797,1.59674381934692));
#34280=CARTESIAN_POINT('Ctrl Pts',(21.5560673896166,31.1207759431929,1.48722887165912));
#34281=CARTESIAN_POINT('Ctrl Pts',(21.5445748242466,31.1213125929552,1.37773703412493));
#34282=CARTESIAN_POINT('Ctrl Pts',(21.4955875131045,31.123596553574,0.91097150907293));
#34283=CARTESIAN_POINT('Ctrl Pts',(21.4548458070374,31.1211847265943,0.486453085713372));
#34284=CARTESIAN_POINT('Ctrl Pts',(21.3200195090543,31.2068426511148,-1.86860431095823));
#34285=CARTESIAN_POINT('Ctrl Pts',(21.4172046995109,31.5813261451026,-3.70979114472278));
#34286=CARTESIAN_POINT('Ctrl Pts',(21.9749346552545,32.9219916750036,-7.17014261467265));
#34287=CARTESIAN_POINT('Ctrl Pts',(22.4407105406093,33.871458674577,-8.73670574475808));
#34288=CARTESIAN_POINT('Ctrl Pts',(23.6544622808885,36.2249030242105,-11.3734544105068));
#34289=CARTESIAN_POINT('Ctrl Pts',(24.3997952522761,37.6093693845942,-12.4221714958608));
#34290=CARTESIAN_POINT('Ctrl Pts',(26.0548745078767,40.6575436656595,-13.8545909095247));
#34291=CARTESIAN_POINT('Ctrl Pts',(26.952580829692,42.2789313088625,-14.2195188100196));
#34292=CARTESIAN_POINT('Ctrl Pts',(27.8526693689676,43.9126516878549,-14.2201291128082));
#34293=CARTESIAN_POINT('Ctrl Pts',(19.4238236466312,32.4262389885811,0.));
#34294=CARTESIAN_POINT('Ctrl Pts',(19.3175602025089,32.4953140197786,-1.8685863617208));
#34295=CARTESIAN_POINT('Ctrl Pts',(19.4132791554013,32.8675162009675,-3.71029995872154));
#34296=CARTESIAN_POINT('Ctrl Pts',(19.9726455810625,34.2107277071049,-7.16936247491372));
#34297=CARTESIAN_POINT('Ctrl Pts',(20.4374176293853,35.1586329709693,-8.73699595766551));
#34298=CARTESIAN_POINT('Ctrl Pts',(21.1062276306836,36.455367830626,-10.1890856763532));
#34299=CARTESIAN_POINT('Ctrl Pts',(21.169405150186,36.5772356450468,-10.3203928635223));
#34300=CARTESIAN_POINT('Ctrl Pts',(21.2339499719776,36.7011717789779,-10.4488603766068));
#34301=CARTESIAN_POINT('Ctrl Pts',(21.4269965197897,31.1388779522826,-4.87765838243573E-9));
#34302=CARTESIAN_POINT('Ctrl Pts',(21.3200195090168,31.2068426517351,-1.86860431418425));
#34303=CARTESIAN_POINT('Ctrl Pts',(21.4172046995881,31.5813261456637,-3.70979114626052));
#34304=CARTESIAN_POINT('Ctrl Pts',(21.6960696772569,32.251658910038,-5.43996687972819));
#34305=CARTESIAN_POINT('Ctrl Pts',(21.9749346551692,32.9219916749975,-7.17014261470629));
#34306=CARTESIAN_POINT('Ctrl Pts',(22.440710540563,33.871458674577,-8.73670574478158));
#34307=CARTESIAN_POINT('Ctrl Pts',(23.0475864107378,35.0481808493939,-10.0550800776383));
#34308=CARTESIAN_POINT('Ctrl Pts',(23.1127335196115,35.1745000052616,-10.1966053555741));
#34309=CARTESIAN_POINT('Ctrl Pts',(23.179476161479,35.3032131351426,-10.3350231942268));
#34310=CARTESIAN_POINT('Ctrl Pts',(23.2477447519554,35.434235967254,-10.4702558450963));
#34311=CARTESIAN_POINT('Ctrl Pts',(21.2519768052529,39.2156436908075,1.24689101061695));
#34312=CARTESIAN_POINT('Ctrl Pts',(21.2404837810657,39.2161799489647,1.13738844654561));
#34313=CARTESIAN_POINT('Ctrl Pts',(21.22898934975,39.2167159192913,1.02786761081392));
#34314=CARTESIAN_POINT('Ctrl Pts',(21.1800044517766,39.2190030341997,0.561172897522604));
#34315=CARTESIAN_POINT('Ctrl Pts',(21.1450268012714,39.2243674537804,0.254828874451871));
#34316=CARTESIAN_POINT('Ctrl Pts',(21.0158614973502,39.3102413217381,-0.978870002765215));
#34317=CARTESIAN_POINT('Ctrl Pts',(21.0136870730547,39.5446400894209,-1.98783577088475));
#34318=CARTESIAN_POINT('Ctrl Pts',(21.2163201816873,40.3156627552368,-3.80852727284064));
#34319=CARTESIAN_POINT('Ctrl Pts',(21.4133857819021,40.8582554869398,-4.65544360715122));
#34320=CARTESIAN_POINT('Ctrl Pts',(21.959303041511,42.1674955178466,-6.04997283350267));
#34321=CARTESIAN_POINT('Ctrl Pts',(22.3081680038698,42.9462925342929,-6.61832169897219));
#34322=CARTESIAN_POINT('Ctrl Pts',(23.0872105663855,44.6142260746892,-7.36768403084516));
#34323=CARTESIAN_POINT('Ctrl Pts',(23.5251300589823,45.5338656769717,-7.57138648667118));
#34324=CARTESIAN_POINT('Ctrl Pts',(23.9494005117261,46.4212082443696,-7.56962581969484));
#34325=CARTESIAN_POINT('Ctrl Pts',(21.141903454163,36.8491669828396,1.35489339099692));
#34326=CARTESIAN_POINT('Ctrl Pts',(21.1304100288482,36.8497032597153,1.24538700508779));
#34327=CARTESIAN_POINT('Ctrl Pts',(21.1189161718497,36.8502394372903,1.13587511894501));
#34328=CARTESIAN_POINT('Ctrl Pts',(21.0699305357382,36.8525255891216,0.669158551049937));
#34329=CARTESIAN_POINT('Ctrl Pts',(21.0331867839281,36.8555102414576,0.326351368867465));
#34330=CARTESIAN_POINT('Ctrl Pts',(20.9023665809823,36.9414623773007,-1.25360819504018));
#34331=CARTESIAN_POINT('Ctrl Pts',(20.9307214263708,37.2188814500163,-2.51960912780411));
#34332=CARTESIAN_POINT('Ctrl Pts',(21.2431739952935,38.1660672052508,-4.84647586781696));
#34333=CARTESIAN_POINT('Ctrl Pts',(21.5231103629303,38.8341364170866,-5.91572199041885));
#34334=CARTESIAN_POINT('Ctrl Pts',(22.2752850426782,40.4658735625663,-7.69376028696859));
#34335=CARTESIAN_POINT('Ctrl Pts',(22.7465133961687,41.4315988262065,-8.41063186553296));
#34336=CARTESIAN_POINT('Ctrl Pts',(23.7961349710495,43.5258421132212,-9.37059840623374));
#34337=CARTESIAN_POINT('Ctrl Pts',(24.3759711162347,44.6621144270458,-9.62435378613789));
#34338=CARTESIAN_POINT('Ctrl Pts',(24.9471970554252,45.7799392638234,-9.62320046360578));
#34339=CARTESIAN_POINT('Ctrl Pts',(20.5719668778723,34.5502037758216,1.47293210467427));
#34340=CARTESIAN_POINT('Ctrl Pts',(20.5604730144019,34.5507400731433,1.36342154412501));
#34341=CARTESIAN_POINT('Ctrl Pts',(20.5489797813727,34.5512764718092,1.25391943405454));
#34342=CARTESIAN_POINT('Ctrl Pts',(20.4999933533187,34.5535615942045,0.787178992715231));
#34343=CARTESIAN_POINT('Ctrl Pts',(20.461348221816,34.5539904564244,0.404559744676866));
#34344=CARTESIAN_POINT('Ctrl Pts',(20.3289202010264,34.6403421915839,-1.55402875456067));
#34345=CARTESIAN_POINT('Ctrl Pts',(20.3903296068372,34.9642917997669,-3.10121432125053));
#34346=CARTESIAN_POINT('Ctrl Pts',(20.8232363200805,36.1046821531124,-5.98129145449374));
#34347=CARTESIAN_POINT('Ctrl Pts',(21.1935661261622,36.9096087088253,-7.29389406572193));
#34348=CARTESIAN_POINT('Ctrl Pts',(22.1713634554357,38.8941211502969,-9.49113593808493));
#34349=CARTESIAN_POINT('Ctrl Pts',(22.7762621832304,40.0640440127247,-10.3708286017076));
#34350=CARTESIAN_POINT('Ctrl Pts',(24.1219089895441,42.6246857849171,-11.5604045561349));
#34351=CARTESIAN_POINT('Ctrl Pts',(24.8568545017351,43.9976714500213,-11.8694761540621));
#34352=CARTESIAN_POINT('Ctrl Pts',(25.5887811923518,45.3675918458115,-11.8687142284814));
#34353=CARTESIAN_POINT('Ctrl Pts',(19.5640700378123,32.4071044310924,1.59647086199746));
#34354=CARTESIAN_POINT('Ctrl Pts',(19.5525757159953,32.407640749801,1.48695593443965));
#34355=CARTESIAN_POINT('Ctrl Pts',(19.541083132609,32.4081773749034,1.37746405122479));
#34356=CARTESIAN_POINT('Ctrl Pts',(19.4920958892454,32.4104614410692,0.910698635070432));
#34357=CARTESIAN_POINT('Ctrl Pts',(19.4514871706788,32.4082567106452,0.486448412994875));
#34358=CARTESIAN_POINT('Ctrl Pts',(19.3175602025089,32.4953140197786,-1.8685863617208));
#34359=CARTESIAN_POINT('Ctrl Pts',(19.4132791554013,32.8675162009675,-3.71029995872154));
#34360=CARTESIAN_POINT('Ctrl Pts',(19.9726455810625,34.2107277071049,-7.16936247491372));
#34361=CARTESIAN_POINT('Ctrl Pts',(20.4374176293853,35.1586329709693,-8.73699595766551));
#34362=CARTESIAN_POINT('Ctrl Pts',(21.6515320408687,37.5126415502755,-11.3730256982544));
#34363=CARTESIAN_POINT('Ctrl Pts',(22.3962711035816,38.8961839423097,-12.4235805192178));
#34364=CARTESIAN_POINT('Ctrl Pts',(24.0520129555327,41.9453889999262,-13.8529470821647));
#34365=CARTESIAN_POINT('Ctrl Pts',(24.9492907715565,43.5660774805847,-14.2204718556122));
#34366=CARTESIAN_POINT('Ctrl Pts',(25.849496507756,45.2000127177926,-14.2198708430668));
#34367=CARTESIAN_POINT('Ctrl Pts',(21.5675617135471,31.1202396243797,1.59674381934692));
#34368=CARTESIAN_POINT('Ctrl Pts',(21.5560673896166,31.1207759431929,1.48722887165912));
#34369=CARTESIAN_POINT('Ctrl Pts',(21.5445748242466,31.1213125929552,1.37773703412493));
#34370=CARTESIAN_POINT('Ctrl Pts',(21.4955875131045,31.123596553574,0.91097150907293));
#34371=CARTESIAN_POINT('Ctrl Pts',(21.4548458070375,31.1211847265943,0.486453085713372));
#34372=CARTESIAN_POINT('Ctrl Pts',(21.3200195090543,31.2068426511148,-1.86860431095823));
#34373=CARTESIAN_POINT('Ctrl Pts',(21.4172046995109,31.5813261451074,-3.70979114472278));
#34374=CARTESIAN_POINT('Ctrl Pts',(21.9749346552545,32.9219916749988,-7.17014261467265));
#34375=CARTESIAN_POINT('Ctrl Pts',(22.440710540607,33.8714586745723,-8.73670574475808));
#34376=CARTESIAN_POINT('Ctrl Pts',(23.6544622808909,36.2249030242152,-11.3734544105068));
#34377=CARTESIAN_POINT('Ctrl Pts',(24.3997952522713,37.609369384599,-12.4221714958608));
#34378=CARTESIAN_POINT('Ctrl Pts',(26.0548745078815,40.6575436656547,-13.8545909095247));
#34379=CARTESIAN_POINT('Ctrl Pts',(26.9525808296926,42.2789313088637,-14.2195188100053));
#34380=CARTESIAN_POINT('Ctrl Pts',(27.8526693689676,43.9126516878549,-14.2201291128082));
#34381=CARTESIAN_POINT('Ctrl Pts',(23.0974263782809,32.9280732767457,1.47327617534837));
#34382=CARTESIAN_POINT('Ctrl Pts',(23.0859325121477,32.9286095741995,1.36376558942454));
#34383=CARTESIAN_POINT('Ctrl Pts',(23.0744393018274,32.9291460039488,1.25426353693597));
#34384=CARTESIAN_POINT('Ctrl Pts',(23.0254527883363,32.9314309933027,0.787522958328138));
#34385=CARTESIAN_POINT('Ctrl Pts',(22.9866400222227,32.9315988042883,0.404565634774376));
#34386=CARTESIAN_POINT('Ctrl Pts',(22.8530783700626,33.0161865744744,-1.55405138009626));
#34387=CARTESIAN_POINT('Ctrl Pts',(22.9163360109425,33.3430118437575,-3.1005729464118));
#34388=CARTESIAN_POINT('Ctrl Pts',(23.3471799062865,34.480192920029,-5.98227484334081));
#34389=CARTESIAN_POINT('Ctrl Pts',(23.7187750781269,35.2870880890085,-7.29352824391455));
#34390=CARTESIAN_POINT('Ctrl Pts',(24.696115249804,37.2708893025804,-9.49167634234292));
#34391=CARTESIAN_POINT('Ctrl Pts',(25.3017626167546,38.4419768539684,-10.369052486792));
#34392=CARTESIAN_POINT('Ctrl Pts',(26.6465742010944,41.0013193023568,-11.5624766483221));
#34393=CARTESIAN_POINT('Ctrl Pts',(27.3820564590451,42.3751889385584,-11.8682745706114));
#34394=CARTESIAN_POINT('Ctrl Pts',(28.1138388177857,43.7448358429351,-11.8690397849985));
#34395=CARTESIAN_POINT('Ctrl Pts',(24.9511692381921,34.4024335442869,1.35541236849225));
#34396=CARTESIAN_POINT('Ctrl Pts',(24.9396758088609,34.4029698213615,1.24590594430949));
#34397=CARTESIAN_POINT('Ctrl Pts',(24.9281819861154,34.4035060458225,1.13639414502018));
#34398=CARTESIAN_POINT('Ctrl Pts',(24.8791962211348,34.4057919969771,0.669677370076627));
#34399=CARTESIAN_POINT('Ctrl Pts',(24.842199618394,34.4083828938322,0.326360253170264));
#34400=CARTESIAN_POINT('Ctrl Pts',(24.7096695075292,34.4916743608159,-1.25364232216775));
#34401=CARTESIAN_POINT('Ctrl Pts',(24.7408121301953,34.7734309243714,-2.5186417128748));
#34402=CARTESIAN_POINT('Ctrl Pts',(25.050153256772,35.7157759805858,-4.84795915807885));
#34403=CARTESIAN_POINT('Ctrl Pts',(25.3319982333083,36.3868145416154,-5.91517020469683));
#34404=CARTESIAN_POINT('Ctrl Pts',(26.0834833614016,38.0174789096184,-7.69457540336587));
#34405=CARTESIAN_POINT('Ctrl Pts',(26.5558409214786,38.9849609267486,-8.40795287038243));
#34406=CARTESIAN_POINT('Ctrl Pts',(27.6042026929608,41.0772443843887,-9.37372383740648));
#34407=CARTESIAN_POINT('Ctrl Pts',(28.1848409838016,42.2148554922686,-9.62254086011052));
#34408=CARTESIAN_POINT('Ctrl Pts',(28.7558566730953,43.3322623493509,-9.62369151535347));
#34409=CARTESIAN_POINT('Ctrl Pts',(27.0575499833001,35.4866599889488,1.2476819666693));
#34410=CARTESIAN_POINT('Ctrl Pts',(27.0460569529913,35.4871962474067,1.13817934426647));
#34411=CARTESIAN_POINT('Ctrl Pts',(27.0345625738794,35.4877322891927,1.02865864090515));
#34412=CARTESIAN_POINT('Ctrl Pts',(26.9855774795026,35.4900190982578,0.561963612058281));
#34413=CARTESIAN_POINT('Ctrl Pts',(26.9502144674433,35.4947834084228,0.254842414717359));
#34414=CARTESIAN_POINT('Ctrl Pts',(26.8184431506756,35.5766022409397,-0.978922014766397));
#34415=CARTESIAN_POINT('Ctrl Pts',(26.8205174834718,35.817611631747,-1.98636136650704));
#34416=CARTESIAN_POINT('Ctrl Pts',(27.0184085480269,36.5812567518629,-3.81078790536934));
#34417=CARTESIAN_POINT('Ctrl Pts',(27.2183829945314,37.128374968267,-4.65460264919051));
#34418=CARTESIAN_POINT('Ctrl Pts',(27.7632493317807,38.4359800153026,-6.05121512484151));
#34419=CARTESIAN_POINT('Ctrl Pts',(28.1138352797144,39.2174544403461,-6.61423873304951));
#34420=CARTESIAN_POINT('Ctrl Pts',(28.8909578184702,40.8824010710446,-7.37244739481389));
#34421=CARTESIAN_POINT('Ctrl Pts',(29.3300828960074,41.8040923654821,-7.56862230188999));
#34422=CARTESIAN_POINT('Ctrl Pts',(29.7540498521219,42.6907866227634,-7.57037421505949));
#34423=CARTESIAN_POINT('Ctrl Pts',(23.9769478445539,29.2929893708796,1.59647090706345));
#34424=CARTESIAN_POINT('Ctrl Pts',(23.9311433314981,29.301771192775,1.15259179090668));
#34425=CARTESIAN_POINT('Ctrl Pts',(23.8732845217093,29.3034887354955,0.635573104324147));
#34426=CARTESIAN_POINT('Ctrl Pts',(23.745500652653,29.4153831213306,-1.86858636177993));
#34427=CARTESIAN_POINT('Ctrl Pts',(23.8932152177665,29.7701745938172,-3.71029995869774));
#34428=CARTESIAN_POINT('Ctrl Pts',(24.6380470281269,31.0201080009988,-7.16936247493752));
#34429=CARTESIAN_POINT('Ctrl Pts',(25.232989351462,31.8922209971783,-8.73699595769178));
#34430=CARTESIAN_POINT('Ctrl Pts',(26.7697561790069,34.0494826673513,-11.373025698228));
#34431=CARTESIAN_POINT('Ctrl Pts',(27.703813483812,35.3129551733154,-12.4235805192707));
#34432=CARTESIAN_POINT('Ctrl Pts',(29.7766493955075,38.0954870863474,-13.8529470821116));
#34433=CARTESIAN_POINT('Ctrl Pts',(30.8954422364859,39.571983347561,-14.2204718557262));
#34434=CARTESIAN_POINT('Ctrl Pts',(32.019018405086,41.061174846415,-14.2198708430667));
#34435=CARTESIAN_POINT('Ctrl Pts',(24.1050578112645,28.3497570418623,1.62964634867101));
#34436=CARTESIAN_POINT('Ctrl Pts',(24.0596354334595,28.3584655992891,1.18947040158512));
#34437=CARTESIAN_POINT('Ctrl Pts',(24.0007720917071,28.359588878909,0.664244065124536));
#34438=CARTESIAN_POINT('Ctrl Pts',(23.8722870320971,28.4713886672015,-1.95287905126951));
#34439=CARTESIAN_POINT('Ctrl Pts',(24.031412384867,28.8382130746775,-3.87337387078473));
#34440=CARTESIAN_POINT('Ctrl Pts',(24.8169940396062,30.1365118993409,-7.48792130214111));
#34441=CARTESIAN_POINT('Ctrl Pts',(25.4427599557747,31.0433175237852,-9.12360836231226));
#34442=CARTESIAN_POINT('Ctrl Pts',(27.0561790920272,33.2894343746957,-11.877404992719));
#34443=CARTESIAN_POINT('Ctrl Pts',(28.0356631207126,34.6044524432662,-12.9732563609014));
#34444=CARTESIAN_POINT('Ctrl Pts',(30.2091636815192,37.5044951006041,-14.4676858045335));
#34445=CARTESIAN_POINT('Ctrl Pts',(31.380597539451,39.0406651371208,-14.8501851005532));
#34446=CARTESIAN_POINT('Ctrl Pts',(32.558834555691,40.5934132658113,-14.8499483202528));
#34447=CARTESIAN_POINT('Ctrl Pts',(24.8250414362346,27.7261998529422,1.62975553161075));
#34448=CARTESIAN_POINT('Ctrl Pts',(24.7796252351451,27.7349072261548,1.18963944140105));
#34449=CARTESIAN_POINT('Ctrl Pts',(24.7207188400682,27.7359890779467,0.664246507192925));
#34450=CARTESIAN_POINT('Ctrl Pts',(24.591770457568,27.8472541630883,-1.9528862309561));
#34451=CARTESIAN_POINT('Ctrl Pts',(24.7516062015319,28.2148983405182,-3.87317034518888));
#34452=CARTESIAN_POINT('Ctrl Pts',(25.5363949990201,29.5122822980524,-7.48823335804114));
#34453=CARTESIAN_POINT('Ctrl Pts',(26.1626472662176,30.419649113926,-9.12349227713835));
#34454=CARTESIAN_POINT('Ctrl Pts',(27.7758906912504,32.6655632155555,-11.877576477631));
#34455=CARTESIAN_POINT('Ctrl Pts',(28.7556624631346,33.9809133008155,-12.9726927515241));
#34456=CARTESIAN_POINT('Ctrl Pts',(30.9288420051759,36.8805855631592,-14.4683433355121));
#34457=CARTESIAN_POINT('Ctrl Pts',(32.1004855202045,38.4170078110479,-14.849803898529));
#34458=CARTESIAN_POINT('Ctrl Pts',(33.2786637049095,39.969677756751,-14.8500516281494));
#34459=CARTESIAN_POINT('Ctrl Pts',(25.7769069069792,27.7340963985794,1.59674386441279));
#34460=CARTESIAN_POINT('Ctrl Pts',(25.731117835711,27.7428752599414,1.15301439044677));
#34461=CARTESIAN_POINT('Ctrl Pts',(25.6731513926117,27.7444892330921,0.63557920949513));
#34462=CARTESIAN_POINT('Ctrl Pts',(25.5442092163314,27.8550468610404,-1.86860431099641));
#34463=CARTESIAN_POINT('Ctrl Pts',(25.6936997594266,28.2118877584239,-3.7097911447099));
#34464=CARTESIAN_POINT('Ctrl Pts',(26.4365494266639,29.4595339977728,-7.1701426146858));
#34465=CARTESIAN_POINT('Ctrl Pts',(27.0327076275608,30.3330499725183,-8.73670574475581));
#34466=CARTESIAN_POINT('Ctrl Pts',(28.5690351770732,32.4898047695127,-11.3734544105093));
#34467=CARTESIAN_POINT('Ctrl Pts',(29.5038118398612,33.7541073171817,-12.4221714958132));
#34468=CARTESIAN_POINT('Ctrl Pts',(31.5758452046551,36.5357132427424,-13.8545909095725));
#34469=CARTESIAN_POINT('Ctrl Pts',(32.6951616911097,38.012840567309,-14.2195188099579));
#34470=CARTESIAN_POINT('Ctrl Pts',(33.8185912781324,39.5018360737641,-14.2201291128083));
#34471=CARTESIAN_POINT('Ctrl Pts',(23.8408520862202,29.3318883095339,0.));
#34472=CARTESIAN_POINT('Ctrl Pts',(23.745500652653,29.4153831213306,-1.86858636177993));
#34473=CARTESIAN_POINT('Ctrl Pts',(23.8932152177665,29.7701745938172,-3.71029995869894));
#34474=CARTESIAN_POINT('Ctrl Pts',(24.6380470281269,31.0201080009988,-7.16936247493632));
#34475=CARTESIAN_POINT('Ctrl Pts',(25.232989351462,31.8922209971783,-8.73699595769657));
#34476=CARTESIAN_POINT('Ctrl Pts',(26.0795364430743,33.0805753785968,-10.1890856763504));
#34477=CARTESIAN_POINT('Ctrl Pts',(26.15941450482,33.1922116559193,-10.3203928635178));
#34478=CARTESIAN_POINT('Ctrl Pts',(26.2409403042474,33.3057006128359,-10.4488603766015));
#34479=CARTESIAN_POINT('Ctrl Pts',(25.6404249706861,27.7725495286735,-4.44089209850063E-16));
#34480=CARTESIAN_POINT('Ctrl Pts',(25.5442092163314,27.8550468610404,-1.86860431099641));
#34481=CARTESIAN_POINT('Ctrl Pts',(25.6936997594266,28.2118877584239,-3.7097911447099));
#34482=CARTESIAN_POINT('Ctrl Pts',(26.4365494266639,29.4595339977728,-7.1701426146858));
#34483=CARTESIAN_POINT('Ctrl Pts',(27.0327076275608,30.3330499725183,-8.73670574475581));
#34484=CARTESIAN_POINT('Ctrl Pts',(27.8833324977841,31.5271893797555,-10.1966053555712));
#34485=CARTESIAN_POINT('Ctrl Pts',(27.9677135840473,31.6450939272834,-10.3350231942261));
#34486=CARTESIAN_POINT('Ctrl Pts',(28.0539337918646,31.7650675024726,-10.4702558450975));
#34487=CARTESIAN_POINT('Ctrl Pts',(26.6166303184858,35.7920133394052,1.246891055683));
#34488=CARTESIAN_POINT('Ctrl Pts',(26.5668264024408,35.8015619425913,0.764254809540097));
#34489=CARTESIAN_POINT('Ctrl Pts',(26.5193322761004,35.8093225655949,0.332948724830185));
#34490=CARTESIAN_POINT('Ctrl Pts',(26.3963809658133,35.9192508155907,-0.978870002769003));
#34491=CARTESIAN_POINT('Ctrl Pts',(26.4275870969047,36.1515731946735,-1.98783577087676));
#34492=CARTESIAN_POINT('Ctrl Pts',(26.73788565842,36.8859102633353,-3.80852727284811));
#34493=CARTESIAN_POINT('Ctrl Pts',(27.010164411852,37.3949348243697,-4.65544360718925));
#34494=CARTESIAN_POINT('Ctrl Pts',(27.7368493043565,38.6131565530536,-6.04997283346413));
#34495=CARTESIAN_POINT('Ctrl Pts',(28.1929976956625,39.33437787813,-6.61832169910145));
#34496=CARTESIAN_POINT('Ctrl Pts',(29.2014824204412,40.8744649436741,-7.36768403071517));
#34497=CARTESIAN_POINT('Ctrl Pts',(29.7658228849981,41.7224214991986,-7.57138648699933));
#34498=CARTESIAN_POINT('Ctrl Pts',(30.3120568904488,42.5403522177283,-7.56962581969453));
#34499=CARTESIAN_POINT('Ctrl Pts',(26.1708926054255,33.4652890233053,1.35489343606293));
#34500=CARTESIAN_POINT('Ctrl Pts',(26.122326829298,33.4746002454361,0.884255668131405));
#34501=CARTESIAN_POINT('Ctrl Pts',(26.071610116799,33.4804735791579,0.426397017785922));
#34502=CARTESIAN_POINT('Ctrl Pts',(25.9469288716926,33.5907346359619,-1.25360819505675));
#34503=CARTESIAN_POINT('Ctrl Pts',(26.0144759561813,33.8612946673471,-2.51960912779128));
#34504=CARTESIAN_POINT('Ctrl Pts',(26.4585467959407,34.754372800441,-4.84647586782949));
#34505=CARTESIAN_POINT('Ctrl Pts',(26.8307099768296,35.3758029321005,-5.91572199044501));
#34506=CARTESIAN_POINT('Ctrl Pts',(27.8074490109455,36.8838857283533,-7.6937602869421));
#34507=CARTESIAN_POINT('Ctrl Pts',(28.4113179738729,37.7727185143267,-8.41063186561923));
#34508=CARTESIAN_POINT('Ctrl Pts',(29.7482978093313,39.6962686996606,-9.37059840614699));
#34509=CARTESIAN_POINT('Ctrl Pts',(30.4839404690741,40.7384561124946,-9.62435378637083));
#34510=CARTESIAN_POINT('Ctrl Pts',(31.2084352127806,41.7636091770244,-9.62320046360557));
#34511=CARTESIAN_POINT('Ctrl Pts',(25.279580584698,31.2708363785843,1.47293214974027));
#34512=CARTESIAN_POINT('Ctrl Pts',(25.232365242191,31.2798886902605,1.01538106787277));
#34513=CARTESIAN_POINT('Ctrl Pts',(25.1781488031011,31.283721524738,0.528580803097958));
#34514=CARTESIAN_POINT('Ctrl Pts',(25.0518358019869,31.3946464646171,-1.55402875459593));
#34515=CARTESIAN_POINT('Ctrl Pts',(25.1587229846854,31.7065592633067,-3.10121432123402));
#34516=CARTESIAN_POINT('Ctrl Pts',(25.7495178005035,32.7737330381764,-5.98129145451011));
#34517=CARTESIAN_POINT('Ctrl Pts',(26.2306311757221,33.5177631757119,-7.29389406574337));
#34518=CARTESIAN_POINT('Ctrl Pts',(27.480901505213,35.3429210732599,-9.4911359380633));
#34519=CARTESIAN_POINT('Ctrl Pts',(28.2461406191471,36.414849743132,-10.3708286017604));
#34520=CARTESIAN_POINT('Ctrl Pts',(29.942508000842,38.7579223667066,-11.5604045560817));
#34521=CARTESIAN_POINT('Ctrl Pts',(30.8653690604319,40.0123393655871,-11.8694761542142));
#34522=CARTESIAN_POINT('Ctrl Pts',(31.7848057921743,41.2641519184869,-11.8687142284813));
#34523=CARTESIAN_POINT('Ctrl Pts',(23.9769478445539,29.2929893708796,1.59647090706345));
#34524=CARTESIAN_POINT('Ctrl Pts',(23.9311433314981,29.301771192775,1.15259179090668));
#34525=CARTESIAN_POINT('Ctrl Pts',(23.8732845217093,29.3034887354955,0.635573104324147));
#34526=CARTESIAN_POINT('Ctrl Pts',(23.7455006526529,29.4153831213306,-1.86858636177993));
#34527=CARTESIAN_POINT('Ctrl Pts',(23.8932152177665,29.7701745938172,-3.71029995869894));
#34528=CARTESIAN_POINT('Ctrl Pts',(24.6380470281269,31.0201080009988,-7.16936247493632));
#34529=CARTESIAN_POINT('Ctrl Pts',(25.232989351462,31.8922209971783,-8.73699595769657));
#34530=CARTESIAN_POINT('Ctrl Pts',(26.7697561790069,34.0494826673513,-11.3730256982232));
#34531=CARTESIAN_POINT('Ctrl Pts',(27.7038134838072,35.3129551733154,-12.423580519266));
#34532=CARTESIAN_POINT('Ctrl Pts',(29.7766493955123,38.0954870863474,-13.8529470821163));
#34533=CARTESIAN_POINT('Ctrl Pts',(30.895442236499,39.5719833475484,-14.220471855731));
#34534=CARTESIAN_POINT('Ctrl Pts',(32.019018405086,41.061174846415,-14.2198708430667));
#34535=CARTESIAN_POINT('Ctrl Pts',(25.7769069069792,27.7340963985794,1.59674386441279));
#34536=CARTESIAN_POINT('Ctrl Pts',(25.731117835711,27.7428752599414,1.15301439044677));
#34537=CARTESIAN_POINT('Ctrl Pts',(25.6731513926117,27.7444892330921,0.63557920949513));
#34538=CARTESIAN_POINT('Ctrl Pts',(25.5442092163314,27.8550468610404,-1.86860431099641));
#34539=CARTESIAN_POINT('Ctrl Pts',(25.6936997594266,28.2118877584239,-3.70979114470751));
#34540=CARTESIAN_POINT('Ctrl Pts',(26.4365494266639,29.4595339977728,-7.1701426146882));
#34541=CARTESIAN_POINT('Ctrl Pts',(27.0327076275608,30.3330499725231,-8.73670574475342));
#34542=CARTESIAN_POINT('Ctrl Pts',(28.5690351770732,32.4898047695079,-11.3734544105117));
#34543=CARTESIAN_POINT('Ctrl Pts',(29.5038118398636,33.7541073171817,-12.422171495818));
#34544=CARTESIAN_POINT('Ctrl Pts',(31.5758452046528,36.5357132427424,-13.8545909095677));
#34545=CARTESIAN_POINT('Ctrl Pts',(32.6951616911013,38.0128405673168,-14.2195188099532));
#34546=CARTESIAN_POINT('Ctrl Pts',(33.8185912781324,39.5018360737641,-14.2201291128083));
#34547=CARTESIAN_POINT('Ctrl Pts',(27.5484813091701,29.3058064687037,1.47327622041421));
#34548=CARTESIAN_POINT('Ctrl Pts',(27.501285431483,29.3148550485427,1.01591376687871));
#34549=CARTESIAN_POINT('Ctrl Pts',(27.4469333174788,29.3185573305647,0.528588498843467));
#34550=CARTESIAN_POINT('Ctrl Pts',(27.3191602364349,29.4277972482694,-1.5540513801051));
#34551=CARTESIAN_POINT('Ctrl Pts',(27.4282860910127,29.7422934066244,-3.10057294640986));
#34552=CARTESIAN_POINT('Ctrl Pts',(28.0165823577943,30.8065841399386,-5.98227484334298));
#34553=CARTESIAN_POINT('Ctrl Pts',(28.4992283820343,31.5523827727542,-7.29352824390031));
#34554=CARTESIAN_POINT('Ctrl Pts',(29.7489449887858,33.3769017419141,-9.49167634235738));
#34555=CARTESIAN_POINT('Ctrl Pts',(30.5150908743753,34.4498767034893,-10.3690524867348));
#34556=CARTESIAN_POINT('Ctrl Pts',(32.2104466223682,36.7917820929403,-11.5624766483796));
#34557=CARTESIAN_POINT('Ctrl Pts',(33.1339647666548,38.0469976785123,-11.8682745705069));
#34558=CARTESIAN_POINT('Ctrl Pts',(34.0532197137074,39.2985600643045,-11.8690397849987));
#34559=CARTESIAN_POINT('Ctrl Pts',(29.5931790826756,30.5013447592648,1.35541241355804));
#34560=CARTESIAN_POINT('Ctrl Pts',(29.5446426662243,30.5106503524935,0.88505916234556));
#34561=CARTESIAN_POINT('Ctrl Pts',(29.4937213090621,30.5163267679927,0.426408625629975));
#34562=CARTESIAN_POINT('Ctrl Pts',(29.3668377587824,30.624046228974,-1.25364232214448));
#34563=CARTESIAN_POINT('Ctrl Pts',(29.437761534203,30.8985028595929,-2.51864171288381));
#34564=CARTESIAN_POINT('Ctrl Pts',(29.8780636984596,31.7872323695978,-4.84795915807006));
#34565=CARTESIAN_POINT('Ctrl Pts',(30.2525386437882,32.4113300033619,-5.91517020466588));
#34566=CARTESIAN_POINT('Ctrl Pts',(31.2284424726404,33.9184490747759,-7.69457540339711));
#34567=CARTESIAN_POINT('Ctrl Pts',(31.8336791606301,34.8088600302697,-8.40795287029653));
#34568=CARTESIAN_POINT('Ctrl Pts',(33.1691331028056,36.7306496231043,-9.37372383749281));
#34569=CARTESIAN_POINT('Ctrl Pts',(33.9057602738327,37.7740480458422,-9.62254085997281));
#34570=CARTESIAN_POINT('Ctrl Pts',(34.6299874229482,38.798817306756,-9.62369151535367));
#34571=CARTESIAN_POINT('Ctrl Pts',(31.8324214200722,31.2747661069636,1.24768201173503));
#34572=CARTESIAN_POINT('Ctrl Pts',(31.7826622501159,31.2843061313282,0.765479387903577));
#34573=CARTESIAN_POINT('Ctrl Pts',(31.7348562317645,31.2917666379315,0.332966415952804));
#34574=CARTESIAN_POINT('Ctrl Pts',(31.6085484626321,31.3978213276647,-0.978922014709456));
#34575=CARTESIAN_POINT('Ctrl Pts',(31.6449008941903,31.6360823818921,-1.98636136652822));
#34576=CARTESIAN_POINT('Ctrl Pts',(31.949455744811,32.3637918611397,-3.81078790534844));
#34577=CARTESIAN_POINT('Ctrl Pts',(32.2252577802499,32.8768818719365,-4.65460264913809));
#34578=CARTESIAN_POINT('Ctrl Pts',(32.9506697646596,34.0936348201821,-6.05121512489433));
#34579=CARTESIAN_POINT('Ctrl Pts',(33.4089026594735,34.8172613800546,-6.61423873291092));
#34580=CARTESIAN_POINT('Ctrl Pts',(34.4150618219131,36.3546651861137,-7.37244739495311));
#34581=CARTESIAN_POINT('Ctrl Pts',(34.9808875866065,37.2044809779791,-7.56862230166205));
#34582=CARTESIAN_POINT('Ctrl Pts',(35.5267289204026,38.0218131772948,-7.57037421505979));
#34583=CARTESIAN_POINT('Ctrl Pts',(27.9017241322581,25.5825535213022,1.59647090706387));
#34584=CARTESIAN_POINT('Ctrl Pts',(27.8576356266577,25.5977646187872,1.15259179090232));
#34585=CARTESIAN_POINT('Ctrl Pts',(27.8006101679621,25.6076988465176,0.635573104328414));
#34586=CARTESIAN_POINT('Ctrl Pts',(27.6900511858084,25.7366398496321,-1.86858636179196));
#34587=CARTESIAN_POINT('Ctrl Pts',(27.8867543207108,26.066798081921,-3.71029995868804));
#34588=CARTESIAN_POINT('Ctrl Pts',(28.8018888878892,27.1980083507072,-7.16936247494692));
#34589=CARTESIAN_POINT('Ctrl Pts',(29.5148901762539,27.9765753734475,-8.73699595770123));
#34590=CARTESIAN_POINT('Ctrl Pts',(31.343025278964,29.8931745079276,-11.3730256982183));
#34591=CARTESIAN_POINT('Ctrl Pts',(32.4473861126917,31.0108564710822,-12.4235805193185));
#34592=CARTESIAN_POINT('Ctrl Pts',(34.8951191225769,33.4700709140672,-13.8529470820634));
#34593=CARTESIAN_POINT('Ctrl Pts',(36.212651592373,34.7723177498292,-14.220471855745));
#34594=CARTESIAN_POINT('Ctrl Pts',(37.5367254229124,36.0864498658149,-14.2198708430665));
#34595=CARTESIAN_POINT('Ctrl Pts',(27.8942941678687,24.6306899881718,1.62964634867146));
#34596=CARTESIAN_POINT('Ctrl Pts',(27.8505734813074,24.6457741833924,1.1894704015781));
#34597=CARTESIAN_POINT('Ctrl Pts',(27.7924691428913,24.6552631565739,0.664244065131922));
#34598=CARTESIAN_POINT('Ctrl Pts',(27.6812026446259,24.7842103148325,-1.9528790512907));
#34599=CARTESIAN_POINT('Ctrl Pts',(27.8909128870511,25.1246550797834,-3.87337387077626));
#34600=CARTESIAN_POINT('Ctrl Pts',(28.853265640495,26.2979391683251,-7.48792130214933));
#34601=CARTESIAN_POINT('Ctrl Pts',(29.6017140577639,27.1064590437666,-9.1236083623074));
#34602=CARTESIAN_POINT('Ctrl Pts',(31.5183666698576,29.1001001804498,-11.8774049927236));
#34603=CARTESIAN_POINT('Ctrl Pts',(32.6750275473655,30.2623381498283,-12.9732563609205));
#34604=CARTESIAN_POINT('Ctrl Pts',(35.2391241078866,32.8235411739476,-14.4676858045142));
#34605=CARTESIAN_POINT('Ctrl Pts',(36.6172542487155,34.1773627941932,-14.8501851005341));
#34606=CARTESIAN_POINT('Ctrl Pts',(38.0044776097607,35.5466255754747,-14.8499483202527));
#34607=CARTESIAN_POINT('Ctrl Pts',(28.518207957172,23.9110153591927,1.62975553161122));
#34608=CARTESIAN_POINT('Ctrl Pts',(28.4744932159205,23.9260975032119,1.18963944139232));
#34609=CARTESIAN_POINT('Ctrl Pts',(28.4163403666156,23.9355515973761,0.664246507202821));
#34610=CARTESIAN_POINT('Ctrl Pts',(28.3045391652058,24.0640354326903,-1.95288623098466));
#34611=CARTESIAN_POINT('Ctrl Pts',(28.5150692335159,24.4051905243397,-3.87317034518165));
#34612=CARTESIAN_POINT('Ctrl Pts',(29.4765070006746,25.5776818931087,-7.48823335804822));
#34613=CARTESIAN_POINT('Ctrl Pts',(30.2255166845004,26.386688032904,-9.12349227711924));
#34614=CARTESIAN_POINT('Ctrl Pts',(32.1419665196151,28.3801534903142,-11.8775764776501));
#34615=CARTESIAN_POINT('Ctrl Pts',(33.2989594624334,29.5426791468127,-12.9726927515002));
#34616=CARTESIAN_POINT('Ctrl Pts',(35.8626855589669,32.1035612317429,-14.4683433355361));
#34617=CARTESIAN_POINT('Ctrl Pts',(37.2410591163412,33.4576026588985,-14.8498038984768));
#34618=CARTESIAN_POINT('Ctrl Pts',(38.628213118051,34.8267964255888,-14.8500516281495));
#34619=CARTESIAN_POINT('Ctrl Pts',(29.4615086055164,23.7833669488543,1.59674386441327));
#34620=CARTESIAN_POINT('Ctrl Pts',(29.4174349631896,23.7985729183272,1.15301439043766));
#34621=CARTESIAN_POINT('Ctrl Pts',(29.3602882272755,23.8084199485255,0.63557920950567));
#34622=CARTESIAN_POINT('Ctrl Pts',(29.248392487251,23.9362026442694,-1.86860431102687));
#34623=CARTESIAN_POINT('Ctrl Pts',(29.447145186874,24.2681366933022,-3.70979114470513));
#34624=CARTESIAN_POINT('Ctrl Pts',(30.3599922883371,25.3973651626758,-7.17014261469054));
#34625=CARTESIAN_POINT('Ctrl Pts',(31.0743967430845,26.1771478462959,-8.73670574472719));
#34626=CARTESIAN_POINT('Ctrl Pts',(32.9020249033686,28.0933077825839,-11.373454410538));
#34627=CARTESIAN_POINT('Ctrl Pts',(34.0072159003542,29.2117089635432,-12.422171495751));
#34628=CARTESIAN_POINT('Ctrl Pts',(36.4540227502848,31.6701210585555,-13.8545909096349));
#34629=CARTESIAN_POINT('Ctrl Pts',(37.7721633453246,32.9729180118925,-14.2195188098725));
#34630=CARTESIAN_POINT('Ctrl Pts',(39.0960641936379,34.2868769911002,-14.2201291128085));
#34631=CARTESIAN_POINT('Ctrl Pts',(27.7725495286739,25.6404249706856,0.));
#34632=CARTESIAN_POINT('Ctrl Pts',(27.6900511858084,25.7366398496321,-1.86858636179196));
#34633=CARTESIAN_POINT('Ctrl Pts',(27.8867543207108,26.066798081921,-3.71029995868804));
#34634=CARTESIAN_POINT('Ctrl Pts',(28.8018888878892,27.1980083507072,-7.16936247494692));
#34635=CARTESIAN_POINT('Ctrl Pts',(29.5148901762515,27.9765753734499,-8.73699595769884));
#34636=CARTESIAN_POINT('Ctrl Pts',(30.5219411006583,29.0323578083609,-10.1890856763493));
#34637=CARTESIAN_POINT('Ctrl Pts',(30.6168936176608,29.1314899559103,-10.3203928635164));
#34638=CARTESIAN_POINT('Ctrl Pts',(30.7137407645493,29.2322214279229,-10.4488603766001));
#34639=CARTESIAN_POINT('Ctrl Pts',(29.3318883095343,23.8408520862197,1.66533453693773E-15));
#34640=CARTESIAN_POINT('Ctrl Pts',(29.248392487251,23.9362026442694,-1.86860431102687));
#34641=CARTESIAN_POINT('Ctrl Pts',(29.447145186874,24.2681366933022,-3.70979114470513));
#34642=CARTESIAN_POINT('Ctrl Pts',(30.3599922883371,25.3973651626758,-7.17014261469054));
#34643=CARTESIAN_POINT('Ctrl Pts',(31.0743967430845,26.1771478462959,-8.73670574472719));
#34644=CARTESIAN_POINT('Ctrl Pts',(32.0863072351869,27.238076095385,-10.1966053555739));
#34645=CARTESIAN_POINT('Ctrl Pts',(32.1866090102694,27.3427718639805,-10.3350231942301));
#34646=CARTESIAN_POINT('Ctrl Pts',(32.2890256406393,27.4492538662307,-10.4702558451018));
#34647=CARTESIAN_POINT('Ctrl Pts',(31.439445989728,31.6397608122765,1.24689105568327));
#34648=CARTESIAN_POINT('Ctrl Pts',(31.3915079136658,31.6563000607303,0.76425480955427));
#34649=CARTESIAN_POINT('Ctrl Pts',(31.3456016608091,31.6707408106671,0.332948724815391));
#34650=CARTESIAN_POINT('Ctrl Pts',(31.2395462388519,31.7970479454231,-0.978870002725275));
#34651=CARTESIAN_POINT('Ctrl Pts',(31.3034976581799,32.0225645221549,-1.98783577087666));
#34652=CARTESIAN_POINT('Ctrl Pts',(31.7151448889925,32.7052670087094,-3.80852727284797));
#34653=CARTESIAN_POINT('Ctrl Pts',(32.057093985311,33.1703611269161,-4.6554436072416));
#34654=CARTESIAN_POINT('Ctrl Pts',(32.9497533017817,34.2727650719351,-6.04997283341119));
#34655=CARTESIAN_POINT('Ctrl Pts',(33.5038992562213,34.9217287193948,-6.61832169924966));
#34656=CARTESIAN_POINT('Ctrl Pts',(34.7212963025802,36.3026175785815,-7.36768403056607));
#34657=CARTESIAN_POINT('Ctrl Pts',(35.4005693947338,37.0616291371886,-7.57138648705115));
#34658=CARTESIAN_POINT('Ctrl Pts',(36.0576472036359,37.7934972961793,-7.56962581969384));
#34659=CARTESIAN_POINT('Ctrl Pts',(30.6671178491337,29.4001542854015,1.35489343606325));
#34660=CARTESIAN_POINT('Ctrl Pts',(30.6203715276499,29.4162823633067,0.884255668139386));
#34661=CARTESIAN_POINT('Ctrl Pts',(30.5710069006797,29.4293136556717,0.42639701777831));
#34662=CARTESIAN_POINT('Ctrl Pts',(30.4632865154137,29.5561964051748,-1.25360819503402));
#34663=CARTESIAN_POINT('Ctrl Pts',(30.5686507750139,29.8143895731083,-2.5196091277888));
#34664=CARTESIAN_POINT('Ctrl Pts',(31.1352998840349,30.6351795888019,-4.84647586783175));
#34665=CARTESIAN_POINT('Ctrl Pts',(31.5921137090151,31.1973201148293,-5.91572199047832));
#34666=CARTESIAN_POINT('Ctrl Pts',(32.773533507375,32.5510483450333,-7.69376028690839));
#34667=CARTESIAN_POINT('Ctrl Pts',(33.4977500490821,33.344894581043,-8.41063186571964));
#34668=CARTESIAN_POINT('Ctrl Pts',(35.0948710912443,35.0585937299385,-9.37059840604598));
#34669=CARTESIAN_POINT('Ctrl Pts',(35.9713447024329,35.9854803114778,-9.62435378637997));
#34670=CARTESIAN_POINT('Ctrl Pts',(36.8343596268993,36.8970924436848,-9.62320046360512));
#34671=CARTESIAN_POINT('Ctrl Pts',(29.4725749263796,27.3548849305452,1.47293214974065));
#34672=CARTESIAN_POINT('Ctrl Pts',(29.4271284462509,27.3705645465863,1.01538106787412));
#34673=CARTESIAN_POINT('Ctrl Pts',(29.3740093215553,27.3820741720646,0.528580803096777));
#34674=CARTESIAN_POINT('Ctrl Pts',(29.2647682695535,27.5098462703966,-1.55402875459203));
#34675=CARTESIAN_POINT('Ctrl Pts',(29.4149573143405,27.8033726143444,-3.10121432122795));
#34676=CARTESIAN_POINT('Ctrl Pts',(30.1516133539766,28.7756052302924,-5.98129145451597));
#34677=CARTESIAN_POINT('Ctrl Pts',(30.7337162174557,29.4435926416019,-7.29389406576238));
#34678=CARTESIAN_POINT('Ctrl Pts',(32.2310076487024,31.0722410437258,-9.49113593804398));
#34679=CARTESIAN_POINT('Ctrl Pts',(33.1410090871746,32.0243541445035,-10.3708286018225));
#34680=CARTESIAN_POINT('Ctrl Pts',(35.153563896332,34.1021594177494,-11.5604045560192));
#34681=CARTESIAN_POINT('Ctrl Pts',(36.2455537133318,35.2124714377622,-11.8694761542139));
#34682=CARTESIAN_POINT('Ctrl Pts',(37.333783405879,36.3206928540896,-11.868714228481));
#34683=CARTESIAN_POINT('Ctrl Pts',(27.9017241322581,25.5825535213022,1.59647090706387));
#34684=CARTESIAN_POINT('Ctrl Pts',(27.8576356266577,25.5977646187872,1.15259179090232));
#34685=CARTESIAN_POINT('Ctrl Pts',(27.8006101679621,25.6076988465176,0.635573104328414));
#34686=CARTESIAN_POINT('Ctrl Pts',(27.6900511858084,25.7366398496321,-1.86858636179196));
#34687=CARTESIAN_POINT('Ctrl Pts',(27.8867543207108,26.066798081921,-3.71029995868804));
#34688=CARTESIAN_POINT('Ctrl Pts',(28.8018888878892,27.1980083507072,-7.16936247494692));
#34689=CARTESIAN_POINT('Ctrl Pts',(29.5148901762515,27.9765753734499,-8.73699595769884));
#34690=CARTESIAN_POINT('Ctrl Pts',(31.3430252789664,29.8931745079252,-11.3730256982207));
#34691=CARTESIAN_POINT('Ctrl Pts',(32.4473861126964,31.0108564710774,-12.4235805193185));
#34692=CARTESIAN_POINT('Ctrl Pts',(34.8951191225721,33.4700709140719,-13.8529470820634));
#34693=CARTESIAN_POINT('Ctrl Pts',(36.212651592373,34.7723177498292,-14.220471855726));
#34694=CARTESIAN_POINT('Ctrl Pts',(37.5367254229124,36.0864498658149,-14.2198708430665));
#34695=CARTESIAN_POINT('Ctrl Pts',(29.4615086055164,23.7833669488543,1.59674386441327));
#34696=CARTESIAN_POINT('Ctrl Pts',(29.4174349631896,23.7985729183272,1.15301439043765));
#34697=CARTESIAN_POINT('Ctrl Pts',(29.3602882272755,23.8084199485255,0.63557920950567));
#34698=CARTESIAN_POINT('Ctrl Pts',(29.248392487251,23.9362026442694,-1.86860431102687));
#34699=CARTESIAN_POINT('Ctrl Pts',(29.447145186874,24.2681366933022,-3.70979114470393));
#34700=CARTESIAN_POINT('Ctrl Pts',(30.3599922883371,25.3973651626758,-7.17014261469174));
#34701=CARTESIAN_POINT('Ctrl Pts',(31.0743967430845,26.1771478463006,-8.7367057447272));
#34702=CARTESIAN_POINT('Ctrl Pts',(32.9020249033686,28.0933077825791,-11.373454410538));
#34703=CARTESIAN_POINT('Ctrl Pts',(34.0072159003542,29.2117089635455,-12.4221714957558));
#34704=CARTESIAN_POINT('Ctrl Pts',(36.4540227502848,31.6701210585531,-13.8545909096301));
#34705=CARTESIAN_POINT('Ctrl Pts',(37.7721633453302,32.9729180118886,-14.2195188098868));
#34706=CARTESIAN_POINT('Ctrl Pts',(39.0960641936379,34.2868769911002,-14.2201291128085));
#34707=CARTESIAN_POINT('Ctrl Pts',(31.4387285991345,25.0869579521467,1.47327622041466));
#34708=CARTESIAN_POINT('Ctrl Pts',(31.3933008545913,25.1026311041785,1.01591376687384));
#34709=CARTESIAN_POINT('Ctrl Pts',(31.3400288564412,25.1140308146322,0.52858849885019));
#34710=CARTESIAN_POINT('Ctrl Pts',(31.2291027822745,25.240342832856,-1.55405138012444));
#34711=CARTESIAN_POINT('Ctrl Pts',(31.3818753629811,25.5361076454315,-3.10057294640994));
#34712=CARTESIAN_POINT('Ctrl Pts',(32.1156479855831,26.5058421456039,-5.98227484334299));
#34713=CARTESIAN_POINT('Ctrl Pts',(32.6995195810716,27.175361932793,-7.29352824387175));
#34714=CARTESIAN_POINT('Ctrl Pts',(34.1961719966689,28.8034567128308,-9.49167634238618));
#34715=CARTESIAN_POINT('Ctrl Pts',(35.1072198800537,29.7564764085591,-10.3690524866583));
#34716=CARTESIAN_POINT('Ctrl Pts',(37.1186072376635,31.8332702988585,-11.5624766484565));
#34717=CARTESIAN_POINT('Ctrl Pts',(38.2113611019924,32.9442792642618,-11.8682745704453));
#34718=CARTESIAN_POINT('Ctrl Pts',(39.2993752576344,34.0522789304535,-11.869039784999));
#34719=CARTESIAN_POINT('Ctrl Pts',(33.6327571359872,25.9793365537797,1.35541241355847));
#34720=CARTESIAN_POINT('Ctrl Pts',(33.5860390742467,25.9954548817286,0.885059162344105));
#34721=CARTESIAN_POINT('Ctrl Pts',(33.5364438612611,26.0083203842444,0.426408625634281));
#34722=CARTESIAN_POINT('Ctrl Pts',(33.4261818802043,26.1330008283034,-1.2536423221568));
#34723=CARTESIAN_POINT('Ctrl Pts',(33.5354430048848,26.3945703805904,-2.51864171288876));
#34724=CARTESIAN_POINT('Ctrl Pts',(34.0977429244508,27.2115923743002,-4.84795915806537));
#34725=CARTESIAN_POINT('Ctrl Pts',(34.5572246086239,27.776044252781,-5.91517020463262));
#34726=CARTESIAN_POINT('Ctrl Pts',(35.7376805505017,29.1289374295172,-7.6945754034308));
#34727=CARTESIAN_POINT('Ctrl Pts',(36.4634754928303,29.9241511240645,-8.40795287018175));
#34728=CARTESIAN_POINT('Ctrl Pts',(38.0588356145493,31.6363247579131,-9.37372383760818));
#34729=CARTESIAN_POINT('Ctrl Pts',(38.9364560608935,32.5642699125464,-9.62254085985904));
#34730=CARTESIAN_POINT('Ctrl Pts',(39.799151493507,33.4755402303452,-9.62369151535412));
#34731=CARTESIAN_POINT('Ctrl Pts',(35.9592765491248,26.4262081762391,1.24768201173545));
#34732=CARTESIAN_POINT('Ctrl Pts',(35.9113815427739,26.4427325651126,0.765479387903452));
#34733=CARTESIAN_POINT('Ctrl Pts',(35.8651238615809,26.4569206403468,0.332966415956187));
#34734=CARTESIAN_POINT('Ctrl Pts',(35.7551948793994,26.5798713158462,-0.97892201471915));
#34735=CARTESIAN_POINT('Ctrl Pts',(35.8250853790549,26.8105337258072,-1.98636136654047));
#34736=CARTESIAN_POINT('Ctrl Pts',(36.2301041572592,27.4874934974547,-3.81078790533667));
#34737=CARTESIAN_POINT('Ctrl Pts',(36.5761192475709,27.9561102697751,-4.6546026490906));
#34738=CARTESIAN_POINT('Ctrl Pts',(37.467309582976,29.0572415380629,-6.05121512494251));
#34739=CARTESIAN_POINT('Ctrl Pts',(38.0238611244248,29.7082892828337,-6.61423873273877));
#34740=CARTESIAN_POINT('Ctrl Pts',(39.2385744114853,31.0868531561125,-7.3724473951262));
#34741=CARTESIAN_POINT('Ctrl Pts',(39.9195822826463,31.8474936466127,-7.56862230151042));
#34742=CARTESIAN_POINT('Ctrl Pts',(40.5761862384902,32.578825261391,-7.57037421506047));
#34743=CARTESIAN_POINT('Ctrl Pts',(31.2585017743465,21.3513306581892,1.59647086199721));
#34744=CARTESIAN_POINT('Ctrl Pts',(31.2170267923954,21.3726613764951,1.15259176008521));
#34745=CARTESIAN_POINT('Ctrl Pts',(31.1619955607637,21.3906100567509,0.635573083900845));
#34746=CARTESIAN_POINT('Ctrl Pts',(31.0709121284139,21.5339728087887,-1.86858636186358));
#34747=CARTESIAN_POINT('Ctrl Pts',(31.312599524452,21.8327767315482,-3.71029995871917));
#34748=CARTESIAN_POINT('Ctrl Pts',(32.3794073476761,22.8222356829394,-7.1693624749162));
#34749=CARTESIAN_POINT('Ctrl Pts',(33.1959529509213,23.4914073529601,-8.73699595768941));
#34750=CARTESIAN_POINT('Ctrl Pts',(35.2782407701143,25.1283275202519,-11.3730256982305));
#34751=CARTESIAN_POINT('Ctrl Pts',(36.5304235306165,26.0774661593887,-12.4235805192369));
#34752=CARTESIAN_POINT('Ctrl Pts',(39.303224853761,28.1633006173233,-13.8529470821455));
#34753=CARTESIAN_POINT('Ctrl Pts',(40.7926757902182,29.2647880382365,-14.2204718556216));
#34754=CARTESIAN_POINT('Ctrl Pts',(42.2902929581068,30.3771088306738,-14.2198708430667));
#34755=CARTESIAN_POINT('Ctrl Pts',(31.1156831315058,20.4102131175327,1.62964630360479));
#34756=CARTESIAN_POINT('Ctrl Pts',(31.0745541646295,20.431365879152,1.18947037063688));
#34757=CARTESIAN_POINT('Ctrl Pts',(31.0183916683982,20.4490273774992,0.664244043783199));
#34758=CARTESIAN_POINT('Ctrl Pts',(30.9266087974273,20.5924969120704,-1.95287905136656));
#34759=CARTESIAN_POINT('Ctrl Pts',(31.1826348335975,20.8996315610168,-3.87337387080978));
#34760=CARTESIAN_POINT('Ctrl Pts',(32.3021679589004,21.9240162328045,-7.48792130211613));
#34761=CARTESIAN_POINT('Ctrl Pts',(33.1580626257629,22.6177912262544,-9.12360836230029));
#34762=CARTESIAN_POINT('Ctrl Pts',(35.3389311938233,24.3183718642228,-11.877404992731));
#34763=CARTESIAN_POINT('Ctrl Pts',(36.6492226398428,25.3041699214331,-12.9732563608915));
#34764=CARTESIAN_POINT('Ctrl Pts',(39.5517175889713,27.4743946038673,-14.4676858045434));
#34765=CARTESIAN_POINT('Ctrl Pts',(41.1084892565448,28.6183079046667,-14.8501851005199));
#34766=CARTESIAN_POINT('Ctrl Pts',(42.6764590955603,29.7762110964235,-14.8499483202528));
#34767=CARTESIAN_POINT('Ctrl Pts',(31.6308259996108,19.6090715485702,1.62975548654455));
#34768=CARTESIAN_POINT('Ctrl Pts',(31.5897026256139,19.6302214337507,1.18963941044875));
#34769=CARTESIAN_POINT('Ctrl Pts',(31.5334871484553,19.6478553119239,0.664246485850905));
#34770=CARTESIAN_POINT('Ctrl Pts',(31.4411090791311,19.7909423357087,-1.95288623105134));
#34771=CARTESIAN_POINT('Ctrl Pts',(31.6980476865711,20.0986634078557,-3.8731703452115));
#34772=CARTESIAN_POINT('Ctrl Pts',(32.816562323028,21.1223936447507,-7.48823335801853));
#34773=CARTESIAN_POINT('Ctrl Pts',(33.6730817462005,21.8165700765197,-9.1234922771144));
#34774=CARTESIAN_POINT('Ctrl Pts',(35.8537245994984,23.5170056815502,-11.877576477655));
#34775=CARTESIAN_POINT('Ctrl Pts',(37.1643856729968,24.5030412398075,-12.9726927515238));
#34776=CARTESIAN_POINT('Ctrl Pts',(40.0664682545742,26.6730009722967,-14.4683433355124));
#34777=CARTESIAN_POINT('Ctrl Pts',(41.6235121428062,27.8170972008726,-14.8498038985718));
#34778=CARTESIAN_POINT('Ctrl Pts',(43.191403506678,28.9749419513879,-14.8500516281495));
#34779=CARTESIAN_POINT('Ctrl Pts',(32.5463589446091,19.348476735783,1.5967438193466));
#34780=CARTESIAN_POINT('Ctrl Pts',(32.5048979448445,19.3698002629923,1.15301435961605));
#34781=CARTESIAN_POINT('Ctrl Pts',(32.4497342609043,19.3876798928093,0.635579189070094));
#34782=CARTESIAN_POINT('Ctrl Pts',(32.3571628326792,19.5300863678938,-1.86860431107553));
#34783=CARTESIAN_POINT('Ctrl Pts',(32.6011316568668,19.8303563486502,-3.70979114472406));
#34784=CARTESIAN_POINT('Ctrl Pts',(33.6653932580141,20.8181792128001,-7.1701426146716));
#34785=CARTESIAN_POINT('Ctrl Pts',(34.4835007520102,21.4883544786281,-8.73670574472706));
#34786=CARTESIAN_POINT('Ctrl Pts',(36.5652242843068,23.1249120635655,-11.373454410538));
#34787=CARTESIAN_POINT('Ctrl Pts',(37.818331113499,24.0746444553115,-12.4221714958225));
#34788=CARTESIAN_POINT('Ctrl Pts',(40.5901015177707,26.1598165384099,-13.8545909095632));
#34789=CARTESIAN_POINT('Ctrl Pts',(42.0802326794091,27.2617619321778,-14.2195188100673));
#34790=CARTESIAN_POINT('Ctrl Pts',(43.5776539859011,28.3739359680848,-14.2201291128083));
#34791=CARTESIAN_POINT('Ctrl Pts',(31.1388779521431,21.4269965203138,0.));
#34792=CARTESIAN_POINT('Ctrl Pts',(31.0709121284139,21.5339728087887,-1.86858636186358));
#34793=CARTESIAN_POINT('Ctrl Pts',(31.312599524452,21.8327767315482,-3.71029995871917));
#34794=CARTESIAN_POINT('Ctrl Pts',(32.3794073476761,22.8222356829394,-7.1693624749162));
#34795=CARTESIAN_POINT('Ctrl Pts',(33.1959529509165,23.4914073529577,-8.73699595768941));
#34796=CARTESIAN_POINT('Ctrl Pts',(34.3430070554486,24.3931251555465,-10.18908567635));
#34797=CARTESIAN_POINT('Ctrl Pts',(34.4511010682837,24.4777351286714,-10.3203928635166));
#34798=CARTESIAN_POINT('Ctrl Pts',(34.5612980340057,24.5636585134986,-10.4488603765991));
#34799=CARTESIAN_POINT('Ctrl Pts',(32.4262389885814,19.4238236466306,2.77555756156289E-16));
#34800=CARTESIAN_POINT('Ctrl Pts',(32.3571628326792,19.5300863678938,-1.86860431107553));
#34801=CARTESIAN_POINT('Ctrl Pts',(32.6011316568668,19.8303563486502,-3.70979114472406));
#34802=CARTESIAN_POINT('Ctrl Pts',(33.6653932580141,20.8181792128001,-7.1701426146716));
#34803=CARTESIAN_POINT('Ctrl Pts',(34.4835007520102,21.4883544786281,-8.73670574472706));
#34804=CARTESIAN_POINT('Ctrl Pts',(35.636097286559,22.3944741298323,-10.1966053555735));
#34805=CARTESIAN_POINT('Ctrl Pts',(35.7502778955686,22.4838298155642,-10.3350231942303));
#34806=CARTESIAN_POINT('Ctrl Pts',(35.8668060412402,22.5746525783813,-10.4702558451031));
#34807=CARTESIAN_POINT('Ctrl Pts',(35.6222452002842,26.8434139987111,1.24689101061669));
#34808=CARTESIAN_POINT('Ctrl Pts',(35.577148846646,26.8666072002712,0.764254780048341));
#34809=CARTESIAN_POINT('Ctrl Pts',(35.5337649883011,26.8874341048554,0.332948714093336));
#34810=CARTESIAN_POINT('Ctrl Pts',(35.4467644377115,27.0275488741943,-0.978870002701186));
#34811=CARTESIAN_POINT('Ctrl Pts',(35.5421592789952,27.241668781443,-1.98783577088219));
#34812=CARTESIAN_POINT('Ctrl Pts',(36.0467752285198,27.8588388319605,-3.80852727284291));
#34813=CARTESIAN_POINT('Ctrl Pts',(36.45143357029,28.2705345323201,-4.6554436072276));
#34814=CARTESIAN_POINT('Ctrl Pts',(37.491895341187,29.234678928466,-6.04997283342596));
#34815=CARTESIAN_POINT('Ctrl Pts',(38.1327580455662,29.7981738697163,-6.6183216990295));
#34816=CARTESIAN_POINT('Ctrl Pts',(39.5342847195712,30.99175360786,-7.36768403078741));
#34817=CARTESIAN_POINT('Ctrl Pts',(40.3146623988312,31.6463688825513,-7.57138648665175));
#34818=CARTESIAN_POINT('Ctrl Pts',(41.0692078014242,32.2772757571271,-7.56962581969453));
#34819=CARTESIAN_POINT('Ctrl Pts',(34.5390490058878,24.7365171914564,1.35489339099665));
#34820=CARTESIAN_POINT('Ctrl Pts',(34.4950737607895,24.7591338032453,0.884255638226709));
#34821=CARTESIAN_POINT('Ctrl Pts',(34.4480661428698,24.7790577744548,0.426397004057655));
#34822=CARTESIAN_POINT('Ctrl Pts',(34.3594994944659,24.9199792485653,-1.25360819503478));
#34823=CARTESIAN_POINT('Ctrl Pts',(34.5005360167875,25.1605494847776,-2.51960912779922));
#34824=CARTESIAN_POINT('Ctrl Pts',(35.1782280532683,25.89234246528,-4.84647586782171));
#34825=CARTESIAN_POINT('Ctrl Pts',(35.7103931102114,26.3837498256795,-5.91572199046418));
#34826=CARTESIAN_POINT('Ctrl Pts',(37.0724433726659,27.5555654868626,-7.69376028692305));
#34827=CARTESIAN_POINT('Ctrl Pts',(37.9022645329909,28.238264752807,-8.41063186556637));
#34828=CARTESIAN_POINT('Ctrl Pts',(39.727014002825,29.7072268925279,-9.37059840620004));
#34829=CARTESIAN_POINT('Ctrl Pts',(40.7264760905888,30.4999439048231,-9.62435378614244));
#34830=CARTESIAN_POINT('Ctrl Pts',(41.7104427005356,31.27945731062,-9.62320046360557));
#34831=CARTESIAN_POINT('Ctrl Pts',(33.0655926302368,22.88206691246,1.47293210467401));
#34832=CARTESIAN_POINT('Ctrl Pts',(33.0228401731551,22.904054640381,1.0153810375198));
#34833=CARTESIAN_POINT('Ctrl Pts',(32.9718997171366,22.9230067538168,0.528580786098969));
#34834=CARTESIAN_POINT('Ctrl Pts',(32.8819544477726,23.0650249378754,-1.55402875462511));
#34835=CARTESIAN_POINT('Ctrl Pts',(33.0723879388185,23.3341894772782,-3.1012143212481));
#34836=CARTESIAN_POINT('Ctrl Pts',(33.9399090096248,24.191689081893,-5.98129145449616));
#34837=CARTESIAN_POINT('Ctrl Pts',(34.6111514256731,24.7700354696468,-7.29389406575296));
#34838=CARTESIAN_POINT('Ctrl Pts',(36.3249834230628,26.1690197914561,-9.49113593805381));
#34839=CARTESIAN_POINT('Ctrl Pts',(37.3612221809303,26.981935046264,-10.3708286017266));
#34840=CARTESIAN_POINT('Ctrl Pts',(39.6489946054353,28.7521748453928,-11.5604045561156));
#34841=CARTESIAN_POINT('Ctrl Pts',(40.8878834161031,29.6957791360353,-11.869476154081));
#34842=CARTESIAN_POINT('Ctrl Pts',(42.1227528511812,30.6378492234117,-11.8687142284813));
#34843=CARTESIAN_POINT('Ctrl Pts',(31.2585017743465,21.3513306581892,1.59647086199721));
#34844=CARTESIAN_POINT('Ctrl Pts',(31.2170267923954,21.3726613764951,1.15259176008522));
#34845=CARTESIAN_POINT('Ctrl Pts',(31.1619955607637,21.3906100567509,0.635573083900845));
#34846=CARTESIAN_POINT('Ctrl Pts',(31.0709121284139,21.5339728087887,-1.86858636186358));
#34847=CARTESIAN_POINT('Ctrl Pts',(31.312599524452,21.8327767315482,-3.71029995871917));
#34848=CARTESIAN_POINT('Ctrl Pts',(32.3794073476761,22.8222356829394,-7.1693624749162));
#34849=CARTESIAN_POINT('Ctrl Pts',(33.1959529509165,23.4914073529577,-8.73699595768941));
#34850=CARTESIAN_POINT('Ctrl Pts',(35.2782407701191,25.1283275202542,-11.3730256982305));
#34851=CARTESIAN_POINT('Ctrl Pts',(36.5304235306164,26.0774661593863,-12.4235805192369));
#34852=CARTESIAN_POINT('Ctrl Pts',(39.303224853761,28.1633006173257,-13.8529470821455));
#34853=CARTESIAN_POINT('Ctrl Pts',(40.7926757902106,29.264788038245,-14.2204718556263));
#34854=CARTESIAN_POINT('Ctrl Pts',(42.2902929581068,30.3771088306738,-14.2198708430667));
#34855=CARTESIAN_POINT('Ctrl Pts',(32.5463589446091,19.348476735783,1.5967438193466));
#34856=CARTESIAN_POINT('Ctrl Pts',(32.5048979448444,19.3698002629924,1.15301435961605));
#34857=CARTESIAN_POINT('Ctrl Pts',(32.4497342609043,19.3876798928093,0.635579189070094));
#34858=CARTESIAN_POINT('Ctrl Pts',(32.3571628326792,19.5300863678938,-1.86860431107553));
#34859=CARTESIAN_POINT('Ctrl Pts',(32.6011316568668,19.8303563486502,-3.70979114472526));
#34860=CARTESIAN_POINT('Ctrl Pts',(33.6653932580141,20.8181792128001,-7.1701426146704));
#34861=CARTESIAN_POINT('Ctrl Pts',(34.4835007520103,21.4883544786329,-8.73670574472945));
#34862=CARTESIAN_POINT('Ctrl Pts',(36.5652242843068,23.1249120635607,-11.3734544105356));
#34863=CARTESIAN_POINT('Ctrl Pts',(37.818331113499,24.0746444553139,-12.4221714958273));
#34864=CARTESIAN_POINT('Ctrl Pts',(40.5901015177707,26.1598165384076,-13.8545909095584));
#34865=CARTESIAN_POINT('Ctrl Pts',(42.080232679402,27.2617619321892,-14.2195188100863));
#34866=CARTESIAN_POINT('Ctrl Pts',(43.5776539859011,28.3739359680848,-14.2201291128083));
#34867=CARTESIAN_POINT('Ctrl Pts',(34.6889740324161,20.3574113186623,1.47327617534801));
#34868=CARTESIAN_POINT('Ctrl Pts',(34.6462392002948,20.3793899820061,1.01591373651327));
#34869=CARTESIAN_POINT('Ctrl Pts',(34.5951317842845,20.3982550553479,0.528588481842291));
#34870=CARTESIAN_POINT('Ctrl Pts',(34.5033108528571,20.5390678245046,-1.55405138012857));
#34871=CARTESIAN_POINT('Ctrl Pts',(34.6966201504081,20.8100803726295,-3.10057294641664));
#34872=CARTESIAN_POINT('Ctrl Pts',(35.5609316342745,21.665517641723,-5.98227484333611));
#34873=CARTESIAN_POINT('Ctrl Pts',(36.2341428590225,22.2451290911678,-7.29352824387633));
#34874=CARTESIAN_POINT('Ctrl Pts',(37.9472635563608,23.6436563673688,-9.49167634238129));
#34875=CARTESIAN_POINT('Ctrl Pts',(38.9846671296744,24.4573200646104,-10.3690524867537));
#34876=CARTESIAN_POINT('Ctrl Pts',(41.2711400509868,26.2267249209946,-11.5624766483606));
#34877=CARTESIAN_POINT('Ctrl Pts',(42.5108843176087,27.1709103277471,-11.8682745706876));
#34878=CARTESIAN_POINT('Ctrl Pts',(43.745508851356,28.1127915962416,-11.8690397849987));
#34879=CARTESIAN_POINT('Ctrl Pts',(36.9876692386614,20.928463976445,1.35541236849184));
#34880=CARTESIAN_POINT('Ctrl Pts',(36.9437205780947,20.9510669157118,0.885059132421862));
#34881=CARTESIAN_POINT('Ctrl Pts',(36.8964611268002,20.9708596003835,0.426408611898412));
#34882=CARTESIAN_POINT('Ctrl Pts',(36.8050653317411,21.109962892202,-1.2536423221139));
#34883=CARTESIAN_POINT('Ctrl Pts',(36.9504395642185,21.353320564284,-2.51864171287721));
#34884=CARTESIAN_POINT('Ctrl Pts',(37.6232904342718,22.082002830026,-4.84795915807652));
#34885=CARTESIAN_POINT('Ctrl Pts',(38.1584251352155,22.5753183406925,-5.91517020464188));
#34886=CARTESIAN_POINT('Ctrl Pts',(39.5194025113344,23.7464446191315,-7.694575403421));
#34887=CARTESIAN_POINT('Ctrl Pts',(40.3509806159645,24.4302727949463,-8.40795287032022));
#34888=CARTESIAN_POINT('Ctrl Pts',(42.1737699858116,25.8979755524313,-9.37372383746895));
#34889=CARTESIAN_POINT('Ctrl Pts',(43.1745178860489,26.691577151262,-9.62254086020588));
#34890=CARTESIAN_POINT('Ctrl Pts',(44.1581196109331,27.4707976903311,-9.62369151535367));
#34891=CARTESIAN_POINT('Ctrl Pts',(39.3541045014166,21.0396888561031,1.24768196666885));
#34892=CARTESIAN_POINT('Ctrl Pts',(39.3090486643696,21.0628612198304,0.76547935838156));
#34893=CARTESIAN_POINT('Ctrl Pts',(39.2652809952897,21.0834880350444,0.332966405210928));
#34894=CARTESIAN_POINT('Ctrl Pts',(39.1739686379382,21.2208317742353,-0.978922014628528));
#34895=CARTESIAN_POINT('Ctrl Pts',(39.2759744366035,21.4391999182347,-1.98636136650944));
#34896=CARTESIAN_POINT('Ctrl Pts',(39.7732121280721,22.0516290335747,-3.81078790536698));
#34897=CARTESIAN_POINT('Ctrl Pts',(40.1823964038332,22.4662328812349,-4.65460264910927));
#34898=CARTESIAN_POINT('Ctrl Pts',(41.2212230249773,23.4293266124464,-6.05121512492297));
#34899=CARTESIAN_POINT('Ctrl Pts',(41.8647634287383,23.9945420870636,-6.61423873296337));
#34900=CARTESIAN_POINT('Ctrl Pts',(43.2633027806486,25.1862024433187,-7.37244739490039));
#34901=CARTESIAN_POINT('Ctrl Pts',(44.0456294021745,25.8421831847417,-7.56862230200933));
#34902=CARTESIAN_POINT('Ctrl Pts',(44.7996294168197,26.47262641274,-7.57037421505979));
#34903=CARTESIAN_POINT('Ctrl Pts',(33.9789464595044,16.6854562787121,1.59647077610296));
#34904=CARTESIAN_POINT('Ctrl Pts',(33.940929313104,16.7124723847533,1.1525917013978));
#34905=CARTESIAN_POINT('Ctrl Pts',(33.8890125875519,16.7380701329784,0.635573044906332));
#34906=CARTESIAN_POINT('Ctrl Pts',(33.8192589011608,16.8929361805061,-1.8685863618215));
#34907=CARTESIAN_POINT('Ctrl Pts',(34.1010104999226,17.1543030074917,-3.71029995867386));
#34908=CARTESIAN_POINT('Ctrl Pts',(35.2977744483967,17.9818681105204,-7.16936247496116));
#34909=CARTESIAN_POINT('Ctrl Pts',(36.2012418527514,18.5280220223856,-8.73699595771064));
#34910=CARTESIAN_POINT('Ctrl Pts',(38.4952930132093,19.8519402483835,-11.373025698209));
#34911=CARTESIAN_POINT('Ctrl Pts',(39.8698068705931,20.6132138377451,-12.4235805192036));
#34912=CARTESIAN_POINT('Ctrl Pts',(42.9112302679695,22.283206736412,-13.8529470821785));
#34913=CARTESIAN_POINT('Ctrl Pts',(44.5422787457951,23.1615116341824,-14.2204718557499));
#34914=CARTESIAN_POINT('Ctrl Pts',(46.1829520838074,24.0493774600891,-14.2198708430666));
#34915=CARTESIAN_POINT('Ctrl Pts',(33.7036465139255,15.7742431696984,1.62964621771056));
#34916=CARTESIAN_POINT('Ctrl Pts',(33.6659465347851,15.8010338873333,1.18947031171078));
#34917=CARTESIAN_POINT('Ctrl Pts',(33.6128691890261,15.8265083724714,0.664244003030573));
#34918=CARTESIAN_POINT('Ctrl Pts',(33.5424383800233,15.9815796561337,-1.95287905132536));
#34919=CARTESIAN_POINT('Ctrl Pts',(33.8395682581975,16.2491518132771,-3.87337387076446));
#34920=CARTESIAN_POINT('Ctrl Pts',(35.0934912894487,17.1037835503796,-7.48792130216115));
#34921=CARTESIAN_POINT('Ctrl Pts',(36.0394086586928,17.6686904036902,-9.12360836231917));
#34922=CARTESIAN_POINT('Ctrl Pts',(38.440096987709,19.0415916252445,-11.877404992712));
#34923=CARTESIAN_POINT('Ctrl Pts',(39.8773452471315,19.8308817644926,-12.9732563608726));
#34924=CARTESIAN_POINT('Ctrl Pts',(43.0591521575499,21.5659485894108,-14.4676858045621));
#34925=CARTESIAN_POINT('Ctrl Pts',(44.7628739707833,22.4766667937664,-14.8501851005436));
#34926=CARTESIAN_POINT('Ctrl Pts',(46.4796709429185,23.3996388269522,-14.8499483202528));
#34927=CARTESIAN_POINT('Ctrl Pts',(34.0995316375869,14.9079435927952,1.62975540065032));
#34928=CARTESIAN_POINT('Ctrl Pts',(34.0618367850428,14.9347306673263,1.18963935151253));
#34929=CARTESIAN_POINT('Ctrl Pts',(34.0087030668513,14.9601853533851,0.664246445100363));
#34930=CARTESIAN_POINT('Ctrl Pts',(33.9376286808045,15.1149627252298,-1.95288623101673));
#34931=CARTESIAN_POINT('Ctrl Pts',(34.2357452982906,15.3829854641993,-3.87317034517582));
#34932=CARTESIAN_POINT('Ctrl Pts',(35.4885670716917,16.2371143736886,-7.48823335805401));
#34933=CARTESIAN_POINT('Ctrl Pts',(36.4351599687256,16.8023296671644,-9.12349227712854));
#34934=CARTESIAN_POINT('Ctrl Pts',(38.8356042401095,18.1751194545612,-11.8775764776408));
#34935=CARTESIAN_POINT('Ctrl Pts',(40.2732521646523,18.9645920739613,-12.9726927515338));
#34936=CARTESIAN_POINT('Ctrl Pts',(43.4546131985136,20.6994553317739,-14.4683433355024));
#34937=CARTESIAN_POINT('Ctrl Pts',(45.1586304949261,21.6103158609297,-14.8498038985005));
#34938=CARTESIAN_POINT('Ctrl Pts',(46.8753414736305,22.5332412158905,-14.8500516281495));
#34939=CARTESIAN_POINT('Ctrl Pts',(34.968659268658,14.5197073364541,1.59674373345235));
#34940=CARTESIAN_POINT('Ctrl Pts',(34.9306549387561,14.5467143347325,1.15301430090095));
#34941=CARTESIAN_POINT('Ctrl Pts',(34.8785972821206,14.5722625852625,0.635579150080806));
#34942=CARTESIAN_POINT('Ctrl Pts',(34.8072346530973,14.7263938532467,-1.86860431104991));
#34943=CARTESIAN_POINT('Ctrl Pts',(35.0914531001646,14.9888871347947,-3.70979114470167));
#34944=CARTESIAN_POINT('Ctrl Pts',(36.2854639039945,15.8151951687953,-7.17014261469392));
#34945=CARTESIAN_POINT('Ctrl Pts',(37.1906201278479,16.3621201810638,-8.73670574473169));
#34946=CARTESIAN_POINT('Ctrl Pts',(39.4840611441962,17.6857598216825,-11.3734544105334));
#34947=CARTESIAN_POINT('Ctrl Pts',(40.8595741643879,18.4474896114217,-12.4221714958565));
#34948=CARTESIAN_POINT('Ctrl Pts',(43.899882870386,20.1169735923147,-13.8545909095293));
#34949=CARTESIAN_POINT('Ctrl Pts',(45.5316698260147,20.9956349953166,-14.2195188099295));
#34950=CARTESIAN_POINT('Ctrl Pts',(47.1721284105873,21.8833834324346,-14.2201291128084));
#34951=CARTESIAN_POINT('Ctrl Pts',(33.8713086176154,16.777376211144,0.));
#34952=CARTESIAN_POINT('Ctrl Pts',(33.8192589011608,16.8929361805061,-1.8685863618215));
#34953=CARTESIAN_POINT('Ctrl Pts',(34.1010104999226,17.1543030074917,-3.71029995867386));
#34954=CARTESIAN_POINT('Ctrl Pts',(35.2977744483967,17.9818681105204,-7.16936247496116));
#34955=CARTESIAN_POINT('Ctrl Pts',(36.2012418527514,18.5280220223832,-8.73699595770825));
#34956=CARTESIAN_POINT('Ctrl Pts',(37.4649484236425,19.2573188185314,-10.1890856763496));
#34957=CARTESIAN_POINT('Ctrl Pts',(37.5839834499269,19.3256842021738,-10.3203928635159));
#34958=CARTESIAN_POINT('Ctrl Pts',(37.705286942044,19.3950503474818,-10.4488603765981));
#34959=CARTESIAN_POINT('Ctrl Pts',(34.8604849513724,14.611382171278,1.77635683940025E-15));
#34960=CARTESIAN_POINT('Ctrl Pts',(34.8072346530973,14.7263938532467,-1.86860431104991));
#34961=CARTESIAN_POINT('Ctrl Pts',(35.0914531001646,14.9888871347947,-3.70979114470167));
#34962=CARTESIAN_POINT('Ctrl Pts',(36.2854639039945,15.8151951687953,-7.17014261469392));
#34963=CARTESIAN_POINT('Ctrl Pts',(37.1906201278479,16.3621201810638,-8.73670574473169));
#34964=CARTESIAN_POINT('Ctrl Pts',(38.4604391631928,17.0949852513288,-10.1966053555733));
#34965=CARTESIAN_POINT('Ctrl Pts',(38.5861742182004,17.1671818301162,-10.3350231942304));
#34966=CARTESIAN_POINT('Ctrl Pts',(38.7144417021696,17.2404964639596,-10.4702558451038));
#34967=CARTESIAN_POINT('Ctrl Pts',(39.0798782217544,21.5006126898291,1.2468909247222));
#34968=CARTESIAN_POINT('Ctrl Pts',(39.0385416232006,21.5299876964993,0.764254723810705));
#34969=CARTESIAN_POINT('Ctrl Pts',(38.998563331349,21.5567767789524,0.332948693668265));
#34970=CARTESIAN_POINT('Ctrl Pts',(38.9323887327488,21.7078468488828,-0.978870002686299));
#34971=CARTESIAN_POINT('Ctrl Pts',(39.0572850320743,21.9062112228022,-1.98783577086007));
#34972=CARTESIAN_POINT('Ctrl Pts',(39.6445971746525,22.4452850348741,-3.80852727286476));
#34973=CARTESIAN_POINT('Ctrl Pts',(40.1037270850429,22.7952013801406,-4.6554436072369));
#34974=CARTESIAN_POINT('Ctrl Pts',(41.2708105091343,23.6014590278601,-6.0499728334163));
#34975=CARTESIAN_POINT('Ctrl Pts',(41.9853438467173,24.0680141309112,-6.61832169894315));
#34976=CARTESIAN_POINT('Ctrl Pts',(43.5424691073156,25.0499869064955,-7.36768403087327));
#34977=CARTESIAN_POINT('Ctrl Pts',(44.4080651338049,25.5868798186403,-7.57138648703229));
#34978=CARTESIAN_POINT('Ctrl Pts',(45.2447177621913,26.1039819636361,-7.56962581969415));
#34979=CARTESIAN_POINT('Ctrl Pts',(37.707864724394,19.5693159454017,1.35489330510224));
#34980=CARTESIAN_POINT('Ctrl Pts',(37.6675557657705,19.5979606808254,0.884255581228092));
#34981=CARTESIAN_POINT('Ctrl Pts',(37.6238620982185,19.6243717351804,0.426396977899622));
#34982=CARTESIAN_POINT('Ctrl Pts',(37.5562521484826,19.7764631777486,-1.25360819501488));
#34983=CARTESIAN_POINT('Ctrl Pts',(37.7300898366261,19.9945131659699,-2.5196091277746));
#34984=CARTESIAN_POINT('Ctrl Pts',(38.5050289449343,20.6224119165152,-4.8464758678461));
#34985=CARTESIAN_POINT('Ctrl Pts',(39.1017118879826,21.0330824745219,-5.91572199047591));
#34986=CARTESIAN_POINT('Ctrl Pts',(40.6166651989596,21.9991307790772,-7.69376028691107));
#34987=CARTESIAN_POINT('Ctrl Pts',(41.5351982120318,22.5567852866117,-8.41063186550891));
#34988=CARTESIAN_POINT('Ctrl Pts',(43.550429472638,23.7511065841766,-9.37059840625714));
#34989=CARTESIAN_POINT('Ctrl Pts',(44.6525338708088,24.3935165950095,-9.62435378637539));
#34990=CARTESIAN_POINT('Ctrl Pts',(45.7374214437733,25.0250626292171,-9.62320046360533));
#34991=CARTESIAN_POINT('Ctrl Pts',(35.9854902185572,17.9434360021527,1.47293201877968));
#34992=CARTESIAN_POINT('Ctrl Pts',(35.9463021021743,17.9712842340133,1.0153809796928));
#34993=CARTESIAN_POINT('Ctrl Pts',(35.8985773174017,17.9972930238834,0.528580753670798));
#34994=CARTESIAN_POINT('Ctrl Pts',(35.8297588571711,18.150666211701,-1.55402875459602));
#34995=CARTESIAN_POINT('Ctrl Pts',(36.0565601177425,18.3899895327227,-3.10121432121615));
#34996=CARTESIAN_POINT('Ctrl Pts',(37.0372859924633,19.1152999068356,-5.98129145452784));
#34997=CARTESIAN_POINT('Ctrl Pts',(37.7840034012197,19.5922318064067,-7.29389406576467));
#34998=CARTESIAN_POINT('Ctrl Pts',(39.6794872874942,20.7330727614611,-9.49113593804186));
#34999=CARTESIAN_POINT('Ctrl Pts',(40.8208685319567,21.3902415598895,-10.3708286016837));
#35000=CARTESIAN_POINT('Ctrl Pts',(43.3372861226234,22.8168789076785,-11.5604045561583));
#35001=CARTESIAN_POINT('Ctrl Pts',(44.6978537235956,23.5745664063952,-11.8694761542236));
#35002=CARTESIAN_POINT('Ctrl Pts',(46.0542245204214,24.3313073348067,-11.8687142284811));
#35003=CARTESIAN_POINT('Ctrl Pts',(33.9789464595044,16.6854562787121,1.59647077610296));
#35004=CARTESIAN_POINT('Ctrl Pts',(33.940929313104,16.7124723847533,1.1525917013978));
#35005=CARTESIAN_POINT('Ctrl Pts',(33.8890125875519,16.7380701329784,0.635573044906332));
#35006=CARTESIAN_POINT('Ctrl Pts',(33.8192589011608,16.8929361805061,-1.8685863618215));
#35007=CARTESIAN_POINT('Ctrl Pts',(34.1010104999226,17.1543030074917,-3.71029995867386));
#35008=CARTESIAN_POINT('Ctrl Pts',(35.2977744483967,17.9818681105204,-7.16936247496116));
#35009=CARTESIAN_POINT('Ctrl Pts',(36.2012418527514,18.5280220223832,-8.73699595770825));
#35010=CARTESIAN_POINT('Ctrl Pts',(38.4952930132093,19.8519402483859,-11.3730256982114));
#35011=CARTESIAN_POINT('Ctrl Pts',(39.8698068705931,20.6132138377451,-12.4235805192036));
#35012=CARTESIAN_POINT('Ctrl Pts',(42.9112302679695,22.283206736412,-13.8529470821785));
#35013=CARTESIAN_POINT('Ctrl Pts',(44.5422787457922,23.1615116341878,-14.2204718557499));
#35014=CARTESIAN_POINT('Ctrl Pts',(46.1829520838074,24.0493774600891,-14.2198708430666));
#35015=CARTESIAN_POINT('Ctrl Pts',(34.968659268658,14.5197073364541,1.59674373345235));
#35016=CARTESIAN_POINT('Ctrl Pts',(34.930654938756,14.5467143347324,1.15301430090095));
#35017=CARTESIAN_POINT('Ctrl Pts',(34.8785972821206,14.5722625852624,0.635579150080806));
#35018=CARTESIAN_POINT('Ctrl Pts',(34.8072346530973,14.7263938532467,-1.86860431104991));
#35019=CARTESIAN_POINT('Ctrl Pts',(35.0914531001646,14.9888871347947,-3.70979114470287));
#35020=CARTESIAN_POINT('Ctrl Pts',(36.2854639039945,15.8151951687953,-7.17014261469272));
#35021=CARTESIAN_POINT('Ctrl Pts',(37.1906201278479,16.3621201810662,-8.73670574473408));
#35022=CARTESIAN_POINT('Ctrl Pts',(39.4840611441962,17.6857598216801,-11.373454410531));
#35023=CARTESIAN_POINT('Ctrl Pts',(40.8595741643879,18.4474896114217,-12.4221714958565));
#35024=CARTESIAN_POINT('Ctrl Pts',(43.8998828703861,20.1169735923147,-13.8545909095293));
#35025=CARTESIAN_POINT('Ctrl Pts',(45.531669826027,20.9956349952939,-14.2195188099295));
#35026=CARTESIAN_POINT('Ctrl Pts',(47.1721284105873,21.8833834324346,-14.2201291128084));
#35027=CARTESIAN_POINT('Ctrl Pts',(37.2330519862578,15.2134465003399,1.47327608945368));
#35028=CARTESIAN_POINT('Ctrl Pts',(37.1938800254435,15.2412832516015,1.01591367865198));
#35029=CARTESIAN_POINT('Ctrl Pts',(37.1459775929436,15.2672296481878,0.528588449420692));
#35030=CARTESIAN_POINT('Ctrl Pts',(37.0751310137516,15.4196766250279,-1.55405138012023));
#35031=CARTESIAN_POINT('Ctrl Pts',(37.3050418083334,15.66041987477,-3.10057294641005));
#35032=CARTESIAN_POINT('Ctrl Pts',(38.2822972641785,16.3841456768374,-5.9822748433428));
#35033=CARTESIAN_POINT('Ctrl Pts',(39.0311434790186,16.8620495708873,-7.29352824387147));
#35034=CARTESIAN_POINT('Ctrl Pts',(40.9258582609005,18.0025393609562,-9.49167634238628));
#35035=CARTESIAN_POINT('Ctrl Pts',(42.0684989791267,18.6602832132252,-10.3690524867972));
#35036=CARTESIAN_POINT('Ctrl Pts',(44.5835114689155,20.0862790553768,-11.5624766483172));
#35037=CARTESIAN_POINT('Ctrl Pts',(45.9450085199795,20.8444200112153,-11.8682745704832));
#35038=CARTESIAN_POINT('Ctrl Pts',(47.3011100364939,21.6010088957268,-11.8690397849988));
#35039=CARTESIAN_POINT('Ctrl Pts',(39.5896190563862,15.4515482289399,1.35541228259744));
#35040=CARTESIAN_POINT('Ctrl Pts',(39.5493344659561,15.4801756476478,0.885059075370257));
#35041=CARTESIAN_POINT('Ctrl Pts',(39.5053728442213,15.5064925913696,0.426408585750303));
#35042=CARTESIAN_POINT('Ctrl Pts',(39.4347037901216,15.6571869876679,-1.25364232212529));
#35043=CARTESIAN_POINT('Ctrl Pts',(39.6132317302818,15.8773787191618,-2.51864171289602));
#35044=CARTESIAN_POINT('Ctrl Pts',(40.382936247472,16.5028873873876,-4.84795915805801));
#35045=CARTESIAN_POINT('Ctrl Pts',(40.9828301658549,16.9150240490132,-5.91517020462755));
#35046=CARTESIAN_POINT('Ctrl Pts',(42.4966234015924,17.8805426754076,-7.6945754034356));
#35047=CARTESIAN_POINT('Ctrl Pts',(43.4170561364029,18.4390645628875,-8.40795287039257));
#35048=CARTESIAN_POINT('Ctrl Pts',(45.4301680192463,19.6324182482204,-9.37372383739693));
#35049=CARTESIAN_POINT('Ctrl Pts',(46.5336710319636,20.2755208515651,-9.62254085992063));
#35050=CARTESIAN_POINT('Ctrl Pts',(47.6181557545822,20.9068289285805,-9.62369151535394));
#35051=CARTESIAN_POINT('Ctrl Pts',(41.9477963710449,15.2248621479927,1.24768188077437));
#35052=CARTESIAN_POINT('Ctrl Pts',(41.9064969112189,15.2542107628473,0.765479302065719));
#35053=CARTESIAN_POINT('Ctrl Pts',(41.8661102394687,15.2808564144635,0.332966384800994));
#35054=CARTESIAN_POINT('Ctrl Pts',(41.795273363349,15.4297972934032,-0.978922014661338));
#35055=CARTESIAN_POINT('Ctrl Pts',(41.9273179171871,15.6314258258285,-1.98636136655007));
#35056=CARTESIAN_POINT('Ctrl Pts',(42.5066521964225,16.1668569942609,-3.81078790532691));
#35057=CARTESIAN_POINT('Ctrl Pts',(42.9706758457638,16.5190077784711,-4.65460264908071));
#35058=CARTESIAN_POINT('Ctrl Pts',(44.1359912383933,17.3244581616248,-6.051215124952));
#35059=CARTESIAN_POINT('Ctrl Pts',(44.8534198776544,17.7923352091155,-6.61423873305977));
#35060=CARTESIAN_POINT('Ctrl Pts',(46.4073150662577,18.7728332796184,-7.37244739480456));
#35061=CARTESIAN_POINT('Ctrl Pts',(47.2750345238088,19.3108003965529,-7.56862230161463));
#35062=CARTESIAN_POINT('Ctrl Pts',(48.1110813316863,19.8275212310755,-7.57037421506018));
#35063=CARTESIAN_POINT('Ctrl Pts',(36.0076777827441,11.6799141290247,1.59647068126612));
#35064=CARTESIAN_POINT('Ctrl Pts',(35.9738923911208,11.7120656519291,1.152591636598));
#35065=CARTESIAN_POINT('Ctrl Pts',(35.9261470465084,11.7447913705166,0.635573001854836));
#35066=CARTESIAN_POINT('Ctrl Pts',(35.879143089373,11.9080080866873,-1.86858636178295));
#35067=CARTESIAN_POINT('Ctrl Pts',(36.1952232408275,12.126617143028,-3.71029995869426));
#35068=CARTESIAN_POINT('Ctrl Pts',(37.497580651705,12.7754415588947,-7.16936247494101));
#35069=CARTESIAN_POINT('Ctrl Pts',(38.4695778661834,13.1874595938719,-8.73699595767948));
#35070=CARTESIAN_POINT('Ctrl Pts',(40.9286921018507,14.1714247212918,-11.3730256982404));
#35071=CARTESIAN_POINT('Ctrl Pts',(42.397555917808,14.7293359258803,-12.4235805192179));
#35072=CARTESIAN_POINT('Ctrl Pts',(45.6456867795974,15.9494910258928,-13.8529470821646));
#35073=CARTESIAN_POINT('Ctrl Pts',(47.3851293551906,16.5867336459556,-14.2204718557025));
#35074=CARTESIAN_POINT('Ctrl Pts',(49.1354594857183,17.2320701170938,-14.2198708430667));
#35075=CARTESIAN_POINT('Ctrl Pts',(35.6055008474197,10.8171551228317,1.62964612287373));
#35076=CARTESIAN_POINT('Ctrl Pts',(35.5719973185988,10.849038413867,1.18947024665197));
#35077=CARTESIAN_POINT('Ctrl Pts',(35.5230856250742,10.8818072974761,0.664243958036444));
#35078=CARTESIAN_POINT('Ctrl Pts',(35.47544064564,11.0453235253574,-1.95287905128342));
#35079=CARTESIAN_POINT('Ctrl Pts',(35.8076256583526,11.2678861931943,-3.87337387078009));
#35080=CARTESIAN_POINT('Ctrl Pts',(37.1704123385812,11.9353671582151,-7.48792130214571));
#35081=CARTESIAN_POINT('Ctrl Pts',(38.1870962603493,12.3599059968478,-9.12360836229034));
#35082=CARTESIAN_POINT('Ctrl Pts',(40.7587332590659,13.3771794921454,-11.8774049927409));
#35083=CARTESIAN_POINT('Ctrl Pts',(42.2936801020575,13.9538940422629,-12.973256360882));
#35084=CARTESIAN_POINT('Ctrl Pts',(45.6900265604413,15.2184820528374,-14.4676858045529));
#35085=CARTESIAN_POINT('Ctrl Pts',(47.5060156561426,15.8774655648044,-14.8501851005246));
#35086=CARTESIAN_POINT('Ctrl Pts',(49.3366907261822,16.5467173899494,-14.8499483202528));
#35087=CARTESIAN_POINT('Ctrl Pts',(35.8740691471582,9.90333289917181,1.62975530581352));
#35088=CARTESIAN_POINT('Ctrl Pts',(35.8405701742713,9.93521185459246,1.18963928644524));
#35089=CARTESIAN_POINT('Ctrl Pts',(35.7915998644016,9.96796916327873,0.664246400106497));
#35090=CARTESIAN_POINT('Ctrl Pts',(35.7432760306146,10.1312860615133,-1.95288623097604));
#35091=CARTESIAN_POINT('Ctrl Pts',(36.076501863553,10.3541542972526,-3.87317034518541));
#35092=CARTESIAN_POINT('Ctrl Pts',(37.4381269352739,11.0212942780538,-7.48823335804453));
#35093=CARTESIAN_POINT('Ctrl Pts',(38.4555234045685,11.4460422797433,-9.12349227711401));
#35094=CARTESIAN_POINT('Ctrl Pts',(41.0269029710712,12.4632402081524,-11.8775764776553));
#35095=CARTESIAN_POINT('Ctrl Pts',(42.5622713808008,13.0400785027576,-12.9726927515287));
#35096=CARTESIAN_POINT('Ctrl Pts',(45.9581475303923,14.3045284730937,-14.4683433355075));
#35097=CARTESIAN_POINT('Ctrl Pts',(47.7744493566106,14.9636108095524,-14.8498038985005));
#35098=CARTESIAN_POINT('Ctrl Pts',(49.6050326655027,15.6328286697383,-14.8500516281494));
#35099=CARTESIAN_POINT('Ctrl Pts',(36.6790985320904,9.39535856987503,1.59674363861559));
#35100=CARTESIAN_POINT('Ctrl Pts',(36.6453245302972,9.42749925373858,1.15301423608143));
#35101=CARTESIAN_POINT('Ctrl Pts',(36.5974326448246,9.46019603502289,0.635579107029969));
#35102=CARTESIAN_POINT('Ctrl Pts',(36.5487315518166,9.62291442707752,-1.86860431101451));
#35103=CARTESIAN_POINT('Ctrl Pts',(36.8674137538261,9.84228740317919,-3.70979114470517));
#35104=CARTESIAN_POINT('Ctrl Pts',(38.1668671434391,10.490259358486,-7.17014261469043));
#35105=CARTESIAN_POINT('Ctrl Pts',(39.1406457267337,10.9028003011106,-8.73670574472907));
#35106=CARTESIAN_POINT('Ctrl Pts',(41.5991163818614,11.8865765113095,-11.373454410536));
#35107=CARTESIAN_POINT('Ctrl Pts',(43.0690341146615,12.4447970771195,-12.4221714958514));
#35108=CARTESIAN_POINT('Ctrl Pts',(46.3159892044796,13.6646070765311,-13.8545909095343));
#35109=CARTESIAN_POINT('Ctrl Pts',(48.0562134772207,14.3020974767513,-14.2195188099531));
#35110=CARTESIAN_POINT('Ctrl Pts',(49.8063143340195,14.9473483165658,-14.2201291128083));
#35111=CARTESIAN_POINT('Ctrl Pts',(35.9142171164211,11.7862169042729,0.));
#35112=CARTESIAN_POINT('Ctrl Pts',(35.879143089373,11.9080080866873,-1.86858636178295));
#35113=CARTESIAN_POINT('Ctrl Pts',(36.1952232408275,12.126617143028,-3.71029995869426));
#35114=CARTESIAN_POINT('Ctrl Pts',(37.497580651705,12.7754415588947,-7.16936247494101));
#35115=CARTESIAN_POINT('Ctrl Pts',(38.4695778661786,13.1874595938719,-8.73699595767948));
#35116=CARTESIAN_POINT('Ctrl Pts',(39.8242114819224,13.7294890038866,-10.1890856763506));
#35117=CARTESIAN_POINT('Ctrl Pts',(39.9517643117909,13.7802180759794,-10.3203928635175));
#35118=CARTESIAN_POINT('Ctrl Pts',(40.081704941015,13.8316148870794,-10.4488603766));
#35119=CARTESIAN_POINT('Ctrl Pts',(36.5850719698906,9.50149509066483,1.60982338570648E-15));
#35120=CARTESIAN_POINT('Ctrl Pts',(36.5487315518166,9.62291442707752,-1.86860431101451));
#35121=CARTESIAN_POINT('Ctrl Pts',(36.8674137538261,9.84228740317919,-3.70979114470517));
#35122=CARTESIAN_POINT('Ctrl Pts',(38.1668671434391,10.490259358486,-7.17014261469043));
#35123=CARTESIAN_POINT('Ctrl Pts',(39.1406457267337,10.9028003011106,-8.73670574472907));
#35124=CARTESIAN_POINT('Ctrl Pts',(40.5018374092149,11.4474917709691,-10.196605355572));
#35125=CARTESIAN_POINT('Ctrl Pts',(40.6365673070934,11.5010595286606,-10.3350231942278));
#35126=CARTESIAN_POINT('Ctrl Pts',(40.773962973282,11.555373559002,-10.4702558450999));
#35127=CARTESIAN_POINT('Ctrl Pts',(41.7419576204998,15.7201209119706,1.2468908298854));
#35128=CARTESIAN_POINT('Ctrl Pts',(41.7052222707517,15.7550797324017,0.764254661706054));
#35129=CARTESIAN_POINT('Ctrl Pts',(41.6694633881772,15.7872856429817,0.332948671123798));
#35130=CARTESIAN_POINT('Ctrl Pts',(41.6254618648117,15.9462356620175,-0.978870002690552));
#35131=CARTESIAN_POINT('Ctrl Pts',(41.7773170936967,16.1248063760006,-1.98783577088475));
#35132=CARTESIAN_POINT('Ctrl Pts',(42.4353694479977,16.5748099612961,-3.80852727284034));
#35133=CARTESIAN_POINT('Ctrl Pts',(42.9396243659783,16.8558236637775,-4.65544360721786));
#35134=CARTESIAN_POINT('Ctrl Pts',(44.209570990269,17.4877814824514,-6.04997283343574));
#35135=CARTESIAN_POINT('Ctrl Pts',(44.9832291228105,17.8478990308906,-6.61832169896729));
#35136=CARTESIAN_POINT('Ctrl Pts',(46.6642543902182,18.5982747098438,-7.36768403084973));
#35137=CARTESIAN_POINT('Ctrl Pts',(47.5974477252292,19.0065156676782,-7.57138648690887));
#35138=CARTESIAN_POINT('Ctrl Pts',(48.4991757443116,19.3992863750339,-7.56962581969459));
#35139=CARTESIAN_POINT('Ctrl Pts',(40.1090570584213,14.0037398626873,1.35489321026543));
#35140=CARTESIAN_POINT('Ctrl Pts',(40.0732349602079,14.0378295966234,0.884255518285701));
#35141=CARTESIAN_POINT('Ctrl Pts',(40.0337447201316,14.0701900799517,0.426396949022936));
#35142=CARTESIAN_POINT('Ctrl Pts',(39.9884678119704,14.2303553472431,-1.25360819500655));
#35143=CARTESIAN_POINT('Ctrl Pts',(40.1915678319233,14.4214462185201,-2.51960912779463));
#35144=CARTESIAN_POINT('Ctrl Pts',(41.0479784866768,14.9326685312526,-4.84647586782628));
#35145=CARTESIAN_POINT('Ctrl Pts',(41.6970325717428,15.254242218588,-5.91572199045678));
#35146=CARTESIAN_POINT('Ctrl Pts',(43.3340488505895,15.9948572088803,-7.69376028693048));
#35147=CARTESIAN_POINT('Ctrl Pts',(44.322595033069,16.4161147204054,-8.41063186553294));
#35148=CARTESIAN_POINT('Ctrl Pts',(46.487283787483,17.31148223828,-9.37059840623356));
#35149=CARTESIAN_POINT('Ctrl Pts',(47.6695948287921,17.7905076322617,-9.6243537862995));
#35150=CARTESIAN_POINT('Ctrl Pts',(48.8333181822474,18.2612298390047,-9.62320046360562));
#35151=CARTESIAN_POINT('Ctrl Pts',(38.1728270004196,12.6395284821795,1.47293192394287));
#35152=CARTESIAN_POINT('Ctrl Pts',(38.1380009815219,12.6726703073971,1.01538091584187));
#35153=CARTESIAN_POINT('Ctrl Pts',(38.0944634070468,12.7052063084745,0.528580717869739));
#35154=CARTESIAN_POINT('Ctrl Pts',(38.0481727007018,12.8668122636064,-1.55402875457325));
#35155=CARTESIAN_POINT('Ctrl Pts',(38.3067247111946,13.0714224335833,-3.10121432123275));
#35156=CARTESIAN_POINT('Ctrl Pts',(39.3806906392157,13.6497783496954,-5.98129145451145));
#35157=CARTESIAN_POINT('Ctrl Pts',(40.187682027567,14.0155868029452,-7.2938940657431));
#35158=CARTESIAN_POINT('Ctrl Pts',(42.226231216963,14.8750601592607,-9.49113593806368));
#35159=CARTESIAN_POINT('Ctrl Pts',(43.4495197173632,15.3631044396819,-10.3708286016932));
#35160=CARTESIAN_POINT('Ctrl Pts',(46.1433554687415,16.4170971138854,-11.5604045561491));
#35161=CARTESIAN_POINT('Ctrl Pts',(47.5979046271564,16.9734434882805,-11.8694761541619));
#35162=CARTESIAN_POINT('Ctrl Pts',(49.0481649878424,17.529450194561,-11.8687142284813));
#35163=CARTESIAN_POINT('Ctrl Pts',(36.0076777827441,11.6799141290247,1.59647068126612));
#35164=CARTESIAN_POINT('Ctrl Pts',(35.9738923911208,11.7120656519291,1.152591636598));
#35165=CARTESIAN_POINT('Ctrl Pts',(35.9261470465084,11.7447913705166,0.635573001854836));
#35166=CARTESIAN_POINT('Ctrl Pts',(35.879143089373,11.9080080866873,-1.86858636178295));
#35167=CARTESIAN_POINT('Ctrl Pts',(36.1952232408275,12.126617143028,-3.71029995869426));
#35168=CARTESIAN_POINT('Ctrl Pts',(37.497580651705,12.7754415588947,-7.16936247494101));
#35169=CARTESIAN_POINT('Ctrl Pts',(38.4695778661786,13.1874595938719,-8.73699595767948));
#35170=CARTESIAN_POINT('Ctrl Pts',(40.9286921018555,14.1714247212918,-11.3730256982404));
#35171=CARTESIAN_POINT('Ctrl Pts',(42.3975559178032,14.7293359258803,-12.4235805192227));
#35172=CARTESIAN_POINT('Ctrl Pts',(45.6456867796022,15.9494910258928,-13.8529470821598));
#35173=CARTESIAN_POINT('Ctrl Pts',(47.3851293551851,16.5867336459606,-14.2204718557025));
#35174=CARTESIAN_POINT('Ctrl Pts',(49.1354594857183,17.2320701170938,-14.2198708430667));
#35175=CARTESIAN_POINT('Ctrl Pts',(36.6790985320904,9.39535856987503,1.59674363861559));
#35176=CARTESIAN_POINT('Ctrl Pts',(36.6453245302972,9.42749925373858,1.15301423608143));
#35177=CARTESIAN_POINT('Ctrl Pts',(36.5974326448246,9.46019603502288,0.635579107029969));
#35178=CARTESIAN_POINT('Ctrl Pts',(36.5487315518166,9.62291442707752,-1.86860431101452));
#35179=CARTESIAN_POINT('Ctrl Pts',(36.8674137538261,9.84228740317919,-3.70979114470517));
#35180=CARTESIAN_POINT('Ctrl Pts',(38.1668671434391,10.490259358486,-7.17014261469044));
#35181=CARTESIAN_POINT('Ctrl Pts',(39.1406457267289,10.9028003011094,-8.73670574472908));
#35182=CARTESIAN_POINT('Ctrl Pts',(41.5991163818662,11.8865765113107,-11.373454410536));
#35183=CARTESIAN_POINT('Ctrl Pts',(43.0690341146567,12.4447970771206,-12.4221714958514));
#35184=CARTESIAN_POINT('Ctrl Pts',(46.3159892044845,13.6646070765299,-13.8545909095343));
#35185=CARTESIAN_POINT('Ctrl Pts',(48.0562134772158,14.302097476756,-14.2195188099531));
#35186=CARTESIAN_POINT('Ctrl Pts',(49.8063143340195,14.9473483165658,-14.2201291128083));
#35187=CARTESIAN_POINT('Ctrl Pts',(39.019172373722,9.75977978596914,1.47327599461697));
#35188=CARTESIAN_POINT('Ctrl Pts',(38.9843607120455,9.79290794826382,1.01591361477532));
#35189=CARTESIAN_POINT('Ctrl Pts',(38.9406384185497,9.82540747302622,0.528588413620481));
#35190=CARTESIAN_POINT('Ctrl Pts',(38.8922084230886,9.98638527612265,-1.55405138010143));
#35191=CARTESIAN_POINT('Ctrl Pts',(39.1540403939528,10.191958389164,-3.10057294640731));
#35192=CARTESIAN_POINT('Ctrl Pts',(40.2243457187589,10.7692397539633,-5.98227484334544));
#35193=CARTESIAN_POINT('Ctrl Pts',(41.0335825742787,11.1357073475014,-7.29352824388559));
#35194=CARTESIAN_POINT('Ctrl Pts',(43.0713205117044,11.9949425681683,-9.49167634237202));
#35195=CARTESIAN_POINT('Ctrl Pts',(44.295937504919,12.483376807401,-10.3690524867825));
#35196=CARTESIAN_POINT('Ctrl Pts',(46.9882911615459,13.5369344722676,-11.5624766483317));
#35197=CARTESIAN_POINT('Ctrl Pts',(48.4438248432725,14.0935974137064,-11.8682745705354));
#35198=CARTESIAN_POINT('Ctrl Pts',(49.8937970264263,14.6494919462605,-11.8690397849986));
#35199=CARTESIAN_POINT('Ctrl Pts',(41.3856383979639,9.66008352082062,1.35541218776079));
#35200=CARTESIAN_POINT('Ctrl Pts',(41.3498379553998,9.6941526463457,0.885059012390845));
#35201=CARTESIAN_POINT('Ctrl Pts',(41.3100690951945,9.72645811078577,0.426408556874883));
#35202=CARTESIAN_POINT('Ctrl Pts',(41.2615653996783,9.88567590770113,-1.25364232212296));
#35203=CARTESIAN_POINT('Ctrl Pts',(41.4696127334802,10.0782192299378,-2.51864171288225));
#35204=CARTESIAN_POINT('Ctrl Pts',(42.3205019334091,10.5878207478988,-4.84795915807154));
#35205=CARTESIAN_POINT('Ctrl Pts',(42.9729429590446,10.9103886466027,-5.91517020465837));
#35206=CARTESIAN_POINT('Ctrl Pts',(44.6087355895318,11.6506444460343,-7.69457540340448));
#35207=CARTESIAN_POINT('Ctrl Pts',(45.5992855983381,12.072490150225,-8.40795287036824));
#35208=CARTESIAN_POINT('Ctrl Pts',(47.7617388416121,12.9672015236695,-9.3737238374209));
#35209=CARTESIAN_POINT('Ctrl Pts',(48.9455328277801,13.446713416983,-9.62254085998223));
#35210=CARTESIAN_POINT('Ctrl Pts',(50.1088235664895,13.9172574201602,-9.62369151535363));
#35211=CARTESIAN_POINT('Ctrl Pts',(43.6875520748214,9.10010115416761,1.24768178593779));
#35212=CARTESIAN_POINT('Ctrl Pts',(43.6508497297321,9.13502856601518,0.765479239901494));
#35213=CARTESIAN_POINT('Ctrl Pts',(43.6146662116266,9.16715062416918,0.332966362258436));
#35214=CARTESIAN_POINT('Ctrl Pts',(43.5657468507513,9.32465663564124,-0.978922014674724));
#35215=CARTESIAN_POINT('Ctrl Pts',(43.7251421133956,9.50544098102187,-1.98636136652885));
#35216=CARTESIAN_POINT('Ctrl Pts',(44.3747794050985,9.95297436780749,-3.8107879053477));
#35217=CARTESIAN_POINT('Ctrl Pts',(44.8841962446775,10.2355033142224,-4.65460264913776));
#35218=CARTESIAN_POINT('Ctrl Pts',(46.1522779478775,10.8669137022454,-6.05121512489442));
#35219=CARTESIAN_POINT('Ctrl Pts',(46.928990044369,11.227927695242,-6.61423873303054));
#35220=CARTESIAN_POINT('Ctrl Pts',(48.6066082448372,11.9773033666524,-7.37244739483315));
#35221=CARTESIAN_POINT('Ctrl Pts',(49.5420562727261,12.3863053996828,-7.56862230169514));
#35222=CARTESIAN_POINT('Ctrl Pts',(50.4431303715411,12.7787848949965,-7.57037421505972));
#35223=CARTESIAN_POINT('Ctrl Pts',(37.3033966274915,6.43660260973346,1.59647061166179));
#35224=CARTESIAN_POINT('Ctrl Pts',(37.2745307626595,6.47323503721765,1.15259158904714));
#35225=CARTESIAN_POINT('Ctrl Pts',(37.2319287549545,6.51242252436852,0.635572970245465));
#35226=CARTESIAN_POINT('Ctrl Pts',(37.2086313911938,6.68066728815551,-1.86858636171891));
#35227=CARTESIAN_POINT('Ctrl Pts',(37.5526056149563,6.85206832386134,-3.7102999587003));
#35228=CARTESIAN_POINT('Ctrl Pts',(38.934044247035,7.30894385840886,-7.16936247493491));
#35229=CARTESIAN_POINT('Ctrl Pts',(39.9547842114115,7.57843851744906,-8.73699595770386));
#35230=CARTESIAN_POINT('Ctrl Pts',(42.5289010478496,8.20241985396081,-11.3730256982159));
#35231=CARTESIAN_POINT('Ctrl Pts',(44.0622129909515,8.5456112103854,-12.4235805192521));
#35232=CARTESIAN_POINT('Ctrl Pts',(47.4509287397227,9.29108967269768,-13.8529470821302));
#35233=CARTESIAN_POINT('Ctrl Pts',(49.263355378306,9.67429759302916,-14.2204718556739));
#35234=CARTESIAN_POINT('Ctrl Pts',(51.0877106274638,10.0639675197017,-14.2198708430667));
#35235=CARTESIAN_POINT('Ctrl Pts',(36.7825298650421,5.63986099173568,1.62964605326941));
#35236=CARTESIAN_POINT('Ctrl Pts',(36.7539048206817,5.67618780432166,1.1894701989102));
#35237=CARTESIAN_POINT('Ctrl Pts',(36.7101544788329,5.71558400588172,0.664243924999381));
#35238=CARTESIAN_POINT('Ctrl Pts',(36.68626524241,5.88421645976228,-1.95287905121125));
#35239=CARTESIAN_POINT('Ctrl Pts',(37.0467430607544,6.05723890417281,-3.87337387078733));
#35240=CARTESIAN_POINT('Ctrl Pts',(38.490650983132,6.52398110941273,-7.48792130213842));
#35241=CARTESIAN_POINT('Ctrl Pts',(39.5574047047037,6.79950954685247,-9.12360836231238));
#35242=CARTESIAN_POINT('Ctrl Pts',(42.2476392596819,7.44044656126999,-11.8774049927189));
#35243=CARTESIAN_POINT('Ctrl Pts',(43.8490375949839,7.79284527694883,-12.9732563608924));
#35244=CARTESIAN_POINT('Ctrl Pts',(47.3907837817412,8.56121110823887,-14.4676858045425));
#35245=CARTESIAN_POINT('Ctrl Pts',(49.2820718587551,8.95504492393606,-14.8501851005532));
#35246=CARTESIAN_POINT('Ctrl Pts',(51.1893577615276,9.35695250368056,-14.8499483202528));
#35247=CARTESIAN_POINT('Ctrl Pts',(36.9183140647621,4.69711890654721,1.62975523620918));
#35248=CARTESIAN_POINT('Ctrl Pts',(36.8896929129492,4.7334407792703,1.18963923869573));
#35249=CARTESIAN_POINT('Ctrl Pts',(36.845882904082,4.77283386569958,0.664246367069779));
#35250=CARTESIAN_POINT('Ctrl Pts',(36.8212933555167,4.9413656298699,-1.95288623090525));
#35251=CARTESIAN_POINT('Ctrl Pts',(37.1828448868692,5.11454240778225,-3.87317034519028));
#35252=CARTESIAN_POINT('Ctrl Pts',(38.6255544971408,5.58111241365379,-7.48823335803965));
#35253=CARTESIAN_POINT('Ctrl Pts',(39.6930432805366,5.85674647908816,-9.12349227712411));
#35254=CARTESIAN_POINT('Ctrl Pts',(42.3830122692892,6.49764533220215,-11.8775764776452));
#35255=CARTESIAN_POINT('Ctrl Pts',(43.9848454910782,6.8501065376293,-12.9726927515247));
#35256=CARTESIAN_POINT('Ctrl Pts',(47.5261065109178,7.61840266564566,-14.4683433355115));
#35257=CARTESIAN_POINT('Ctrl Pts',(49.4177181995078,8.01228979376185,-14.8498038985861));
#35258=CARTESIAN_POINT('Ctrl Pts',(51.3249084414063,8.41417681322607,-14.8500516281495));
#35259=CARTESIAN_POINT('Ctrl Pts',(37.6428571267913,4.07974739676227,1.59674356901122));
#35260=CARTESIAN_POINT('Ctrl Pts',(37.6140009933336,4.11636747459116,1.15301418851043));
#35261=CARTESIAN_POINT('Ctrl Pts',(37.5712498180838,4.15554717391331,0.635579075421461));
#35262=CARTESIAN_POINT('Ctrl Pts',(37.5462016739414,4.32354021342426,-1.86860431095391));
#35263=CARTESIAN_POINT('Ctrl Pts',(37.8928601802626,4.49532708288615,-3.70979114470765));
#35264=CARTESIAN_POINT('Ctrl Pts',(39.2713030320377,4.95177211901035,-7.17014261468797));
#35265=CARTESIAN_POINT('Ctrl Pts',(40.2938806509913,5.2215308480374,-8.736705744732));
#35266=CARTESIAN_POINT('Ctrl Pts',(42.8673335718703,5.84541678129212,-11.3734544105331));
#35267=CARTESIAN_POINT('Ctrl Pts',(44.4017327311872,6.18876436208449,-12.4221714958281));
#35268=CARTESIAN_POINT('Ctrl Pts',(47.7892355626643,6.9340685662168,-13.8545909095575));
#35269=CARTESIAN_POINT('Ctrl Pts',(49.6024712046817,7.31741049756506,-14.2195188100863));
#35270=CARTESIAN_POINT('Ctrl Pts',(51.4265873271606,7.70702829356553,-14.2201291128083));
#35271=CARTESIAN_POINT('Ctrl Pts',(37.2260157227863,6.55512420987368,0.));
#35272=CARTESIAN_POINT('Ctrl Pts',(37.2086313911938,6.68066728815551,-1.86858636171891));
#35273=CARTESIAN_POINT('Ctrl Pts',(37.5526056149563,6.85206832386134,-3.7102999587003));
#35274=CARTESIAN_POINT('Ctrl Pts',(38.934044247035,7.30894385840886,-7.16936247493491));
#35275=CARTESIAN_POINT('Ctrl Pts',(39.9547842114115,7.57843851744906,-8.73699595770386));
#35276=CARTESIAN_POINT('Ctrl Pts',(41.3727684379698,7.92216638570883,-10.1890856763496));
#35277=CARTESIAN_POINT('Ctrl Pts',(41.5062424636367,7.95422644864134,-10.3203928635163));
#35278=CARTESIAN_POINT('Ctrl Pts',(41.6421750134739,7.98660763468041,-10.4488603765993));
#35279=CARTESIAN_POINT('Ctrl Pts',(37.5648924257372,4.19818497005497,3.88578058618805E-16));
#35280=CARTESIAN_POINT('Ctrl Pts',(37.5462016739414,4.32354021342426,-1.86860431095391));
#35281=CARTESIAN_POINT('Ctrl Pts',(37.8928601802626,4.49532708288615,-3.70979114470765));
#35282=CARTESIAN_POINT('Ctrl Pts',(39.2713030320377,4.95177211901035,-7.17014261468797));
#35283=CARTESIAN_POINT('Ctrl Pts',(40.2938806509913,5.2215308480374,-8.736705744732));
#35284=CARTESIAN_POINT('Ctrl Pts',(41.7187350432347,5.56696037000169,-10.1966053555729));
#35285=CARTESIAN_POINT('Ctrl Pts',(41.8597170717888,5.60080882153324,-10.3350231942292));
#35286=CARTESIAN_POINT('Ctrl Pts',(42.0034439406476,5.63501657134798,-10.4702558451016));
#35287=CARTESIAN_POINT('Ctrl Pts',(43.5542911395533,9.61961280540173,1.24689076028089));
#35288=CARTESIAN_POINT('Ctrl Pts',(43.52290486313,9.65944377882137,0.764254616120504));
#35289=CARTESIAN_POINT('Ctrl Pts',(43.4920933360762,9.69641089756346,0.332948654586433));
#35290=CARTESIAN_POINT('Ctrl Pts',(43.4711606313105,9.86000510220811,-0.97887000271989));
#35291=CARTESIAN_POINT('Ctrl Pts',(43.6468834551771,10.0151469714622,-1.98783577087993));
#35292=CARTESIAN_POINT('Ctrl Pts',(44.3622799728308,10.3669195547339,-3.80852727284503));
#35293=CARTESIAN_POINT('Ctrl Pts',(44.901394722402,10.5733099858341,-4.65544360723717));
#35294=CARTESIAN_POINT('Ctrl Pts',(46.2483520959891,11.0181031366242,-6.04997283341623));
#35295=CARTESIAN_POINT('Ctrl Pts',(47.0653855748544,11.2644521757558,-6.61832169905383));
#35296=CARTESIAN_POINT('Ctrl Pts',(48.8360900223635,11.7679552730305,-7.36768403076287));
#35297=CARTESIAN_POINT('Ctrl Pts',(49.8178835406694,12.0392336678406,-7.57138648671366));
#35298=CARTESIAN_POINT('Ctrl Pts',(50.7663303683513,12.2996772587577,-7.56962581969442));
#35299=CARTESIAN_POINT('Ctrl Pts',(41.6937446593044,8.15308801979167,1.35489314066098));
#35300=CARTESIAN_POINT('Ctrl Pts',(41.6631386548959,8.19192878357257,0.884255472089525));
#35301=CARTESIAN_POINT('Ctrl Pts',(41.6286557481959,8.22957992923818,0.426396927831693));
#35302=CARTESIAN_POINT('Ctrl Pts',(41.6066335880765,8.3945585188291,-1.25360819500777));
#35303=CARTESIAN_POINT('Ctrl Pts',(41.834861409093,8.55480021407296,-2.51960912779223));
#35304=CARTESIAN_POINT('Ctrl Pts',(42.7553095590059,8.93893907695881,-4.84647586782858));
#35305=CARTESIAN_POINT('Ctrl Pts',(43.4435219166219,9.1648695806861,-5.9157219904738));
#35306=CARTESIAN_POINT('Ctrl Pts',(45.169276232732,9.66497447126936,-7.69376028691332));
#35307=CARTESIAN_POINT('Ctrl Pts',(46.2077116350196,9.94125939867244,-8.41063186558128));
#35308=CARTESIAN_POINT('Ctrl Pts',(48.4777910626938,10.5194460361889,-9.37059840618501));
#35309=CARTESIAN_POINT('Ctrl Pts',(49.7162403038048,10.8253352376576,-9.62435378619477));
#35310=CARTESIAN_POINT('Ctrl Pts',(50.9351093861917,11.1256510703083,-9.62320046360551));
#35311=CARTESIAN_POINT('Ctrl Pts',(39.5830751094924,7.07831661167166,1.47293185433847));
#35312=CARTESIAN_POINT('Ctrl Pts',(39.5533201442405,7.11607735826543,1.01538086898131));
#35313=CARTESIAN_POINT('Ctrl Pts',(39.5148560779746,7.15447823086686,0.528580691589297));
#35314=CARTESIAN_POINT('Ctrl Pts',(39.4920354699322,7.3210271226842,-1.55402875454293));
#35315=CARTESIAN_POINT('Ctrl Pts',(39.7770748570079,7.486758868588,-3.10121432123517));
#35316=CARTESIAN_POINT('Ctrl Pts',(40.9224179890784,7.90638666804373,-5.98129145450895));
#35317=CARTESIAN_POINT('Ctrl Pts',(41.7732553395417,8.15362486975184,-7.29389406576261));
#35318=CARTESIAN_POINT('Ctrl Pts',(43.9133708492461,8.71423422838807,-9.49113593804405));
#35319=CARTESIAN_POINT('Ctrl Pts',(45.1936639793709,9.02321881659059,-10.3708286017369));
#35320=CARTESIAN_POINT('Ctrl Pts',(48.010079163986,9.68311056587906,-11.5604045561052));
#35321=CARTESIAN_POINT('Ctrl Pts',(49.5289994535062,10.0267902081681,-11.8694761541095));
#35322=CARTESIAN_POINT('Ctrl Pts',(51.0436262593386,10.3707439991142,-11.8687142284812));
#35323=CARTESIAN_POINT('Ctrl Pts',(37.3033966274915,6.43660260973346,1.59647061166179));
#35324=CARTESIAN_POINT('Ctrl Pts',(37.2745307626595,6.47323503721765,1.15259158904714));
#35325=CARTESIAN_POINT('Ctrl Pts',(37.2319287549545,6.51242252436852,0.635572970245465));
#35326=CARTESIAN_POINT('Ctrl Pts',(37.2086313911938,6.68066728815551,-1.86858636171891));
#35327=CARTESIAN_POINT('Ctrl Pts',(37.5526056149563,6.85206832386134,-3.7102999587003));
#35328=CARTESIAN_POINT('Ctrl Pts',(38.934044247035,7.30894385840886,-7.16936247493491));
#35329=CARTESIAN_POINT('Ctrl Pts',(39.9547842114115,7.57843851744906,-8.73699595770386));
#35330=CARTESIAN_POINT('Ctrl Pts',(42.5289010478496,8.20241985396081,-11.3730256982159));
#35331=CARTESIAN_POINT('Ctrl Pts',(44.0622129909515,8.5456112103854,-12.4235805192521));
#35332=CARTESIAN_POINT('Ctrl Pts',(47.4509287397227,9.29108967269768,-13.8529470821302));
#35333=CARTESIAN_POINT('Ctrl Pts',(49.263355378306,9.67429759302916,-14.2204718556739));
#35334=CARTESIAN_POINT('Ctrl Pts',(51.0877106274638,10.0639675197017,-14.2198708430667));
#35335=CARTESIAN_POINT('Ctrl Pts',(37.6428571267913,4.07974739676227,1.59674356901122));
#35336=CARTESIAN_POINT('Ctrl Pts',(37.6140009933336,4.11636747459113,1.15301418851043));
#35337=CARTESIAN_POINT('Ctrl Pts',(37.5712498180838,4.15554717391332,0.635579075421461));
#35338=CARTESIAN_POINT('Ctrl Pts',(37.5462016739414,4.32354021342426,-1.86860431095391));
#35339=CARTESIAN_POINT('Ctrl Pts',(37.8928601802626,4.49532708288675,-3.70979114470885));
#35340=CARTESIAN_POINT('Ctrl Pts',(39.2713030320377,4.95177211900975,-7.17014261468677));
#35341=CARTESIAN_POINT('Ctrl Pts',(40.2938806509865,5.221530848038,-8.736705744732));
#35342=CARTESIAN_POINT('Ctrl Pts',(42.867333571875,5.84541678129152,-11.3734544105331));
#35343=CARTESIAN_POINT('Ctrl Pts',(44.4017327311872,6.18876436208449,-12.4221714958282));
#35344=CARTESIAN_POINT('Ctrl Pts',(47.7892355626643,6.9340685662168,-13.8545909095575));
#35345=CARTESIAN_POINT('Ctrl Pts',(49.6024712046821,7.31741049756335,-14.2195188100863));
#35346=CARTESIAN_POINT('Ctrl Pts',(51.4265873271606,7.70702829356553,-14.2201291128083));
#35347=CARTESIAN_POINT('Ctrl Pts',(40.0109749372547,4.10743210000906,1.47327592501251));
#35348=CARTESIAN_POINT('Ctrl Pts',(39.9812322386681,4.14517727950216,1.01591356789114));
#35349=CARTESIAN_POINT('Ctrl Pts',(39.9425801423883,4.18356833531983,0.528588387341121));
#35350=CARTESIAN_POINT('Ctrl Pts',(39.9175526247866,4.34979992137089,-1.55405138007544));
#35351=CARTESIAN_POINT('Ctrl Pts',(40.2059756280488,4.51601802193941,-3.1005729464062));
#35352=CARTESIAN_POINT('Ctrl Pts',(41.3475424919703,4.93510316561798,-5.9822748433466));
#35353=CARTESIAN_POINT('Ctrl Pts',(42.2006962594468,5.18267423522182,-7.29352824387409));
#35354=CARTESIAN_POINT('Ctrl Pts',(44.3399748842815,5.74316333527757,-9.49167634238358));
#35355=CARTESIAN_POINT('Ctrl Pts',(45.6216384820559,6.05234484883939,-10.3690524867496));
#35356=CARTESIAN_POINT('Ctrl Pts',(48.4365247491596,6.71201694062345,-11.5624766483647));
#35357=CARTESIAN_POINT('Ctrl Pts',(49.9564645932056,7.05586981550164,-11.8682745706924));
#35358=CARTESIAN_POINT('Ctrl Pts',(51.4707901907297,7.39975358641479,-11.8690397849987));
#35359=CARTESIAN_POINT('Ctrl Pts',(42.3391654916811,3.67196736957026,1.35541211815624));
#35360=CARTESIAN_POINT('Ctrl Pts',(42.3085779896465,3.71078465278407,0.885058966158364));
#35361=CARTESIAN_POINT('Ctrl Pts',(42.2738114686987,3.7484209913462,0.426408535685267));
#35362=CARTESIAN_POINT('Ctrl Pts',(42.2484605261895,3.91292097417181,-1.2536423221307));
#35363=CARTESIAN_POINT('Ctrl Pts',(42.4817920098845,4.07389626034862,-2.51864171287515));
#35364=CARTESIAN_POINT('Ctrl Pts',(43.3965442422595,4.45721661076415,-4.84795915807873));
#35365=CARTESIAN_POINT('Ctrl Pts',(44.0882505573344,4.68364919432671,-5.91517020463247));
#35366=CARTESIAN_POINT('Ctrl Pts',(45.8127425618267,5.18357269340712,-7.69457540343052));
#35367=CARTESIAN_POINT('Ctrl Pts',(46.8532451029934,5.46015465231276,-8.40795287032088));
#35368=CARTESIAN_POINT('Ctrl Pts',(49.1210183946222,6.03800997039568,-9.37372383746844));
#35369=CARTESIAN_POINT('Ctrl Pts',(50.3610047225093,6.3441696742926,-9.6225408601964));
#35370=CARTESIAN_POINT('Ctrl Pts',(51.5794202324977,6.64437068472149,-9.62369151535374));
#35371=CARTESIAN_POINT('Ctrl Pts',(44.5379552064474,2.79008834334071,1.24768171633314));
#35372=CARTESIAN_POINT('Ctrl Pts',(44.5065971288807,2.82988353082186,0.765479194261193));
#35373=CARTESIAN_POINT('Ctrl Pts',(44.4753533549286,2.86682808255862,0.332966345723582));
#35374=CARTESIAN_POINT('Ctrl Pts',(44.4493473654757,3.02969285881443,-0.978922014714018));
#35375=CARTESIAN_POINT('Ctrl Pts',(44.6328485090626,3.18595276920499,-1.98636136651458));
#35376=CARTESIAN_POINT('Ctrl Pts',(45.3395640713933,3.53647788529764,-3.81078790536211));
#35377=CARTESIAN_POINT('Ctrl Pts',(45.8840038433944,3.74363351929919,-4.65460264909031));
#35378=CARTESIAN_POINT('Ctrl Pts',(47.2290373705107,4.18815021742991,-6.05121512494211));
#35379=CARTESIAN_POINT('Ctrl Pts',(48.0492213058428,4.43495195223039,-6.61423873295915));
#35380=CARTESIAN_POINT('Ctrl Pts',(49.8164110494045,4.9379500967639,-7.37244739490483));
#35381=CARTESIAN_POINT('Ctrl Pts',(50.8005446234618,5.20966094390348,-7.56862230199509));
#35382=CARTESIAN_POINT('Ctrl Pts',(51.7483027430072,5.46990934942745,-7.57037421505989));
#35383=CARTESIAN_POINT('Ctrl Pts',(37.8397258902528,1.0622604283696,1.59647049649025));
#35384=CARTESIAN_POINT('Ctrl Pts',(37.8339627771316,1.07222001191037,1.48695569078595));
#35385=CARTESIAN_POINT('Ctrl Pts',(37.8282008616259,1.08217829864126,1.37746392936641));
#35386=CARTESIAN_POINT('Ctrl Pts',(37.803637843476,1.12462383849689,0.910698635110369));
#35387=CARTESIAN_POINT('Ctrl Pts',(37.7798283754123,1.15759409919791,0.486448413031079));
#35388=CARTESIAN_POINT('Ctrl Pts',(37.7806592587321,1.31732736909012,-1.86858636174431));
#35389=CARTESIAN_POINT('Ctrl Pts',(38.1455252315258,1.43803115335118,-3.71029995870316));
#35390=CARTESIAN_POINT('Ctrl Pts',(39.5779229780183,1.69365713822224,-7.16936247493209));
#35391=CARTESIAN_POINT('Ctrl Pts',(40.6266263701611,1.81514228728193,-8.73699595769941));
#35392=CARTESIAN_POINT('Ctrl Pts',(43.2633442117545,2.06643737216945,-11.3730256982204));
#35393=CARTESIAN_POINT('Ctrl Pts',(44.8298904725261,2.18792249429946,-12.4235805192368));
#35394=CARTESIAN_POINT('Ctrl Pts',(48.290206627889,2.44354852691157,-13.8529470821456));
#35395=CARTESIAN_POINT('Ctrl Pts',(50.138721549822,2.56492073913256,-14.2204718556691));
#35396=CARTESIAN_POINT('Ctrl Pts',(51.9999633056261,2.69099156569408,-14.2198708430667));
#35397=CARTESIAN_POINT('Ctrl Pts',(37.2107726459064,0.347755560296454,1.62964593809789));
#35398=CARTESIAN_POINT('Ctrl Pts',(37.2050094709227,0.35771525074062,1.52012995689155));
#35399=CARTESIAN_POINT('Ctrl Pts',(37.1992477086583,0.367673423350967,1.4106409479282));
#35400=CARTESIAN_POINT('Ctrl Pts',(37.1746843010492,0.410118993966263,0.943868932648104));
#35401=CARTESIAN_POINT('Ctrl Pts',(37.1499314621533,0.443150337937791,0.508392298460196));
#35402=CARTESIAN_POINT('Ctrl Pts',(37.1502632733139,0.603323715727814,-1.95287905124252));
#35403=CARTESIAN_POINT('Ctrl Pts',(37.5316956084151,0.723283698694339,-3.87337387079016));
#35404=CARTESIAN_POINT('Ctrl Pts',(39.0273309715468,0.979785618832962,-7.48792130213564));
#35405=CARTESIAN_POINT('Ctrl Pts',(40.1224384633774,1.10069469071835,-9.12360836230794));
#35406=CARTESIAN_POINT('Ctrl Pts',(42.87650515713,1.35224759481403,-11.8774049927233));
#35407=CARTESIAN_POINT('Ctrl Pts',(44.51175513264,1.47315665467739,-12.9732563608865));
#35408=CARTESIAN_POINT('Ctrl Pts',(48.1268013089989,1.72965859379905,-14.4676858045483));
#35409=CARTESIAN_POINT('Ctrl Pts',(50.0548871962082,1.850325392223,-14.8501851005389));
#35410=CARTESIAN_POINT('Ctrl Pts',(51.9999570907663,1.97670704765929,-14.8499483202528));
#35411=CARTESIAN_POINT('Ctrl Pts',(37.2110085708707,-0.604714876209846,
1.62975512103766));
#35412=CARTESIAN_POINT('Ctrl Pts',(37.2052453954626,-0.594755185033613,
1.52023913178141));
#35413=CARTESIAN_POINT('Ctrl Pts',(37.1994836453944,-0.584797013151259,
1.41075014108546));
#35414=CARTESIAN_POINT('Ctrl Pts',(37.174920187614,-0.542351442553382,0.943978082258184));
#35415=CARTESIAN_POINT('Ctrl Pts',(37.1500689010425,-0.509320134040885,
0.508394167547144));
#35416=CARTESIAN_POINT('Ctrl Pts',(37.1497353315483,-0.349146756273058,
-1.95288623093576));
#35417=CARTESIAN_POINT('Ctrl Pts',(37.5322524147587,-0.229186815991632,
-3.8731703451907));
#35418=CARTESIAN_POINT('Ctrl Pts',(39.0266771563473,0.0273151951141526,
-7.48823335803926));
#35419=CARTESIAN_POINT('Ctrl Pts',(40.1225272605589,0.148224209648788,-9.12349227712685));
#35420=CARTESIAN_POINT('Ctrl Pts',(42.8763256602578,0.399777134881894,-11.8775764776425));
#35421=CARTESIAN_POINT('Ctrl Pts',(44.5120149889433,0.520686157637575,-12.9726927515332));
#35422=CARTESIAN_POINT('Ctrl Pts',(48.1265710168889,0.777188149417136,-14.468343335503));
#35423=CARTESIAN_POINT('Ctrl Pts',(50.0549848089105,0.897861662882116,-14.8498038985576));
#35424=CARTESIAN_POINT('Ctrl Pts',(51.9999570902568,1.02423658127858,-14.8500516281495));
#35425=CARTESIAN_POINT('Ctrl Pts',(37.8403157026637,-1.31891566289614,1.59674345383971));
#35426=CARTESIAN_POINT('Ctrl Pts',(37.8345525884796,-1.30895607752527,1.48722862801069));
#35427=CARTESIAN_POINT('Ctrl Pts',(37.828790703466,-1.29899779261428,1.37773691225954));
#35428=CARTESIAN_POINT('Ctrl Pts',(37.8042275598881,-1.25655225280221,0.910971509135609));
#35429=CARTESIAN_POINT('Ctrl Pts',(37.7801719726404,-1.22358208074877,0.486453085748451));
#35430=CARTESIAN_POINT('Ctrl Pts',(37.779339404299,-1.06384881091203,-1.8686043109774));
#35431=CARTESIAN_POINT('Ctrl Pts',(38.1469172474041,-0.943145133364113,
-3.7097911447081));
#35432=CARTESIAN_POINT('Ctrl Pts',(39.5762884400003,-0.687518921074427,
-7.17014261468754));
#35433=CARTESIAN_POINT('Ctrl Pts',(40.6268483631124,-0.566033915391893,
-8.7367057447395));
#35434=CARTESIAN_POINT('Ctrl Pts',(43.2628954695764,-0.31473877766099,-11.3734544105255));
#35435=CARTESIAN_POINT('Ctrl Pts',(44.8305401132913,-0.193253748299652,
-12.4221714958415));
#35436=CARTESIAN_POINT('Ctrl Pts',(48.2896308976067,0.0623724159563386,
-13.8545909095442));
#35437=CARTESIAN_POINT('Ctrl Pts',(50.1389656602224,0.183762141962158,-14.2195188100102));
#35438=CARTESIAN_POINT('Ctrl Pts',(51.9999633043522,0.309815399742307,-14.2201291128083));
#35439=CARTESIAN_POINT('Ctrl Pts',(37.78,1.19058808997869,0.));
#35440=CARTESIAN_POINT('Ctrl Pts',(37.7806592587321,1.31732736909012,-1.86858636174431));
#35441=CARTESIAN_POINT('Ctrl Pts',(38.1455252315258,1.43803115335118,-3.71029995870316));
#35442=CARTESIAN_POINT('Ctrl Pts',(39.5779229780183,1.69365713822224,-7.16936247493209));
#35443=CARTESIAN_POINT('Ctrl Pts',(40.6266263701611,1.81514228728193,-8.73699595769941));
#35444=CARTESIAN_POINT('Ctrl Pts',(42.079095137833,1.95357130555262,-10.1890856763502));
#35445=CARTESIAN_POINT('Ctrl Pts',(42.2157732130433,1.96630970889328,-10.3203928635173));
#35446=CARTESIAN_POINT('Ctrl Pts',(42.3549304887758,1.97901608230145,-10.4488603766003));
#35447=CARTESIAN_POINT('Ctrl Pts',(37.7799999998341,-1.19058808946242,-4.87766813886054E-9));
#35448=CARTESIAN_POINT('Ctrl Pts',(37.7793394048005,-1.0638488105451,-1.86860431420344));
#35449=CARTESIAN_POINT('Ctrl Pts',(38.1469172479177,-0.943145133125576,
-3.70979114624586));
#35450=CARTESIAN_POINT('Ctrl Pts',(38.8616028436213,-0.815332027121487,
-5.43996687972834));
#35451=CARTESIAN_POINT('Ctrl Pts',(39.5762884399489,-0.687518921005817,
-7.17014261472125));
#35452=CARTESIAN_POINT('Ctrl Pts',(40.6268483630872,-0.566033915352764,
-8.73670574476311));
#35453=CARTESIAN_POINT('Ctrl Pts',(41.9448719163384,-0.440386346516728,
-10.0550800776386));
#35454=CARTESIAN_POINT('Ctrl Pts',(42.0863595386707,-0.426898290311208,
-10.1966053555765));
#35455=CARTESIAN_POINT('Ctrl Pts',(42.2307237103618,-0.41345820180873,-10.3350231942305));
#35456=CARTESIAN_POINT('Ctrl Pts',(42.3778559173178,-0.400053103664619,
-10.470255845101));
#35457=CARTESIAN_POINT('Ctrl Pts',(44.4799848904464,3.32327712821972,1.24689064510934));
#35458=CARTESIAN_POINT('Ctrl Pts',(44.4742224279398,3.33323558739414,1.13738820285035));
#35459=CARTESIAN_POINT('Ctrl Pts',(44.4684589625378,3.34319507469509,1.02786748900887));
#35460=CARTESIAN_POINT('Ctrl Pts',(44.4438997771526,3.38564028976811,0.56117289744884));
#35461=CARTESIAN_POINT('Ctrl Pts',(44.4295022685185,3.41796558601113,0.254828874445209));
#35462=CARTESIAN_POINT('Ctrl Pts',(44.4319119278293,3.5730532724159,-0.978870002679086));
#35463=CARTESIAN_POINT('Ctrl Pts',(44.6279251367323,3.70160805589233,-1.98783577088195));
#35464=CARTESIAN_POINT('Ctrl Pts',(45.386102407664,3.94798856175628,-3.80852727284305));
#35465=CARTESIAN_POINT('Ctrl Pts',(45.9491021672716,4.07555420745019,-4.65544360723259));
#35466=CARTESIAN_POINT('Ctrl Pts',(47.3456501222045,4.32412798455813,-6.04997283342086));
#35467=CARTESIAN_POINT('Ctrl Pts',(48.1894265020301,4.45169355820927,-6.61832169901019));
#35468=CARTESIAN_POINT('Ctrl Pts',(50.0137636932357,4.69807420295008,-7.36768403080661));
#35469=CARTESIAN_POINT('Ctrl Pts',(51.0241709100486,4.82686758914895,-7.57138648680884));
#35470=CARTESIAN_POINT('Ctrl Pts',(52.000028904099,4.9496821828336,-7.56962581969449));
#35471=CARTESIAN_POINT('Ctrl Pts',(42.429667852992,2.13646282180974,1.35489302548942));
#35472=CARTESIAN_POINT('Ctrl Pts',(42.4239051893647,2.14642162855157,1.24538676140638));
#35473=CARTESIAN_POINT('Ctrl Pts',(42.4181422088106,2.15638074475633,1.13587499712206));
#35474=CARTESIAN_POINT('Ctrl Pts',(42.393581814172,2.19882606010976,0.669158551015892));
#35475=CARTESIAN_POINT('Ctrl Pts',(42.3762274914793,2.23135049600752,0.326351368873808));
#35476=CARTESIAN_POINT('Ctrl Pts',(42.3778082879602,2.38787268687572,-1.25360819498701));
#35477=CARTESIAN_POINT('Ctrl Pts',(42.6265178497614,2.51400314727895,-2.51960912779653));
#35478=CARTESIAN_POINT('Ctrl Pts',(43.592265824835,2.76323860082472,-4.84647586782431));
#35479=CARTESIAN_POINT('Ctrl Pts',(44.3056264360906,2.88892662741303,-5.91572199047166));
#35480=CARTESIAN_POINT('Ctrl Pts',(46.0849874081721,3.13834072491811,-7.69376028691551));
#35481=CARTESIAN_POINT('Ctrl Pts',(47.1521724801633,3.26402870377935,-8.41063186555665));
#35482=CARTESIAN_POINT('Ctrl Pts',(49.481430310228,3.51326424840639,-9.3705984062097));
#35483=CARTESIAN_POINT('Ctrl Pts',(50.7508064960181,3.63979023543883,-9.62435378624233));
#35484=CARTESIAN_POINT('Ctrl Pts',(52.0000086477592,3.76358612954873,-9.62320046360555));
#35485=CARTESIAN_POINT('Ctrl Pts',(40.1875259567355,1.37301063256203,1.47293173916693));
#35486=CARTESIAN_POINT('Ctrl Pts',(40.1817630734217,1.38296981895596,1.36342130045779));
#35487=CARTESIAN_POINT('Ctrl Pts',(40.1760006162045,1.39292852977775,1.25391931221354));
#35488=CARTESIAN_POINT('Ctrl Pts',(40.1514389273988,1.43537395479689,0.78717899271973));
#35489=CARTESIAN_POINT('Ctrl Pts',(40.1309065737656,1.46811616862065,0.404559744697675));
#35490=CARTESIAN_POINT('Ctrl Pts',(40.1319542826336,1.6262069816417,-1.55402875454452));
#35491=CARTESIAN_POINT('Ctrl Pts',(40.4376784663362,1.7496864830589,-3.10121432123695));
#35492=CARTESIAN_POINT('Ctrl Pts',(41.6310829191998,2.00204375396605,-5.98129145450721));
#35493=CARTESIAN_POINT('Ctrl Pts',(42.5084456369411,2.12567864734774,-7.29389406576051));
#35494=CARTESIAN_POINT('Ctrl Pts',(44.7065608867256,2.37601161837676,-9.49113593804618));
#35495=CARTESIAN_POINT('Ctrl Pts',(46.0177955705402,2.49964647926445,-10.3708286017169));
#35496=CARTESIAN_POINT('Ctrl Pts',(48.8994560970704,2.75200381047966,-11.5604045561253));
#35497=CARTESIAN_POINT('Ctrl Pts',(50.4518266808763,2.87602039418504,-11.8694761541333));
#35498=CARTESIAN_POINT('Ctrl Pts',(51.9999864978575,3.00091936260147,-11.8687142284813));
#35499=CARTESIAN_POINT('Ctrl Pts',(37.8397258902528,1.0622604283696,1.59647049649025));
#35500=CARTESIAN_POINT('Ctrl Pts',(37.8339627771316,1.07222001191037,1.48695569078595));
#35501=CARTESIAN_POINT('Ctrl Pts',(37.8282008616259,1.08217829864126,1.37746392936641));
#35502=CARTESIAN_POINT('Ctrl Pts',(37.803637843476,1.12462383849689,0.910698635110369));
#35503=CARTESIAN_POINT('Ctrl Pts',(37.7798283754123,1.15759409919791,0.486448413031079));
#35504=CARTESIAN_POINT('Ctrl Pts',(37.7806592587321,1.31732736909012,-1.86858636174431));
#35505=CARTESIAN_POINT('Ctrl Pts',(38.1455252315258,1.43803115335118,-3.71029995870316));
#35506=CARTESIAN_POINT('Ctrl Pts',(39.5779229780183,1.69365713822224,-7.16936247493209));
#35507=CARTESIAN_POINT('Ctrl Pts',(40.6266263701611,1.81514228728193,-8.73699595769941));
#35508=CARTESIAN_POINT('Ctrl Pts',(43.2633442117545,2.06643737216945,-11.3730256982204));
#35509=CARTESIAN_POINT('Ctrl Pts',(44.8298904725261,2.18792249429946,-12.4235805192368));
#35510=CARTESIAN_POINT('Ctrl Pts',(48.290206627889,2.44354852691157,-13.8529470821456));
#35511=CARTESIAN_POINT('Ctrl Pts',(50.138721549822,2.56492073913256,-14.2204718556691));
#35512=CARTESIAN_POINT('Ctrl Pts',(51.9999633056261,2.69099156569408,-14.2198708430667));
#35513=CARTESIAN_POINT('Ctrl Pts',(37.8403157026637,-1.31891566289614,1.59674345383971));
#35514=CARTESIAN_POINT('Ctrl Pts',(37.8345525884796,-1.30895607752529,1.48722862801069));
#35515=CARTESIAN_POINT('Ctrl Pts',(37.828790703466,-1.29899779261428,1.37773691225954));
#35516=CARTESIAN_POINT('Ctrl Pts',(37.8042275598881,-1.25655225280221,0.910971509135609));
#35517=CARTESIAN_POINT('Ctrl Pts',(37.7801719726404,-1.22358208074877,0.486453085748451));
#35518=CARTESIAN_POINT('Ctrl Pts',(37.779339404299,-1.06384881091203,-1.8686043109774));
#35519=CARTESIAN_POINT('Ctrl Pts',(38.1469172474041,-0.943145133364111,
-3.7097911447081));
#35520=CARTESIAN_POINT('Ctrl Pts',(39.5762884400003,-0.68751892107443,-7.17014261468754));
#35521=CARTESIAN_POINT('Ctrl Pts',(40.6268483631172,-0.566033915391893,
-8.7367057447419));
#35522=CARTESIAN_POINT('Ctrl Pts',(43.2628954695716,-0.31473877766099,-11.3734544105232));
#35523=CARTESIAN_POINT('Ctrl Pts',(44.8305401132913,-0.193253748299652,
-12.4221714958415));
#35524=CARTESIAN_POINT('Ctrl Pts',(48.2896308976067,0.0623724159563386,
-13.8545909095442));
#35525=CARTESIAN_POINT('Ctrl Pts',(50.1389656602224,0.183762141962158,-14.2195188100102));
#35526=CARTESIAN_POINT('Ctrl Pts',(51.9999633043522,0.309815399742307,-14.2201291128083));
#35527=CARTESIAN_POINT('Ctrl Pts',(40.1882694324257,-1.62853105321875,1.47327580984102));
#35528=CARTESIAN_POINT('Ctrl Pts',(40.1825065477754,-1.61857186451787,1.3637653457639));
#35529=CARTESIAN_POINT('Ctrl Pts',(40.1767441289915,-1.60861315599014,1.25426341508618));
#35530=CARTESIAN_POINT('Ctrl Pts',(40.1521822820784,-1.56616773102595,0.787522958361224));
#35531=CARTESIAN_POINT('Ctrl Pts',(40.1313396880605,-1.53342562894499,0.404565634793769));
#35532=CARTESIAN_POINT('Ctrl Pts',(40.1302905677502,-1.37533481599403,-1.55405138007464));
#35533=CARTESIAN_POINT('Ctrl Pts',(40.4394331428155,-1.25185544909165,-3.10057294640437));
#35534=CARTESIAN_POINT('Ctrl Pts',(41.6290225365131,-0.999497891516836,
-5.98227484334843));
#35535=CARTESIAN_POINT('Ctrl Pts',(42.5087254655197,-0.87586317886622,-7.29352824389111));
#35536=CARTESIAN_POINT('Ctrl Pts',(44.7059952341549,-0.62553014122646,-9.49167634236655));
#35537=CARTESIAN_POINT('Ctrl Pts',(46.018614461608,-0.501895397277342,-10.3690524867728));
#35538=CARTESIAN_POINT('Ctrl Pts',(48.898730372315,-0.249537900119364,-11.5624766483416));
#35539=CARTESIAN_POINT('Ctrl Pts',(50.4521347865894,-0.125494944822144,
-11.8682745705925));
#35540=CARTESIAN_POINT('Ctrl Pts',(51.9999864962518,-0.000622417323211651,
-11.8690397849987));
#35541=CARTESIAN_POINT('Ctrl Pts',(42.4307892712953,-2.39089944281272,1.35541200298475));
#35542=CARTESIAN_POINT('Ctrl Pts',(42.4250266056522,-2.38094063259133,1.24590570063802));
#35543=CARTESIAN_POINT('Ctrl Pts',(42.4192636830689,-2.37098151984669,1.13639402318395));
#35544=CARTESIAN_POINT('Ctrl Pts',(42.3947030499486,-2.3285362045761,0.669677370085716));
#35545=CARTESIAN_POINT('Ctrl Pts',(42.3768807775288,-2.29601193722516,0.326360253174464));
#35546=CARTESIAN_POINT('Ctrl Pts',(42.3752988309042,-2.13948974646263,-1.25364232210634));
#35547=CARTESIAN_POINT('Ctrl Pts',(42.6291645083452,-2.01335948895392,-2.51864171287222));
#35548=CARTESIAN_POINT('Ctrl Pts',(43.5891580556312,-1.7641236030149,-4.84795915808161));
#35549=CARTESIAN_POINT('Ctrl Pts',(44.3060485143003,-1.63843584903174,-5.91517020465899));
#35550=CARTESIAN_POINT('Ctrl Pts',(46.084134208595,-1.38902165105357,-7.69457540340396));
#35551=CARTESIAN_POINT('Ctrl Pts',(47.1534076509197,-1.26333384857635,-8.40795287035376));
#35552=CARTESIAN_POINT('Ctrl Pts',(49.4803356664711,-1.01409805365085,-9.37372383743556));
#35553=CARTESIAN_POINT('Ctrl Pts',(50.7512717901641,-0.887523067774766,
-9.62254086007749));
#35554=CARTESIAN_POINT('Ctrl Pts',(52.0000086453373,-0.763776277075275,
-9.62369151535372));
#35555=CARTESIAN_POINT('Ctrl Pts',(44.4816940061638,-3.5767226147739,1.24768160116169));
#35556=CARTESIAN_POINT('Ctrl Pts',(44.4759315405831,-3.5667641502963,1.13817910058646));
#35557=CARTESIAN_POINT('Ctrl Pts',(44.4701681635331,-3.55680466826894,1.02865851907984));
#35558=CARTESIAN_POINT('Ctrl Pts',(44.445608614691,-3.51435945332208,0.561963612050326));
#35559=CARTESIAN_POINT('Ctrl Pts',(44.4304979196961,-3.48203441395558,0.25484241470743));
#35560=CARTESIAN_POINT('Ctrl Pts',(44.4280873491857,-3.32694672771197,-0.978922014667701));
#35561=CARTESIAN_POINT('Ctrl Pts',(44.6319588195988,-3.19839225346,-1.98636136651175));
#35562=CARTESIAN_POINT('Ctrl Pts',(45.3813659616932,-2.95201108860042,-3.81078790536488));
#35563=CARTESIAN_POINT('Ctrl Pts',(45.9497454423979,-2.8244458583741,-4.65460264913353));
#35564=CARTESIAN_POINT('Ctrl Pts',(47.3443497895797,-2.57587192813957,-6.05121512489886));
#35565=CARTESIAN_POINT('Ctrl Pts',(48.191308984017,-2.44830662330919,-6.61423873299696));
#35566=CARTESIAN_POINT('Ctrl Pts',(50.0120953836972,-2.20192559709628,-7.37244739486701));
#35567=CARTESIAN_POINT('Ctrl Pts',(51.0248803821898,-2.07303718496541,-7.56862230181907));
#35568=CARTESIAN_POINT('Ctrl Pts',(52.0000289004077,-1.95031777657975,-7.57037421505986));
#35569=CARTESIAN_POINT('Ctrl Pts',(37.6057474666452,-4.33370633274517,1.59647061166166));
#35570=CARTESIAN_POINT('Ctrl Pts',(37.6014604087227,-4.32302794314919,1.48695576757045));
#35571=CARTESIAN_POINT('Ctrl Pts',(37.5971743516732,-4.31235100760126,1.37746396775187));
#35572=CARTESIAN_POINT('Ctrl Pts',(37.5789019782671,-4.26684181644427,0.910698635138339));
#35573=CARTESIAN_POINT('Ctrl Pts',(37.5600270135782,-4.23081870486248,0.486448413027734));
#35574=CARTESIAN_POINT('Ctrl Pts',(37.583581854176,-4.07282953634437,-1.8685863617679));
#35575=CARTESIAN_POINT('Ctrl Pts',(37.9619119570128,-4.00528018447453,-3.71029995872063));
#35576=CARTESIAN_POINT('Ctrl Pts',(39.4161093304535,-3.95610755722229,-7.1693624749145));
#35577=CARTESIAN_POINT('Ctrl Pts',(40.4714275735129,-3.98510500541578,-8.7369959576895));
#35578=CARTESIAN_POINT('Ctrl Pts',(43.1170704487074,-4.11161181540662,-11.3730256982303));
#35579=CARTESIAN_POINT('Ctrl Pts',(44.6849606627931,-4.21430601438156,-12.4235805192282));
#35580=CARTESIAN_POINT('Ctrl Pts',(48.1464351665831,-4.45373622021211,-13.8529470821542));
#35581=CARTESIAN_POINT('Ctrl Pts',(49.9934079386735,-4.59667050425296,-14.2204718556502));
#35582=CARTESIAN_POINT('Ctrl Pts',(51.8536466863968,-4.73676521641239,-14.2198708430668));
#35583=CARTESIAN_POINT('Ctrl Pts',(36.8815114147052,-4.95142919224173,1.6296460532693));
#35584=CARTESIAN_POINT('Ctrl Pts',(36.8772243107676,-4.940750688027,1.52013003367661));
#35585=CARTESIAN_POINT('Ctrl Pts',(36.8729383891546,-4.93007388724583,1.41064098631263));
#35586=CARTESIAN_POINT('Ctrl Pts',(36.8546656346322,-4.88456461021745,0.943868932681406));
#35587=CARTESIAN_POINT('Ctrl Pts',(36.8348655943188,-4.84834678143695,0.508392298457217));
#35588=CARTESIAN_POINT('Ctrl Pts',(36.857989076486,-4.68985095930904,-1.95287905126917));
#35589=CARTESIAN_POINT('Ctrl Pts',(37.2526110659712,-4.62539547707885,-3.87337387081003));
#35590=CARTESIAN_POINT('Ctrl Pts',(38.7695270468993,-4.58435548151087,-7.48792130211559));
#35591=CARTESIAN_POINT('Ctrl Pts',(39.8706950784794,-4.62052713517624,-9.12360836230037));
#35592=CARTESIAN_POINT('Ctrl Pts',(42.6325290552245,-4.76347923311373,-11.8774049927308));
#35593=CARTESIAN_POINT('Ctrl Pts',(44.2683416970863,-4.8765211889194,-12.9732563608876));
#35594=CARTESIAN_POINT('Ctrl Pts',(47.883095947851,-5.13710478161822,-14.4676858045473));
#35595=CARTESIAN_POINT('Ctrl Pts',(49.8087293766755,-5.29206142841395,-14.8501851005199));
#35596=CARTESIAN_POINT('Ctrl Pts',(51.7519872491301,-5.44377846350007,-14.8499483202528));
#35597=CARTESIAN_POINT('Ctrl Pts',(36.7461942621622,-5.89423842867652,1.62975523620908));
#35598=CARTESIAN_POINT('Ctrl Pts',(36.741907157911,-5.88355992367708,1.52023920856652));
#35599=CARTESIAN_POINT('Ctrl Pts',(36.7376212482637,-5.87288312535188,1.41075017946966));
#35600=CARTESIAN_POINT('Ctrl Pts',(36.7193484440797,-5.82737384120054,0.943978082292227));
#35601=CARTESIAN_POINT('Ctrl Pts',(36.6994509531013,-5.79114203695372,0.508394167544537));
#35602=CARTESIAN_POINT('Ctrl Pts',(36.7219158272129,-5.63255152130492,-1.95288623096384));
#35603=CARTESIAN_POINT('Ctrl Pts',(37.1176115175746,-5.56825045708003,-3.87317034521415));
#35604=CARTESIAN_POINT('Ctrl Pts',(38.6333292122811,-5.52703808205988,-7.4882333580156));
#35605=CARTESIAN_POINT('Ctrl Pts',(39.7352322893592,-5.56331547725347,-9.12349227712403));
#35606=CARTESIAN_POINT('Ctrl Pts',(42.4968007059073,-5.70622937204501,-11.8775764776452));
#35607=CARTESIAN_POINT('Ctrl Pts',(44.1330482236775,-5.81933389105681,-12.9726927515199));
#35608=CARTESIAN_POINT('Ctrl Pts',(47.7473173225335,-6.07984767624027,-14.4683433355162));
#35609=CARTESIAN_POINT('Ctrl Pts',(49.6732762742163,-6.23484434206627,-14.849803898529));
#35610=CARTESIAN_POINT('Ctrl Pts',(51.6164365682427,-6.3865541538095,-14.8500516281494));
#35611=CARTESIAN_POINT('Ctrl Pts',(37.2674545852876,-6.69072942383213,1.59674356901113));
#35612=CARTESIAN_POINT('Ctrl Pts',(37.2631675265797,-6.68005103227416,1.4872287047953));
#35613=CARTESIAN_POINT('Ctrl Pts',(37.2588814994465,-6.66937410286626,1.37773695064445));
#35614=CARTESIAN_POINT('Ctrl Pts',(37.240609001884,-6.62386489390232,0.910971509165356));
#35615=CARTESIAN_POINT('Ctrl Pts',(37.2214904105334,-6.58780684365416,0.486453085746033));
#35616=CARTESIAN_POINT('Ctrl Pts',(37.2433987309978,-6.42958094133495,-1.86860431100456));
#35617=CARTESIAN_POINT('Ctrl Pts',(37.624413086019,-6.36241763447689,-3.70979114473031));
#35618=CARTESIAN_POINT('Ctrl Pts',(39.0756147439104,-6.31281405859542,-7.17014261466511));
#35619=CARTESIAN_POINT('Ctrl Pts',(40.13277060071,-6.34207586060887,-8.73670574474625));
#35620=CARTESIAN_POINT('Ctrl Pts',(42.7777495754168,-6.46848716273484,-11.3734544105186));
#35621=CARTESIAN_POINT('Ctrl Pts',(44.3467269792879,-6.57133776972387,-12.4221714958281));
#35622=CARTESIAN_POINT('Ctrl Pts',(47.8069886032727,-6.81059345676843,-13.8545909095574));
#35623=CARTESIAN_POINT('Ctrl Pts',(49.6547753637234,-6.95362708078685,-14.2195188099959));
#35624=CARTESIAN_POINT('Ctrl Pts',(51.5147699841783,-7.093704442186,-14.2201291128083));
#35625=CARTESIAN_POINT('Ctrl Pts',(37.5648924257371,-4.19818497005578,0.));
#35626=CARTESIAN_POINT('Ctrl Pts',(37.583581854176,-4.07282953634436,-1.86858636176791));
#35627=CARTESIAN_POINT('Ctrl Pts',(37.9619119570128,-4.00528018447453,-3.71029995872063));
#35628=CARTESIAN_POINT('Ctrl Pts',(39.4161093304535,-3.95610755722229,-7.1693624749145));
#35629=CARTESIAN_POINT('Ctrl Pts',(40.4714275735129,-3.98510500541578,-8.7369959576895));
#35630=CARTESIAN_POINT('Ctrl Pts',(41.9288128067803,-4.05479285275038,-10.1890856763502));
#35631=CARTESIAN_POINT('Ctrl Pts',(42.0659125600698,-4.06163542615967,-10.320392863517));
#35632=CARTESIAN_POINT('Ctrl Pts',(42.2054617208597,-4.06886253050386,-10.4488603765996));
#35633=CARTESIAN_POINT('Ctrl Pts',(37.2260157226955,-6.55512420933908,-4.87766791140768E-9));
#35634=CARTESIAN_POINT('Ctrl Pts',(37.2433987315464,-6.42958094104316,-1.8686043142306));
#35635=CARTESIAN_POINT('Ctrl Pts',(37.6244130865613,-6.36241763431395,-3.70979114626806));
#35636=CARTESIAN_POINT('Ctrl Pts',(38.3500139148987,-6.33761584642798,-5.43996687972819));
#35637=CARTESIAN_POINT('Ctrl Pts',(39.0756147438694,-6.31281405852036,-7.17014261469875));
#35638=CARTESIAN_POINT('Ctrl Pts',(40.1327706006907,-6.34207586056676,-8.73670574476976));
#35639=CARTESIAN_POINT('Ctrl Pts',(41.4552600880589,-6.40528151166162,-10.0550800776384));
#35640=CARTESIAN_POINT('Ctrl Pts',(41.5972271209431,-6.41206653251295,-10.196605355575));
#35641=CARTESIAN_POINT('Ctrl Pts',(41.7420345975448,-6.41930840848147,-10.3350231942279));
#35642=CARTESIAN_POINT('Ctrl Pts',(41.8895769551558,-6.42697885114752,-10.4702558450972));
#35643=CARTESIAN_POINT('Ctrl Pts',(44.5001944306518,-3.04071090848738,1.24689076028073));
#35644=CARTESIAN_POINT('Ctrl Pts',(44.4959078567059,-3.03003372440451,1.13738827962796));
#35645=CARTESIAN_POINT('Ctrl Pts',(44.4916204363964,-3.01935537993571,1.02786752740425));
#35646=CARTESIAN_POINT('Ctrl Pts',(44.4733518105209,-2.97384705570815,0.561172897423655));
#35647=CARTESIAN_POINT('Ctrl Pts',(44.463701217072,-2.93980180525762,0.254828874440047));
#35648=CARTESIAN_POINT('Ctrl Pts',(44.488157628544,-2.78663561817574,-0.97887000267835));
#35649=CARTESIAN_POINT('Ctrl Pts',(44.7004709588316,-2.68728492516155,-1.98783577086809));
#35650=CARTESIAN_POINT('Ctrl Pts',(45.4859946801691,-2.55131209325765,-3.80852727285718));
#35651=CARTESIAN_POINT('Ctrl Pts',(46.0614183982484,-2.50516810167956,-4.65544360722297));
#35652=CARTESIAN_POINT('Ctrl Pts',(47.4791272455479,-2.45787394350806,-6.04997283343074));
#35653=CARTESIAN_POINT('Ctrl Pts',(48.3324696724574,-2.45168870251593,-6.61832169902524));
#35654=CARTESIAN_POINT('Ctrl Pts',(50.1733013630956,-2.46744610981745,-7.36768403079182));
#35655=CARTESIAN_POINT('Ctrl Pts',(51.1917533012975,-2.48375959424081,-7.57138648676607));
#35656=CARTESIAN_POINT('Ctrl Pts',(52.1751568070596,-2.50107414862821,-7.56962581969462));
#35657=CARTESIAN_POINT('Ctrl Pts',(42.3018453782486,-3.92365461890892,1.35489314066083));
#35658=CARTESIAN_POINT('Ctrl Pts',(42.2975586546956,-3.91297706217431,1.24538683818609));
#35659=CARTESIAN_POINT('Ctrl Pts',(42.2932716614843,-3.90229915402469,1.13587503551432));
#35660=CARTESIAN_POINT('Ctrl Pts',(42.275001852934,-3.85679055844476,0.669158551007349));
#35661=CARTESIAN_POINT('Ctrl Pts',(42.2624528820614,-3.82212739678043,0.326351368869398));
#35662=CARTESIAN_POINT('Ctrl Pts',(42.2862930185905,-3.66742334692941,-1.25360819499453));
#35663=CARTESIAN_POINT('Ctrl Pts',(42.5504213117423,-3.57797177381408,-2.5196091277947));
#35664=CARTESIAN_POINT('Ctrl Pts',(43.5418092681772,-3.46871344469322,-4.84647586782627));
#35665=CARTESIAN_POINT('Ctrl Pts',(44.2657961681648,-3.44582654102279,-5.91572199046432));
#35666=CARTESIAN_POINT('Ctrl Pts',(46.0625411381427,-3.45218058836019,-7.69376028692298));
#35667=CARTESIAN_POINT('Ctrl Pts',(47.1367510692373,-3.47964820283172,-8.41063186557179));
#35668=CARTESIAN_POINT('Ctrl Pts',(49.4777703293181,-3.56443746806574,-9.3705984061947));
#35669=CARTESIAN_POINT('Ctrl Pts',(50.7522326212184,-3.61985039973288,-9.62435378619005));
#35670=CARTESIAN_POINT('Ctrl Pts',(52.0063376889004,-3.67509457152228,-9.62320046360564));
#35671=CARTESIAN_POINT('Ctrl Pts',(39.9738746787522,-4.36024590432593,1.47293185433834));
#35672=CARTESIAN_POINT('Ctrl Pts',(39.9695877917789,-4.3495679405393,1.36342137723986));
#35673=CARTESIAN_POINT('Ctrl Pts',(39.965301258885,-4.33889050812412,1.2539193506024));
#35674=CARTESIAN_POINT('Ctrl Pts',(39.9470301849507,-4.29338161981782,0.787178992729243));
#35675=CARTESIAN_POINT('Ctrl Pts',(39.9313665239358,-4.25805061593422,0.404559744693875));
#35676=CARTESIAN_POINT('Ctrl Pts',(39.9549022371336,-4.10171804395135,-1.55402875456025));
#35677=CARTESIAN_POINT('Ctrl Pts',(40.2750875547397,-4.02300447357647,-3.10121432124357));
#35678=CARTESIAN_POINT('Ctrl Pts',(41.4922590552009,-3.94305499753475,-5.98129145450059));
#35679=CARTESIAN_POINT('Ctrl Pts',(42.3782865653796,-3.94554026236852,-7.29389406575307));
#35680=CARTESIAN_POINT('Ctrl Pts',(44.589654267654,-4.01057973632999,-9.49113593805367));
#35681=CARTESIAN_POINT('Ctrl Pts',(45.9051375482496,-4.07481145201866,-10.3708286017226));
#35682=CARTESIAN_POINT('Ctrl Pts',(48.7933811184127,-4.2351258063533,-11.5604045561197));
#35683=CARTESIAN_POINT('Ctrl Pts',(50.3476002080607,-4.33329690122034,-11.8694761541096));
#35684=CARTESIAN_POINT('Ctrl Pts',(51.8977769668582,-4.42999533819711,-11.8687142284813));
#35685=CARTESIAN_POINT('Ctrl Pts',(37.6057474666452,-4.33370633274517,1.59647061166166));
#35686=CARTESIAN_POINT('Ctrl Pts',(37.6014604087227,-4.32302794314919,1.48695576757045));
#35687=CARTESIAN_POINT('Ctrl Pts',(37.5971743516732,-4.31235100760126,1.37746396775187));
#35688=CARTESIAN_POINT('Ctrl Pts',(37.5789019782671,-4.26684181644427,0.910698635138339));
#35689=CARTESIAN_POINT('Ctrl Pts',(37.5600270135782,-4.23081870486248,0.486448413027734));
#35690=CARTESIAN_POINT('Ctrl Pts',(37.583581854176,-4.07282953634436,-1.8685863617679));
#35691=CARTESIAN_POINT('Ctrl Pts',(37.9619119570128,-4.00528018447453,-3.71029995872063));
#35692=CARTESIAN_POINT('Ctrl Pts',(39.4161093304535,-3.95610755722229,-7.1693624749145));
#35693=CARTESIAN_POINT('Ctrl Pts',(40.4714275735129,-3.98510500541578,-8.7369959576895));
#35694=CARTESIAN_POINT('Ctrl Pts',(43.1170704487074,-4.11161181540662,-11.3730256982303));
#35695=CARTESIAN_POINT('Ctrl Pts',(44.6849606627931,-4.21430601438036,-12.4235805192282));
#35696=CARTESIAN_POINT('Ctrl Pts',(48.1464351665831,-4.45373622021331,-13.8529470821542));
#35697=CARTESIAN_POINT('Ctrl Pts',(49.9934079386734,-4.59667050425296,-14.2204718556502));
#35698=CARTESIAN_POINT('Ctrl Pts',(51.8536466863968,-4.73676521641239,-14.2198708430668));
#35699=CARTESIAN_POINT('Ctrl Pts',(37.2674545852876,-6.69072942383213,1.59674356901113));
#35700=CARTESIAN_POINT('Ctrl Pts',(37.2631675265797,-6.68005103227415,1.4872287047953));
#35701=CARTESIAN_POINT('Ctrl Pts',(37.2588814994465,-6.66937410286626,1.37773695064445));
#35702=CARTESIAN_POINT('Ctrl Pts',(37.240609001884,-6.62386489390232,0.910971509165356));
#35703=CARTESIAN_POINT('Ctrl Pts',(37.2214904105334,-6.58780684365416,0.486453085746033));
#35704=CARTESIAN_POINT('Ctrl Pts',(37.2433987309978,-6.42958094133495,-1.86860431100456));
#35705=CARTESIAN_POINT('Ctrl Pts',(37.624413086019,-6.36241763447689,-3.70979114473031));
#35706=CARTESIAN_POINT('Ctrl Pts',(39.0756147439104,-6.31281405859542,-7.17014261466511));
#35707=CARTESIAN_POINT('Ctrl Pts',(40.13277060071,-6.34207586060887,-8.73670574474625));
#35708=CARTESIAN_POINT('Ctrl Pts',(42.7777495754168,-6.46848716273484,-11.3734544105186));
#35709=CARTESIAN_POINT('Ctrl Pts',(44.3467269792879,-6.57133776972387,-12.4221714958281));
#35710=CARTESIAN_POINT('Ctrl Pts',(47.8069886032727,-6.81059345676843,-13.8545909095574));
#35711=CARTESIAN_POINT('Ctrl Pts',(49.6547753637234,-6.95362708078685,-14.2195188099959));
#35712=CARTESIAN_POINT('Ctrl Pts',(51.5147699841783,-7.093704442186,-14.2201291128083));
#35713=CARTESIAN_POINT('Ctrl Pts',(39.5474466673498,-7.33134203123383,1.47327592501242));
#35714=CARTESIAN_POINT('Ctrl Pts',(39.5431597793878,-7.32066406497413,1.36376542254622));
#35715=CARTESIAN_POINT('Ctrl Pts',(39.5388732842035,-7.3099866402986,1.25426345347434));
#35716=CARTESIAN_POINT('Ctrl Pts',(39.5206020537639,-7.26447772954601,0.787522958372976));
#35717=CARTESIAN_POINT('Ctrl Pts',(39.5046312942629,-7.22910268445771,0.404565634791133));
#35718=CARTESIAN_POINT('Ctrl Pts',(39.5260915209589,-7.07247170263716,-1.55405138009485));
#35719=CARTESIAN_POINT('Ctrl Pts',(39.8496604164864,-6.99424475322044,-3.10057294641932));
#35720=CARTESIAN_POINT('Ctrl Pts',(41.0630557304034,-6.91375205390619,-5.98227484333336));
#35721=CARTESIAN_POINT('Ctrl Pts',(41.9513996061261,-6.91657054441245,-7.29352824389794));
#35722=CARTESIAN_POINT('Ctrl Pts',(44.1619304425351,-6.98148962793616,-9.4916763423596));
#35723=CARTESIAN_POINT('Ctrl Pts',(45.4787841574493,-7.0459185004724,-10.3690524867687));
#35724=CARTESIAN_POINT('Ctrl Pts',(48.3654988573818,-7.20601286880373,-11.5624766483454));
#35725=CARTESIAN_POINT('Ctrl Pts',(49.9207450076504,-7.30430498992435,-11.8682745706019));
#35726=CARTESIAN_POINT('Ctrl Pts',(51.4706130322883,-7.40098575043949,-11.8690397849986));
#35727=CARTESIAN_POINT('Ctrl Pts',(41.6586445536367,-8.40509445805938,1.35541211815617));
#35728=CARTESIAN_POINT('Ctrl Pts',(41.6543578285897,-8.39441689759457,1.24590577741826));
#35729=CARTESIAN_POINT('Ctrl Pts',(41.6500708922589,-8.38373900111893,1.13639406157512));
#35730=CARTESIAN_POINT('Ctrl Pts',(41.6318008476496,-8.33823037168233,0.669677370080662));
#35731=CARTESIAN_POINT('Ctrl Pts',(41.6187886661145,-8.30350078066026,0.326360253171814));
#35732=CARTESIAN_POINT('Ctrl Pts',(41.6394982516696,-8.14834662563339,-1.25364232212061));
#35733=CARTESIAN_POINT('Ctrl Pts',(41.9087301497588,-8.05962904511281,-2.51864171287989));
#35734=CARTESIAN_POINT('Ctrl Pts',(42.8944223117582,-7.94955134754687,-4.8479591580739));
#35735=CARTESIAN_POINT('Ctrl Pts',(43.621903091562,-7.92716706336173,-5.91517020467067));
#35736=CARTESIAN_POINT('Ctrl Pts',(45.4173857785914,-7.93333952030752,-7.69457540339218));
#35737=CARTESIAN_POINT('Ctrl Pts',(46.4936627982988,-7.96110451544899,-8.40795287034955));
#35738=CARTESIAN_POINT('Ctrl Pts',(48.8323759936291,-8.04556196575582,-9.37372383743957));
#35739=CARTESIAN_POINT('Ctrl Pts',(50.1083893187855,-8.1011483996294,-9.62254086008693));
#35740=CARTESIAN_POINT('Ctrl Pts',(51.3620268377998,-8.15637495641971,-9.62369151535362));
#35741=CARTESIAN_POINT('Ctrl Pts',(43.5199138025263,-9.87072183560237,1.24768171633309));
#35742=CARTESIAN_POINT('Ctrl Pts',(43.5156272263023,-9.86004464583426,1.13817917736476));
#35743=CARTESIAN_POINT('Ctrl Pts',(43.5113398926843,-9.84936631915757,1.02865855747361));
#35744=CARTESIAN_POINT('Ctrl Pts',(43.4930709070365,-9.80385794333019,0.561963612030324));
#35745=CARTESIAN_POINT('Ctrl Pts',(43.4827143498846,-9.76971145014119,0.254842414704953));
#35746=CARTESIAN_POINT('Ctrl Pts',(43.5023995944571,-9.61585927298276,-0.978922014677277));
#35747=CARTESIAN_POINT('Ctrl Pts',(43.7224911564668,-9.51762723326116,-1.98636136651214));
#35748=CARTESIAN_POINT('Ctrl Pts',(44.4993341101079,-9.38040562961654,-3.81078790536449));
#35749=CARTESIAN_POINT('Ctrl Pts',(45.0800827322703,-9.33502766340239,-4.65460264915721));
#35750=CARTESIAN_POINT('Ctrl Pts',(46.495867776811,-9.28745674945108,-6.05121512487505));
#35751=CARTESIAN_POINT('Ctrl Pts',(47.3523605835685,-9.28172473628545,-6.61423873299739));
#35752=CARTESIAN_POINT('Ctrl Pts',(49.1896776789186,-9.2969764356746,-7.37244739486635));
#35753=CARTESIAN_POINT('Ctrl Pts',(50.2104967200023,-9.31353425501145,-7.56862230181894));
#35754=CARTESIAN_POINT('Ctrl Pts',(51.1931844250963,-9.33084205690778,-7.5703742150597));
#35755=CARTESIAN_POINT('Ctrl Pts',(36.6062244663074,-9.64145132693369,1.5964706812661));
#35756=CARTESIAN_POINT('Ctrl Pts',(36.5951848118711,-9.59613798296326,1.15259163662005));
#35757=CARTESIAN_POINT('Ctrl Pts',(36.5727117312847,-9.54279427445071,0.635573001824062));
#35758=CARTESIAN_POINT('Ctrl Pts',(36.6214111051582,-9.38007537751166,-1.86858636169253));
#35759=CARTESIAN_POINT('Ctrl Pts',(37.005503628143,-9.36705556805879,-3.71029995870864));
#35760=CARTESIAN_POINT('Ctrl Pts',(38.4518973636206,-9.52533731123247,-7.16936247492662));
#35761=CARTESIAN_POINT('Ctrl Pts',(39.492347221447,-9.70422705237809,-8.73699595770811));
#35762=CARTESIAN_POINT('Ctrl Pts',(42.0930574706692,-10.2059604432482,-11.3730256982116));
#35763=CARTESIAN_POINT('Ctrl Pts',(43.6303739147809,-10.5307434056714,-12.4235805192465));
#35764=CARTESIAN_POINT('Ctrl Pts',(47.0225411281103,-11.260355741399,-13.8529470821356));
#35765=CARTESIAN_POINT('Ctrl Pts',(48.830372711006,-11.664686791883,-14.2204718556452));
#35766=CARTESIAN_POINT('Ctrl Pts',(50.6517393542017,-12.0680951184149,-14.2198708430666));
#35767=CARTESIAN_POINT('Ctrl Pts',(35.8014489642672,-10.1498171217999,1.62964612287371));
#35768=CARTESIAN_POINT('Ctrl Pts',(35.7905014108312,-10.1048818153799,1.18947024667652));
#35769=CARTESIAN_POINT('Ctrl Pts',(35.7670704718575,-10.0508712183064,0.664243958000225));
#35770=CARTESIAN_POINT('Ctrl Pts',(35.8153925117057,-9.88755379325372,-1.95287905117699));
#35771=CARTESIAN_POINT('Ctrl Pts',(36.215170789872,-9.87991493952696,-3.87337387079453));
#35772=CARTESIAN_POINT('Ctrl Pts',(37.7224873536725,-10.0551723243901,-7.4879213021314));
#35773=CARTESIAN_POINT('Ctrl Pts',(38.8072993194045,-10.2476883531955,-9.12360836232144));
#35774=CARTESIAN_POINT('Ctrl Pts',(41.520677603786,-10.7822353604969,-11.8774049927099));
#35775=CARTESIAN_POINT('Ctrl Pts',(43.1237524839592,-11.1269271238462,-12.9732563609012));
#35776=CARTESIAN_POINT('Ctrl Pts',(46.6646288366278,-11.8992915178566,-14.4676858045336));
#35777=CARTESIAN_POINT('Ctrl Pts',(48.5486094635743,-12.3267171394201,-14.8501851005103));
#35778=CARTESIAN_POINT('Ctrl Pts',(50.4504961875093,-12.7534443437025,-14.8499483202528));
#35779=CARTESIAN_POINT('Ctrl Pts',(35.5333334012201,-11.0637722809467,1.62975530581349));
#35780=CARTESIAN_POINT('Ctrl Pts',(35.5223873364831,-11.0188430850085,1.18963928646871));
#35781=CARTESIAN_POINT('Ctrl Pts',(35.4989008284158,-10.9648105349846,0.664246400070066));
#35782=CARTESIAN_POINT('Ctrl Pts',(35.5465440138856,-10.8012937803281,-1.95288623086898));
#35783=CARTESIAN_POINT('Ctrl Pts',(35.947363088238,-10.7939605764187,-3.87317034519632));
#35784=CARTESIAN_POINT('Ctrl Pts',(37.453518094782,-10.9688768024953,-7.48823335803387));
#35785=CARTESIAN_POINT('Ctrl Pts',(38.5390425757361,-11.1616021044182,-9.12349227713323));
#35786=CARTESIAN_POINT('Ctrl Pts',(41.2521634397981,-11.6960735042602,-11.8775764776363));
#35787=CARTESIAN_POINT('Ctrl Pts',(42.855659865817,-12.0408890833115,-12.9726927515384));
#35788=CARTESIAN_POINT('Ctrl Pts',(46.3960659393469,-12.8131153360318,-14.468343335498));
#35789=CARTESIAN_POINT('Ctrl Pts',(48.280363080515,-13.2406268960268,-14.8498038985481));
#35790=CARTESIAN_POINT('Ctrl Pts',(50.1821542472111,-13.6673330636266,-14.8500516281495));
#35791=CARTESIAN_POINT('Ctrl Pts',(35.9359355586898,-11.9263392248007,1.59674363861555));
#35792=CARTESIAN_POINT('Ctrl Pts',(35.9248996260065,-11.8810411570359,1.15301423610032));
#35793=CARTESIAN_POINT('Ctrl Pts',(35.9022876226764,-11.827642566146,0.63557910699865));
#35794=CARTESIAN_POINT('Ctrl Pts',(35.9492898606198,-11.6644253451977,-1.8686043109225));
#35795=CARTESIAN_POINT('Ctrl Pts',(36.335984374051,-11.6521696602917,-3.70979114471011));
#35796=CARTESIAN_POINT('Ctrl Pts',(37.7794742164015,-11.8095985064919,-7.1701426146858));
#35797=CARTESIAN_POINT('Ctrl Pts',(38.8217053622758,-11.9890114304293,-8.73670574474357));
#35798=CARTESIAN_POINT('Ctrl Pts',(41.4217720606995,-12.4905558026619,-11.3734544105218));
#35799=CARTESIAN_POINT('Ctrl Pts',(42.9601423694208,-12.81564830434,-12.4221714958419));
#35800=CARTESIAN_POINT('Ctrl Pts',(46.3511338849127,-13.5449152868315,-13.854590909544));
#35801=CARTESIAN_POINT('Ctrl Pts',(48.1597570333989,-13.9494605087848,-14.2195188100056));
#35802=CARTESIAN_POINT('Ctrl Pts',(49.9808845034561,-14.3528169182251,-14.2201291128085));
#35803=CARTESIAN_POINT('Ctrl Pts',(36.5850719698904,-9.50149509066561,0.));
#35804=CARTESIAN_POINT('Ctrl Pts',(36.6214111051582,-9.38007537751166,-1.86858636169253));
#35805=CARTESIAN_POINT('Ctrl Pts',(37.005503628143,-9.36705556805998,-3.71029995870864));
#35806=CARTESIAN_POINT('Ctrl Pts',(38.4518973636206,-9.52533731123127,-7.16936247492662));
#35807=CARTESIAN_POINT('Ctrl Pts',(39.492347221447,-9.70422705237809,-8.7369959577105));
#35808=CARTESIAN_POINT('Ctrl Pts',(40.9249807596937,-9.98061312161967,-10.1890856763493));
#35809=CARTESIAN_POINT('Ctrl Pts',(41.0597112354494,-10.0068973767103,-10.3203928635158));
#35810=CARTESIAN_POINT('Ctrl Pts',(41.1968114628114,-10.0339108357988,-10.4488603765985));
#35811=CARTESIAN_POINT('Ctrl Pts',(35.9142171164209,-11.7862169042736,-4.44089209850063E-16));
#35812=CARTESIAN_POINT('Ctrl Pts',(35.9492898606198,-11.6644253451977,-1.8686043109225));
#35813=CARTESIAN_POINT('Ctrl Pts',(36.335984374051,-11.6521696602917,-3.70979114471011));
#35814=CARTESIAN_POINT('Ctrl Pts',(37.7794742164015,-11.8095985064919,-7.1701426146858));
#35815=CARTESIAN_POINT('Ctrl Pts',(38.8217053622758,-11.9890114304293,-8.73670574474357));
#35816=CARTESIAN_POINT('Ctrl Pts',(40.2612951155294,-12.2667035909826,-10.196605355573));
#35817=CARTESIAN_POINT('Ctrl Pts',(40.4035980344059,-12.2944800077005,-10.3350231942297));
#35818=CARTESIAN_POINT('Ctrl Pts',(40.5485470057469,-12.3230698430749,-10.4702558451028));
#35819=CARTESIAN_POINT('Ctrl Pts',(43.6145083358835,-9.34279883641536,1.24689082988539));
#35820=CARTESIAN_POINT('Ctrl Pts',(43.6025047583517,-9.2935289757009,0.764254661689123));
#35821=CARTESIAN_POINT('Ctrl Pts',(43.5898343019063,-9.24710292813879,0.332948671149295));
#35822=CARTESIAN_POINT('Ctrl Pts',(43.6387527331667,-9.08959664355163,-0.978870002765541));
#35823=CARTESIAN_POINT('Ctrl Pts',(43.8630440977107,-9.02147253459711,-1.98783577089164));
#35824=CARTESIAN_POINT('Ctrl Pts',(44.6599232717754,-8.99867539146223,-3.80852727283284));
#35825=CARTESIAN_POINT('Ctrl Pts',(45.2360569807709,-9.03489241248372,-4.65544360723186));
#35826=CARTESIAN_POINT('Ctrl Pts',(46.6460662566965,-9.18984064609203,-6.04997283342104));
#35827=CARTESIAN_POINT('Ctrl Pts',(47.4916031396324,-9.30516165132963,-6.61832169902913));
#35828=CARTESIAN_POINT('Ctrl Pts',(49.3114553051098,-9.58273633533165,-7.3676840307869));
#35829=CARTESIAN_POINT('Ctrl Pts',(50.3172192201087,-9.74382459488535,-7.57138648674191));
#35830=CARTESIAN_POINT('Ctrl Pts',(51.2881489781557,-9.90091582292662,-7.56962581969414));
#35831=CARTESIAN_POINT('Ctrl Pts',(41.3128793157231,-9.90389776310366,1.35489321026542));
#35832=CARTESIAN_POINT('Ctrl Pts',(41.3011741506616,-9.85585276552939,0.884255518280862));
#35833=CARTESIAN_POINT('Ctrl Pts',(41.2854482448493,-9.80727935893269,0.426396949030956));
#35834=CARTESIAN_POINT('Ctrl Pts',(41.3339507669543,-9.64806121735613,-1.25360819503015));
#35835=CARTESIAN_POINT('Ctrl Pts',(41.6081209011006,-9.59710950760114,-2.51960912780404));
#35836=CARTESIAN_POINT('Ctrl Pts',(42.6049670390268,-9.63005248743076,-4.84647586781651));
#35837=CARTESIAN_POINT('Ctrl Pts',(43.3248419422611,-9.71043261799562,-5.91572199047331));
#35838=CARTESIAN_POINT('Ctrl Pts',(45.1023943639496,-9.97242546015736,-7.69376028691353));
#35839=CARTESIAN_POINT('Ctrl Pts',(46.1617613376869,-10.152489506502,-8.41063186557578));
#35840=CARTESIAN_POINT('Ctrl Pts',(48.4668856266305,-10.5695775166851,-9.37059840619009));
#35841=CARTESIAN_POINT('Ctrl Pts',(49.7204896475851,-10.8058013195656,-9.62435378619457));
#35842=CARTESIAN_POINT('Ctrl Pts',(50.9539676685887,-11.0389609452148,-9.62320046360532));
#35843=CARTESIAN_POINT('Ctrl Pts',(38.9464705831154,-10.0047404051441,1.47293192394285));
#35844=CARTESIAN_POINT('Ctrl Pts',(38.9350908951694,-9.95803136027261,1.0153809158493));
#35845=CARTESIAN_POINT('Ctrl Pts',(38.9160550470399,-9.90712214456902,0.528580717858753));
#35846=CARTESIAN_POINT('Ctrl Pts',(38.9644836024862,-9.74614391855282,-1.55402875454098));
#35847=CARTESIAN_POINT('Ctrl Pts',(39.2926120042887,-9.71379866053015,-3.10121432124465));
#35848=CARTESIAN_POINT('Ctrl Pts',(40.5087724506345,-9.80788452010349,-5.98129145449939));
#35849=CARTESIAN_POINT('Ctrl Pts',(41.3854277882457,-9.93643935036519,-7.29389406576689));
#35850=CARTESIAN_POINT('Ctrl Pts',(43.565030873626,-10.3155272531378,-9.49113593803963));
#35851=CARTESIAN_POINT('Ctrl Pts',(44.8579833049588,-10.5663179729255,-10.3708286017266));
#35852=CARTESIAN_POINT('Ctrl Pts',(47.6940136086793,-11.1360404748617,-11.5604045561153));
#35853=CARTESIAN_POINT('Ctrl Pts',(49.2184417854976,-11.4544007679218,-11.8694761540999));
#35854=CARTESIAN_POINT('Ctrl Pts',(50.7390783576437,-11.7707281089613,-11.8687142284811));
#35855=CARTESIAN_POINT('Ctrl Pts',(36.6062244663074,-9.64145132693368,1.5964706812661));
#35856=CARTESIAN_POINT('Ctrl Pts',(36.595184811871,-9.59613798296326,1.15259163662005));
#35857=CARTESIAN_POINT('Ctrl Pts',(36.5727117312847,-9.54279427445071,0.635573001824062));
#35858=CARTESIAN_POINT('Ctrl Pts',(36.6214111051582,-9.38007537751166,-1.86858636169253));
#35859=CARTESIAN_POINT('Ctrl Pts',(37.005503628143,-9.36705556805998,-3.71029995870864));
#35860=CARTESIAN_POINT('Ctrl Pts',(38.4518973636206,-9.52533731123127,-7.16936247492662));
#35861=CARTESIAN_POINT('Ctrl Pts',(39.492347221447,-9.70422705237809,-8.7369959577105));
#35862=CARTESIAN_POINT('Ctrl Pts',(42.0930574706692,-10.2059604432482,-11.3730256982092));
#35863=CARTESIAN_POINT('Ctrl Pts',(43.6303739147809,-10.5307434056702,-12.4235805192465));
#35864=CARTESIAN_POINT('Ctrl Pts',(47.0225411281103,-11.2603557414002,-13.8529470821356));
#35865=CARTESIAN_POINT('Ctrl Pts',(48.830372711005,-11.6646867918863,-14.2204718556452));
#35866=CARTESIAN_POINT('Ctrl Pts',(50.6517393542018,-12.0680951184149,-14.2198708430666));
#35867=CARTESIAN_POINT('Ctrl Pts',(35.9359355586898,-11.9263392248007,1.59674363861555));
#35868=CARTESIAN_POINT('Ctrl Pts',(35.9248996260064,-11.8810411570359,1.15301423610033));
#35869=CARTESIAN_POINT('Ctrl Pts',(35.9022876226764,-11.827642566146,0.63557910699865));
#35870=CARTESIAN_POINT('Ctrl Pts',(35.9492898606198,-11.6644253451977,-1.8686043109225));
#35871=CARTESIAN_POINT('Ctrl Pts',(36.335984374051,-11.6521696602917,-3.70979114471011));
#35872=CARTESIAN_POINT('Ctrl Pts',(37.7794742164015,-11.8095985064919,-7.1701426146858));
#35873=CARTESIAN_POINT('Ctrl Pts',(38.8217053622758,-11.9890114304293,-8.73670574474597));
#35874=CARTESIAN_POINT('Ctrl Pts',(41.4217720606995,-12.4905558026619,-11.3734544105194));
#35875=CARTESIAN_POINT('Ctrl Pts',(42.960142369416,-12.81564830434,-12.4221714958419));
#35876=CARTESIAN_POINT('Ctrl Pts',(46.3511338849175,-13.5449152868315,-13.854590909544));
#35877=CARTESIAN_POINT('Ctrl Pts',(48.1597570333954,-13.949460508784,-14.2195188100056));
#35878=CARTESIAN_POINT('Ctrl Pts',(49.9808845034561,-14.3528169182251,-14.2201291128085));
#35879=CARTESIAN_POINT('Ctrl Pts',(38.1015519292155,-12.8849080239691,1.47327599461691));
#35880=CARTESIAN_POINT('Ctrl Pts',(38.0901769326353,-12.8382182351976,1.01591361478005));
#35881=CARTESIAN_POINT('Ctrl Pts',(38.0709659683616,-12.7872398386631,0.528588413608809));
#35882=CARTESIAN_POINT('Ctrl Pts',(38.1172552346281,-12.6256334607469,-1.55405138006716));
#35883=CARTESIAN_POINT('Ctrl Pts',(38.4486635210265,-12.594251403927,-3.10057294640624));
#35884=CARTESIAN_POINT('Ctrl Pts',(39.6611635256788,-12.6872621620748,-5.98227484334677));
#35885=CARTESIAN_POINT('Ctrl Pts',(40.5400642286605,-12.8164764794555,-7.29352824388334));
#35886=CARTESIAN_POINT('Ctrl Pts',(42.7188560995337,-13.1953261187354,-9.49167634237456));
#35887=CARTESIAN_POINT('Ctrl Pts',(44.0131369578425,-13.4465070217538,-10.3690524867684));
#35888=CARTESIAN_POINT('Ctrl Pts',(46.8476852602796,-14.0157941958989,-11.5624766483463));
#35889=CARTESIAN_POINT('Ctrl Pts',(48.3731128199089,-14.3344204493097,-11.8682745705926));
#35890=CARTESIAN_POINT('Ctrl Pts',(49.8934463159786,-14.650686356357,-11.8690397849988));
#35891=CARTESIAN_POINT('Ctrl Pts',(40.0384499621468,-14.2481859850624,1.35541218776073));
#35892=CARTESIAN_POINT('Ctrl Pts',(40.0267518732903,-14.2001700323427,0.885059012381398));
#35893=CARTESIAN_POINT('Ctrl Pts',(40.0107618318057,-14.1514922771428,0.426408556881866));
#35894=CARTESIAN_POINT('Ctrl Pts',(40.0560375664345,-13.9913266653943,-1.25364232214352));
#35895=CARTESIAN_POINT('Ctrl Pts',(40.3351549001603,-13.9418277959606,-2.51864171287518));
#35896=CARTESIAN_POINT('Ctrl Pts',(41.3264798268773,-13.9731491512594,-4.84795915807886));
#35897=CARTESIAN_POINT('Ctrl Pts',(42.0497415171332,-14.0545240163318,-5.91517020463943));
#35898=CARTESIAN_POINT('Ctrl Pts',(43.8260703469873,-14.316157474802,-7.69457540342382));
#35899=CARTESIAN_POINT('Ctrl Pts',(44.887441047737,-14.4968100523122,-8.40795287033977));
#35900=CARTESIAN_POINT('Ctrl Pts',(47.1903299665195,-14.9132414377274,-9.37372383744997));
#35901=CARTESIAN_POINT('Ctrl Pts',(48.4454445415193,-15.1498577118716,-9.62254086007292));
#35902=CARTESIAN_POINT('Ctrl Pts',(49.678462279699,-15.3829333626946,-9.62369151535395));
#35903=CARTESIAN_POINT('Ctrl Pts',(41.6721936506076,-15.9637816213008,1.24768178593771));
#35904=CARTESIAN_POINT('Ctrl Pts',(41.6602008577063,-15.9145560268665,0.765479239878682));
#35905=CARTESIAN_POINT('Ctrl Pts',(41.6471278409845,-15.8679709451274,0.332966362282368));
#35906=CARTESIAN_POINT('Ctrl Pts',(41.6911284345756,-15.7090206532874,-0.978922014745105));
#35907=CARTESIAN_POINT('Ctrl Pts',(41.922959658712,-15.6431107691407,-1.98636136650983));
#35908=CARTESIAN_POINT('Ctrl Pts',(42.7114241414519,-15.6178421628933,-3.81078790536703));
#35909=CARTESIAN_POINT('Ctrl Pts',(43.2927195380239,-15.6555752251425,-4.65460264909979));
#35910=CARTESIAN_POINT('Ctrl Pts',(44.7008639790291,-15.8099757342161,-6.051215124933));
#35911=CARTESIAN_POINT('Ctrl Pts',(45.5494546745409,-15.9261936999035,-6.61423873298305));
#35912=CARTESIAN_POINT('Ctrl Pts',(47.3658999879423,-16.2027676443008,-7.37244739488157));
#35913=CARTESIAN_POINT('Ctrl Pts',(48.3739721396802,-16.3644346256642,-7.56862230182889));
#35914=CARTESIAN_POINT('Ctrl Pts',(49.3441943438428,-16.5214173008841,-7.5703742150602));
#35915=CARTESIAN_POINT('Ctrl Pts',(34.8615042977018,-14.7529241788872,1.596470776103));
#35916=CARTESIAN_POINT('Ctrl Pts',(34.8570257719499,-14.7065009496497,1.15259170141934));
#35917=CARTESIAN_POINT('Ctrl Pts',(34.8423730342718,-14.6505019462243,0.63557304487636));
#35918=CARTESIAN_POINT('Ctrl Pts',(34.9137340335215,-14.4963699338552,-1.86858636173319));
#35919=CARTESIAN_POINT('Ctrl Pts',(35.2957699604174,-14.5381447126848,-3.71029995872548));
#35920=CARTESIAN_POINT('Ctrl Pts',(36.704915652626,-14.9006586663418,-7.16936247490966));
#35921=CARTESIAN_POINT('Ctrl Pts',(37.7093165664698,-15.2257990211601,-8.73699595768435));
#35922=CARTESIAN_POINT('Ctrl Pts',(40.2121512288891,-16.0925451480995,-11.3730256982353));
#35923=CARTESIAN_POINT('Ctrl Pts',(41.6875985735119,-16.6328052292317,-12.4235805191845));
#35924=CARTESIAN_POINT('Ctrl Pts',(44.9414037540397,-17.8377468920231,-13.8529470821977));
#35925=CARTESIAN_POINT('Ctrl Pts',(46.6732919100491,-18.4952436947556,-14.2204718556833));
#35926=CARTESIAN_POINT('Ctrl Pts',(48.4187086763093,-19.1537534053196,-14.2198708430666));
#35927=CARTESIAN_POINT('Ctrl Pts',(33.9925722540018,-15.1415840475455,1.6296462177106));
#35928=CARTESIAN_POINT('Ctrl Pts',(33.9881310914301,-15.0955481153421,1.1894703117361));
#35929=CARTESIAN_POINT('Ctrl Pts',(33.9726251531405,-15.0387526938512,0.66424400299639));
#35930=CARTESIAN_POINT('Ctrl Pts',(34.0436978384923,-14.8839745452648,-1.95287905122465));
#35931=CARTESIAN_POINT('Ctrl Pts',(34.4404940723683,-14.9333078251896,-3.87337387080411));
#35932=CARTESIAN_POINT('Ctrl Pts',(35.907526600646,-15.3212948554071,-7.48792130212165));
#35933=CARTESIAN_POINT('Ctrl Pts',(36.9538988571648,-15.6662361881476,-9.12360836229528));
#35934=CARTESIAN_POINT('Ctrl Pts',(39.5635848921121,-16.5814962694294,-11.8774049927359));
#35935=CARTESIAN_POINT('Ctrl Pts',(41.1012880289339,-17.150820909756,-12.9732563608631));
#35936=CARTESIAN_POINT('Ctrl Pts',(44.496204451925,-18.4192429936996,-14.4676858045717));
#35937=CARTESIAN_POINT('Ctrl Pts',(46.3001798643446,-19.1104364369604,-14.8501851005199));
#35938=CARTESIAN_POINT('Ctrl Pts',(48.1219785107275,-19.8034868749643,-14.8499483202528));
#35939=CARTESIAN_POINT('Ctrl Pts',(33.5971163401329,-16.0080796379932,1.62975540065039));
#35940=CARTESIAN_POINT('Ctrl Pts',(33.5926757814804,-15.9620499659334,1.18963935153781));
#35941=CARTESIAN_POINT('Ctrl Pts',(33.5771179639697,-15.905224906648,0.664246445067017));
#35942=CARTESIAN_POINT('Ctrl Pts',(33.6475470722393,-15.7501528462821,-1.9528862309185));
#35943=CARTESIAN_POINT('Ctrl Pts',(34.0453300100182,-15.7999367857058,-3.8731703451939));
#35944=CARTESIAN_POINT('Ctrl Pts',(35.5112613559415,-16.1874208227894,-7.4882333580361));
#35945=CARTESIAN_POINT('Ctrl Pts',(36.5583090926487,-16.5326707000397,-9.12349227710467));
#35946=CARTESIAN_POINT('Ctrl Pts',(39.1677510875134,-17.44781930872,-11.8775764776647));
#35947=CARTESIAN_POINT('Ctrl Pts',(40.705853858616,-18.0173264966996,-12.9726927515386));
#35948=CARTESIAN_POINT('Ctrl Pts',(44.1003244488303,-19.2855449177437,-14.4683433354976));
#35949=CARTESIAN_POINT('Ctrl Pts',(45.9046009234659,-19.9768684693553,-14.8498038985148));
#35950=CARTESIAN_POINT('Ctrl Pts',(47.7263079790886,-20.6698844856028,-14.8500516281495));
#35951=CARTESIAN_POINT('Ctrl Pts',(33.8728645130295,-16.9191631550063,1.59674373345245));
#35952=CARTESIAN_POINT('Ctrl Pts',(33.8683874970823,-16.8727555761308,1.15301430092323));
#35953=CARTESIAN_POINT('Ctrl Pts',(33.8536050613457,-16.8166824782156,0.635579150052946));
#35954=CARTESIAN_POINT('Ctrl Pts',(33.9233571178867,-16.6618156864003,-1.86860431096782));
#35955=CARTESIAN_POINT('Ctrl Pts',(34.3078598045374,-16.7047171139728,-3.70979114470055));
#35956=CARTESIAN_POINT('Ctrl Pts',(35.7142525408696,-17.0659735847998,-7.17014261469517));
#35957=CARTESIAN_POINT('Ctrl Pts',(36.7203421551699,-17.3918853008964,-8.7367057447198));
#35958=CARTESIAN_POINT('Ctrl Pts',(39.2225667174021,-18.2583527463199,-11.3734544105454));
#35959=CARTESIAN_POINT('Ctrl Pts',(40.6990131477269,-18.7990691965894,-12.4221714958709));
#35960=CARTESIAN_POINT('Ctrl Pts',(43.9517037462933,-20.0035017021346,-13.8545909095149));
#35961=CARTESIAN_POINT('Ctrl Pts',(45.6843449310537,-20.6613231478665,-14.2195188099675));
#35962=CARTESIAN_POINT('Ctrl Pts',(47.4295323472119,-21.3197474319158,-14.2201291128084));
#35963=CARTESIAN_POINT('Ctrl Pts',(34.8604849513721,-14.6113821712787,0.));
#35964=CARTESIAN_POINT('Ctrl Pts',(34.9137340335215,-14.4963699338552,-1.86858636173319));
#35965=CARTESIAN_POINT('Ctrl Pts',(35.2957699604174,-14.5381447126848,-3.71029995872548));
#35966=CARTESIAN_POINT('Ctrl Pts',(36.704915652626,-14.9006586663418,-7.16936247490966));
#35967=CARTESIAN_POINT('Ctrl Pts',(37.7093165664698,-15.2257990211577,-8.73699595768434));
#35968=CARTESIAN_POINT('Ctrl Pts',(39.0880341222367,-15.7032568890521,-10.1890856763509));
#35969=CARTESIAN_POINT('Ctrl Pts',(39.2176525965017,-15.7484477541922,-10.3203928635178));
#35970=CARTESIAN_POINT('Ctrl Pts',(39.3495129251698,-15.7946976519001,-10.4488603766002));
#35971=CARTESIAN_POINT('Ctrl Pts',(33.871308617615,-16.7773762111447,8.88178419700125E-16));
#35972=CARTESIAN_POINT('Ctrl Pts',(33.9233571178867,-16.6618156864003,-1.86860431096782));
#35973=CARTESIAN_POINT('Ctrl Pts',(34.3078598045374,-16.7047171139728,-3.70979114470055));
#35974=CARTESIAN_POINT('Ctrl Pts',(35.7142525408696,-17.0659735847998,-7.17014261469517));
#35975=CARTESIAN_POINT('Ctrl Pts',(36.7203421551699,-17.3918853008964,-8.7367057447198));
#35976=CARTESIAN_POINT('Ctrl Pts',(38.1057592455497,-17.8716259385938,-10.1966053555733));
#35977=CARTESIAN_POINT('Ctrl Pts',(38.2426607296422,-17.919371448325,-10.3350231942302));
#35978=CARTESIAN_POINT('Ctrl Pts',(38.3820655716557,-17.9682986698104,-10.4702558451034));
#35979=CARTESIAN_POINT('Ctrl Pts',(41.8409566234846,-15.4546943255726,1.24689092472231));
#35980=CARTESIAN_POINT('Ctrl Pts',(41.8360870570327,-15.4042176704004,0.764254723794704));
#35981=CARTESIAN_POINT('Ctrl Pts',(41.8301526811214,-15.3564609751279,0.332948693687485));
#35982=CARTESIAN_POINT('Ctrl Pts',(41.9009886759631,-15.2075196935603,-0.978870002742722));
#35983=CARTESIAN_POINT('Ctrl Pts',(42.1326921492877,-15.1720089789358,-1.98783577092476));
#35984=CARTESIAN_POINT('Ctrl Pts',(42.924704614198,-15.2628516088035,-3.80852727279997));
#35985=CARTESIAN_POINT('Ctrl Pts',(43.4898198932461,-15.3806923683367,-4.65544360723683));
#35986=CARTESIAN_POINT('Ctrl Pts',(44.8634258749406,-15.7347286943442,-6.04997283341622));
#35987=CARTESIAN_POINT('Ctrl Pts',(45.6839445214076,-15.9692083429551,-6.61832169890477));
#35988=CARTESIAN_POINT('Ctrl Pts',(47.4457702195574,-16.5029496832246,-7.3676840309116));
#35989=CARTESIAN_POINT('Ctrl Pts',(48.4183716585838,-16.8055334255027,-7.57138648687994));
#35990=CARTESIAN_POINT('Ctrl Pts',(49.3570623388651,-17.0992034029534,-7.5696258196942));
#35991=CARTESIAN_POINT('Ctrl Pts',(39.4829021650676,-15.6825261124559,1.35489330510234));
#35992=CARTESIAN_POINT('Ctrl Pts',(39.4781536574544,-15.6333043216819,0.884255581223509));
#35993=CARTESIAN_POINT('Ctrl Pts',(39.4695005333267,-15.5829872885748,0.426396977904085));
#35994=CARTESIAN_POINT('Ctrl Pts',(39.5401684750088,-15.4322923841402,-1.25360819502788));
#35995=CARTESIAN_POINT('Ctrl Pts',(39.8187991367757,-15.420877767565,-2.51960912782495));
#35996=CARTESIAN_POINT('Ctrl Pts',(40.8008105435898,-15.595351432329,-4.84647586779572));
#35997=CARTESIAN_POINT('Ctrl Pts',(41.5019188729783,-15.7773622894765,-5.91572199046869));
#35998=CARTESIAN_POINT('Ctrl Pts',(43.2240929050328,-16.2896605076506,-7.69376028691819));
#35999=CARTESIAN_POINT('Ctrl Pts',(44.2470512648663,-16.618655401243,-8.41063186548494));
#36000=CARTESIAN_POINT('Ctrl Pts',(46.4693548995031,-17.3595514471479,-9.37059840628112));
#36001=CARTESIAN_POINT('Ctrl Pts',(47.6765808868325,-17.7717772858459,-9.62435378629451));
#36002=CARTESIAN_POINT('Ctrl Pts',(48.8643218056536,-18.1781059077972,-9.62320046360535));
#36003=CARTESIAN_POINT('Ctrl Pts',(37.126228656985,-15.4455672457341,1.47293201877976));
#36004=CARTESIAN_POINT('Ctrl Pts',(37.121612187704,-15.3977141299041,1.01538097970151));
#36005=CARTESIAN_POINT('Ctrl Pts',(37.1100152319929,-15.3446140089033,0.528580753658652));
#36006=CARTESIAN_POINT('Ctrl Pts',(37.1808604460319,-15.1921664085262,-1.55402875456015));
#36007=CARTESIAN_POINT('Ctrl Pts',(37.5102521839154,-15.2068479190487,-3.10121432125934));
#36008=CARTESIAN_POINT('Ctrl Pts',(38.7006440566771,-15.4730537974356,-5.9812914544847));
#36009=CARTESIAN_POINT('Ctrl Pts',(39.5500810470697,-15.725061187495,-7.29389406575031));
#36010=CARTESIAN_POINT('Ctrl Pts',(41.6535490821772,-16.4104803826146,-9.4911359380562));
#36011=CARTESIAN_POINT('Ctrl Pts',(42.8976498813582,-16.8427247306038,-10.3708286016645));
#36012=CARTESIAN_POINT('Ctrl Pts',(45.6237335200129,-17.8102574730359,-11.5604045561775));
#36013=CARTESIAN_POINT('Ctrl Pts',(47.0873378224419,-18.3423260668147,-11.8694761541617));
#36014=CARTESIAN_POINT('Ctrl Pts',(48.5474784324869,-18.8718427994042,-11.8687142284811));
#36015=CARTESIAN_POINT('Ctrl Pts',(34.8615042977018,-14.7529241788872,1.596470776103));
#36016=CARTESIAN_POINT('Ctrl Pts',(34.8570257719499,-14.7065009496497,1.15259170141934));
#36017=CARTESIAN_POINT('Ctrl Pts',(34.8423730342718,-14.6505019462243,0.63557304487636));
#36018=CARTESIAN_POINT('Ctrl Pts',(34.9137340335215,-14.4963699338552,-1.86858636173319));
#36019=CARTESIAN_POINT('Ctrl Pts',(35.2957699604174,-14.5381447126848,-3.71029995872548));
#36020=CARTESIAN_POINT('Ctrl Pts',(36.704915652626,-14.9006586663418,-7.16936247490966));
#36021=CARTESIAN_POINT('Ctrl Pts',(37.7093165664698,-15.2257990211577,-8.73699595768434));
#36022=CARTESIAN_POINT('Ctrl Pts',(40.2121512288891,-16.0925451481019,-11.3730256982353));
#36023=CARTESIAN_POINT('Ctrl Pts',(41.6875985735119,-16.6328052292293,-12.4235805191845));
#36024=CARTESIAN_POINT('Ctrl Pts',(44.9414037540397,-17.8377468920255,-13.8529470821977));
#36025=CARTESIAN_POINT('Ctrl Pts',(46.6732919100429,-18.4952436947699,-14.2204718556833));
#36026=CARTESIAN_POINT('Ctrl Pts',(48.4187086763093,-19.1537534053196,-14.2198708430666));
#36027=CARTESIAN_POINT('Ctrl Pts',(33.8728645130295,-16.9191631550063,1.59674373345245));
#36028=CARTESIAN_POINT('Ctrl Pts',(33.8683874970823,-16.8727555761308,1.15301430092323));
#36029=CARTESIAN_POINT('Ctrl Pts',(33.8536050613457,-16.8166824782156,0.635579150052946));
#36030=CARTESIAN_POINT('Ctrl Pts',(33.9233571178867,-16.6618156864003,-1.86860431096782));
#36031=CARTESIAN_POINT('Ctrl Pts',(34.3078598045374,-16.7047171139705,-3.70979114470055));
#36032=CARTESIAN_POINT('Ctrl Pts',(35.7142525408696,-17.0659735848022,-7.17014261469517));
#36033=CARTESIAN_POINT('Ctrl Pts',(36.7203421551699,-17.391885300894,-8.7367057447174));
#36034=CARTESIAN_POINT('Ctrl Pts',(39.2225667174021,-18.2583527463223,-11.3734544105478));
#36035=CARTESIAN_POINT('Ctrl Pts',(40.6990131477221,-18.7990691965894,-12.4221714958709));
#36036=CARTESIAN_POINT('Ctrl Pts',(43.9517037462981,-20.0035017021346,-13.8545909095149));
#36037=CARTESIAN_POINT('Ctrl Pts',(45.684344931045,-20.66132314788,-14.2195188099485));
#36038=CARTESIAN_POINT('Ctrl Pts',(47.4295323472119,-21.3197474319158,-14.2201291128084));
#36039=CARTESIAN_POINT('Ctrl Pts',(35.8800194678368,-18.1761744494744,1.47327608945384));
#36040=CARTESIAN_POINT('Ctrl Pts',(35.8754049017066,-18.1283410613852,1.01591367866102));
#36041=CARTESIAN_POINT('Ctrl Pts',(35.863644457821,-18.0751475421218,0.528588449411221));
#36042=CARTESIAN_POINT('Ctrl Pts',(35.9324615528156,-17.9217737308913,-1.5540513800922));
#36043=CARTESIAN_POINT('Ctrl Pts',(36.2649627130594,-17.9378754149084,-3.10057294639211));
#36044=CARTESIAN_POINT('Ctrl Pts',(37.4518844049313,-18.2024961996302,-5.98227484336081));
#36045=CARTESIAN_POINT('Ctrl Pts',(38.3034500513313,-18.4554759130049,-7.29352824386674));
#36046=CARTESIAN_POINT('Ctrl Pts',(40.4061490374134,-19.140543821974,-9.49167634239111));
#36047=CARTESIAN_POINT('Ctrl Pts',(41.6515092131697,-19.5733634365314,-10.3690524868117));
#36048=CARTESIAN_POINT('Ctrl Pts',(44.3761878888565,-20.5402543714441,-11.5624766483028));
#36049=CARTESIAN_POINT('Ctrl Pts',(45.840743551652,-21.0727284454479,-11.8682745705403));
#36050=CARTESIAN_POINT('Ctrl Pts',(47.3005929134931,-21.60214123715,-11.8690397849988));
#36051=CARTESIAN_POINT('Ctrl Pts',(37.6031879890149,-19.8012255369167,1.35541228259766));
#36052=CARTESIAN_POINT('Ctrl Pts',(37.5984423520111,-19.7520335023888,0.885059075368103));
#36053=CARTESIAN_POINT('Ctrl Pts',(37.5895426312094,-19.7015755924258,0.42640858575879));
#36054=CARTESIAN_POINT('Ctrl Pts',(37.6571514684129,-19.5494836419063,-1.25364232215011));
#36055=CARTESIAN_POINT('Ctrl Pts',(37.9404722137893,-19.5402111378009,-2.51864171285047));
#36056=CARTESIAN_POINT('Ctrl Pts',(38.917249388435,-19.7122939334798,-4.84795915810355));
#36057=CARTESIAN_POINT('Ctrl Pts',(39.6215684668002,-19.8957713902408,-5.91517020463238));
#36058=CARTESIAN_POINT('Ctrl Pts',(41.3425825071256,-20.4075397474874,-7.69457540343085));
#36059=CARTESIAN_POINT('Ctrl Pts',(42.3674404420954,-20.7374023418912,-8.40795287042136));
#36060=CARTESIAN_POINT('Ctrl Pts',(44.5876249070044,-21.4773303202308,-9.37372383736816));
#36061=CARTESIAN_POINT('Ctrl Pts',(45.7962902185093,-21.8901596096101,-9.62254085998721));
#36062=CARTESIAN_POINT('Ctrl Pts',(46.9835874904385,-22.2963396064216,-9.62369151535389));
#36063=CARTESIAN_POINT('Ctrl Pts',(38.9761478068775,-21.7318648520661,1.24768188077466));
#36064=CARTESIAN_POINT('Ctrl Pts',(38.9712826154239,-21.681433547381,0.765479302051883));
#36065=CARTESIAN_POINT('Ctrl Pts',(38.9649724098635,-21.6334621464569,0.332966384826352));
#36066=CARTESIAN_POINT('Ctrl Pts',(39.0311461269946,-21.4823916741919,-0.978922014735768));
#36067=CARTESIAN_POINT('Ctrl Pts',(39.269997598184,-21.450145680751,-1.98636136647091));
#36068=CARTESIAN_POINT('Ctrl Pts',(40.0540327468074,-21.5373444678863,-3.81078790540598));
#36069=CARTESIAN_POINT('Ctrl Pts',(40.6240414198136,-21.6574204222982,-4.65460264909513));
#36070=CARTESIAN_POINT('Ctrl Pts',(41.9958794973451,-22.0106492051883,-6.05121512493769));
#36071=CARTESIAN_POINT('Ctrl Pts',(42.8192932220523,-22.2464512872586,-6.61423873311251));
#36072=CARTESIAN_POINT('Ctrl Pts',(44.5778891652563,-22.7787172284945,-7.3724473947518));
#36073=CARTESIAN_POINT('Ctrl Pts',(45.5526929856258,-23.0822022983042,-7.56862230172406));
#36074=CARTESIAN_POINT('Ctrl Pts',(46.4906987626547,-23.3756641324473,-7.57037421506012));
#36075=CARTESIAN_POINT('Ctrl Pts',(31.1202396243796,-21.5675617135473,1.59674381934713));
#36076=CARTESIAN_POINT('Ctrl Pts',(31.1224126652406,-21.5209893482701,1.15301435964445));
#36077=CARTESIAN_POINT('Ctrl Pts',(31.1157607260978,-21.4633832297129,0.635579189033741));
#36078=CARTESIAN_POINT('Ctrl Pts',(31.2068426510981,-21.320019509083,-1.86860431096819));
#36079=CARTESIAN_POINT('Ctrl Pts',(31.5813261451123,-21.4172046995034,-3.70979114473245));
#36080=CARTESIAN_POINT('Ctrl Pts',(32.9219916749941,-21.9749346552614,-7.17014261466314));
#36081=CARTESIAN_POINT('Ctrl Pts',(33.8714586745532,-22.4407105406785,-8.73670574474145));
#36082=CARTESIAN_POINT('Ctrl Pts',(36.2249030242345,-23.6544622808189,-11.3734544105236));
#36083=CARTESIAN_POINT('Ctrl Pts',(37.6093693845368,-24.399795252403,-12.4221714958129));
#36084=CARTESIAN_POINT('Ctrl Pts',(40.6575436657172,-26.0548745077493,-13.8545909095728));
#36085=CARTESIAN_POINT('Ctrl Pts',(42.2789313088874,-26.9525808296639,-14.2195188100293));
#36086=CARTESIAN_POINT('Ctrl Pts',(43.9126516878551,-27.8526693689673,-14.2201291128084));
#36087=CARTESIAN_POINT('Ctrl Pts',(32.9280732767456,-23.097426378281,1.47327617534843));
#36088=CARTESIAN_POINT('Ctrl Pts',(32.9303130813041,-23.0494231409482,1.01591373652235));
#36089=CARTESIAN_POINT('Ctrl Pts',(32.9262425677183,-22.9950973654526,0.528588481831309));
#36090=CARTESIAN_POINT('Ctrl Pts',(33.0161865744695,-22.8530783700746,-1.55405138009592));
#36091=CARTESIAN_POINT('Ctrl Pts',(33.3430118437574,-22.91633601094,-3.1005729464167));
#36092=CARTESIAN_POINT('Ctrl Pts',(34.4801929200289,-23.3471799062887,-5.98227484333611));
#36093=CARTESIAN_POINT('Ctrl Pts',(35.2870880890083,-23.718775078158,-7.29352824389314));
#36094=CARTESIAN_POINT('Ctrl Pts',(37.2708893025803,-24.6961152497729,-9.49167634236457));
#36095=CARTESIAN_POINT('Ctrl Pts',(38.441976853954,-25.3017626168073,-10.3690524867346));
#36096=CARTESIAN_POINT('Ctrl Pts',(41.0013193023712,-26.6465742010416,-11.5624766483798));
#36097=CARTESIAN_POINT('Ctrl Pts',(42.3751889385695,-27.3820564590436,-11.8682745706496));
#36098=CARTESIAN_POINT('Ctrl Pts',(43.7448358429351,-28.1138388177857,-11.8690397849987));
#36099=CARTESIAN_POINT('Ctrl Pts',(34.4024335442869,-24.9511692381922,1.35541236849217));
#36100=CARTESIAN_POINT('Ctrl Pts',(34.4047369676381,-24.9018025300741,0.885059132411614));
#36101=CARTESIAN_POINT('Ctrl Pts',(34.4031087413041,-24.8505916427402,0.426408611912723));
#36102=CARTESIAN_POINT('Ctrl Pts',(34.49167436083,-24.7096695075246,-1.25364232215568));
#36103=CARTESIAN_POINT('Ctrl Pts',(34.7734309243662,-24.7408121301906,-2.51864171287734));
#36104=CARTESIAN_POINT('Ctrl Pts',(35.7157759805903,-25.0501532567769,-4.8479591580766));
#36105=CARTESIAN_POINT('Ctrl Pts',(36.3868145416534,-25.331998233306,-5.91517020466113));
#36106=CARTESIAN_POINT('Ctrl Pts',(38.0174789095799,-26.0834833614041,-7.69457540340194));
#36107=CARTESIAN_POINT('Ctrl Pts',(38.9849609267772,-26.5558409214644,-8.40795287029638));
#36108=CARTESIAN_POINT('Ctrl Pts',(41.0772443843597,-27.6042026929754,-9.37372383749305));
#36109=CARTESIAN_POINT('Ctrl Pts',(42.2148554922723,-28.1848409838253,-9.62254086017268));
#36110=CARTESIAN_POINT('Ctrl Pts',(43.3322623493507,-28.7558566730956,-9.62369151535378));
#36111=CARTESIAN_POINT('Ctrl Pts',(35.4866599889488,-27.0575499833002,1.2476819666691));
#36112=CARTESIAN_POINT('Ctrl Pts',(35.4890214412832,-27.0069396045641,0.7654793583525));
#36113=CARTESIAN_POINT('Ctrl Pts',(35.4896025055219,-26.9585584437039,0.33296640524947));
#36114=CARTESIAN_POINT('Ctrl Pts',(35.5766022409729,-26.8184431506615,-0.978922014741607));
#36115=CARTESIAN_POINT('Ctrl Pts',(35.8176116317321,-26.820517483472,-1.98636136650726));
#36116=CARTESIAN_POINT('Ctrl Pts',(36.5812567518767,-27.0184085480271,-3.81078790536956));
#36117=CARTESIAN_POINT('Ctrl Pts',(37.1283749683431,-27.2183829945029,-4.65460264913816));
#36118=CARTESIAN_POINT('Ctrl Pts',(38.4359800152256,-27.7632493318097,-6.05121512489442));
#36119=CARTESIAN_POINT('Ctrl Pts',(39.2174544404224,-28.1138352796404,-6.61423873291563));
#36120=CARTESIAN_POINT('Ctrl Pts',(40.8824010709675,-28.8909578185449,-7.37244739494853));
#36121=CARTESIAN_POINT('Ctrl Pts',(41.8040923654846,-29.3300828960655,-7.56862230196192));
#36122=CARTESIAN_POINT('Ctrl Pts',(42.6907866227632,-29.7540498521225,-7.57037421505996));
#36123=CARTESIAN_POINT('Ctrl Pts',(31.1388779521426,-21.4269965203145,7.38298311375729E-15));
#36124=CARTESIAN_POINT('Ctrl Pts',(31.2068426510981,-21.320019509083,-1.86860431096819));
#36125=CARTESIAN_POINT('Ctrl Pts',(31.5813261451123,-21.4172046995034,-3.70979114473245));
#36126=CARTESIAN_POINT('Ctrl Pts',(32.9219916749941,-21.9749346552614,-7.17014261466314));
#36127=CARTESIAN_POINT('Ctrl Pts',(33.8714586745532,-22.4407105406785,-8.73670574474145));
#36128=CARTESIAN_POINT('Ctrl Pts',(35.1745000052642,-23.1127335196113,-10.1966053555721));
#36129=CARTESIAN_POINT('Ctrl Pts',(35.3032131351466,-23.1794761614708,-10.3350231942276));
#36130=CARTESIAN_POINT('Ctrl Pts',(35.4342359672587,-23.2477447519414,-10.4702558450994));
#36131=CARTESIAN_POINT('Ctrl Pts',(39.2156436908074,-21.2519768052529,1.24689101061683));
#36132=CARTESIAN_POINT('Ctrl Pts',(39.218007266706,-21.2013209149703,0.764254780031375));
#36133=CARTESIAN_POINT('Ctrl Pts',(39.2189297793915,-21.1532057605279,0.332948714116346));
#36134=CARTESIAN_POINT('Ctrl Pts',(39.310241321719,-21.0158614973052,-0.978870002768584));
#36135=CARTESIAN_POINT('Ctrl Pts',(39.544640089421,-21.0136870730577,-1.98783577086775));
#36136=CARTESIAN_POINT('Ctrl Pts',(40.3156627552369,-21.2163201816855,-3.8085272728572));
#36137=CARTESIAN_POINT('Ctrl Pts',(40.8582554869254,-21.4133857818212,-4.65544360719877));
#36138=CARTESIAN_POINT('Ctrl Pts',(42.1674955178609,-21.9593030415928,-6.04997283345453));
#36139=CARTESIAN_POINT('Ctrl Pts',(42.9462925343071,-22.3081680037623,-6.61832169907729));
#36140=CARTESIAN_POINT('Ctrl Pts',(44.6142260746746,-23.0872105664939,-7.36768403073927));
#36141=CARTESIAN_POINT('Ctrl Pts',(45.5338656769265,-23.5251300590179,-7.57138648664217));
#36142=CARTESIAN_POINT('Ctrl Pts',(46.4212082443693,-23.9494005117266,-7.56962581969437));
#36143=CARTESIAN_POINT('Ctrl Pts',(36.8491669828394,-21.1419034541631,1.3548933909969));
#36144=CARTESIAN_POINT('Ctrl Pts',(36.8514717995482,-21.0925068841199,0.884255638225286));
#36145=CARTESIAN_POINT('Ctrl Pts',(36.8500676110209,-21.0414705341014,0.426397004061771));
#36146=CARTESIAN_POINT('Ctrl Pts',(36.9414623772721,-20.9023665809611,-1.25360819504659));
#36147=CARTESIAN_POINT('Ctrl Pts',(37.2188814500116,-20.9307214263664,-2.51960912779197));
#36148=CARTESIAN_POINT('Ctrl Pts',(38.1660672052557,-21.2431739952986,-4.8464758678288));
#36149=CARTESIAN_POINT('Ctrl Pts',(38.8341364170723,-21.5231103628947,-5.91572199044975));
#36150=CARTESIAN_POINT('Ctrl Pts',(40.4658735625806,-22.2752850427144,-7.69376028693729));
#36151=CARTESIAN_POINT('Ctrl Pts',(41.4315988261968,-22.7465133961258,-8.41063186560463));
#36152=CARTESIAN_POINT('Ctrl Pts',(43.5258421132307,-23.7961349710929,-9.37059840616155));
#36153=CARTESIAN_POINT('Ctrl Pts',(44.6621144270249,-24.3759711162289,-9.62435378612333));
#36154=CARTESIAN_POINT('Ctrl Pts',(45.7799392638232,-24.9471970554255,-9.62320046360547));
#36155=CARTESIAN_POINT('Ctrl Pts',(34.5502037758215,-20.5719668778725,1.47293210467438));
#36156=CARTESIAN_POINT('Ctrl Pts',(34.5524445041376,-20.5239438427437,1.01538103753427));
#36157=CARTESIAN_POINT('Ctrl Pts',(34.5485225226992,-20.4697337816493,0.528580786081231));
#36158=CARTESIAN_POINT('Ctrl Pts',(34.6403421915648,-20.3289202010265,-1.55402875457259));
#36159=CARTESIAN_POINT('Ctrl Pts',(34.964291799767,-20.3903296068349,-3.10121432124684));
#36160=CARTESIAN_POINT('Ctrl Pts',(36.1046821531125,-20.823236320083,-5.98129145449724));
#36161=CARTESIAN_POINT('Ctrl Pts',(36.9096087087966,-21.1935661261718,-7.29389406574334));
#36162=CARTESIAN_POINT('Ctrl Pts',(38.8941211503257,-22.1713634554262,-9.49113593806328));
#36163=CARTESIAN_POINT('Ctrl Pts',(40.0640440126768,-22.7762621832688,-10.3708286017458));
#36164=CARTESIAN_POINT('Ctrl Pts',(42.6246857849651,-24.1219089895058,-11.5604045560964));
#36165=CARTESIAN_POINT('Ctrl Pts',(43.9976714500081,-24.8568545017212,-11.8694761540667));
#36166=CARTESIAN_POINT('Ctrl Pts',(45.3675918458115,-25.5887811923518,-11.8687142284812));
#36167=CARTESIAN_POINT('Ctrl Pts',(32.4071044310923,-19.5640700378125,1.59647086199769));
#36168=CARTESIAN_POINT('Ctrl Pts',(32.4092782047888,-19.5174819665916,1.15259176011853));
#36169=CARTESIAN_POINT('Ctrl Pts',(32.402744098825,-19.4599676463163,0.635573083859125));
#36170=CARTESIAN_POINT('Ctrl Pts',(32.4953140197357,-19.3175602025281,-1.86858636174048));
#36171=CARTESIAN_POINT('Ctrl Pts',(32.8675162009725,-19.4132791553963,-3.71029995872507));
#36172=CARTESIAN_POINT('Ctrl Pts',(34.2107277071003,-19.9726455810671,-7.16936247491005));
#36173=CARTESIAN_POINT('Ctrl Pts',(35.1586329709169,-20.4374176294354,-8.73699595768695));
#36174=CARTESIAN_POINT('Ctrl Pts',(37.5126415503284,-21.6515320408183,-11.3730256982328));
#36175=CARTESIAN_POINT('Ctrl Pts',(38.8961839422332,-22.3962711036893,-12.4235805192561));
#36176=CARTESIAN_POINT('Ctrl Pts',(41.9453890000031,-24.0520129554246,-13.8529470821262));
#36177=CARTESIAN_POINT('Ctrl Pts',(43.5660774805969,-24.9492907715107,-14.220471855612));
#36178=CARTESIAN_POINT('Ctrl Pts',(45.2000127177927,-25.8494965077557,-14.2198708430667));
#36179=CARTESIAN_POINT('Ctrl Pts',(32.426238988581,-19.4238236466313,0.));
#36180=CARTESIAN_POINT('Ctrl Pts',(32.4953140197357,-19.3175602025281,-1.86858636174048));
#36181=CARTESIAN_POINT('Ctrl Pts',(32.8675162009725,-19.4132791553963,-3.71029995872507));
#36182=CARTESIAN_POINT('Ctrl Pts',(34.2107277071003,-19.9726455810671,-7.16936247491005));
#36183=CARTESIAN_POINT('Ctrl Pts',(35.1586329709169,-20.4374176294354,-8.73699595768695));
#36184=CARTESIAN_POINT('Ctrl Pts',(36.4553678306315,-21.1062276306783,-10.1890856763509));
#36185=CARTESIAN_POINT('Ctrl Pts',(36.5772356450557,-21.1694051501777,-10.3203928635186));
#36186=CARTESIAN_POINT('Ctrl Pts',(36.7011717789887,-21.233949971968,-10.4488603766022));
#36187=CARTESIAN_POINT('Ctrl Pts',(32.4071044310923,-19.5640700378125,1.59647086199769));
#36188=CARTESIAN_POINT('Ctrl Pts',(32.4092782047888,-19.5174819665916,1.15259176011853));
#36189=CARTESIAN_POINT('Ctrl Pts',(32.402744098825,-19.4599676463163,0.635573083859125));
#36190=CARTESIAN_POINT('Ctrl Pts',(32.4953140197357,-19.3175602025281,-1.86858636174048));
#36191=CARTESIAN_POINT('Ctrl Pts',(32.8675162009725,-19.4132791553963,-3.71029995872507));
#36192=CARTESIAN_POINT('Ctrl Pts',(34.2107277071003,-19.9726455810671,-7.16936247491005));
#36193=CARTESIAN_POINT('Ctrl Pts',(35.1586329709169,-20.4374176294354,-8.73699595768695));
#36194=CARTESIAN_POINT('Ctrl Pts',(37.5126415503284,-21.6515320408183,-11.3730256982328));
#36195=CARTESIAN_POINT('Ctrl Pts',(38.8961839422332,-22.3962711036893,-12.4235805192561));
#36196=CARTESIAN_POINT('Ctrl Pts',(41.9453890000031,-24.0520129554246,-13.8529470821262));
#36197=CARTESIAN_POINT('Ctrl Pts',(43.5660774805969,-24.9492907715107,-14.220471855612));
#36198=CARTESIAN_POINT('Ctrl Pts',(45.2000127177927,-25.8494965077557,-14.2198708430667));
#36199=CARTESIAN_POINT('Ctrl Pts',(31.4917047963492,-19.8251119861396,1.62964630360532));
#36200=CARTESIAN_POINT('Ctrl Pts',(31.4938604348119,-19.77891258719,1.18947037067314));
#36201=CARTESIAN_POINT('Ctrl Pts',(31.4865951546911,-19.7204885321049,0.664244043736472));
#36202=CARTESIAN_POINT('Ctrl Pts',(31.5789716511101,-19.5774004975086,-1.95287905122872));
#36203=CARTESIAN_POINT('Ctrl Pts',(31.9647082138114,-19.6827016274975,-3.87337387081569));
#36204=CARTESIAN_POINT('Ctrl Pts',(33.3615921547095,-20.2755200062714,-7.48792130210999));
#36205=CARTESIAN_POINT('Ctrl Pts',(34.3482235804883,-20.7658646319867,-9.12360836230025));
#36206=CARTESIAN_POINT('Ctrl Pts',(36.8010916839413,-22.0432057314202,-11.8774049927309));
#36207=CARTESIAN_POINT('Ctrl Pts',(38.2421198758116,-22.8255734412205,-12.9732563608963));
#36208=CARTESIAN_POINT('Ctrl Pts',(41.4219656611935,-24.5642317985072,-14.4676858045386));
#36209=CARTESIAN_POINT('Ctrl Pts',(43.1092121219652,-25.5051223581494,-14.8501851005009));
#36210=CARTESIAN_POINT('Ctrl Pts',(44.8138361237937,-26.4503875219921,-14.8499483202528));
#36211=CARTESIAN_POINT('Ctrl Pts',(30.9769588736641,-20.6265086564335,1.62975548654509));
#36212=CARTESIAN_POINT('Ctrl Pts',(30.9791142189907,-20.5803155398586,1.18963941048385));
#36213=CARTESIAN_POINT('Ctrl Pts',(30.9718018055999,-20.5218547654632,0.664246485806314));
#36214=CARTESIAN_POINT('Ctrl Pts',(31.063583103656,-20.3783842201315,-1.9528862309198));
#36215=CARTESIAN_POINT('Ctrl Pts',(31.4502321914759,-20.4842718451404,-3.87317034521865));
#36216=CARTESIAN_POINT('Ctrl Pts',(32.8460977418583,-21.0764356359492,-7.48823335801123));
#36217=CARTESIAN_POINT('Ctrl Pts',(33.8333538619476,-21.5671817964815,-9.12349227712397));
#36218=CARTESIAN_POINT('Ctrl Pts',(36.2859962734989,-22.8443778274229,-11.8775764776454));
#36219=CARTESIAN_POINT('Ctrl Pts',(37.7273940527312,-23.6269831007036,-12.972692751519));
#36220=CARTESIAN_POINT('Ctrl Pts',(40.906827527481,-25.3653764194394,-14.4683433355172));
#36221=CARTESIAN_POINT('Ctrl Pts',(42.5943534697789,-26.3064386087592,-14.8498038985433));
#36222=CARTESIAN_POINT('Ctrl Pts',(44.2988917118187,-27.2516566664768,-14.8500516281495));
#36223=CARTESIAN_POINT('Ctrl Pts',(31.1202396243796,-21.5675617135473,1.59674381934713));
#36224=CARTESIAN_POINT('Ctrl Pts',(31.1224126652406,-21.5209893482701,1.15301435964445));
#36225=CARTESIAN_POINT('Ctrl Pts',(31.1157607260978,-21.4633832297129,0.635579189033741));
#36226=CARTESIAN_POINT('Ctrl Pts',(31.2068426510981,-21.320019509083,-1.86860431096819));
#36227=CARTESIAN_POINT('Ctrl Pts',(31.5813261451123,-21.4172046995034,-3.70979114473125));
#36228=CARTESIAN_POINT('Ctrl Pts',(32.9219916749941,-21.9749346552614,-7.17014261466433));
#36229=CARTESIAN_POINT('Ctrl Pts',(33.8714586745532,-22.4407105406785,-8.73670574474144));
#36230=CARTESIAN_POINT('Ctrl Pts',(36.2249030242345,-23.6544622808189,-11.3734544105236));
#36231=CARTESIAN_POINT('Ctrl Pts',(37.609369384532,-24.399795252403,-12.4221714958081));
#36232=CARTESIAN_POINT('Ctrl Pts',(40.657543665722,-26.0548745077493,-13.8545909095776));
#36233=CARTESIAN_POINT('Ctrl Pts',(42.2789313088846,-26.9525808296624,-14.219518810034));
#36234=CARTESIAN_POINT('Ctrl Pts',(43.9126516878551,-27.8526693689673,-14.2201291128084));
#36235=CARTESIAN_POINT('Ctrl Pts',(29.2929893708795,-23.976947844554,1.59647090706345));
#36236=CARTESIAN_POINT('Ctrl Pts',(29.3017711927835,-23.9311433314999,1.15259179091382));
#36237=CARTESIAN_POINT('Ctrl Pts',(29.3034887354727,-23.8732845217247,0.635573104312268));
#36238=CARTESIAN_POINT('Ctrl Pts',(29.4153831213971,-23.7455006526079,-1.86858636174501));
#36239=CARTESIAN_POINT('Ctrl Pts',(29.7701745937406,-23.8932152178192,-3.71029995871689));
#36240=CARTESIAN_POINT('Ctrl Pts',(31.0201080010755,-24.6380470280742,-7.16936247491829));
#36241=CARTESIAN_POINT('Ctrl Pts',(31.8922209971975,-25.2329893514644,-8.73699595769411));
#36242=CARTESIAN_POINT('Ctrl Pts',(34.0494826673323,-26.7697561790045,-11.3730256982256));
#36243=CARTESIAN_POINT('Ctrl Pts',(35.3129551735408,-27.7038134835938,-12.4235805191652));
#36244=CARTESIAN_POINT('Ctrl Pts',(38.0954870861221,-29.7766493957256,-13.852947082217));
#36245=CARTESIAN_POINT('Ctrl Pts',(39.5719833476435,-30.8954422364371,-14.2204718557213));
#36246=CARTESIAN_POINT('Ctrl Pts',(41.0611748464151,-32.0190184050858,-14.2198708430666));
#36247=CARTESIAN_POINT('Ctrl Pts',(28.3497570418621,-24.1050578112646,1.629646348671));
#36248=CARTESIAN_POINT('Ctrl Pts',(28.3584655992913,-24.0596354334659,1.18947040159126));
#36249=CARTESIAN_POINT('Ctrl Pts',(28.359588878887,-24.000772091729,0.664244065112554));
#36250=CARTESIAN_POINT('Ctrl Pts',(28.4713886672656,-23.872287032033,-1.9528790512343));
#36251=CARTESIAN_POINT('Ctrl Pts',(28.8382130746032,-24.031412384946,-3.87337387079909));
#36252=CARTESIAN_POINT('Ctrl Pts',(30.1365118994152,-24.8169940395271,-7.48792130212669));
#36253=CARTESIAN_POINT('Ctrl Pts',(31.0433175237996,-25.4427599557794,-9.12360836231701));
#36254=CARTESIAN_POINT('Ctrl Pts',(33.2894343746814,-27.0561790920224,-11.8774049927142));
#36255=CARTESIAN_POINT('Ctrl Pts',(34.604452443506,-28.0356631204391,-12.9732563608534));
#36256=CARTESIAN_POINT('Ctrl Pts',(37.5044951003644,-30.2091636817924,-14.4676858045814));
#36257=CARTESIAN_POINT('Ctrl Pts',(39.0406651372098,-31.3805975393655,-14.8501851005436));
#36258=CARTESIAN_POINT('Ctrl Pts',(40.5934132658115,-32.5588345556908,-14.8499483202528));
#36259=CARTESIAN_POINT('Ctrl Pts',(27.726199852942,-24.8250414362348,1.62975553161074));
#36260=CARTESIAN_POINT('Ctrl Pts',(27.7349072261468,-24.7796252351492,1.18963944140568));
#36261=CARTESIAN_POINT('Ctrl Pts',(27.7359890779304,-24.7207188400934,0.664246507182928));
#36262=CARTESIAN_POINT('Ctrl Pts',(27.8472541631358,-24.5917704574944,-1.9528862309267));
#36263=CARTESIAN_POINT('Ctrl Pts',(28.214898340463,-24.7516062016254,-3.87317034519845));
#36264=CARTESIAN_POINT('Ctrl Pts',(29.5122822981076,-25.5363949989265,-7.48823335803153));
#36265=CARTESIAN_POINT('Ctrl Pts',(30.4196491139356,-26.1626472662222,-9.12349227713836));
#36266=CARTESIAN_POINT('Ctrl Pts',(32.6655632155459,-27.7758906912455,-11.877576477631));
#36267=CARTESIAN_POINT('Ctrl Pts',(33.9809133010314,-28.7556624628396,-12.9726927515433));
#36268=CARTESIAN_POINT('Ctrl Pts',(36.8805855629435,-30.9288420054706,-14.4683433354929));
#36269=CARTESIAN_POINT('Ctrl Pts',(38.4170078110994,-32.1004855201288,-14.8498038985624));
#36270=CARTESIAN_POINT('Ctrl Pts',(39.9696777567511,-33.2786637049093,-14.8500516281495));
#36271=CARTESIAN_POINT('Ctrl Pts',(27.7340963985793,-25.7769069069793,1.59674386441279));
#36272=CARTESIAN_POINT('Ctrl Pts',(27.7428752599197,-25.7311178357269,1.1530143904477));
#36273=CARTESIAN_POINT('Ctrl Pts',(27.7444892330823,-25.6731513926385,0.635579209488198));
#36274=CARTESIAN_POINT('Ctrl Pts',(27.8550468610688,-25.544209216253,-1.86860431097603));
#36275=CARTESIAN_POINT('Ctrl Pts',(28.2118877583879,-25.6936997595176,-3.7097911447111));
#36276=CARTESIAN_POINT('Ctrl Pts',(29.4595339978087,-26.4365494265728,-7.17014261468459));
#36277=CARTESIAN_POINT('Ctrl Pts',(30.3330499725326,-27.0327076275655,-8.73670574475586));
#36278=CARTESIAN_POINT('Ctrl Pts',(32.4898047694984,-28.5690351770683,-11.3734544105093));
#36279=CARTESIAN_POINT('Ctrl Pts',(33.7541073173495,-29.5038118395949,-12.4221714958996));
#36280=CARTESIAN_POINT('Ctrl Pts',(36.5357132425746,-31.5758452049212,-13.8545909094863));
#36281=CARTESIAN_POINT('Ctrl Pts',(38.0128405673564,-32.6951616910142,-14.2195188100056));
#36282=CARTESIAN_POINT('Ctrl Pts',(39.5018360737642,-33.8185912781322,-14.2201291128084));
#36283=CARTESIAN_POINT('Ctrl Pts',(29.3318883095338,-23.8408520862203,0.));
#36284=CARTESIAN_POINT('Ctrl Pts',(29.4153831213971,-23.7455006526079,-1.86858636174501));
#36285=CARTESIAN_POINT('Ctrl Pts',(29.7701745937406,-23.8932152178192,-3.71029995871809));
#36286=CARTESIAN_POINT('Ctrl Pts',(31.0201080010755,-24.6380470280742,-7.1693624749171));
#36287=CARTESIAN_POINT('Ctrl Pts',(31.8922209971975,-25.2329893514668,-8.73699595769651));
#36288=CARTESIAN_POINT('Ctrl Pts',(33.0805753785957,-26.0795364430743,-10.1890856763513));
#36289=CARTESIAN_POINT('Ctrl Pts',(33.19221165592,-26.1594145048181,-10.3203928635187));
#36290=CARTESIAN_POINT('Ctrl Pts',(33.3057006128401,-26.240940304242,-10.4488603766015));
#36291=CARTESIAN_POINT('Ctrl Pts',(27.7725495286734,-25.6404249706862,-1.49880108324396E-15));
#36292=CARTESIAN_POINT('Ctrl Pts',(27.8550468610688,-25.544209216253,-1.86860431097603));
#36293=CARTESIAN_POINT('Ctrl Pts',(28.2118877583879,-25.6936997595176,-3.7097911447111));
#36294=CARTESIAN_POINT('Ctrl Pts',(29.4595339978087,-26.4365494265728,-7.17014261468459));
#36295=CARTESIAN_POINT('Ctrl Pts',(30.3330499725326,-27.0327076275655,-8.73670574475586));
#36296=CARTESIAN_POINT('Ctrl Pts',(31.5271893797544,-27.8833324977838,-10.1966053555717));
#36297=CARTESIAN_POINT('Ctrl Pts',(31.6450939272834,-27.9677135840438,-10.3350231942281));
#36298=CARTESIAN_POINT('Ctrl Pts',(31.7650675024754,-28.0539337918559,-10.4702558451017));
#36299=CARTESIAN_POINT('Ctrl Pts',(35.7920133394051,-26.616630318486,1.246891055683));
#36300=CARTESIAN_POINT('Ctrl Pts',(35.8015619426228,-26.566826402425,0.764254809544874));
#36301=CARTESIAN_POINT('Ctrl Pts',(35.8093225655931,-26.519332276069,0.332948724830327));
#36302=CARTESIAN_POINT('Ctrl Pts',(35.9192508155954,-26.3963809659062,-0.978870002769423));
#36303=CARTESIAN_POINT('Ctrl Pts',(36.151573194659,-26.4275870967948,-1.9878357709031));
#36304=CARTESIAN_POINT('Ctrl Pts',(36.8859102633496,-26.7378856585306,-3.8085272728217));
#36305=CARTESIAN_POINT('Ctrl Pts',(37.3949348243792,-27.010164411862,-4.65544360718431));
#36306=CARTESIAN_POINT('Ctrl Pts',(38.6131565530439,-27.7368493043474,-6.04997283346876));
#36307=CARTESIAN_POINT('Ctrl Pts',(39.3343778780771,-28.1929976959362,-6.61832169883747));
#36308=CARTESIAN_POINT('Ctrl Pts',(40.8744649437267,-29.2014824201682,-7.36768403097867));
#36309=CARTESIAN_POINT('Ctrl Pts',(41.7224214992404,-29.7658228850822,-7.57138648693213));
#36310=CARTESIAN_POINT('Ctrl Pts',(42.540352217728,-30.3120568904492,-7.56962581969415));
#36311=CARTESIAN_POINT('Ctrl Pts',(33.4652890233051,-26.1708926054257,1.35489343606293));
#36312=CARTESIAN_POINT('Ctrl Pts',(33.4746002454547,-26.1223268292875,0.884255668135784));
#36313=CARTESIAN_POINT('Ctrl Pts',(33.4804735791513,-26.0716101167854,0.426397017783367));
#36314=CARTESIAN_POINT('Ctrl Pts',(33.5907346359808,-25.9469288717332,-1.25360819504925));
#36315=CARTESIAN_POINT('Ctrl Pts',(33.8612946673231,-26.0144759561311,-2.51960912781043));
#36316=CARTESIAN_POINT('Ctrl Pts',(34.7543728004649,-26.4585467959913,-4.84647586781028));
#36317=CARTESIAN_POINT('Ctrl Pts',(35.3758029321052,-26.8307099768394,-5.91572199044252));
#36318=CARTESIAN_POINT('Ctrl Pts',(36.8838857283485,-27.8074490109362,-7.6937602869444));
#36319=CARTESIAN_POINT('Ctrl Pts',(37.7727185143506,-28.4113179739906,-8.41063186543685));
#36320=CARTESIAN_POINT('Ctrl Pts',(39.6962686996365,-29.7482978092141,-9.37059840632905));
#36321=CARTESIAN_POINT('Ctrl Pts',(40.7384561125427,-30.48394046912,-9.62435378631342));
#36322=CARTESIAN_POINT('Ctrl Pts',(41.7636091770243,-31.2084352127809,-9.62320046360533));
#36323=CARTESIAN_POINT('Ctrl Pts',(31.2708363785842,-25.2795805846981,1.47293214974027));
#36324=CARTESIAN_POINT('Ctrl Pts',(31.2798886902773,-25.2323652421901,1.01538106787782));
#36325=CARTESIAN_POINT('Ctrl Pts',(31.2837215247233,-25.1781488031013,0.528580803091344));
#36326=CARTESIAN_POINT('Ctrl Pts',(31.3946464646597,-25.0518358019871,-1.5540287545765));
#36327=CARTESIAN_POINT('Ctrl Pts',(31.7065592632635,-25.1587229846903,-3.10121432124958));
#36328=CARTESIAN_POINT('Ctrl Pts',(32.7737330382195,-25.7495178004988,-5.98129145449449));
#36329=CARTESIAN_POINT('Ctrl Pts',(33.5177631757263,-26.2306311757317,-7.2938940657433));
#36330=CARTESIAN_POINT('Ctrl Pts',(35.3429210732455,-27.4809015052035,-9.49113593806323));
#36331=CARTESIAN_POINT('Ctrl Pts',(36.4148497432471,-28.2461406190897,-10.3708286016404));
#36332=CARTESIAN_POINT('Ctrl Pts',(38.7579223665916,-29.9425080008996,-11.5604045562015));
#36333=CARTESIAN_POINT('Ctrl Pts',(40.0123393656451,-30.8653690604273,-11.8694761542045));
#36334=CARTESIAN_POINT('Ctrl Pts',(41.2641519184868,-31.7848057921744,-11.8687142284811));
#36335=CARTESIAN_POINT('Ctrl Pts',(29.2929893708795,-23.976947844554,1.59647090706345));
#36336=CARTESIAN_POINT('Ctrl Pts',(29.3017711927835,-23.9311433314999,1.15259179091383));
#36337=CARTESIAN_POINT('Ctrl Pts',(29.3034887354727,-23.8732845217247,0.635573104312268));
#36338=CARTESIAN_POINT('Ctrl Pts',(29.4153831213971,-23.7455006526079,-1.86858636174501));
#36339=CARTESIAN_POINT('Ctrl Pts',(29.7701745937406,-23.8932152178192,-3.71029995871809));
#36340=CARTESIAN_POINT('Ctrl Pts',(31.0201080010755,-24.6380470280742,-7.1693624749171));
#36341=CARTESIAN_POINT('Ctrl Pts',(31.8922209971975,-25.2329893514668,-8.73699595769651));
#36342=CARTESIAN_POINT('Ctrl Pts',(34.0494826673323,-26.7697561790021,-11.3730256982232));
#36343=CARTESIAN_POINT('Ctrl Pts',(35.3129551735408,-27.7038134835914,-12.4235805191652));
#36344=CARTESIAN_POINT('Ctrl Pts',(38.0954870861221,-29.776649395728,-13.852947082217));
#36345=CARTESIAN_POINT('Ctrl Pts',(39.5719833476427,-30.8954422364365,-14.2204718557261));
#36346=CARTESIAN_POINT('Ctrl Pts',(41.0611748464151,-32.0190184050858,-14.2198708430666));
#36347=CARTESIAN_POINT('Ctrl Pts',(27.7340963985793,-25.7769069069793,1.59674386441279));
#36348=CARTESIAN_POINT('Ctrl Pts',(27.7428752599197,-25.7311178357269,1.1530143904477));
#36349=CARTESIAN_POINT('Ctrl Pts',(27.7444892330823,-25.6731513926385,0.635579209488198));
#36350=CARTESIAN_POINT('Ctrl Pts',(27.8550468610688,-25.544209216253,-1.86860431097603));
#36351=CARTESIAN_POINT('Ctrl Pts',(28.2118877583879,-25.6936997595176,-3.7097911447087));
#36352=CARTESIAN_POINT('Ctrl Pts',(29.4595339978087,-26.4365494265727,-7.17014261468699));
#36353=CARTESIAN_POINT('Ctrl Pts',(30.3330499725326,-27.0327076275679,-8.73670574475587));
#36354=CARTESIAN_POINT('Ctrl Pts',(32.4898047694983,-28.5690351770659,-11.3734544105093));
#36355=CARTESIAN_POINT('Ctrl Pts',(33.7541073173447,-29.5038118395925,-12.4221714958948));
#36356=CARTESIAN_POINT('Ctrl Pts',(36.5357132425794,-31.5758452049236,-13.8545909094911));
#36357=CARTESIAN_POINT('Ctrl Pts',(38.0128405673532,-32.6951616910118,-14.2195188099676));
#36358=CARTESIAN_POINT('Ctrl Pts',(39.5018360737642,-33.8185912781322,-14.2201291128085));
#36359=CARTESIAN_POINT('Ctrl Pts',(29.3058064687036,-27.5484813091702,1.47327622041421));
#36360=CARTESIAN_POINT('Ctrl Pts',(29.3148550485227,-27.5012854314998,1.01591376687586));
#36361=CARTESIAN_POINT('Ctrl Pts',(29.318557330567,-27.4469333174927,0.52858849884309));
#36362=CARTESIAN_POINT('Ctrl Pts',(29.4277972482622,-27.3191602363946,-1.554051380104));
#36363=CARTESIAN_POINT('Ctrl Pts',(29.7422934066315,-27.428286091063,-3.10057294640268));
#36364=CARTESIAN_POINT('Ctrl Pts',(30.8065841399312,-28.016582357744,-5.98227484335018));
#36365=CARTESIAN_POINT('Ctrl Pts',(31.5523827727636,-28.4992283820367,-7.2935282438956));
#36366=CARTESIAN_POINT('Ctrl Pts',(33.3769017419044,-29.7489449887834,-9.49167634236224));
#36367=CARTESIAN_POINT('Ctrl Pts',(34.4498767035324,-30.5150908742602,-10.3690524868452));
#36368=CARTESIAN_POINT('Ctrl Pts',(36.7917820928971,-32.2104466224834,-11.5624766482694));
#36369=CARTESIAN_POINT('Ctrl Pts',(38.0469976785191,-33.1339647666031,-11.8682745705784));
#36370=CARTESIAN_POINT('Ctrl Pts',(39.2985600643044,-34.0532197137074,-11.8690397849988));
#36371=CARTESIAN_POINT('Ctrl Pts',(30.5013447592647,-29.5931790826757,1.35541241355805));
#36372=CARTESIAN_POINT('Ctrl Pts',(30.5106503524626,-29.5446426662435,0.885059162337716));
#36373=CARTESIAN_POINT('Ctrl Pts',(30.5163267680096,-29.4937213090679,0.426408625636832));
#36374=CARTESIAN_POINT('Ctrl Pts',(30.6240462289239,-29.3668377587659,-1.25364232216464));
#36375=CARTESIAN_POINT('Ctrl Pts',(30.8985028596502,-29.4377615342222,-2.51864171286706));
#36376=CARTESIAN_POINT('Ctrl Pts',(31.78723236954,-29.8780636984406,-4.84795915808689));
#36377=CARTESIAN_POINT('Ctrl Pts',(32.4113300033664,-30.2525386437955,-5.91517020465884));
#36378=CARTESIAN_POINT('Ctrl Pts',(33.9184490747708,-31.2284424726334,-7.69457540340442));
#36379=CARTESIAN_POINT('Ctrl Pts',(34.8088600301736,-31.8336791606447,-8.40795287046934));
#36380=CARTESIAN_POINT('Ctrl Pts',(36.7306496231999,-33.1691331027914,-9.37372383732036));
#36381=CARTESIAN_POINT('Ctrl Pts',(37.7740480457988,-33.905760273803,-9.62254086002536));
#36382=CARTESIAN_POINT('Ctrl Pts',(38.7988173067558,-34.6299874229484,-9.62369151535393));
#36383=CARTESIAN_POINT('Ctrl Pts',(31.2747661069635,-31.8324214200723,1.24768201173505));
#36384=CARTESIAN_POINT('Ctrl Pts',(31.2843061312878,-31.7826622501441,0.765479387889553));
#36385=CARTESIAN_POINT('Ctrl Pts',(31.2917666379653,-31.7348562317647,0.332966415967282));
#36386=CARTESIAN_POINT('Ctrl Pts',(31.3978213275647,-31.6085484626322,-0.978922014752047));
#36387=CARTESIAN_POINT('Ctrl Pts',(31.6360823820021,-31.6449008941856,-1.98636136649952));
#36388=CARTESIAN_POINT('Ctrl Pts',(32.3637918610291,-31.9494557448159,-3.81078790537729));
#36389=CARTESIAN_POINT('Ctrl Pts',(32.8768818719313,-32.2252577802596,-4.65460264913351));
#36390=CARTESIAN_POINT('Ctrl Pts',(34.0936348201865,-32.9506697646502,-6.05121512489931));
#36391=CARTESIAN_POINT('Ctrl Pts',(34.817261379824,-33.4089026595985,-6.61423873317492));
#36392=CARTESIAN_POINT('Ctrl Pts',(36.3546651863436,-34.4150618217887,-7.37244739468963));
#36393=CARTESIAN_POINT('Ctrl Pts',(37.2044809778681,-34.9808875866076,-7.56862230174318));
#36394=CARTESIAN_POINT('Ctrl Pts',(38.0218131772945,-35.526728920403,-7.57037421506017));
#36395=CARTESIAN_POINT('Ctrl Pts',(25.5825535213021,-27.9017241322582,1.59647090706388));
#36396=CARTESIAN_POINT('Ctrl Pts',(25.5977646187892,-27.8576356266642,1.15259179092905));
#36397=CARTESIAN_POINT('Ctrl Pts',(25.6076988465248,-27.8006101679573,0.635573104293147));
#36398=CARTESIAN_POINT('Ctrl Pts',(25.7366398496106,-27.6900511858228,-1.86858636168828));
#36399=CARTESIAN_POINT('Ctrl Pts',(26.0667980819016,-27.8867543207229,-3.71029995869047));
#36400=CARTESIAN_POINT('Ctrl Pts',(27.1980083507262,-28.8018888878774,-7.16936247494455));
#36401=CARTESIAN_POINT('Ctrl Pts',(27.9765753735429,-29.5148901762063,-8.73699595768931));
#36402=CARTESIAN_POINT('Ctrl Pts',(29.8931745078317,-31.3430252790121,-11.3730256982303));
#36403=CARTESIAN_POINT('Ctrl Pts',(31.0108564713313,-32.4473861125001,-12.4235805192179));
#36404=CARTESIAN_POINT('Ctrl Pts',(33.4700709138175,-34.895119122769,-13.8529470821642));
#36405=CARTESIAN_POINT('Ctrl Pts',(34.7723177498495,-36.2126515923945,-14.2204718557167));
#36406=CARTESIAN_POINT('Ctrl Pts',(36.0864498658144,-37.5367254229129,-14.2198708430666));
#36407=CARTESIAN_POINT('Ctrl Pts',(24.6306899881717,-27.8942941678688,1.62964634867148));
#36408=CARTESIAN_POINT('Ctrl Pts',(24.6457741833895,-27.8505734813151,1.18947040160635));
#36409=CARTESIAN_POINT('Ctrl Pts',(24.655263156581,-27.7924691428841,0.664244065094566));
#36410=CARTESIAN_POINT('Ctrl Pts',(24.784210314811,-27.6812026446474,-1.95287905118087));
#36411=CARTESIAN_POINT('Ctrl Pts',(25.124655079764,-27.8909128870729,-3.87337387077627));
#36412=CARTESIAN_POINT('Ctrl Pts',(26.297939168344,-28.8532656404736,-7.48792130214935));
#36413=CARTESIAN_POINT('Ctrl Pts',(27.1064590438596,-29.6017140576996,-9.12360836230742));
#36414=CARTESIAN_POINT('Ctrl Pts',(29.1001001803562,-31.5183666699225,-11.8774049927237));
#36415=CARTESIAN_POINT('Ctrl Pts',(30.2623381501061,-32.6750275471261,-12.9732563608774));
#36416=CARTESIAN_POINT('Ctrl Pts',(32.8235411736691,-35.2391241081266,-14.4676858045574));
#36417=CARTESIAN_POINT('Ctrl Pts',(34.1773627942034,-36.6172542487315,-14.8501851005199));
#36418=CARTESIAN_POINT('Ctrl Pts',(35.5466255754742,-38.0044776097613,-14.8499483202528));
#36419=CARTESIAN_POINT('Ctrl Pts',(23.9110153591926,-28.5182079571721,1.62975553161124));
#36420=CARTESIAN_POINT('Ctrl Pts',(23.9260975032016,-28.474493215928,1.18963944141743));
#36421=CARTESIAN_POINT('Ctrl Pts',(23.9355515973832,-28.4163403666077,0.664246507169477));
#36422=CARTESIAN_POINT('Ctrl Pts',(24.0640354326688,-28.3045391652297,-1.95288623088664));
#36423=CARTESIAN_POINT('Ctrl Pts',(24.4051905243227,-28.5150692335449,-3.87317034517924));
#36424=CARTESIAN_POINT('Ctrl Pts',(25.5776818931252,-29.4765070006461,-7.48823335805061));
#36425=CARTESIAN_POINT('Ctrl Pts',(26.3866880329899,-30.225516684417,-9.12349227713595));
#36426=CARTESIAN_POINT('Ctrl Pts',(28.3801534902278,-32.1419665196991,-11.8775764776333));
#36427=CARTESIAN_POINT('Ctrl Pts',(29.5426791470737,-33.29895946217,-12.9726927515289));
#36428=CARTESIAN_POINT('Ctrl Pts',(32.1035612314812,-35.8626855592309,-14.4683433355073));
#36429=CARTESIAN_POINT('Ctrl Pts',(33.457602658903,-37.2410591163324,-14.849803898472));
#36430=CARTESIAN_POINT('Ctrl Pts',(34.8267964255883,-38.6282131180514,-14.8500516281495));
#36431=CARTESIAN_POINT('Ctrl Pts',(23.7833669488542,-29.4615086055165,1.59674386441329));
#36432=CARTESIAN_POINT('Ctrl Pts',(23.7985729183117,-29.4174349631987,1.15301439045616));
#36433=CARTESIAN_POINT('Ctrl Pts',(23.8084199485279,-29.3602882272675,0.63557920948043));
#36434=CARTESIAN_POINT('Ctrl Pts',(23.9362026442621,-29.2483924872748,-1.86860431095269));
#36435=CARTESIAN_POINT('Ctrl Pts',(24.2681366932972,-29.447145186903,-3.70979114469791));
#36436=CARTESIAN_POINT('Ctrl Pts',(25.3973651626803,-30.3599922883086,-7.1701426146977));
#36437=CARTESIAN_POINT('Ctrl Pts',(26.1771478463626,-31.0743967430082,-8.73670574476063));
#36438=CARTESIAN_POINT('Ctrl Pts',(28.0933077825166,-32.9020249034454,-11.3734544105045));
#36439=CARTESIAN_POINT('Ctrl Pts',(29.2117089637491,-34.00721590011,-12.4221714958469));
#36440=CARTESIAN_POINT('Ctrl Pts',(31.670121058349,-36.4540227505297,-13.854590909539));
#36441=CARTESIAN_POINT('Ctrl Pts',(32.972918011877,-37.7721633453099,-14.2195188098581));
#36442=CARTESIAN_POINT('Ctrl Pts',(34.2868769910997,-39.0960641936384,-14.2201291128084));
#36443=CARTESIAN_POINT('Ctrl Pts',(25.6404249706855,-27.772549528674,0.));
#36444=CARTESIAN_POINT('Ctrl Pts',(25.7366398496106,-27.6900511858228,-1.86858636168828));
#36445=CARTESIAN_POINT('Ctrl Pts',(26.0667980819016,-27.8867543207229,-3.71029995869047));
#36446=CARTESIAN_POINT('Ctrl Pts',(27.1980083507262,-28.8018888878774,-7.16936247494455));
#36447=CARTESIAN_POINT('Ctrl Pts',(27.9765753735453,-29.5148901762039,-8.73699595768932));
#36448=CARTESIAN_POINT('Ctrl Pts',(29.0323578083518,-30.5219411006642,-10.1890856763515));
#36449=CARTESIAN_POINT('Ctrl Pts',(29.1314899558969,-30.6168936176694,-10.3203928635195));
#36450=CARTESIAN_POINT('Ctrl Pts',(29.2322214279089,-30.7137407645584,-10.4488603766032));
#36451=CARTESIAN_POINT('Ctrl Pts',(23.8408520862196,-29.3318883095344,-9.99200722162641E-16));
#36452=CARTESIAN_POINT('Ctrl Pts',(23.9362026442621,-29.2483924872748,-1.86860431095269));
#36453=CARTESIAN_POINT('Ctrl Pts',(24.2681366932972,-29.447145186903,-3.70979114469791));
#36454=CARTESIAN_POINT('Ctrl Pts',(25.3973651626803,-30.3599922883086,-7.1701426146977));
#36455=CARTESIAN_POINT('Ctrl Pts',(26.1771478463626,-31.0743967430082,-8.73670574476063));
#36456=CARTESIAN_POINT('Ctrl Pts',(27.2380760953776,-32.0863072351954,-10.1966053555702));
#36457=CARTESIAN_POINT('Ctrl Pts',(27.3427718639698,-32.1866090102816,-10.3350231942247));
#36458=CARTESIAN_POINT('Ctrl Pts',(27.4492538662197,-32.2890256406517,-10.4702558450961));
#36459=CARTESIAN_POINT('Ctrl Pts',(31.6397608122763,-31.4394459897282,1.24689105568321));
#36460=CARTESIAN_POINT('Ctrl Pts',(31.6563000607434,-31.3915079136663,0.764254809547067));
#36461=CARTESIAN_POINT('Ctrl Pts',(31.670740810667,-31.345601660819,0.332948724824433));
#36462=CARTESIAN_POINT('Ctrl Pts',(31.797047945423,-31.2395462388234,-0.978870002751864));
#36463=CARTESIAN_POINT('Ctrl Pts',(32.0225645221739,-31.3034976581367,-1.98783577088394));
#36464=CARTESIAN_POINT('Ctrl Pts',(32.7052670086901,-31.7151448890356,-3.80852727284086));
#36465=CARTESIAN_POINT('Ctrl Pts',(33.1703611269064,-32.0570939854067,-4.65544360718913));
#36466=CARTESIAN_POINT('Ctrl Pts',(34.2727650719446,-32.949753301686,-6.04997283346398));
#36467=CARTESIAN_POINT('Ctrl Pts',(34.9217287192798,-33.5038992564753,-6.61832169897661));
#36468=CARTESIAN_POINT('Ctrl Pts',(36.3026175786965,-34.721296302326,-7.36768403083967));
#36469=CARTESIAN_POINT('Ctrl Pts',(37.0616291372384,-35.4005693947735,-7.57138648704198));
#36470=CARTESIAN_POINT('Ctrl Pts',(37.7934972961795,-36.0576472036358,-7.56962581969431));
#36471=CARTESIAN_POINT('Ctrl Pts',(29.4001542854013,-30.6671178491339,1.35489343606322));
#36472=CARTESIAN_POINT('Ctrl Pts',(29.4162823633167,-30.6203715276518,0.884255668141129));
#36473=CARTESIAN_POINT('Ctrl Pts',(29.4293136556724,-30.5710069006846,0.426397017775727));
#36474=CARTESIAN_POINT('Ctrl Pts',(29.5561964051723,-30.4632865153995,-1.25360819502645));
#36475=CARTESIAN_POINT('Ctrl Pts',(29.8143895731129,-30.5686507749899,-2.51960912779365));
#36476=CARTESIAN_POINT('Ctrl Pts',(30.6351795887969,-31.1352998840589,-4.84647586782702));
#36477=CARTESIAN_POINT('Ctrl Pts',(31.1973201148578,-31.5921137090582,-5.91572199044493));
#36478=CARTESIAN_POINT('Ctrl Pts',(32.5510483450044,-32.7735335073319,-7.69376028694199));
#36479=CARTESIAN_POINT('Ctrl Pts',(33.3448945810284,-33.4977500491925,-8.41063186553761));
#36480=CARTESIAN_POINT('Ctrl Pts',(35.0585937299527,-35.094871091134,-9.37059840622839));
#36481=CARTESIAN_POINT('Ctrl Pts',(35.9854803115295,-35.9713447024497,-9.62435378637548));
#36482=CARTESIAN_POINT('Ctrl Pts',(36.8970924436847,-36.8343596268993,-9.62320046360544));
#36483=CARTESIAN_POINT('Ctrl Pts',(27.3548849305451,-29.4725749263797,1.47293214974064));
#36484=CARTESIAN_POINT('Ctrl Pts',(27.3705645465914,-29.4271284462517,1.0153810678876));
#36485=CARTESIAN_POINT('Ctrl Pts',(27.3820741720678,-29.3740093215554,0.528580803079223));
#36486=CARTESIAN_POINT('Ctrl Pts',(27.509846270387,-29.2647682695536,-1.55402875454047));
#36487=CARTESIAN_POINT('Ctrl Pts',(27.803372614337,-29.4149573143382,-3.10121432123038));
#36488=CARTESIAN_POINT('Ctrl Pts',(28.7756052302995,-30.1516133539791,-5.9812914545136));
#36489=CARTESIAN_POINT('Ctrl Pts',(29.4435926416543,-30.7337162174463,-7.29389406574569));
#36490=CARTESIAN_POINT('Ctrl Pts',(31.072241043673,-32.2310076487121,-9.49113593806079));
#36491=CARTESIAN_POINT('Ctrl Pts',(32.0243541446183,-33.1410090871316,-10.3708286017028));
#36492=CARTESIAN_POINT('Ctrl Pts',(34.1021594176341,-35.1535638963754,-11.5604045561392));
#36493=CARTESIAN_POINT('Ctrl Pts',(35.2124714377991,-36.2455537133498,-11.8694761542189));
#36494=CARTESIAN_POINT('Ctrl Pts',(36.3206928540894,-37.3337834058792,-11.8687142284812));
#36495=CARTESIAN_POINT('Ctrl Pts',(25.5825535213021,-27.9017241322582,1.59647090706388));
#36496=CARTESIAN_POINT('Ctrl Pts',(25.5977646187892,-27.8576356266642,1.15259179092905));
#36497=CARTESIAN_POINT('Ctrl Pts',(25.6076988465248,-27.8006101679573,0.635573104293147));
#36498=CARTESIAN_POINT('Ctrl Pts',(25.7366398496106,-27.6900511858228,-1.86858636168828));
#36499=CARTESIAN_POINT('Ctrl Pts',(26.0667980819016,-27.8867543207229,-3.71029995869047));
#36500=CARTESIAN_POINT('Ctrl Pts',(27.1980083507262,-28.8018888878774,-7.16936247494455));
#36501=CARTESIAN_POINT('Ctrl Pts',(27.9765753735453,-29.5148901762039,-8.73699595768932));
#36502=CARTESIAN_POINT('Ctrl Pts',(29.8931745078293,-31.3430252790145,-11.3730256982303));
#36503=CARTESIAN_POINT('Ctrl Pts',(31.010856471336,-32.4473861125001,-12.4235805192179));
#36504=CARTESIAN_POINT('Ctrl Pts',(33.4700709138127,-34.895119122769,-13.8529470821642));
#36505=CARTESIAN_POINT('Ctrl Pts',(34.7723177498585,-36.2126515923892,-14.2204718557167));
#36506=CARTESIAN_POINT('Ctrl Pts',(36.0864498658144,-37.5367254229129,-14.2198708430666));
#36507=CARTESIAN_POINT('Ctrl Pts',(23.7833669488542,-29.4615086055165,1.59674386441329));
#36508=CARTESIAN_POINT('Ctrl Pts',(23.7985729183117,-29.4174349631987,1.15301439045615));
#36509=CARTESIAN_POINT('Ctrl Pts',(23.8084199485278,-29.3602882272675,0.635579209480434));
#36510=CARTESIAN_POINT('Ctrl Pts',(23.9362026442621,-29.2483924872748,-1.86860431095269));
#36511=CARTESIAN_POINT('Ctrl Pts',(24.2681366932972,-29.447145186903,-3.70979114469911));
#36512=CARTESIAN_POINT('Ctrl Pts',(25.3973651626803,-30.3599922883086,-7.17014261469651));
#36513=CARTESIAN_POINT('Ctrl Pts',(26.1771478463602,-31.0743967430034,-8.73670574475585));
#36514=CARTESIAN_POINT('Ctrl Pts',(28.093307782519,-32.9020249034502,-11.3734544105093));
#36515=CARTESIAN_POINT('Ctrl Pts',(29.2117089637491,-34.00721590011,-12.4221714958517));
#36516=CARTESIAN_POINT('Ctrl Pts',(31.670121058349,-36.4540227505297,-13.8545909095342));
#36517=CARTESIAN_POINT('Ctrl Pts',(32.9729180118699,-37.772163345317,-14.2195188098628));
#36518=CARTESIAN_POINT('Ctrl Pts',(34.2868769910997,-39.0960641936384,-14.2201291128084));
#36519=CARTESIAN_POINT('Ctrl Pts',(25.0869579521465,-31.4387285991346,1.47327622041466));
#36520=CARTESIAN_POINT('Ctrl Pts',(25.1026311041632,-31.3933008545996,1.01591376687672));
#36521=CARTESIAN_POINT('Ctrl Pts',(25.1140308146305,-31.3400288564348,0.52858849884529));
#36522=CARTESIAN_POINT('Ctrl Pts',(25.2403428328606,-31.2291027822936,-1.55405138011005));
#36523=CARTESIAN_POINT('Ctrl Pts',(25.5361076454386,-31.3818753629957,-3.10057294640152));
#36524=CARTESIAN_POINT('Ctrl Pts',(26.5058421455966,-32.1156479855689,-5.98227484335136));
#36525=CARTESIAN_POINT('Ctrl Pts',(27.1753619328071,-32.6995195810239,-7.29352824390757));
#36526=CARTESIAN_POINT('Ctrl Pts',(28.8034567128163,-34.196171996717,-9.49167634235024));
#36527=CARTESIAN_POINT('Ctrl Pts',(29.7564764086093,-35.1072198799437,-10.3690524867829));
#36528=CARTESIAN_POINT('Ctrl Pts',(31.833270298808,-37.118607237774,-11.5624766483317));
#36529=CARTESIAN_POINT('Ctrl Pts',(32.944279264244,-38.2113611019662,-11.8682745704546));
#36530=CARTESIAN_POINT('Ctrl Pts',(34.0522789304532,-39.2993752576346,-11.8690397849988));
#36531=CARTESIAN_POINT('Ctrl Pts',(25.9793365537795,-33.6327571359873,1.35541241355846));
#36532=CARTESIAN_POINT('Ctrl Pts',(25.9954548817075,-33.5860390742511,0.885059162330388));
#36533=CARTESIAN_POINT('Ctrl Pts',(26.0083203842378,-33.5364438612596,0.426408625650778));
#36534=CARTESIAN_POINT('Ctrl Pts',(26.1330008283223,-33.4261818802092,-1.2536423222053));
#36535=CARTESIAN_POINT('Ctrl Pts',(26.3945703806216,-33.5354430048945,-2.51864171287673));
#36536=CARTESIAN_POINT('Ctrl Pts',(27.211592374269,-34.0977429244413,-4.84795915807732));
#36537=CARTESIAN_POINT('Ctrl Pts',(27.7760442527403,-34.5572246086001,-5.91517020467798));
#36538=CARTESIAN_POINT('Ctrl Pts',(29.1289374295578,-35.7376805505258,-7.69457540338525));
#36539=CARTESIAN_POINT('Ctrl Pts',(29.9241511239614,-36.4634754928305,-8.40795287036384));
#36540=CARTESIAN_POINT('Ctrl Pts',(31.6363247580161,-38.0588356145494,-9.37372383742583));
#36541=CARTESIAN_POINT('Ctrl Pts',(32.5642699125034,-38.9364560608574,-9.62254085984917));
#36542=CARTESIAN_POINT('Ctrl Pts',(33.4755402303451,-39.799151493507,-9.62369151535381));
#36543=CARTESIAN_POINT('Ctrl Pts',(26.426208176239,-35.9592765491249,1.24768201173542));
#36544=CARTESIAN_POINT('Ctrl Pts',(26.4427325650799,-35.9113815427798,0.765479387872765));
#36545=CARTESIAN_POINT('Ctrl Pts',(26.4569206403346,-35.8651238615762,0.332966415994299));
#36546=CARTESIAN_POINT('Ctrl Pts',(26.5798713158818,-35.7551948794137,-0.978922014831213));
#36547=CARTESIAN_POINT('Ctrl Pts',(26.81053372586,-35.8250853790502,-1.98636136652122));
#36548=CARTESIAN_POINT('Ctrl Pts',(27.487493497402,-36.2301041572641,-3.81078790535579));
#36549=CARTESIAN_POINT('Ctrl Pts',(27.9561102696818,-36.576119247571,-4.65460264916223));
#36550=CARTESIAN_POINT('Ctrl Pts',(29.0572415381562,-37.467309582976,-6.0512151248706));
#36551=CARTESIAN_POINT('Ctrl Pts',(29.7082892825749,-38.0238611245159,-6.61423873302147));
#36552=CARTESIAN_POINT('Ctrl Pts',(31.0868531563715,-39.2385744113942,-7.37244739484306));
#36553=CARTESIAN_POINT('Ctrl Pts',(31.847493646553,-39.9195822825653,-7.56862230150026));
#36554=CARTESIAN_POINT('Ctrl Pts',(32.5788252613912,-40.57618623849,-7.57037421506001));
#36555=CARTESIAN_POINT('Ctrl Pts',(21.3513306581891,-31.2585017743467,1.59647086199746));
#36556=CARTESIAN_POINT('Ctrl Pts',(21.3726613764945,-31.2170267923822,1.15259176012307));
#36557=CARTESIAN_POINT('Ctrl Pts',(21.3906100567637,-31.161995560763,0.635573083853244));
#36558=CARTESIAN_POINT('Ctrl Pts',(21.5339728087505,-31.0709121284164,-1.86858636172315));
#36559=CARTESIAN_POINT('Ctrl Pts',(21.8327767315744,-31.3125995244281,-3.71029995869404));
#36560=CARTESIAN_POINT('Ctrl Pts',(22.8222356829128,-32.3794073477002,-7.16936247494135));
#36561=CARTESIAN_POINT('Ctrl Pts',(23.4914073530124,-33.1959529509023,-8.73699595767989));
#36562=CARTESIAN_POINT('Ctrl Pts',(25.128327520199,-35.2782407701336,-11.3730256982401));
#36563=CARTESIAN_POINT('Ctrl Pts',(26.0774661593741,-36.5304235306262,-12.4235805192514));
#36564=CARTESIAN_POINT('Ctrl Pts',(28.1633006173374,-39.3032248537516,-13.8529470821311));
#36565=CARTESIAN_POINT('Ctrl Pts',(29.2647880382297,-40.7926757902223,-14.2204718555883));
#36566=CARTESIAN_POINT('Ctrl Pts',(30.3771088306736,-42.290292958107,-14.2198708430668));
#36567=CARTESIAN_POINT('Ctrl Pts',(20.4102131175326,-31.1156831315059,1.62964630360506));
#36568=CARTESIAN_POINT('Ctrl Pts',(20.4313658791523,-31.0745541646277,1.18947037067355));
#36569=CARTESIAN_POINT('Ctrl Pts',(20.4490273775128,-31.0183916683951,0.664244043735995));
#36570=CARTESIAN_POINT('Ctrl Pts',(20.5924969120299,-30.9266087974369,-1.95287905122728));
#36571=CARTESIAN_POINT('Ctrl Pts',(20.8996315610477,-31.1826348335737,-3.87337387078343));
#36572=CARTESIAN_POINT('Ctrl Pts',(21.9240162327731,-32.3021679589246,-7.48792130214246));
#36573=CARTESIAN_POINT('Ctrl Pts',(22.6177912263091,-33.1580626257345,-9.12360836229315));
#36574=CARTESIAN_POINT('Ctrl Pts',(24.3183718641675,-35.3389311938522,-11.8774049927382));
#36575=CARTESIAN_POINT('Ctrl Pts',(25.3041699214186,-36.6492226398526,-12.9732563608963));
#36576=CARTESIAN_POINT('Ctrl Pts',(27.4743946038814,-39.5517175889618,-14.4676858045386));
#36577=CARTESIAN_POINT('Ctrl Pts',(28.6183079046584,-41.10848925655,-14.8501851004819));
#36578=CARTESIAN_POINT('Ctrl Pts',(29.7762110964233,-42.6764590955605,-14.8499483202528));
#36579=CARTESIAN_POINT('Ctrl Pts',(19.6090715485701,-31.6308259996109,1.62975548654487));
#36580=CARTESIAN_POINT('Ctrl Pts',(19.6302214337609,-31.5897026256071,1.18963941047971));
#36581=CARTESIAN_POINT('Ctrl Pts',(19.6478553119351,-31.5334871484505,0.66424648581248));
#36582=CARTESIAN_POINT('Ctrl Pts',(19.7909423356753,-31.4411090791454,-1.95288623093789));
#36583=CARTESIAN_POINT('Ctrl Pts',(20.0986634078842,-31.6980476865377,-3.87317034519232));
#36584=CARTESIAN_POINT('Ctrl Pts',(21.1223936447217,-32.8165623230617,-7.48823335803764));
#36585=CARTESIAN_POINT('Ctrl Pts',(21.8165700765696,-33.6730817461624,-9.12349227711679));
#36586=CARTESIAN_POINT('Ctrl Pts',(23.5170056814996,-35.8537245995369,-11.8775764776525));
#36587=CARTESIAN_POINT('Ctrl Pts',(24.5030412397929,-37.1643856730114,-12.9726927515286));
#36588=CARTESIAN_POINT('Ctrl Pts',(26.6730009723108,-40.0664682545599,-14.4683433355076));
#36589=CARTESIAN_POINT('Ctrl Pts',(27.8170972008577,-41.6235121428201,-14.8498038985433));
#36590=CARTESIAN_POINT('Ctrl Pts',(28.9749419513877,-43.1914035066782,-14.8500516281494));
#36591=CARTESIAN_POINT('Ctrl Pts',(19.3484767357829,-32.5463589446092,1.59674381934696));
#36592=CARTESIAN_POINT('Ctrl Pts',(19.3698002630062,-32.5048979448321,1.15301435963818));
#36593=CARTESIAN_POINT('Ctrl Pts',(19.3876798928189,-32.4497342608979,0.635579189044451));
#36594=CARTESIAN_POINT('Ctrl Pts',(19.5300863678652,-32.3571628326983,-1.86860431099967));
#36595=CARTESIAN_POINT('Ctrl Pts',(19.8303563486669,-32.6011316568334,-3.70979114471326));
#36596=CARTESIAN_POINT('Ctrl Pts',(20.8181792127831,-33.6653932580479,-7.17014261468231));
#36597=CARTESIAN_POINT('Ctrl Pts',(21.4883544786661,-34.4835007519627,-8.7367057447366));
#36598=CARTESIAN_POINT('Ctrl Pts',(23.124912063527,-36.5652242843549,-11.3734544105284));
#36599=CARTESIAN_POINT('Ctrl Pts',(24.0746444553041,-37.8183311135135,-12.4221714958272));
#36600=CARTESIAN_POINT('Ctrl Pts',(26.1598165384169,-40.5901015177564,-13.8545909095583));
#36601=CARTESIAN_POINT('Ctrl Pts',(27.2617619321778,-42.0802326794159,-14.2195188100387));
#36602=CARTESIAN_POINT('Ctrl Pts',(28.3739359680845,-43.5776539859013,-14.2201291128083));
#36603=CARTESIAN_POINT('Ctrl Pts',(21.4269965203137,-31.1388779521432,0.));
#36604=CARTESIAN_POINT('Ctrl Pts',(21.5339728087505,-31.0709121284164,-1.86858636172315));
#36605=CARTESIAN_POINT('Ctrl Pts',(21.8327767315744,-31.3125995244281,-3.71029995869284));
#36606=CARTESIAN_POINT('Ctrl Pts',(22.8222356829128,-32.3794073477002,-7.16936247494255));
#36607=CARTESIAN_POINT('Ctrl Pts',(23.4914073530124,-33.1959529508975,-8.7369959576799));
#36608=CARTESIAN_POINT('Ctrl Pts',(24.3931251555408,-34.3430070554509,-10.1890856763512));
#36609=CARTESIAN_POINT('Ctrl Pts',(24.4777351286612,-34.4511010682878,-10.320392863519));
#36610=CARTESIAN_POINT('Ctrl Pts',(24.5636585134848,-34.5612980340113,-10.4488603766026));
#36611=CARTESIAN_POINT('Ctrl Pts',(19.4238236466304,-32.4262389885815,-1.83186799063151E-15));
#36612=CARTESIAN_POINT('Ctrl Pts',(19.5300863678652,-32.3571628326983,-1.86860431099967));
#36613=CARTESIAN_POINT('Ctrl Pts',(19.8303563486669,-32.6011316568334,-3.70979114471326));
#36614=CARTESIAN_POINT('Ctrl Pts',(20.8181792127831,-33.6653932580479,-7.17014261468231));
#36615=CARTESIAN_POINT('Ctrl Pts',(21.4883544786661,-34.4835007519627,-8.7367057447366));
#36616=CARTESIAN_POINT('Ctrl Pts',(22.3944741298276,-35.6360972865638,-10.1966053555717));
#36617=CARTESIAN_POINT('Ctrl Pts',(22.4838298155557,-35.750277895577,-10.3350231942271));
#36618=CARTESIAN_POINT('Ctrl Pts',(22.5746525783696,-35.8668060412515,-10.4702558450987));
#36619=CARTESIAN_POINT('Ctrl Pts',(26.8434139987109,-35.6222452002844,1.24689101061693));
#36620=CARTESIAN_POINT('Ctrl Pts',(26.866607200265,-35.5771488466461,0.764254780049364));
#36621=CARTESIAN_POINT('Ctrl Pts',(26.8874341048552,-35.5337649883207,0.332948714090238));
#36622=CARTESIAN_POINT('Ctrl Pts',(27.0275488741942,-35.4467644376545,-0.978870002691829));
#36623=CARTESIAN_POINT('Ctrl Pts',(27.2416687814358,-35.5421592790288,-1.9878357708727));
#36624=CARTESIAN_POINT('Ctrl Pts',(27.8588388319676,-36.0467752284862,-3.80852727285255));
#36625=CARTESIAN_POINT('Ctrl Pts',(28.2705345323081,-36.4514335703569,-4.6554436072038));
#36626=CARTESIAN_POINT('Ctrl Pts',(29.2346789284779,-37.4918953411199,-6.04997283344998));
#36627=CARTESIAN_POINT('Ctrl Pts',(29.7981738697234,-38.1327580455423,-6.61832169904879));
#36628=CARTESIAN_POINT('Ctrl Pts',(30.9917536078527,-39.5342847195952,-7.36768403076832));
#36629=CARTESIAN_POINT('Ctrl Pts',(31.6463688825543,-40.3146623988151,-7.57138648661861));
#36630=CARTESIAN_POINT('Ctrl Pts',(32.2772757571271,-41.0692078014243,-7.56962581969465));
#36631=CARTESIAN_POINT('Ctrl Pts',(24.7365171914562,-34.539049005888,1.35489339099691));
#36632=CARTESIAN_POINT('Ctrl Pts',(24.7591338032426,-34.4950737607861,0.884255638235974));
#36633=CARTESIAN_POINT('Ctrl Pts',(24.7790577744578,-34.4480661428797,0.426397004045326));
#36634=CARTESIAN_POINT('Ctrl Pts',(24.9199792485556,-34.3594994944374,-1.25360819499821));
#36635=CARTESIAN_POINT('Ctrl Pts',(25.1605494847799,-34.5005360168067,-2.5196091277897));
#36636=CARTESIAN_POINT('Ctrl Pts',(25.8923424652774,-35.1782280532491,-4.84647586783132));
#36637=CARTESIAN_POINT('Ctrl Pts',(26.3837498256842,-35.7103931102545,-5.91572199044753));
#36638=CARTESIAN_POINT('Ctrl Pts',(27.5555654868577,-37.0724433726229,-7.69376028693985));
#36639=CARTESIAN_POINT('Ctrl Pts',(28.2382647528021,-37.9022645329766,-8.41063186558564));
#36640=CARTESIAN_POINT('Ctrl Pts',(29.7072268925326,-39.7270140028395,-9.37059840618092));
#36641=CARTESIAN_POINT('Ctrl Pts',(30.4999439048052,-40.7264760905893,-9.62435378611397));
#36642=CARTESIAN_POINT('Ctrl Pts',(31.27945731062,-41.7104427005358,-9.62320046360565));
#36643=CARTESIAN_POINT('Ctrl Pts',(22.8820669124599,-33.065592630237,1.47293210467427));
#36644=CARTESIAN_POINT('Ctrl Pts',(22.9040546403826,-33.0228401731498,1.01538103754122));
#36645=CARTESIAN_POINT('Ctrl Pts',(22.9230067538248,-32.9718997171416,0.528580786071612));
#36646=CARTESIAN_POINT('Ctrl Pts',(23.0650249378515,-32.8819544477584,-1.55402875454427));
#36647=CARTESIAN_POINT('Ctrl Pts',(23.3341894772925,-33.072387938809,-3.10121432123136));
#36648=CARTESIAN_POINT('Ctrl Pts',(24.1916890818784,-33.9399090096345,-5.98129145451293));
#36649=CARTESIAN_POINT('Ctrl Pts',(24.7700354696729,-34.6111514256828,-7.29389406574346));
#36650=CARTESIAN_POINT('Ctrl Pts',(26.1690197914296,-36.3249834230533,-9.4911359380634));
#36651=CARTESIAN_POINT('Ctrl Pts',(26.981935046259,-37.3612221809256,-10.3708286017411));
#36652=CARTESIAN_POINT('Ctrl Pts',(28.7521748453974,-39.6489946054402,-11.5604045561013));
#36653=CARTESIAN_POINT('Ctrl Pts',(29.6957791360107,-40.8878834161155,-11.869476154062));
#36654=CARTESIAN_POINT('Ctrl Pts',(30.6378492234115,-42.1227528511813,-11.8687142284813));
#36655=CARTESIAN_POINT('Ctrl Pts',(21.3513306581891,-31.2585017743466,1.59647086199746));
#36656=CARTESIAN_POINT('Ctrl Pts',(21.3726613764946,-31.2170267923868,1.15259176012262));
#36657=CARTESIAN_POINT('Ctrl Pts',(21.3906100567637,-31.161995560763,0.635573083853244));
#36658=CARTESIAN_POINT('Ctrl Pts',(21.5339728087505,-31.0709121284164,-1.86858636172315));
#36659=CARTESIAN_POINT('Ctrl Pts',(21.8327767315744,-31.3125995244281,-3.71029995869284));
#36660=CARTESIAN_POINT('Ctrl Pts',(22.8222356829128,-32.3794073477002,-7.16936247494255));
#36661=CARTESIAN_POINT('Ctrl Pts',(23.4914073530124,-33.1959529508975,-8.7369959576799));
#36662=CARTESIAN_POINT('Ctrl Pts',(25.1283275201989,-35.2782407701384,-11.3730256982401));
#36663=CARTESIAN_POINT('Ctrl Pts',(26.0774661593717,-36.5304235306214,-12.4235805192514));
#36664=CARTESIAN_POINT('Ctrl Pts',(28.1633006173398,-39.3032248537564,-13.8529470821311));
#36665=CARTESIAN_POINT('Ctrl Pts',(29.2647880382258,-40.7926757902203,-14.2204718555836));
#36666=CARTESIAN_POINT('Ctrl Pts',(30.3771088306736,-42.290292958107,-14.2198708430668));
#36667=CARTESIAN_POINT('Ctrl Pts',(19.3484767357829,-32.5463589446092,1.59674381934696));
#36668=CARTESIAN_POINT('Ctrl Pts',(19.3698002630062,-32.5048979448321,1.15301435963818));
#36669=CARTESIAN_POINT('Ctrl Pts',(19.3876798928189,-32.4497342608979,0.635579189044451));
#36670=CARTESIAN_POINT('Ctrl Pts',(19.5300863678652,-32.3571628326983,-1.86860431099967));
#36671=CARTESIAN_POINT('Ctrl Pts',(19.8303563486669,-32.6011316568334,-3.70979114471326));
#36672=CARTESIAN_POINT('Ctrl Pts',(20.8181792127831,-33.6653932580479,-7.17014261468231));
#36673=CARTESIAN_POINT('Ctrl Pts',(21.4883544786661,-34.4835007519627,-8.7367057447366));
#36674=CARTESIAN_POINT('Ctrl Pts',(23.124912063527,-36.5652242843549,-11.3734544105284));
#36675=CARTESIAN_POINT('Ctrl Pts',(24.0746444553089,-37.8183311135135,-12.4221714958272));
#36676=CARTESIAN_POINT('Ctrl Pts',(26.1598165384121,-40.5901015177564,-13.8545909095583));
#36677=CARTESIAN_POINT('Ctrl Pts',(27.261761932179,-42.0802326794176,-14.2195188100435));
#36678=CARTESIAN_POINT('Ctrl Pts',(28.3739359680845,-43.5776539859013,-14.2201291128083));
#36679=CARTESIAN_POINT('Ctrl Pts',(20.3574113186621,-34.6889740324162,1.47327617534843));
#36680=CARTESIAN_POINT('Ctrl Pts',(20.379389982015,-34.6462392002803,1.01591373651561));
#36681=CARTESIAN_POINT('Ctrl Pts',(20.398255055351,-34.5951317842797,0.528588481842604));
#36682=CARTESIAN_POINT('Ctrl Pts',(20.539067824495,-34.5033108528715,-1.55405138012912));
#36683=CARTESIAN_POINT('Ctrl Pts',(20.8100803726341,-34.6966201503891,-3.10057294642143));
#36684=CARTESIAN_POINT('Ctrl Pts',(21.6655176417181,-35.5609316342938,-5.98227484333125));
#36685=CARTESIAN_POINT('Ctrl Pts',(22.2451290911725,-36.234142858994,-7.29352824388825));
#36686=CARTESIAN_POINT('Ctrl Pts',(23.6436563673638,-37.9472635563897,-9.49167634236925));
#36687=CARTESIAN_POINT('Ctrl Pts',(24.457320064615,-38.9846671296937,-10.3690524867584));
#36688=CARTESIAN_POINT('Ctrl Pts',(26.2267249209897,-41.2711400509677,-11.5624766483557));
#36689=CARTESIAN_POINT('Ctrl Pts',(27.1709103277658,-42.5108843176116,-11.86827457064));
#36690=CARTESIAN_POINT('Ctrl Pts',(28.1127915962414,-43.7455088513561,-11.8690397849986));
#36691=CARTESIAN_POINT('Ctrl Pts',(20.9284639764449,-36.9876692386616,1.35541236849233));
#36692=CARTESIAN_POINT('Ctrl Pts',(20.9510669157225,-36.9437205780704,0.885059132402747));
#36693=CARTESIAN_POINT('Ctrl Pts',(20.9708596003777,-36.8964611268003,0.426408611927824));
#36694=CARTESIAN_POINT('Ctrl Pts',(21.1099628922185,-36.8050653317413,-1.25364232220009));
#36695=CARTESIAN_POINT('Ctrl Pts',(21.353320564272,-36.950439564209,-2.51864171289876));
#36696=CARTESIAN_POINT('Ctrl Pts',(22.0820028300379,-37.6232904342815,-4.84795915805486));
#36697=CARTESIAN_POINT('Ctrl Pts',(22.575318340659,-38.1584251351965,-5.91517020465855));
#36698=CARTESIAN_POINT('Ctrl Pts',(23.7464446191649,-39.5194025113536,-7.69457540340414));
#36699=CARTESIAN_POINT('Ctrl Pts',(24.430272794963,-40.3509806159742,-8.40795287032015));
#36700=CARTESIAN_POINT('Ctrl Pts',(25.8979755524144,-42.1737699858021,-9.37372383746887));
#36701=CARTESIAN_POINT('Ctrl Pts',(26.6915771512776,-43.1745178860539,-9.62254086016299));
#36702=CARTESIAN_POINT('Ctrl Pts',(27.470797690331,-44.1581196109332,-9.6236915153536));
#36703=CARTESIAN_POINT('Ctrl Pts',(21.0396888561029,-39.3541045014167,1.24768196666942));
#36704=CARTESIAN_POINT('Ctrl Pts',(21.0628612198541,-39.3090486643396,0.765479358340059));
#36705=CARTESIAN_POINT('Ctrl Pts',(21.0834880350321,-39.2652809952898,0.332966405271473));
#36706=CARTESIAN_POINT('Ctrl Pts',(21.2208317742708,-39.1739686379383,-0.978922014806281));
#36707=CARTESIAN_POINT('Ctrl Pts',(21.4391999182059,-39.2759744365989,-1.98636136655255));
#36708=CARTESIAN_POINT('Ctrl Pts',(22.0516290336034,-39.773212128077,-3.81078790532374));
#36709=CARTESIAN_POINT('Ctrl Pts',(22.4662328811655,-40.182396403819,-4.65460264913786));
#36710=CARTESIAN_POINT('Ctrl Pts',(23.4293266125158,-41.2212230249917,-6.05121512489411));
#36711=CARTESIAN_POINT('Ctrl Pts',(23.9945420870899,-41.8647634287527,-6.61423873295368));
#36712=CARTESIAN_POINT('Ctrl Pts',(25.1862024432922,-43.2633027806342,-7.37244739490986));
#36713=CARTESIAN_POINT('Ctrl Pts',(25.8421831847501,-44.0456294021952,-7.56862230195687));
#36714=CARTESIAN_POINT('Ctrl Pts',(26.4726264127399,-44.7996294168198,-7.57037421505967));
#36715=CARTESIAN_POINT('Ctrl Pts',(16.6854562787119,-33.9789464595044,1.5964707761033));
#36716=CARTESIAN_POINT('Ctrl Pts',(16.7124723847588,-33.9409293131124,1.15259170142611));
#36717=CARTESIAN_POINT('Ctrl Pts',(16.7380701329864,-33.8890125875568,0.635573044868113));
#36718=CARTESIAN_POINT('Ctrl Pts',(16.8929361804822,-33.8192589011466,-1.86858636170883));
#36719=CARTESIAN_POINT('Ctrl Pts',(17.1543030075059,-34.1010104999082,-3.71029995866542));
#36720=CARTESIAN_POINT('Ctrl Pts',(17.9818681105058,-35.297774448411,-7.16936247496946));
#36721=CARTESIAN_POINT('Ctrl Pts',(18.5280220223184,-36.2012418527466,-8.7369959577178));
#36722=CARTESIAN_POINT('Ctrl Pts',(19.8519402484503,-38.4952930132141,-11.3730256982018));
#36723=CARTESIAN_POINT('Ctrl Pts',(20.6132138377593,-39.8698068705691,-12.4235805191893));
#36724=CARTESIAN_POINT('Ctrl Pts',(22.2832067363974,-42.9112302679935,-13.8529470821929));
#36725=CARTESIAN_POINT('Ctrl Pts',(23.1615116341715,-44.5422787457887,-14.2204718557452));
#36726=CARTESIAN_POINT('Ctrl Pts',(24.0493774600887,-46.1829520838075,-14.2198708430667));
#36727=CARTESIAN_POINT('Ctrl Pts',(15.7742431696982,-33.7036465139256,1.62964621771091));
#36728=CARTESIAN_POINT('Ctrl Pts',(15.801033887339,-33.6659465347865,1.18947031174229));
#36729=CARTESIAN_POINT('Ctrl Pts',(15.8265083724794,-33.6128691890278,0.66424400298923));
#36730=CARTESIAN_POINT('Ctrl Pts',(15.9815796561098,-33.5424383800186,-1.9528790512035));
#36731=CARTESIAN_POINT('Ctrl Pts',(16.2491518132913,-33.8395682581736,-3.8733738707548));
#36732=CARTESIAN_POINT('Ctrl Pts',(17.103783550365,-35.0934912894727,-7.48792130217063));
#36733=CARTESIAN_POINT('Ctrl Pts',(17.6686904036183,-36.0394086587071,-9.12360836231914));
#36734=CARTESIAN_POINT('Ctrl Pts',(19.041591625316,-38.4400969876946,-11.8774049927119));
#36735=CARTESIAN_POINT('Ctrl Pts',(19.8308817645067,-39.8773452471076,-12.9732563608583));
#36736=CARTESIAN_POINT('Ctrl Pts',(21.5659485893962,-43.0591521575738,-14.4676858045765));
#36737=CARTESIAN_POINT('Ctrl Pts',(22.4766667937634,-44.7628739707726,-14.8501851005341));
#36738=CARTESIAN_POINT('Ctrl Pts',(23.3996388269518,-46.4796709429186,-14.8499483202528));
#36739=CARTESIAN_POINT('Ctrl Pts',(14.907943592795,-34.099531637587,1.62975540065068));
#36740=CARTESIAN_POINT('Ctrl Pts',(14.934730667332,-34.0618367850497,1.18963935154091));
#36741=CARTESIAN_POINT('Ctrl Pts',(14.9601853533923,-34.008703066853,0.664246445062532));
#36742=CARTESIAN_POINT('Ctrl Pts',(15.1149627252082,-33.9376286807998,-1.9528862309052));
#36743=CARTESIAN_POINT('Ctrl Pts',(15.3829854642134,-34.2357452982714,-3.87317034516976));
#36744=CARTESIAN_POINT('Ctrl Pts',(16.237114373674,-35.4885670717109,-7.48823335805989));
#36745=CARTESIAN_POINT('Ctrl Pts',(16.8023296670996,-36.4351599687639,-9.12349227712133));
#36746=CARTESIAN_POINT('Ctrl Pts',(18.1751194546256,-38.8356042400712,-11.8775764776479));
#36747=CARTESIAN_POINT('Ctrl Pts',(18.9645920739779,-40.2732521646236,-12.9726927515242));
#36748=CARTESIAN_POINT('Ctrl Pts',(20.6994553317568,-43.4546131985424,-14.468343335512));
#36749=CARTESIAN_POINT('Ctrl Pts',(21.6103158609142,-45.1586304949195,-14.8498038985005));
#36750=CARTESIAN_POINT('Ctrl Pts',(22.53324121589,-46.8753414736306,-14.8500516281495));
#36751=CARTESIAN_POINT('Ctrl Pts',(14.5197073364539,-34.968659268658,1.5967437334527));
#36752=CARTESIAN_POINT('Ctrl Pts',(14.5467143347417,-34.9306549387484,1.15301430092464));
#36753=CARTESIAN_POINT('Ctrl Pts',(14.5722625852684,-34.8785972821207,0.635579150051368));
#36754=CARTESIAN_POINT('Ctrl Pts',(14.7263938532288,-34.8072346530974,-1.86860431096307));
#36755=CARTESIAN_POINT('Ctrl Pts',(14.9888871348065,-35.0914531001455,-3.70979114469921));
#36756=CARTESIAN_POINT('Ctrl Pts',(15.8151951687831,-36.2854639040137,-7.17014261469621));
#36757=CARTESIAN_POINT('Ctrl Pts',(16.3621201810158,-37.190620127891,-8.73670574472687));
#36758=CARTESIAN_POINT('Ctrl Pts',(17.6857598217302,-39.4840611441532,-11.3734544105381));
#36759=CARTESIAN_POINT('Ctrl Pts',(18.4474896114335,-40.8595741643688,-12.4221714958517));
#36760=CARTESIAN_POINT('Ctrl Pts',(20.1169735923025,-43.8998828704052,-13.854590909534));
#36761=CARTESIAN_POINT('Ctrl Pts',(20.995634995294,-45.5316698260174,-14.2195188099104));
#36762=CARTESIAN_POINT('Ctrl Pts',(21.8833834324342,-47.1721284105875,-14.2201291128084));
#36763=CARTESIAN_POINT('Ctrl Pts',(16.7773762111438,-33.8713086176154,0.));
#36764=CARTESIAN_POINT('Ctrl Pts',(16.8929361804822,-33.8192589011466,-1.86858636170883));
#36765=CARTESIAN_POINT('Ctrl Pts',(17.1543030075107,-34.1010104999082,-3.71029995866542));
#36766=CARTESIAN_POINT('Ctrl Pts',(17.981868110501,-35.297774448411,-7.16936247496945));
#36767=CARTESIAN_POINT('Ctrl Pts',(18.5280220223185,-36.2012418527466,-8.73699595771779));
#36768=CARTESIAN_POINT('Ctrl Pts',(19.2573188185374,-37.4649484236423,-10.1890856763477));
#36769=CARTESIAN_POINT('Ctrl Pts',(19.3256842021847,-37.5839834499261,-10.3203928635122));
#36770=CARTESIAN_POINT('Ctrl Pts',(19.3950503474966,-37.7052869420423,-10.4488603765928));
#36771=CARTESIAN_POINT('Ctrl Pts',(14.6113821712778,-34.8604849513725,1.33226762955019E-15));
#36772=CARTESIAN_POINT('Ctrl Pts',(14.7263938532288,-34.8072346530974,-1.86860431096307));
#36773=CARTESIAN_POINT('Ctrl Pts',(14.9888871348065,-35.0914531001455,-3.70979114469921));
#36774=CARTESIAN_POINT('Ctrl Pts',(15.8151951687831,-36.2854639040137,-7.17014261469621));
#36775=CARTESIAN_POINT('Ctrl Pts',(16.3621201810158,-37.190620127891,-8.73670574472687));
#36776=CARTESIAN_POINT('Ctrl Pts',(17.094985251334,-38.4604391631886,-10.1966053555743));
#36777=CARTESIAN_POINT('Ctrl Pts',(17.1671818301258,-38.5861742181928,-10.3350231942322));
#36778=CARTESIAN_POINT('Ctrl Pts',(17.2404964639728,-38.7144417021593,-10.4702558451063));
#36779=CARTESIAN_POINT('Ctrl Pts',(21.5006126898289,-39.0798782217545,1.24689092472231));
#36780=CARTESIAN_POINT('Ctrl Pts',(21.5299876965087,-39.0385416232163,0.764254723798825));
#36781=CARTESIAN_POINT('Ctrl Pts',(21.5567767789514,-38.9985633313588,0.332948693682486));
#36782=CARTESIAN_POINT('Ctrl Pts',(21.707846848885,-38.9323887327204,-0.978870002727929));
#36783=CARTESIAN_POINT('Ctrl Pts',(21.9062112227949,-39.0572850320887,-1.98783577086018));
#36784=CARTESIAN_POINT('Ctrl Pts',(22.4452850348812,-39.6445971746381,-3.80852727286484));
#36785=CARTESIAN_POINT('Ctrl Pts',(22.7952013801788,-40.1037270849617,-4.65544360727524));
#36786=CARTESIAN_POINT('Ctrl Pts',(23.6014590278217,-41.2708105092157,-6.04997283337807));
#36787=CARTESIAN_POINT('Ctrl Pts',(24.0680141308967,-41.9853438467174,-6.61832169891444));
#36788=CARTESIAN_POINT('Ctrl Pts',(25.0499869065097,-43.5424691073157,-7.36768403090209));
#36789=CARTESIAN_POINT('Ctrl Pts',(25.5868798186132,-44.4080651338149,-7.57138648702774));
#36790=CARTESIAN_POINT('Ctrl Pts',(26.1039819636362,-45.2447177621913,-7.56962581969438));
#36791=CARTESIAN_POINT('Ctrl Pts',(19.5693159454015,-37.7078647243941,1.35489330510241));
#36792=CARTESIAN_POINT('Ctrl Pts',(19.5979606808328,-37.6675557657759,0.8842555812278));
#36793=CARTESIAN_POINT('Ctrl Pts',(19.6243717351794,-37.6238620982266,0.426396977899446));
#36794=CARTESIAN_POINT('Ctrl Pts',(19.7764631777508,-37.5562521484589,-1.25360819501416));
#36795=CARTESIAN_POINT('Ctrl Pts',(19.9945131659745,-37.7300898366309,-2.51960912777466));
#36796=CARTESIAN_POINT('Ctrl Pts',(20.6224119165102,-38.5050289449296,-4.84647586784612));
#36797=CARTESIAN_POINT('Ctrl Pts',(21.0330824745289,-39.1017118879348,-5.91572199049987));
#36798=CARTESIAN_POINT('Ctrl Pts',(21.9991307790699,-40.6166651990075,-7.69376028688717));
#36799=CARTESIAN_POINT('Ctrl Pts',(22.5567852866068,-41.5351982120271,-8.41063186549458));
#36800=CARTESIAN_POINT('Ctrl Pts',(23.7511065841813,-43.5504294726429,-9.37059840627156));
#36801=CARTESIAN_POINT('Ctrl Pts',(24.3935165949966,-44.6525338708106,-9.62435378636601));
#36802=CARTESIAN_POINT('Ctrl Pts',(25.025062629217,-45.7374214437733,-9.62320046360548));
#36803=CARTESIAN_POINT('Ctrl Pts',(17.9434360021525,-35.9854902185573,1.47293201877993));
#36804=CARTESIAN_POINT('Ctrl Pts',(17.9712842340237,-35.9463021021765,1.01538097970665));
#36805=CARTESIAN_POINT('Ctrl Pts',(17.9972930238881,-35.8985773174066,0.528580753652916));
#36806=CARTESIAN_POINT('Ctrl Pts',(18.1506662116866,-35.8297588571569,-1.5540287545432));
#36807=CARTESIAN_POINT('Ctrl Pts',(18.3899895327298,-36.0565601177377,-3.10121432121015));
#36808=CARTESIAN_POINT('Ctrl Pts',(19.1152999068282,-37.0372859924681,-5.9812914545338));
#36809=CARTESIAN_POINT('Ctrl Pts',(19.592231806385,-37.7840034012006,-7.29389406577903));
#36810=CARTESIAN_POINT('Ctrl Pts',(20.7330727614825,-39.6794872875133,-9.49113593802749));
#36811=CARTESIAN_POINT('Ctrl Pts',(21.3902415598918,-40.8208685319424,-10.3708286016693));
#36812=CARTESIAN_POINT('Ctrl Pts',(22.8168789076759,-43.3372861226379,-11.5604045561727));
#36813=CARTESIAN_POINT('Ctrl Pts',(23.5745664063873,-44.6978537235901,-11.8694761542189));
#36814=CARTESIAN_POINT('Ctrl Pts',(24.3313073348065,-46.0542245204215,-11.8687142284812));
#36815=CARTESIAN_POINT('Ctrl Pts',(16.6854562787119,-33.9789464595044,1.5964707761033));
#36816=CARTESIAN_POINT('Ctrl Pts',(16.7124723847588,-33.9409293131124,1.15259170142612));
#36817=CARTESIAN_POINT('Ctrl Pts',(16.7380701329864,-33.8890125875568,0.635573044868113));
#36818=CARTESIAN_POINT('Ctrl Pts',(16.8929361804822,-33.8192589011466,-1.86858636170883));
#36819=CARTESIAN_POINT('Ctrl Pts',(17.1543030075107,-34.1010104999082,-3.71029995866542));
#36820=CARTESIAN_POINT('Ctrl Pts',(17.981868110501,-35.297774448411,-7.16936247496945));
#36821=CARTESIAN_POINT('Ctrl Pts',(18.5280220223185,-36.2012418527466,-8.73699595771779));
#36822=CARTESIAN_POINT('Ctrl Pts',(19.8519402484503,-38.4952930132141,-11.3730256982018));
#36823=CARTESIAN_POINT('Ctrl Pts',(20.6132138377593,-39.8698068705739,-12.4235805191845));
#36824=CARTESIAN_POINT('Ctrl Pts',(22.2832067363974,-42.9112302679887,-13.8529470821977));
#36825=CARTESIAN_POINT('Ctrl Pts',(23.161511634173,-44.5422787457915,-14.2204718557262));
#36826=CARTESIAN_POINT('Ctrl Pts',(24.0493774600887,-46.1829520838075,-14.2198708430667));
#36827=CARTESIAN_POINT('Ctrl Pts',(14.5197073364539,-34.968659268658,1.5967437334527));
#36828=CARTESIAN_POINT('Ctrl Pts',(14.5467143347417,-34.9306549387484,1.15301430092464));
#36829=CARTESIAN_POINT('Ctrl Pts',(14.5722625852684,-34.8785972821207,0.635579150051368));
#36830=CARTESIAN_POINT('Ctrl Pts',(14.7263938532288,-34.8072346530974,-1.86860431096307));
#36831=CARTESIAN_POINT('Ctrl Pts',(14.9888871348065,-35.0914531001455,-3.70979114469921));
#36832=CARTESIAN_POINT('Ctrl Pts',(15.8151951687831,-36.2854639040137,-7.17014261469621));
#36833=CARTESIAN_POINT('Ctrl Pts',(16.3621201810157,-37.1906201278862,-8.73670574472927));
#36834=CARTESIAN_POINT('Ctrl Pts',(17.6857598217302,-39.4840611441579,-11.3734544105357));
#36835=CARTESIAN_POINT('Ctrl Pts',(18.4474896114359,-40.8595741643688,-12.4221714958517));
#36836=CARTESIAN_POINT('Ctrl Pts',(20.1169735923001,-43.8998828704052,-13.854590909534));
#36837=CARTESIAN_POINT('Ctrl Pts',(20.9956349952846,-45.5316698260234,-14.2195188099104));
#36838=CARTESIAN_POINT('Ctrl Pts',(21.8833834324342,-47.1721284105874,-14.2201291128084));
#36839=CARTESIAN_POINT('Ctrl Pts',(15.2134465003397,-37.2330519862578,1.47327608945396));
#36840=CARTESIAN_POINT('Ctrl Pts',(15.2412832516114,-37.1938800254387,1.0159136786583));
#36841=CARTESIAN_POINT('Ctrl Pts',(15.2672296481897,-37.1459775929453,0.528588449413895));
#36842=CARTESIAN_POINT('Ctrl Pts',(15.4196766250218,-37.0751310137469,-1.55405138009996));
#36843=CARTESIAN_POINT('Ctrl Pts',(15.6604198747747,-37.3050418083239,-3.10057294641483));
#36844=CARTESIAN_POINT('Ctrl Pts',(16.3841456768324,-38.2822972641882,-5.98227484333796));
#36845=CARTESIAN_POINT('Ctrl Pts',(16.8620495708872,-39.0311434790522,-7.29352824387148));
#36846=CARTESIAN_POINT('Ctrl Pts',(18.002539360956,-40.925858260867,-9.49167634238626));
#36847=CARTESIAN_POINT('Ctrl Pts',(18.6602832132299,-42.0684989791172,-10.3690524867973));
#36848=CARTESIAN_POINT('Ctrl Pts',(20.0862790553718,-44.5835114689251,-11.5624766483172));
#36849=CARTESIAN_POINT('Ctrl Pts',(20.8444200112022,-45.9450085199817,-11.8682745704784));
#36850=CARTESIAN_POINT('Ctrl Pts',(21.6010088957266,-47.301110036494,-11.8690397849987));
#36851=CARTESIAN_POINT('Ctrl Pts',(15.4515482289397,-39.5896190563863,1.35541228259766));
#36852=CARTESIAN_POINT('Ctrl Pts',(15.4801756476595,-39.5493344659312,0.885059075360922));
#36853=CARTESIAN_POINT('Ctrl Pts',(15.5064925913678,-39.505372844223,0.426408585766831));
#36854=CARTESIAN_POINT('Ctrl Pts',(15.6571869876725,-39.434703790117,-1.25364232217367));
#36855=CARTESIAN_POINT('Ctrl Pts',(15.8773787191569,-39.6132317302722,-2.51864171290804));
#36856=CARTESIAN_POINT('Ctrl Pts',(16.5028873873922,-40.3829362474817,-4.84795915804603));
#36857=CARTESIAN_POINT('Ctrl Pts',(16.9150240490585,-40.9828301658884,-5.9151702046228));
#36858=CARTESIAN_POINT('Ctrl Pts',(17.880542675362,-42.496623401559,-7.69457540344039));
#36859=CARTESIAN_POINT('Ctrl Pts',(18.4390645628778,-43.4170561363982,-8.40795287039259));
#36860=CARTESIAN_POINT('Ctrl Pts',(19.6324182482298,-45.4301680192512,-9.37372383739693));
#36861=CARTESIAN_POINT('Ctrl Pts',(20.2755208515495,-46.533671031965,-9.62254085992524));
#36862=CARTESIAN_POINT('Ctrl Pts',(20.9068289285804,-47.6181557545822,-9.62369151535379));
#36863=CARTESIAN_POINT('Ctrl Pts',(15.2248621479926,-41.9477963710449,1.24768188077453));
#36864=CARTESIAN_POINT('Ctrl Pts',(15.254210762862,-41.9064969112026,0.765479302038377));
#36865=CARTESIAN_POINT('Ctrl Pts',(15.2808564144573,-41.8661102394704,0.33296638484066));
#36866=CARTESIAN_POINT('Ctrl Pts',(15.4297972934209,-41.7952733633443,-0.978922014777797));
#36867=CARTESIAN_POINT('Ctrl Pts',(15.6314258258188,-41.9273179171776,-1.98636136657411));
#36868=CARTESIAN_POINT('Ctrl Pts',(16.1668569942704,-42.5066521964322,-3.81078790530298));
#36869=CARTESIAN_POINT('Ctrl Pts',(16.5190077785595,-42.9706758457974,-4.65460264908077));
#36870=CARTESIAN_POINT('Ctrl Pts',(17.3244581615362,-44.1359912383599,-6.05121512495203));
#36871=CARTESIAN_POINT('Ctrl Pts',(17.7923352090986,-44.8534198776545,-6.61423873307417));
#36872=CARTESIAN_POINT('Ctrl Pts',(18.772833279635,-46.4073150662578,-7.37244739479018));
#36873=CARTESIAN_POINT('Ctrl Pts',(19.3108003965517,-47.275034523802,-7.56862230160965));
#36874=CARTESIAN_POINT('Ctrl Pts',(19.8275212310755,-48.1110813316864,-7.57037421505997));
#36875=CARTESIAN_POINT('Ctrl Pts',(11.6799141290245,-36.0076777827442,1.59647068126611));
#36876=CARTESIAN_POINT('Ctrl Pts',(11.7120656519303,-35.9738923911144,1.15259163659876));
#36877=CARTESIAN_POINT('Ctrl Pts',(11.7447913705197,-35.9261470465052,0.635573001855381));
#36878=CARTESIAN_POINT('Ctrl Pts',(11.9080080866776,-35.8791430893826,-1.86858636178463));
#36879=CARTESIAN_POINT('Ctrl Pts',(12.1266171429838,-36.1952232408468,-3.71029995873377));
#36880=CARTESIAN_POINT('Ctrl Pts',(12.7754415589391,-37.4975806516859,-7.16936247490142));
#36881=CARTESIAN_POINT('Ctrl Pts',(13.1874595938576,-38.4695778662026,-8.73699595770811));
#36882=CARTESIAN_POINT('Ctrl Pts',(14.1714247213063,-40.9286921018315,-11.3730256982117));
#36883=CARTESIAN_POINT('Ctrl Pts',(14.7293359257928,-42.3975559178223,-12.4235805192562));
#36884=CARTESIAN_POINT('Ctrl Pts',(15.9494910259804,-45.645686779583,-13.8529470821261));
#36885=CARTESIAN_POINT('Ctrl Pts',(16.5867336458242,-47.3851293552256,-14.2204718557262));
#36886=CARTESIAN_POINT('Ctrl Pts',(17.2320701170938,-49.1354594857183,-14.2198708430667));
#36887=CARTESIAN_POINT('Ctrl Pts',(10.8171551228315,-35.6055008474197,1.6296461228737));
#36888=CARTESIAN_POINT('Ctrl Pts',(10.8490384138683,-35.5719973186181,1.18947024665146));
#36889=CARTESIAN_POINT('Ctrl Pts',(10.8818072974792,-35.5230856250726,0.664243958035779));
#36890=CARTESIAN_POINT('Ctrl Pts',(11.0453235253478,-35.4754406456448,-1.95287905128153));
#36891=CARTESIAN_POINT('Ctrl Pts',(11.2678861931429,-35.8076256583718,-3.87337387082083));
#36892=CARTESIAN_POINT('Ctrl Pts',(11.9353671582668,-37.170412338562,-7.48792130210496));
#36893=CARTESIAN_POINT('Ctrl Pts',(12.3599059968312,-38.1870962603733,-9.12360836232141));
#36894=CARTESIAN_POINT('Ctrl Pts',(13.3771794921622,-40.758733259042,-11.8774049927098));
#36895=CARTESIAN_POINT('Ctrl Pts',(13.9538940421623,-42.2936801020862,-12.9732563609012));
#36896=CARTESIAN_POINT('Ctrl Pts',(15.2184820529382,-45.6900265604125,-14.4676858045336));
#36897=CARTESIAN_POINT('Ctrl Pts',(15.8774655646438,-47.5060156561953,-14.8501851005531));
#36898=CARTESIAN_POINT('Ctrl Pts',(16.5467173899495,-49.3366907261821,-14.8499483202528));
#36899=CARTESIAN_POINT('Ctrl Pts',(9.90333289917165,-35.8740691471583,1.62975530581346));
#36900=CARTESIAN_POINT('Ctrl Pts',(9.93521185458921,-35.840570174317,1.18963928644335));
#36901=CARTESIAN_POINT('Ctrl Pts',(9.96796916328224,-35.7915998643985,0.664246400104493));
#36902=CARTESIAN_POINT('Ctrl Pts',(10.1312860615024,-35.7432760306242,-1.95288623097023));
#36903=CARTESIAN_POINT('Ctrl Pts',(10.354154297206,-36.0765018635817,-3.87317034521659));
#36904=CARTESIAN_POINT('Ctrl Pts',(11.0212942781007,-37.4381269352451,-7.48823335801339));
#36905=CARTESIAN_POINT('Ctrl Pts',(11.446042279729,-38.4555234045924,-9.12349227713555));
#36906=CARTESIAN_POINT('Ctrl Pts',(12.4632402081669,-41.0269029710472,-11.8775764776338));
#36907=CARTESIAN_POINT('Ctrl Pts',(13.0400785026582,-42.5622713808391,-12.9726927515287));
#36908=CARTESIAN_POINT('Ctrl Pts',(14.3045284731933,-45.9581475303539,-14.4683433355075));
#36909=CARTESIAN_POINT('Ctrl Pts',(14.9636108093825,-47.7744493566741,-14.8498038984862));
#36910=CARTESIAN_POINT('Ctrl Pts',(15.6328286697383,-49.6050326655026,-14.8500516281495));
#36911=CARTESIAN_POINT('Ctrl Pts',(9.39535856987488,-36.6790985320905,1.59674363861551));
#36912=CARTESIAN_POINT('Ctrl Pts',(9.42749925373743,-36.6453245303473,1.15301423607977));
#36913=CARTESIAN_POINT('Ctrl Pts',(9.46019603502518,-36.5974326448213,0.635579107027166));
#36914=CARTESIAN_POINT('Ctrl Pts',(9.62291442707024,-36.5487315518261,-1.86860431100636));
#36915=CARTESIAN_POINT('Ctrl Pts',(9.8422874031409,-36.8674137538596,-3.70979114472798));
#36916=CARTESIAN_POINT('Ctrl Pts',(10.4902593585244,-38.1668671434055,-7.17014261466771));
#36917=CARTESIAN_POINT('Ctrl Pts',(10.9028003010987,-39.1406457267576,-8.73670574474347));
#36918=CARTESIAN_POINT('Ctrl Pts',(11.8865765113215,-41.5991163818375,-11.3734544105217));
#36919=CARTESIAN_POINT('Ctrl Pts',(12.4447970770368,-43.0690341146998,-12.4221714958274));
#36920=CARTESIAN_POINT('Ctrl Pts',(13.6646070766139,-46.3159892044412,-13.8545909095583));
#36921=CARTESIAN_POINT('Ctrl Pts',(14.3020974766102,-48.0562134772786,-14.2195188098913));
#36922=CARTESIAN_POINT('Ctrl Pts',(14.9473483165659,-49.8063143340195,-14.2201291128083));
#36923=CARTESIAN_POINT('Ctrl Pts',(11.7862169042728,-35.9142171164212,0.));
#36924=CARTESIAN_POINT('Ctrl Pts',(11.9080080866776,-35.8791430893826,-1.86858636178463));
#36925=CARTESIAN_POINT('Ctrl Pts',(12.1266171429838,-36.1952232408468,-3.71029995873257));
#36926=CARTESIAN_POINT('Ctrl Pts',(12.7754415589391,-37.4975806516859,-7.16936247490261));
#36927=CARTESIAN_POINT('Ctrl Pts',(13.1874595938576,-38.4695778662026,-8.73699595770572));
#36928=CARTESIAN_POINT('Ctrl Pts',(13.7294890038888,-39.8242114819216,-10.1890856763496));
#36929=CARTESIAN_POINT('Ctrl Pts',(13.7802180759825,-39.9517643117901,-10.3203928635163));
#36930=CARTESIAN_POINT('Ctrl Pts',(13.8316148870825,-40.0817049410147,-10.4488603765993));
#36931=CARTESIAN_POINT('Ctrl Pts',(9.50149509066468,-36.5850719698906,-1.49880108324396E-15));
#36932=CARTESIAN_POINT('Ctrl Pts',(9.62291442707024,-36.5487315518261,-1.86860431100636));
#36933=CARTESIAN_POINT('Ctrl Pts',(9.8422874031409,-36.8674137538596,-3.70979114472798));
#36934=CARTESIAN_POINT('Ctrl Pts',(10.4902593585244,-38.1668671434055,-7.17014261466771));
#36935=CARTESIAN_POINT('Ctrl Pts',(10.9028003010987,-39.1406457267576,-8.73670574474347));
#36936=CARTESIAN_POINT('Ctrl Pts',(11.447491770971,-40.5018374092138,-10.1966053555721));
#36937=CARTESIAN_POINT('Ctrl Pts',(11.5010595286631,-40.6365673070921,-10.3350231942278));
#36938=CARTESIAN_POINT('Ctrl Pts',(11.5553735590044,-40.7739629732814,-10.4702558450999));
#36939=CARTESIAN_POINT('Ctrl Pts',(15.7201209119704,-41.7419576204998,1.24689082988543));
#36940=CARTESIAN_POINT('Ctrl Pts',(15.7550797324069,-41.7052222707071,0.764254661705176));
#36941=CARTESIAN_POINT('Ctrl Pts',(15.7872856429791,-41.6694633881789,0.332948671129717));
#36942=CARTESIAN_POINT('Ctrl Pts',(15.9462356620245,-41.6254618648069,-0.978870002708));
#36943=CARTESIAN_POINT('Ctrl Pts',(16.124806376022,-41.7773170936442,-1.9878357708918));
#36944=CARTESIAN_POINT('Ctrl Pts',(16.5748099612742,-42.4353694480507,-3.80852727283301));
#36945=CARTESIAN_POINT('Ctrl Pts',(16.855823663794,-42.939624365945,-4.65544360722247));
#36946=CARTESIAN_POINT('Ctrl Pts',(17.4877814824343,-44.2095709903027,-6.04997283343079));
#36947=CARTESIAN_POINT('Ctrl Pts',(17.8478990309574,-44.9832291227579,-6.61832169904376));
#36948=CARTESIAN_POINT('Ctrl Pts',(18.5982747097764,-46.6642543902711,-7.36768403077276));
#36949=CARTESIAN_POINT('Ctrl Pts',(19.0065156677573,-47.597447725177,-7.57138648702772));
#36950=CARTESIAN_POINT('Ctrl Pts',(19.3992863750335,-48.4991757443116,-7.56962581969437));
#36951=CARTESIAN_POINT('Ctrl Pts',(14.0037398626871,-40.1090570584214,1.35489321026543));
#36952=CARTESIAN_POINT('Ctrl Pts',(14.0378295966279,-40.0732349601815,0.884255518285286));
#36953=CARTESIAN_POINT('Ctrl Pts',(14.0701900799508,-40.0337447201333,0.426396949026514));
#36954=CARTESIAN_POINT('Ctrl Pts',(14.2303553472453,-39.9884678119657,-1.25360819501712));
#36955=CARTESIAN_POINT('Ctrl Pts',(14.4214462185236,-40.191567831885,-2.51960912780892));
#36956=CARTESIAN_POINT('Ctrl Pts',(14.9326685312488,-41.0479784867153,-4.84647586781181));
#36957=CARTESIAN_POINT('Ctrl Pts',(15.2542422185937,-41.6970325717334,-5.91572199047102));
#36958=CARTESIAN_POINT('Ctrl Pts',(15.9948572088741,-43.3340488505992,-7.69376028691602));
#36959=CARTESIAN_POINT('Ctrl Pts',(16.4161147204243,-44.3225950330452,-8.41063186558551));
#36960=CARTESIAN_POINT('Ctrl Pts',(17.3114822382606,-46.487283787507,-9.37059840618065));
#36961=CARTESIAN_POINT('Ctrl Pts',(17.7905076322893,-47.6695948287687,-9.62435378637549));
#36962=CARTESIAN_POINT('Ctrl Pts',(18.2612298390044,-48.8333181822475,-9.62320046360547));
#36963=CARTESIAN_POINT('Ctrl Pts',(12.6395284821794,-38.1728270004197,1.47293192394286));
#36964=CARTESIAN_POINT('Ctrl Pts',(12.6726703074,-38.1380009815193,1.0153809158411));
#36965=CARTESIAN_POINT('Ctrl Pts',(12.7052063084752,-38.0944634070469,0.528580717871503));
#36966=CARTESIAN_POINT('Ctrl Pts',(12.8668122636039,-38.0481727007019,-1.55402875457849));
#36967=CARTESIAN_POINT('Ctrl Pts',(13.0714224335629,-38.3067247111899,-3.10121432125906));
#36968=CARTESIAN_POINT('Ctrl Pts',(13.6497783497158,-39.3806906392206,-5.98129145448502));
#36969=CARTESIAN_POINT('Ctrl Pts',(14.0155868029404,-40.187682027567,-7.29389406575976));
#36970=CARTESIAN_POINT('Ctrl Pts',(14.8750601592654,-42.2262312169631,-9.49113593804686));
#36971=CARTESIAN_POINT('Ctrl Pts',(15.3631044396506,-43.4495197173632,-10.370828601741));
#36972=CARTESIAN_POINT('Ctrl Pts',(16.4170971139165,-46.1433554687416,-11.560404556101));
#36973=CARTESIAN_POINT('Ctrl Pts',(16.9734434882197,-47.5979046271707,-11.8694761542236));
#36974=CARTESIAN_POINT('Ctrl Pts',(17.5294501945609,-49.0481649878424,-11.8687142284812));
#36975=CARTESIAN_POINT('Ctrl Pts',(11.6799141290245,-36.0076777827442,1.59647068126611));
#36976=CARTESIAN_POINT('Ctrl Pts',(11.7120656519303,-35.9738923911144,1.15259163659876));
#36977=CARTESIAN_POINT('Ctrl Pts',(11.7447913705197,-35.9261470465052,0.635573001855381));
#36978=CARTESIAN_POINT('Ctrl Pts',(11.9080080866776,-35.8791430893826,-1.86858636178463));
#36979=CARTESIAN_POINT('Ctrl Pts',(12.1266171429838,-36.1952232408468,-3.71029995873257));
#36980=CARTESIAN_POINT('Ctrl Pts',(12.7754415589391,-37.4975806516859,-7.16936247490261));
#36981=CARTESIAN_POINT('Ctrl Pts',(13.1874595938576,-38.4695778662026,-8.73699595770572));
#36982=CARTESIAN_POINT('Ctrl Pts',(14.1714247213063,-40.9286921018316,-11.3730256982141));
#36983=CARTESIAN_POINT('Ctrl Pts',(14.7293359257928,-42.3975559178223,-12.4235805192514));
#36984=CARTESIAN_POINT('Ctrl Pts',(15.9494910259804,-45.645686779583,-13.8529470821309));
#36985=CARTESIAN_POINT('Ctrl Pts',(16.5867336458133,-47.3851293552296,-14.2204718557262));
#36986=CARTESIAN_POINT('Ctrl Pts',(17.2320701170938,-49.1354594857183,-14.2198708430667));
#36987=CARTESIAN_POINT('Ctrl Pts',(9.39535856987487,-36.6790985320905,1.59674363861551));
#36988=CARTESIAN_POINT('Ctrl Pts',(9.42749925373742,-36.6453245303473,1.15301423607977));
#36989=CARTESIAN_POINT('Ctrl Pts',(9.46019603502516,-36.5974326448213,0.635579107027166));
#36990=CARTESIAN_POINT('Ctrl Pts',(9.62291442707023,-36.5487315518261,-1.86860431100636));
#36991=CARTESIAN_POINT('Ctrl Pts',(9.84228740314089,-36.8674137538596,-3.70979114472798));
#36992=CARTESIAN_POINT('Ctrl Pts',(10.4902593585244,-38.1668671434055,-7.17014261466771));
#36993=CARTESIAN_POINT('Ctrl Pts',(10.9028003010999,-39.1406457267528,-8.73670574474347));
#36994=CARTESIAN_POINT('Ctrl Pts',(11.8865765113203,-41.5991163818423,-11.3734544105217));
#36995=CARTESIAN_POINT('Ctrl Pts',(12.4447970770392,-43.069034114695,-12.4221714958274));
#36996=CARTESIAN_POINT('Ctrl Pts',(13.6646070766115,-46.3159892044461,-13.8545909095583));
#36997=CARTESIAN_POINT('Ctrl Pts',(14.3020974766134,-48.0562134772745,-14.2195188098913));
#36998=CARTESIAN_POINT('Ctrl Pts',(14.9473483165659,-49.8063143340195,-14.2201291128083));
#36999=CARTESIAN_POINT('Ctrl Pts',(9.75977978596898,-39.0191723737221,1.47327599461687));
#37000=CARTESIAN_POINT('Ctrl Pts',(9.79290794825892,-38.9843607121039,1.0159136147723));
#37001=CARTESIAN_POINT('Ctrl Pts',(9.82540747302648,-38.9406384185465,0.528588413618024));
#37002=CARTESIAN_POINT('Ctrl Pts',(9.98638527612132,-38.8922084230982,-1.55405138009428));
#37003=CARTESIAN_POINT('Ctrl Pts',(10.1919583891532,-39.154040393972,-3.10057294641215));
#37004=CARTESIAN_POINT('Ctrl Pts',(10.7692397539741,-40.2243457187397,-5.9822748433407));
#37005=CARTESIAN_POINT('Ctrl Pts',(11.1357073475001,-41.033582574293,-7.29352824388565));
#37006=CARTESIAN_POINT('Ctrl Pts',(11.9949425681694,-43.07132051169,-9.49167634237209));
#37007=CARTESIAN_POINT('Ctrl Pts',(12.4833768073745,-44.295937504943,-10.369052486749));
#37008=CARTESIAN_POINT('Ctrl Pts',(13.5369344722939,-46.9882911615219,-11.5624766483653));
#37009=CARTESIAN_POINT('Ctrl Pts',(14.0935974136572,-48.4438248433017,-11.8682745704593));
#37010=CARTESIAN_POINT('Ctrl Pts',(14.6494919462604,-49.8937970264263,-11.8690397849987));
#37011=CARTESIAN_POINT('Ctrl Pts',(9.6600835208205,-41.385638397964,1.35541218776066));
#37012=CARTESIAN_POINT('Ctrl Pts',(9.69415264633907,-41.3498379554702,0.885059012386701));
#37013=CARTESIAN_POINT('Ctrl Pts',(9.72645811078361,-41.3100690951929,0.426408556872093));
#37014=CARTESIAN_POINT('Ctrl Pts',(9.88567590770692,-41.2615653996831,-1.25364232211483));
#37015=CARTESIAN_POINT('Ctrl Pts',(10.0782192299531,-41.4696127334993,-2.51864171286793));
#37016=CARTESIAN_POINT('Ctrl Pts',(10.587820747883,-42.3205019333899,-4.847959158086));
#37017=CARTESIAN_POINT('Ctrl Pts',(10.9103886466144,-42.9729429590446,-5.9151702046465));
#37018=CARTESIAN_POINT('Ctrl Pts',(11.6506444460221,-44.6087355895318,-7.69457540341655));
#37019=CARTESIAN_POINT('Ctrl Pts',(12.0724901502524,-45.5992855983477,-8.40795287032041));
#37020=CARTESIAN_POINT('Ctrl Pts',(12.9672015236417,-47.7617388416025,-9.37372383746897));
#37021=CARTESIAN_POINT('Ctrl Pts',(13.446713417008,-48.9455328277857,-9.62254085987295));
#37022=CARTESIAN_POINT('Ctrl Pts',(13.9172574201599,-50.1088235664896,-9.62369151535376));
#37023=CARTESIAN_POINT('Ctrl Pts',(9.10010115416748,-43.6875520748215,1.24768178593761));
#37024=CARTESIAN_POINT('Ctrl Pts',(9.13502856600687,-43.6508497298264,0.76547923989595));
#37025=CARTESIAN_POINT('Ctrl Pts',(9.16715062416417,-43.6146662116234,0.332966362254671));
#37026=CARTESIAN_POINT('Ctrl Pts',(9.32465663565536,-43.5657468507608,-0.978922014663684));
#37027=CARTESIAN_POINT('Ctrl Pts',(9.50544098106106,-43.7251421134196,-1.9863613664906));
#37028=CARTESIAN_POINT('Ctrl Pts',(9.95297436776755,-44.3747794050744,-3.81078790538617));
#37029=CARTESIAN_POINT('Ctrl Pts',(10.2355033142436,-44.8841962446728,-4.65460264910923));
#37030=CARTESIAN_POINT('Ctrl Pts',(10.8669137022235,-46.1522779478823,-6.0512151249233));
#37031=CARTESIAN_POINT('Ctrl Pts',(11.2279276953183,-46.9289900443738,-6.61423873295882));
#37032=CARTESIAN_POINT('Ctrl Pts',(11.9773033665753,-48.6066082448324,-7.37244739490529));
#37033=CARTESIAN_POINT('Ctrl Pts',(12.3863053997921,-49.5420562727077,-7.5686223015431));
#37034=CARTESIAN_POINT('Ctrl Pts',(12.7787848949961,-50.4431303715412,-7.57037421505993));
#37035=CARTESIAN_POINT('Ctrl Pts',(6.43660260973332,-37.3033966274915,1.59647061166181));
#37036=CARTESIAN_POINT('Ctrl Pts',(6.44564064573105,-37.2962747755321,1.48695576755787));
#37037=CARTESIAN_POINT('Ctrl Pts',(6.45467756855567,-37.2891542935595,1.37746396776832));
#37038=CARTESIAN_POINT('Ctrl Pts',(6.49319539523223,-37.2588006588781,0.91069863508483));
#37039=CARTESIAN_POINT('Ctrl Pts',(6.52244162562218,-37.2305413795555,0.486448413028126));
#37040=CARTESIAN_POINT('Ctrl Pts',(6.68066728816074,-37.2086313911891,-1.86858636176938));
#37041=CARTESIAN_POINT('Ctrl Pts',(6.85206832383191,-37.5526056149563,-3.71029995872546));
#37042=CARTESIAN_POINT('Ctrl Pts',(7.30894385843816,-38.934044247035,-7.16936247490972));
#37043=CARTESIAN_POINT('Ctrl Pts',(7.57843851746451,-39.9547842114019,-8.73699595769907));
#37044=CARTESIAN_POINT('Ctrl Pts',(8.20241985394517,-42.5289010478592,-11.3730256982207));
#37045=CARTESIAN_POINT('Ctrl Pts',(8.54561121045842,-44.0622129909516,-12.423580519233));
#37046=CARTESIAN_POINT('Ctrl Pts',(9.29108967262444,-47.4509287397228,-13.8529470821493));
#37047=CARTESIAN_POINT('Ctrl Pts',(9.67429759303427,-49.2633553783165,-14.2204718555978));
#37048=CARTESIAN_POINT('Ctrl Pts',(10.0639675197015,-51.0877106274639,-14.2198708430667));
#37049=CARTESIAN_POINT('Ctrl Pts',(5.63986099173555,-36.7825298650421,1.62964605326942));
#37050=CARTESIAN_POINT('Ctrl Pts',(5.64889912474545,-36.77540793664,1.52013003366147));
#37051=CARTESIAN_POINT('Ctrl Pts',(5.65793595641857,-36.7682876225861,1.41064098633233));
#37052=CARTESIAN_POINT('Ctrl Pts',(5.69645375811678,-36.7379335980319,0.943868932617261));
#37053=CARTESIAN_POINT('Ctrl Pts',(5.72562619436981,-36.7087318569752,0.508392298457236));
#37054=CARTESIAN_POINT('Ctrl Pts',(5.88421645976751,-36.6862652424053,-1.95287905126922));
#37055=CARTESIAN_POINT('Ctrl Pts',(6.05723890413859,-37.0467430607592,-3.87337387081251));
#37056=CARTESIAN_POINT('Ctrl Pts',(6.52398110944683,-38.4906509831273,-7.48792130211325));
#37057=CARTESIAN_POINT('Ctrl Pts',(6.79950954687151,-39.5574047046894,-9.12360836231237));
#37058=CARTESIAN_POINT('Ctrl Pts',(7.44044656125075,-42.2476392596962,-11.8774049927188));
#37059=CARTESIAN_POINT('Ctrl Pts',(7.79284527703385,-43.8490375949744,-12.9732563608828));
#37060=CARTESIAN_POINT('Ctrl Pts',(8.56121110815365,-47.3907837817508,-14.4676858045521));
#37061=CARTESIAN_POINT('Ctrl Pts',(8.95504492393713,-49.2820718587611,-14.8501851004818));
#37062=CARTESIAN_POINT('Ctrl Pts',(9.35695250368037,-51.1893577615277,-14.8499483202528));
#37063=CARTESIAN_POINT('Ctrl Pts',(4.69711890654707,-36.9183140647621,1.62975523620918));
#37064=CARTESIAN_POINT('Ctrl Pts',(4.70615704022186,-36.9111921358362,1.52023920855111));
#37065=CARTESIAN_POINT('Ctrl Pts',(4.71519387290942,-36.9040718339574,1.41075017948988));
#37066=CARTESIAN_POINT('Ctrl Pts',(4.7537116674503,-36.8737177597449,0.943978082226359));
#37067=CARTESIAN_POINT('Ctrl Pts',(4.78287005804029,-36.8444185781148,0.508394167544101));
#37068=CARTESIAN_POINT('Ctrl Pts',(4.94136562987512,-36.8212933555072,-1.95288623096214));
#37069=CARTESIAN_POINT('Ctrl Pts',(5.11454240774922,-37.1828448868836,-3.87317034521066));
#37070=CARTESIAN_POINT('Ctrl Pts',(5.58111241368669,-38.6255544971264,-7.48823335801928));
#37071=CARTESIAN_POINT('Ctrl Pts',(5.8567464791066,-39.6930432805223,-9.1234922771265));
#37072=CARTESIAN_POINT('Ctrl Pts',(6.49764533218352,-42.3830122693035,-11.8775764776428));
#37073=CARTESIAN_POINT('Ctrl Pts',(6.85010653771311,-43.9848454910638,-12.9726927515343));
#37074=CARTESIAN_POINT('Ctrl Pts',(7.61840266556165,-47.5261065109322,-14.4683433355019));
#37075=CARTESIAN_POINT('Ctrl Pts',(8.01228979375816,-49.417718199511,-14.8498038985623));
#37076=CARTESIAN_POINT('Ctrl Pts',(8.4141768132259,-51.3249084414064,-14.8500516281495));
#37077=CARTESIAN_POINT('Ctrl Pts',(4.07974739676214,-37.6428571267913,1.59674356901121));
#37078=CARTESIAN_POINT('Ctrl Pts',(4.08878543442164,-37.6357352735241,1.48722870478182));
#37079=CARTESIAN_POINT('Ctrl Pts',(4.09782235978292,-37.6286148219883,1.37773695066217));
#37080=CARTESIAN_POINT('Ctrl Pts',(4.13634016856563,-37.5982610631587,0.910971509107631));
#37081=CARTESIAN_POINT('Ctrl Pts',(4.16555128479877,-37.5697581824064,0.486453085745287));
#37082=CARTESIAN_POINT('Ctrl Pts',(4.32354021342829,-37.5462016739366,-1.86860431100168));
#37083=CARTESIAN_POINT('Ctrl Pts',(4.4953270828591,-37.8928601802674,-3.70979114472205));
#37084=CARTESIAN_POINT('Ctrl Pts',(4.95177211903725,-39.2713030320329,-7.1701426146736));
#37085=CARTESIAN_POINT('Ctrl Pts',(5.22153084805404,-40.2938806509769,-8.73670574474158));
#37086=CARTESIAN_POINT('Ctrl Pts',(5.84541678127528,-42.8673335718846,-11.3734544105235));
#37087=CARTESIAN_POINT('Ctrl Pts',(6.18876436215572,-44.4017327311633,-12.4221714958474));
#37088=CARTESIAN_POINT('Ctrl Pts',(6.93406856614537,-47.7892355626883,-13.8545909095384));
#37089=CARTESIAN_POINT('Ctrl Pts',(7.31741049756817,-49.6024712046744,-14.2195188100245));
#37090=CARTESIAN_POINT('Ctrl Pts',(7.70702829356537,-51.4265873271607,-14.2201291128084));
#37091=CARTESIAN_POINT('Ctrl Pts',(6.55512420987355,-37.2260157227863,0.));
#37092=CARTESIAN_POINT('Ctrl Pts',(6.68066728816073,-37.2086313911891,-1.86858636176938));
#37093=CARTESIAN_POINT('Ctrl Pts',(6.85206832383192,-37.5526056149563,-3.71029995872546));
#37094=CARTESIAN_POINT('Ctrl Pts',(7.30894385843816,-38.934044247035,-7.16936247490972));
#37095=CARTESIAN_POINT('Ctrl Pts',(7.57843851746451,-39.9547842114019,-8.73699595769907));
#37096=CARTESIAN_POINT('Ctrl Pts',(7.92216638570706,-41.3727684379704,-10.1890856763497));
#37097=CARTESIAN_POINT('Ctrl Pts',(7.95422644863896,-41.5062424636377,-10.3203928635162));
#37098=CARTESIAN_POINT('Ctrl Pts',(7.98660763467823,-41.642175013475,-10.4488603765986));
#37099=CARTESIAN_POINT('Ctrl Pts',(4.198184970543,-37.5648924254994,-4.877668582392E-9));
#37100=CARTESIAN_POINT('Ctrl Pts',(4.32354021386282,-37.5462016743808,-1.86860431422771));
#37101=CARTESIAN_POINT('Ctrl Pts',(4.49532708316823,-37.8928601807419,-3.70979114625979));
#37102=CARTESIAN_POINT('Ctrl Pts',(4.72354960103335,-38.5820816060563,-5.4399668797283));
#37103=CARTESIAN_POINT('Ctrl Pts',(4.95177211909771,-39.2713030319724,-7.17014261470724));
#37104=CARTESIAN_POINT('Ctrl Pts',(5.22153084808902,-40.2938806509466,-8.73670574476508));
#37105=CARTESIAN_POINT('Ctrl Pts',(5.53347381467321,-41.5806071114236,-10.0550800776385));
#37106=CARTESIAN_POINT('Ctrl Pts',(5.56696037000555,-41.7187350432317,-10.196605355576));
#37107=CARTESIAN_POINT('Ctrl Pts',(5.60080882153369,-41.8597170717893,-10.3350231942299));
#37108=CARTESIAN_POINT('Ctrl Pts',(5.63501657134591,-42.0034439406511,-10.4702558451003));
#37109=CARTESIAN_POINT('Ctrl Pts',(9.61961280540157,-43.5542911395533,1.24689076028094));
#37110=CARTESIAN_POINT('Ctrl Pts',(9.62864982106753,-43.5471700916028,1.13738827963977));
#37111=CARTESIAN_POINT('Ctrl Pts',(9.63768771167183,-43.5400479046461,1.02786752738893));
#37112=CARTESIAN_POINT('Ctrl Pts',(9.67620576232687,-43.509698109946,0.561172897473927));
#37113=CARTESIAN_POINT('Ctrl Pts',(9.70615305455088,-43.4908467778853,0.254828874441861));
#37114=CARTESIAN_POINT('Ctrl Pts',(9.86000510220678,-43.4711606313058,-0.978870002685296));
#37115=CARTESIAN_POINT('Ctrl Pts',(10.0151469714872,-43.6468834551436,-1.9878357708895));
#37116=CARTESIAN_POINT('Ctrl Pts',(10.3669195547086,-44.3622799728645,-3.80852727283542));
#37117=CARTESIAN_POINT('Ctrl Pts',(10.5733099858207,-44.9013947224069,-4.65544360722759));
#37118=CARTESIAN_POINT('Ctrl Pts',(11.0181031366371,-46.2483520959844,-6.04997283342579));
#37119=CARTESIAN_POINT('Ctrl Pts',(11.2644521757028,-47.0653855748928,-6.61832169899626));
#37120=CARTESIAN_POINT('Ctrl Pts',(11.767955273083,-48.8360900223252,-7.36768403082038));
#37121=CARTESIAN_POINT('Ctrl Pts',(12.0392336678346,-49.817883540689,-7.57138648665654));
#37122=CARTESIAN_POINT('Ctrl Pts',(12.2996772587575,-50.7663303683513,-7.56962581969443));
#37123=CARTESIAN_POINT('Ctrl Pts',(8.15308801979152,-41.6937446593045,1.354893140661));
#37124=CARTESIAN_POINT('Ctrl Pts',(8.16212535086541,-41.6866233628175,1.24538683819019));
#37125=CARTESIAN_POINT('Ctrl Pts',(8.17116294315093,-41.6795017085853,1.13587503550903));
#37126=CARTESIAN_POINT('Ctrl Pts',(8.20968092097156,-41.649150702668,0.669158551024819));
#37127=CARTESIAN_POINT('Ctrl Pts',(8.23940452738148,-41.6273443121243,0.32635136887054));
#37128=CARTESIAN_POINT('Ctrl Pts',(8.39455851883134,-41.6066335880765,-1.25360819499889));
#37129=CARTESIAN_POINT('Ctrl Pts',(8.55480021408119,-41.8348614090738,-2.5196091278042));
#37130=CARTESIAN_POINT('Ctrl Pts',(8.93893907695026,-42.7553095590252,-4.84647586781658));
#37131=CARTESIAN_POINT('Ctrl Pts',(9.16486958068117,-43.4435219166315,-5.91572199046901));
#37132=CARTESIAN_POINT('Ctrl Pts',(9.66497447127398,-45.1692762327225,-7.69376028691809));
#37133=CARTESIAN_POINT('Ctrl Pts',(9.94125939865908,-46.2077116350436,-8.41063186554769));
#37134=CARTESIAN_POINT('Ctrl Pts',(10.5194460362019,-48.4777910626699,-9.37059840621854));
#37135=CARTESIAN_POINT('Ctrl Pts',(10.8253352376655,-49.7162403038184,-9.62435378615668));
#37136=CARTESIAN_POINT('Ctrl Pts',(11.1256510703081,-50.9351093861918,-9.62320046360551));
#37137=CARTESIAN_POINT('Ctrl Pts',(7.07831661167153,-39.5830751094924,1.47293185433849));
#37138=CARTESIAN_POINT('Ctrl Pts',(7.08735428726966,-39.5759535415238,1.36342137723571));
#37139=CARTESIAN_POINT('Ctrl Pts',(7.09639155277543,-39.5688324629961,1.25391935060785));
#37140=CARTESIAN_POINT('Ctrl Pts',(7.13490945496847,-39.5384801604726,0.787178992711653));
#37141=CARTESIAN_POINT('Ctrl Pts',(7.16439634167976,-39.5134970937345,0.404559744694547));
#37142=CARTESIAN_POINT('Ctrl Pts',(7.32102712268645,-39.4920354699275,-1.55402875456277));
#37143=CARTESIAN_POINT('Ctrl Pts',(7.48675886857651,-39.7770748569936,-3.10121432125195));
#37144=CARTESIAN_POINT('Ctrl Pts',(7.90638666805501,-40.9224179890928,-5.98129145449216));
#37145=CARTESIAN_POINT('Ctrl Pts',(8.15362486975768,-41.7732553395465,-7.29389406576022));
#37146=CARTESIAN_POINT('Ctrl Pts',(8.71423422838196,-43.9133708492413,-9.49113593804644));
#37147=CARTESIAN_POINT('Ctrl Pts',(9.02321881661921,-45.1936639793806,-10.3708286017129));
#37148=CARTESIAN_POINT('Ctrl Pts',(9.68311056585015,-48.0100791639764,-11.5604045561292));
#37149=CARTESIAN_POINT('Ctrl Pts',(10.0267902081664,-49.5289994535186,-11.8694761540572));
#37150=CARTESIAN_POINT('Ctrl Pts',(10.370743999114,-51.0436262593386,-11.8687142284812));
#37151=CARTESIAN_POINT('Ctrl Pts',(6.43660260973332,-37.3033966274915,1.59647061166181));
#37152=CARTESIAN_POINT('Ctrl Pts',(6.44564064573105,-37.2962747755321,1.48695576755787));
#37153=CARTESIAN_POINT('Ctrl Pts',(6.45467756855567,-37.2891542935595,1.37746396776832));
#37154=CARTESIAN_POINT('Ctrl Pts',(6.49319539523223,-37.2588006588781,0.91069863508483));
#37155=CARTESIAN_POINT('Ctrl Pts',(6.52244162562218,-37.2305413795555,0.486448413028126));
#37156=CARTESIAN_POINT('Ctrl Pts',(6.68066728816074,-37.2086313911891,-1.86858636176938));
#37157=CARTESIAN_POINT('Ctrl Pts',(6.85206832383192,-37.5526056149563,-3.71029995872546));
#37158=CARTESIAN_POINT('Ctrl Pts',(7.30894385843816,-38.934044247035,-7.16936247490972));
#37159=CARTESIAN_POINT('Ctrl Pts',(7.57843851746451,-39.9547842114019,-8.73699595769907));
#37160=CARTESIAN_POINT('Ctrl Pts',(8.20241985394517,-42.5289010478592,-11.3730256982207));
#37161=CARTESIAN_POINT('Ctrl Pts',(8.54561121045842,-44.0622129909516,-12.4235805192282));
#37162=CARTESIAN_POINT('Ctrl Pts',(9.29108967262445,-47.4509287397228,-13.8529470821541));
#37163=CARTESIAN_POINT('Ctrl Pts',(9.67429759302972,-49.2633553783174,-14.2204718555978));
#37164=CARTESIAN_POINT('Ctrl Pts',(10.0639675197015,-51.0877106274639,-14.2198708430667));
#37165=CARTESIAN_POINT('Ctrl Pts',(4.07974739676214,-37.6428571267913,1.59674356901121));
#37166=CARTESIAN_POINT('Ctrl Pts',(4.08878543442164,-37.6357352735241,1.48722870478183));
#37167=CARTESIAN_POINT('Ctrl Pts',(4.09782235978292,-37.6286148219883,1.37773695066217));
#37168=CARTESIAN_POINT('Ctrl Pts',(4.13634016856563,-37.5982610631587,0.910971509107631));
#37169=CARTESIAN_POINT('Ctrl Pts',(4.16555128479876,-37.5697581824064,0.486453085745287));
#37170=CARTESIAN_POINT('Ctrl Pts',(4.32354021342829,-37.5462016739366,-1.86860431100168));
#37171=CARTESIAN_POINT('Ctrl Pts',(4.4953270828591,-37.8928601802674,-3.70979114472325));
#37172=CARTESIAN_POINT('Ctrl Pts',(4.95177211903725,-39.2713030320329,-7.1701426146724));
#37173=CARTESIAN_POINT('Ctrl Pts',(5.22153084805404,-40.2938806509721,-8.73670574473919));
#37174=CARTESIAN_POINT('Ctrl Pts',(5.84541678127527,-42.8673335718894,-11.3734544105259));
#37175=CARTESIAN_POINT('Ctrl Pts',(6.18876436215512,-44.4017327311681,-12.4221714958474));
#37176=CARTESIAN_POINT('Ctrl Pts',(6.93406856614598,-47.7892355626836,-13.8545909095384));
#37177=CARTESIAN_POINT('Ctrl Pts',(7.31741049756717,-49.6024712046782,-14.2195188100435));
#37178=CARTESIAN_POINT('Ctrl Pts',(7.70702829356537,-51.4265873271607,-14.2201291128084));
#37179=CARTESIAN_POINT('Ctrl Pts',(4.10743210000891,-40.0109749372547,1.47327592501252));
#37180=CARTESIAN_POINT('Ctrl Pts',(4.1164697777016,-40.0038533676368,1.36376542254105));
#37181=CARTESIAN_POINT('Ctrl Pts',(4.12550704640513,-39.9967323274759,1.25426345348145));
#37182=CARTESIAN_POINT('Ctrl Pts',(4.16402492604217,-39.9663798684617,0.787522958349925));
#37183=CARTESIAN_POINT('Ctrl Pts',(4.19346755033784,-39.9410897350393,0.40456563479037));
#37184=CARTESIAN_POINT('Ctrl Pts',(4.34979992137194,-39.9175526247724,-1.55405138009188));
#37185=CARTESIAN_POINT('Ctrl Pts',(4.51601802193031,-40.2059756280632,-3.10057294641101));
#37186=CARTESIAN_POINT('Ctrl Pts',(4.93510316562684,-41.3475424919559,-5.98227484334182));
#37187=CARTESIAN_POINT('Ctrl Pts',(5.18267423522826,-42.200696259442,-7.29352824388607));
#37188=CARTESIAN_POINT('Ctrl Pts',(5.74316333527085,-44.3399748842863,-9.49167634237164));
#37189=CARTESIAN_POINT('Ctrl Pts',(6.05234484886441,-45.6216384820368,-10.3690524867785));
#37190=CARTESIAN_POINT('Ctrl Pts',(6.71201694059813,-48.4365247491788,-11.5624766483359));
#37191=CARTESIAN_POINT('Ctrl Pts',(7.05586981550236,-49.9564645931953,-11.8682745706448));
#37192=CARTESIAN_POINT('Ctrl Pts',(7.3997535864146,-51.4707901907297,-11.8690397849987));
#37193=CARTESIAN_POINT('Ctrl Pts',(3.67196736957011,-42.3391654916811,1.35541211815626));
#37194=CARTESIAN_POINT('Ctrl Pts',(3.68100470380343,-42.3320441927047,1.24590577742079));
#37195=CARTESIAN_POINT('Ctrl Pts',(3.69004230091196,-42.3249225963454,1.1363940615723));
#37196=CARTESIAN_POINT('Ctrl Pts',(3.72856024471116,-42.2945713543822,0.669677370090017));
#37197=CARTESIAN_POINT('Ctrl Pts',(3.75821708810019,-42.2723018011526,0.326360253170795));
#37198=CARTESIAN_POINT('Ctrl Pts',(3.91292097417106,-42.2484605261848,-1.25364232211669));
#37199=CARTESIAN_POINT('Ctrl Pts',(4.07389626035863,-42.4817920098941,-2.51864171287277));
#37200=CARTESIAN_POINT('Ctrl Pts',(4.45721661075379,-43.39654424225,-4.84795915808115));
#37201=CARTESIAN_POINT('Ctrl Pts',(4.68364919432174,-44.0882505573296,-5.91517020464685));
#37202=CARTESIAN_POINT('Ctrl Pts',(5.18357269341173,-45.8127425618315,-7.6945754034162));
#37203=CARTESIAN_POINT('Ctrl Pts',(5.46015465229401,-46.8532451029695,-8.40795287035928));
#37204=CARTESIAN_POINT('Ctrl Pts',(6.03800997041407,-49.1210183946462,-9.37372383743011));
#37205=CARTESIAN_POINT('Ctrl Pts',(6.34416967429075,-50.3610047224884,-9.62254086013458));
#37206=CARTESIAN_POINT('Ctrl Pts',(6.64437068472131,-51.5794202324977,-9.62369151535376));
#37207=CARTESIAN_POINT('Ctrl Pts',(2.79008834334054,-44.5379552064474,1.24768171633317));
#37208=CARTESIAN_POINT('Ctrl Pts',(2.79912536382142,-44.530834154704,1.13817917737408));
#37209=CARTESIAN_POINT('Ctrl Pts',(2.8081632617768,-44.5237120559476,1.02865855746206));
#37210=CARTESIAN_POINT('Ctrl Pts',(2.84668126057998,-44.4933619015011,0.56196361206819));
#37211=CARTESIAN_POINT('Ctrl Pts',(2.8765268015416,-44.473804678848,0.254842414703475));
#37212=CARTESIAN_POINT('Ctrl Pts',(3.02969285881099,-44.449347365471,-0.978922014671594));
#37213=CARTESIAN_POINT('Ctrl Pts',(3.18595276923174,-44.632848509077,-1.98636136649783));
#37214=CARTESIAN_POINT('Ctrl Pts',(3.53647788527045,-45.3395640713789,-3.81078790537893));
#37215=CARTESIAN_POINT('Ctrl Pts',(3.74363351928522,-45.8840038433848,-4.65460264911906));
#37216=CARTESIAN_POINT('Ctrl Pts',(4.18815021744348,-47.2290373705203,-6.05121512491345));
#37217=CARTESIAN_POINT('Ctrl Pts',(4.43495195217142,-48.0492213058189,-6.61423873300717));
#37218=CARTESIAN_POINT('Ctrl Pts',(4.93795009682242,-49.8164110494284,-7.37244739485694));
#37219=CARTESIAN_POINT('Ctrl Pts',(5.2096609439022,-50.8005446234324,-7.56862230191897));
#37220=CARTESIAN_POINT('Ctrl Pts',(5.46990934942727,-51.7483027430073,-7.57037421505991));
#37858=UNCERTAINTY_MEASURE_WITH_UNIT(LENGTH_MEASURE(0.01),#37882,
'DISTANCE_ACCURACY_VALUE',
'Maximum model space distance between geometric entities at asserted c
onnectivities');
#37867=UNCERTAINTY_MEASURE_WITH_UNIT(LENGTH_MEASURE(0.01),#37882,
'DISTANCE_ACCURACY_VALUE',
'Maximum model space distance between geometric entities at asserted c
onnectivities');
#37872=(
GEOMETRIC_REPRESENTATION_CONTEXT(3)
GLOBAL_UNCERTAINTY_ASSIGNED_CONTEXT((#37858))
GLOBAL_UNIT_ASSIGNED_CONTEXT((#37882,#37884,#37885))
REPRESENTATION_CONTEXT('','3D')
);
#37881=(
GEOMETRIC_REPRESENTATION_CONTEXT(3)
GLOBAL_UNCERTAINTY_ASSIGNED_CONTEXT((#37867))
GLOBAL_UNIT_ASSIGNED_CONTEXT((#37882,#37884,#37885))
REPRESENTATION_CONTEXT('','3D')
);
#37882=(
LENGTH_UNIT()
NAMED_UNIT(*)
SI_UNIT(.MILLI.,.METRE.)
);
#37884=(
NAMED_UNIT(*)
PLANE_ANGLE_UNIT()
SI_UNIT($,.RADIAN.)
);
#37885=(
NAMED_UNIT(*)
SI_UNIT($,.STERADIAN.)
SOLID_ANGLE_UNIT()
);
#37890=SHAPE_DEFINITION_REPRESENTATION(#37903,#37957);
#37903=PRODUCT_DEFINITION_SHAPE('',$,#37971);
#37957=SHAPE_REPRESENTATION('',(#11110),#37872);
#37966=PRODUCT_DEFINITION_CONTEXT('part definition',#38007,'design');
#37971=PRODUCT_DEFINITION('PS05','Worm_Wheel',#37984,#37966);
#37984=PRODUCT_DEFINITION_FORMATION('',$,#38013);
#38007=APPLICATION_CONTEXT(
'Core Data for Automotive Mechanical Design Process');
#38008=PRODUCT_CONTEXT('part definition',#38007,'mechanical');
#38013=PRODUCT('PS05','Worm_Wheel',$,(#38008));
#38023=PRESENTATION_STYLE_ASSIGNMENT((#38025));
#38025=SURFACE_STYLE_USAGE(.BOTH.,#38027);
#38027=SURFACE_SIDE_STYLE('',(#38029));
#38029=SURFACE_STYLE_FILL_AREA(#38031);
#38031=FILL_AREA_STYLE('Opaque(202,209,238)',(#38033));
#38033=FILL_AREA_STYLE_COLOUR('Opaque(202,209,238)',#38035);
#38035=COLOUR_RGB('Opaque(202,209,238)', 0.66274510, 0.83137255, 0.94901961);
ENDSEC;
END-ISO-10303-21;
